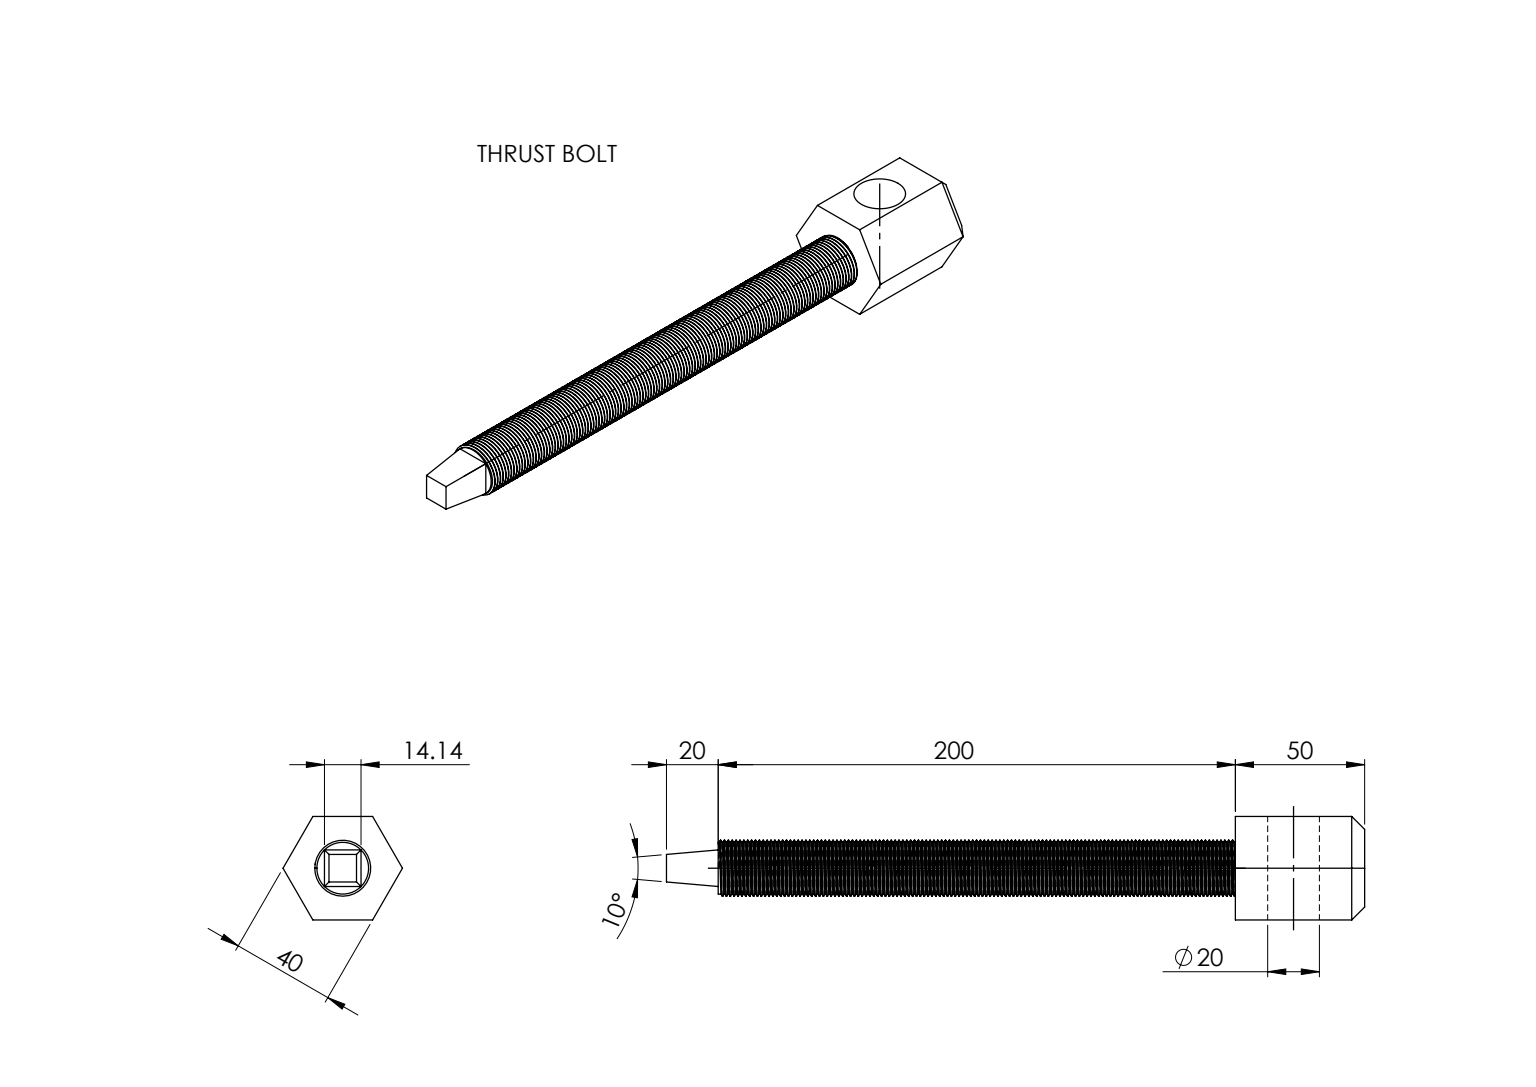
ISO-10303-21;
HEADER;
FILE_DESCRIPTION (('STEP AP203'),
    '1' );
FILE_NAME ('thrust bolt.step',
    '2026-09-28T05:57:06',
    ( '' ),
    ( '' ),
    'SwSTEP 2.0',
    'SolidWorks 2026',
    '' );
FILE_SCHEMA (( 'AUTOMOTIVE_DESIGN' ));
ENDSEC;

DATA;
#2=CARTESIAN_POINT ( 'NONE',  ( 10.81189881249999551, -6.242252689847874514, -42.15625000204836681 ) ) ;
#4=CARTESIAN_POINT ( 'NONE',  ( -10.81189881249999729, 1.324075727343319199E-15, -105.5937500020483810 ) ) ;
#5=CARTESIAN_POINT ( 'NONE',  ( 10.81189881249999729, 6.242252689847867408, -121.4062500020483810 ) ) ;
#6=VERTEX_POINT ( 'NONE', #18708 ) ;
#9=CARTESIAN_POINT ( 'NONE',  ( -5.000000000000003553, -8.660254037844383745, -26.49999999999996803 ) ) ;
#12=CARTESIAN_POINT ( 'NONE',  ( -2.293366432827344421E-15, -12.48450537969573659, -130.7187500020483810 ) ) ;
#14=CARTESIAN_POINT ( 'NONE',  ( -9.999999999999998224, 1.224646799147353059E-15, -200.0000000000000000 ) ) ;
#16=CARTESIAN_POINT ( 'NONE',  ( 5.000000000000000000, 8.660254037844385522, -194.1250000040967905 ) ) ;
#18=CARTESIAN_POINT ( 'NONE',  ( -2.293366432827344421E-15, -12.48450537969573659, -186.4062500020484094 ) ) ;
#19=CARTESIAN_POINT ( 'NONE',  ( 9.999999999999998224, 0.000000000000000000, -46.99999999999998579 ) ) ;
#20=CYLINDRICAL_SURFACE ( 'NONE', #32104, 9.999999999999998224 ) ;
#23=CARTESIAN_POINT ( 'NONE',  ( 5.405949406249999534, 9.363379034771803333, -58.09375000204835970 ) ) ;
#24=CARTESIAN_POINT ( 'NONE',  ( 7.644554776091147741E-16, 12.48450537969573659, -50.46875000204835970 ) ) ;
#26=CARTESIAN_POINT ( 'NONE',  ( 10.81189881249999551, -6.242252689847874514, -15.15625000204837036 ) ) ;
#30=CARTESIAN_POINT ( 'NONE',  ( 7.070501591499377789E-16, 11.54700538379251284, -105.1249999999999858 ) ) ;
#33=CARTESIAN_POINT ( 'NONE',  ( -5.000000000000003553, -8.660254037844383745, -27.99999999999996803 ) ) ;
#36=CARTESIAN_POINT ( 'NONE',  ( 10.81189881249999729, 6.242252689847867408, -113.9062500020483952 ) ) ;
#40=DIRECTION ( 'NONE',  ( -0.000000000000000000, -0.000000000000000000, 1.000000000000000000 ) ) ;
#42=ORIENTED_EDGE ( 'NONE', *, *, #41503, .T. ) ;
#43=CARTESIAN_POINT ( 'NONE',  ( 5.000000000000000000, 8.660254037844385522, -30.24999999999997158 ) ) ;
#44=CARTESIAN_POINT ( 'NONE',  ( 5.000000000000000000, 8.660254037844385522, -18.62500000409675494 ) ) ;
#45=CARTESIAN_POINT ( 'NONE',  ( -10.81189881249999729, 6.242252689847871849, -45.90625000204838102 ) ) ;
#46=CARTESIAN_POINT ( 'NONE',  ( 5.000000000000000000, 8.660254037844385522, -111.6250000040967763 ) ) ;
#48=CARTESIAN_POINT ( 'NONE',  ( 0.000000000000000000, 0.000000000000000000, -200.0000000000000000 ) ) ;
#49=CARTESIAN_POINT ( 'NONE',  ( -5.405949406250003975, -9.363379034771801557, -140.0312500020484094 ) ) ;
#50=CARTESIAN_POINT ( 'NONE',  ( -5.405949406250003975, -9.363379034771801557, -140.0312500020484094 ) ) ;
#51=CARTESIAN_POINT ( 'NONE',  ( -2.121150477449813534E-15, -11.54700538379251284, -123.8749999999999858 ) ) ;
#52=EDGE_LOOP ( 'NONE', ( #2862, #11579, #9941, #38309 ) ) ;
#53=ORIENTED_EDGE ( 'NONE', *, *, #4042, .F. ) ;
#54=ADVANCED_FACE ( 'NONE', ( #19135 ), #5555, .T. ) ;
#57=DIRECTION ( 'NONE',  ( -0.000000000000000000, -0.000000000000000000, 1.000000000000000000 ) ) ;
#58=CARTESIAN_POINT ( 'NONE',  ( -2.293366432827344421E-15, -12.48450537969573659, -177.2187500020484094 ) ) ;
#59=CARTESIAN_POINT ( 'NONE',  ( -10.81189881249999729, 1.324075727343319199E-15, -23.09375000204835615 ) ) ;
#60=CARTESIAN_POINT ( 'NONE',  ( -5.000000000000003553, -8.660254037844383745, -128.8750000040967905 ) ) ;
#61=CARTESIAN_POINT ( 'NONE',  ( 5.405949406249992428, -9.363379034771808662, -157.5937500020483810 ) ) ;
#62=CARTESIAN_POINT ( 'NONE',  ( 5.405949406249999534, 9.363379034771803333, -146.5937500020483810 ) ) ;
#63=CARTESIAN_POINT ( 'NONE',  ( 9.999999999999998224, 0.000000000000000000, -173.3750000040968189 ) ) ;
#66=CARTESIAN_POINT ( 'NONE',  ( 5.405949406249999534, 9.363379034771803333, -16.09375000204835260 ) ) ;
#72=CARTESIAN_POINT ( 'NONE',  ( -2.121150477449813534E-15, -11.54700538379251284, -17.37499999999997158 ) ) ;
#73=CARTESIAN_POINT ( 'NONE',  ( -5.405949406249996869, 9.363379034771805109, -72.84375000204838102 ) ) ;
#74=CARTESIAN_POINT ( 'NONE',  ( -5.405949406250003975, -9.363379034771801557, -39.53125000204838102 ) ) ;
#76=CARTESIAN_POINT ( 'NONE',  ( -2.121150477449813534E-15, -11.54700538379251284, -16.25000000409675849 ) ) ;
#78=VECTOR ( 'NONE', #7244, 1000.000000000000000 ) ;
#79=CARTESIAN_POINT ( 'NONE',  ( -5.000000000000003553, -8.660254037844383745, -130.0000000000000000 ) ) ;
#80=CARTESIAN_POINT ( 'NONE',  ( 7.644554776091147741E-16, 12.48450537969573659, -137.6562500020484094 ) ) ;
#82=CARTESIAN_POINT ( 'NONE',  ( -4.999999999999996447, 8.660254037844387298, -112.8750000040967763 ) ) ;
#85=( BOUNDED_CURVE ( )  B_SPLINE_CURVE ( 2, ( #33505, #9757, #39954, #703, #26171, #36305, #278 ),
 .UNSPECIFIED., .F., .F. ) 
 B_SPLINE_CURVE_WITH_KNOTS ( ( 3, 2, 2, 3 ),
 ( 0.9440298507462689948, 0.9452736318407963800, 0.9465174129353237653, 0.9477611940298510396 ),
 .UNSPECIFIED. ) 
 CURVE ( )  GEOMETRIC_REPRESENTATION_ITEM ( )  RATIONAL_B_SPLINE_CURVE ( ( 0.9999999999999641398, 0.8660254037844745678, 1.000000000000000000, 0.8660254037844387076, 1.000000000000000000, 0.8660254037844028474, 1.000000000000035971 ) ) 
 REPRESENTATION_ITEM ( '' )  );
#89=CARTESIAN_POINT ( 'NONE',  ( -10.81189881249999729, 1.324075727343319199E-15, -171.7812500020484094 ) ) ;
#90=CARTESIAN_POINT ( 'NONE',  ( 5.000000000000000000, 8.660254037844385522, -42.62500000409677625 ) ) ;
#93=CARTESIAN_POINT ( 'NONE',  ( 7.070501591499376803E-16, 11.54700538379251284, -101.0000000040967905 ) ) ;
#94=CARTESIAN_POINT ( 'NONE',  ( -10.81189881249999729, 1.324075727343319199E-15, -164.2812500020484094 ) ) ;
#95=CARTESIAN_POINT ( 'NONE',  ( 5.405949406249999534, 9.363379034771803333, -134.5937500020483810 ) ) ;
#96=DIRECTION ( 'NONE',  ( -0.000000000000000000, -0.000000000000000000, 1.000000000000000000 ) ) ;
#97=CARTESIAN_POINT ( 'NONE',  ( -9.999999999999998224, 1.224646799147353059E-15, -196.2500000000000000 ) ) ;
#98=ORIENTED_EDGE ( 'NONE', *, *, #19816, .T. ) ;
#100=VECTOR ( 'NONE', #1628, 1000.000000000000000 ) ;
#102=CARTESIAN_POINT ( 'NONE',  ( 5.405949406249999534, 9.363379034771803333, -70.28125000204838102 ) ) ;
#103=ORIENTED_EDGE ( 'NONE', *, *, #9830, .F. ) ;
#105=EDGE_CURVE ( 'NONE', #39394, #30784, #41849, .T. ) ;
#106=CARTESIAN_POINT ( 'NONE',  ( -2.293366432827344421E-15, -12.48450537969573659, -121.7187500020483952 ) ) ;
#107=VERTEX_POINT ( 'NONE', #25626 ) ;
#109=EDGE_CURVE ( 'NONE', #35866, #23028, #3547, .T. ) ;
#110=CARTESIAN_POINT ( 'NONE',  ( 10.81189881249999551, -6.242252689847874514, -23.96875000204836681 ) ) ;
#111=CARTESIAN_POINT ( 'NONE',  ( 10.81189881249999551, -6.242252689847874514, -197.9687500020484094 ) ) ;
#112=AXIS2_PLACEMENT_3D ( 'NONE', #13766, #17434, #17222 ) ;
#113=CARTESIAN_POINT ( 'NONE',  ( 10.81189881249999907, 6.242252689847868297, -50.71875000204835970 ) ) ;
#114=ADVANCED_FACE ( 'NONE', ( #26883 ), #29920, .T. ) ;
#117=CARTESIAN_POINT ( 'NONE',  ( -5.405949406249996869, 9.363379034771805109, -182.3437500020483810 ) ) ;
#118=CARTESIAN_POINT ( 'NONE',  ( 10.81189881249999729, 0.000000000000000000, -166.3437500020484094 ) ) ;
#123=FACE_OUTER_BOUND ( 'NONE', #11010, .T. ) ;
#125=CARTESIAN_POINT ( 'NONE',  ( 5.405949406249992428, -9.363379034771808662, -99.09375000204838102 ) ) ;
#127=CARTESIAN_POINT ( 'NONE',  ( -5.405949406250003975, -9.363379034771801557, -63.53125000204837391 ) ) ;
#129=CARTESIAN_POINT ( 'NONE',  ( 7.644554776091147741E-16, 12.48450537969573659, -164.6562500020484094 ) ) ;
#131=CARTESIAN_POINT ( 'NONE',  ( -9.999999999999998224, 1.224646799147353059E-15, -136.6250000040967620 ) ) ;
#137=ADVANCED_FACE ( 'NONE', ( #29707 ), #23658, .T. ) ;
#139=CARTESIAN_POINT ( 'NONE',  ( -10.81189881249999729, 1.324075727343319199E-15, -195.7812500020484094 ) ) ;
#140=LINE ( 'NONE', #33368, #22679 ) ;
#143=CARTESIAN_POINT ( 'NONE',  ( -4.999999999999996447, 8.660254037844387298, -58.49999999999997158 ) ) ;
#145=CARTESIAN_POINT ( 'NONE',  ( -5.000000000000003553, -8.660254037844383745, -62.87500000409676204 ) ) ;
#146=CARTESIAN_POINT ( 'NONE',  ( 7.070501591499376803E-16, 11.54700538379251284, -102.1250000000000000 ) ) ;
#147=CARTESIAN_POINT ( 'NONE',  ( 9.999999999999998224, 0.000000000000000000, -144.5000000000000000 ) ) ;
#149=CARTESIAN_POINT ( 'NONE',  ( -10.81189881249999729, -6.242252689847864744, -62.15625000204838813 ) ) ;
#152=CARTESIAN_POINT ( 'NONE',  ( 9.999999999999998224, 0.000000000000000000, -200.0000000000000000 ) ) ;
#153=CARTESIAN_POINT ( 'NONE',  ( -10.81189881249999907, -6.242252689847864744, -188.1562500020484094 ) ) ;
#155=CARTESIAN_POINT ( 'NONE',  ( 7.644554776091147741E-16, 12.48450537969573659, -0.9687500020483524876 ) ) ;
#157=( BOUNDED_CURVE ( )  B_SPLINE_CURVE ( 2, ( #19226, #13579, #9933, #13155, #20069, #32416, #9303 ),
 .UNSPECIFIED., .F., .F. ) 
 B_SPLINE_CURVE_WITH_KNOTS ( ( 3, 2, 2, 3 ),
 ( 0.3955223880597015795, 0.3967661691542289648, 0.3980099502487563501, 0.3992537313432836799 ),
 .UNSPECIFIED. ) 
 CURVE ( )  GEOMETRIC_REPRESENTATION_ITEM ( )  RATIONAL_B_SPLINE_CURVE ( ( 0.9999999999999880096, 0.8660254037844506980, 1.000000000000000000, 0.8660254037844387076, 1.000000000000000000, 0.8660254037844267172, 1.000000000000011990 ) ) 
 REPRESENTATION_ITEM ( '' )  );
#160=CARTESIAN_POINT ( 'NONE',  ( -10.00000000000000000, -5.773502691896251982, -167.6249999999999716 ) ) ;
#162=CARTESIAN_POINT ( 'NONE',  ( -2.293366432827344421E-15, -12.48450537969573659, -94.90625000204838102 ) ) ;
#163=ORIENTED_EDGE ( 'NONE', *, *, #36914, .F. ) ;
#164=CYLINDRICAL_SURFACE ( 'NONE', #41388, 9.999999999999998224 ) ;
#166=ORIENTED_EDGE ( 'NONE', *, *, #11173, .F. ) ;
#167=ORIENTED_EDGE ( 'NONE', *, *, #19593, .F. ) ;
#169=CARTESIAN_POINT ( 'NONE',  ( 10.81189881249999729, 0.000000000000000000, -31.34375000204836681 ) ) ;
#170=CARTESIAN_POINT ( 'NONE',  ( 10.81189881249999551, -6.242252689847874514, -22.65625000204837391 ) ) ;
#172=CARTESIAN_POINT ( 'NONE',  ( 5.405949406249999534, 9.363379034771803333, -71.59375000204836681 ) ) ;
#173=CARTESIAN_POINT ( 'NONE',  ( 0.000000000000000000, 0.000000000000000000, -200.0000000000000000 ) ) ;
#174=CARTESIAN_POINT ( 'NONE',  ( 5.405949406249992428, -9.363379034771808662, -192.0937500020484094 ) ) ;
#175=CARTESIAN_POINT ( 'NONE',  ( -2.293366432827344421E-15, -12.48450537969573659, -150.2187500020483810 ) ) ;
#176=CARTESIAN_POINT ( 'NONE',  ( 5.000000000000000000, 8.660254037844385522, -99.24999999999998579 ) ) ;
#179=CARTESIAN_POINT ( 'NONE',  ( -10.00000000000000000, -5.773502691896251982, -4.096743805827756695E-09 ) ) ;
#180=VECTOR ( 'NONE', #38036, 1000.000000000000000 ) ;
#181=CARTESIAN_POINT ( 'NONE',  ( -10.00000000000154188, 5.773502691895366468, -49.75000000409671230 ) ) ;
#182=ADVANCED_FACE ( 'NONE', ( #33380 ), #3374, .T. ) ;
#183=CARTESIAN_POINT ( 'NONE',  ( -10.81189881249999907, -6.242252689847864744, -123.4687500020483810 ) ) ;
#184=DIRECTION ( 'NONE',  ( -0.000000000000000000, -0.000000000000000000, 1.000000000000000000 ) ) ;
#185=CARTESIAN_POINT ( 'NONE',  ( 5.405949406249999534, 9.363379034771803333, -91.28125000204838102 ) ) ;
#186=CARTESIAN_POINT ( 'NONE',  ( 5.405949406249999534, 9.363379034771803333, -106.0937500020483810 ) ) ;
#189=CARTESIAN_POINT ( 'NONE',  ( 10.00000000000000000, 5.773502691896255534, -161.2500000040967905 ) ) ;
#195=FACE_OUTER_BOUND ( 'NONE', #14094, .T. ) ;
#197=CARTESIAN_POINT ( 'NONE',  ( 10.00000000000000000, 5.773502691896255534, -81.37499999999998579 ) ) ;
#199=CARTESIAN_POINT ( 'NONE',  ( -9.999999999999998224, 5.773502691896259087, -91.75000000409677625 ) ) ;
#202=CARTESIAN_POINT ( 'NONE',  ( -2.293366432827344421E-15, -12.48450537969573659, -84.40625000204838102 ) ) ;
#203=ORIENTED_EDGE ( 'NONE', *, *, #41316, .F. ) ;
#204=( BOUNDED_CURVE ( )  B_SPLINE_CURVE ( 2, ( #13200, #12782, #19064, #9770, #9143, #32665, #29001 ),
 .UNSPECIFIED., .F., .F. ) 
 B_SPLINE_CURVE_WITH_KNOTS ( ( 3, 2, 2, 3 ),
 ( 0.5373134328358210032, 0.5385572139303483885, 0.5398009950248757738, 0.5410447761194030480 ),
 .UNSPECIFIED. ) 
 CURVE ( )  GEOMETRIC_REPRESENTATION_ITEM ( )  RATIONAL_B_SPLINE_CURVE ( ( 0.9999999999999880096, 0.8660254037844506980, 1.000000000000000000, 0.8660254037844387076, 1.000000000000000000, 0.8660254037844267172, 1.000000000000011990 ) ) 
 REPRESENTATION_ITEM ( '' )  );
#209=CARTESIAN_POINT ( 'NONE',  ( 5.000000000000000000, 8.660254037844385522, -7.749999999999978684 ) ) ;
#210=CARTESIAN_POINT ( 'NONE',  ( -5.000000000000003553, -8.660254037844383745, -142.0000000000000000 ) ) ;
#211=CARTESIAN_POINT ( 'NONE',  ( -9.999999999999998224, 1.224646799147353059E-15, -200.0000000000000000 ) ) ;
#213=VECTOR ( 'NONE', #33847, 1000.000000000000000 ) ;
#214=CARTESIAN_POINT ( 'NONE',  ( 10.00000000000000000, 5.773502691896255534, -189.3750000000000000 ) ) ;
#216=CARTESIAN_POINT ( 'NONE',  ( 5.405949406249992428, -9.363379034771808662, -115.7812500020483952 ) ) ;
#217=ORIENTED_EDGE ( 'NONE', *, *, #1701, .T. ) ;
#219=CARTESIAN_POINT ( 'NONE',  ( -5.405949406249996869, 9.363379034771805109, -47.53125000204838813 ) ) ;
#221=CARTESIAN_POINT ( 'NONE',  ( -10.81189881249999907, -6.242252689847864744, -91.96875000204838102 ) ) ;
#222=CARTESIAN_POINT ( 'NONE',  ( -10.81189881249999729, -6.242252689847864744, -120.6562500020483810 ) ) ;
#224=CARTESIAN_POINT ( 'NONE',  ( -9.999999999999998224, 1.224646799147353059E-15, -112.2499999999999858 ) ) ;
#225=CARTESIAN_POINT ( 'NONE',  ( 4.999999999999992006, -8.660254037844389075, -116.2499999999999858 ) ) ;
#228=CARTESIAN_POINT ( 'NONE',  ( -10.81189881249999729, 6.242252689847871849, -129.7187500020483810 ) ) ;
#230=CYLINDRICAL_SURFACE ( 'NONE', #27006, 9.999999999999998224 ) ;
#232=CARTESIAN_POINT ( 'NONE',  ( 5.000000000000000000, 8.660254037844385522, -189.6250000040967905 ) ) ;
#234=CARTESIAN_POINT ( 'NONE',  ( -2.293366432827344421E-15, -12.48450537969573659, -189.4062500020484094 ) ) ;
#239=CARTESIAN_POINT ( 'NONE',  ( 5.405949406249999534, 9.363379034771803333, -64.09375000204836681 ) ) ;
#240=CARTESIAN_POINT ( 'NONE',  ( 5.405949406249992428, -9.363379034771808662, -51.09375000204835260 ) ) ;
#242=CARTESIAN_POINT ( 'NONE',  ( 10.81189881249999729, 0.000000000000000000, -18.03125000204835970 ) ) ;
#244=CARTESIAN_POINT ( 'NONE',  ( -5.000000000000003553, -8.660254037844383745, -124.3750000040967763 ) ) ;
#246=CARTESIAN_POINT ( 'NONE',  ( 9.999999999999998224, 0.000000000000000000, -108.4999999999999858 ) ) ;
#248=FACE_OUTER_BOUND ( 'NONE', #19771, .T. ) ;
#251=CARTESIAN_POINT ( 'NONE',  ( 5.405949406249999534, 9.363379034771803333, -112.2812500020483952 ) ) ;
#252=EDGE_CURVE ( 'NONE', #311, #38192, #33161, .T. ) ;
#258=VERTEX_POINT ( 'NONE', #36387 ) ;
#259=CARTESIAN_POINT ( 'NONE',  ( -4.999999999999996447, 8.660254037844387298, -35.99999999999997868 ) ) ;
#260=CARTESIAN_POINT ( 'NONE',  ( -5.000000000000003553, -8.660254037844383745, -20.87500000409675494 ) ) ;
#261=CARTESIAN_POINT ( 'NONE',  ( -10.81189881249999729, 6.242252689847871849, -39.90625000204835970 ) ) ;
#262=CARTESIAN_POINT ( 'NONE',  ( 9.999999999999998224, 0.000000000000000000, -35.37500000409676915 ) ) ;
#264=LINE ( 'NONE', #16194, #5231 ) ;
#265=CARTESIAN_POINT ( 'NONE',  ( 5.405949406249992428, -9.363379034771808662, -145.7812500020483810 ) ) ;
#266=CARTESIAN_POINT ( 'NONE',  ( -2.121150477449813534E-15, -11.54700538379251284, -110.3749999999999858 ) ) ;
#267=EDGE_LOOP ( 'NONE', ( #11226, #4653, #4074, #29262 ) ) ;
#271=DIRECTION ( 'NONE',  ( -0.000000000000000000, -0.000000000000000000, 1.000000000000000000 ) ) ;
#272=CARTESIAN_POINT ( 'NONE',  ( 7.644554776091147741E-16, 12.48450537969573659, -170.4687500020483810 ) ) ;
#273=CARTESIAN_POINT ( 'NONE',  ( -10.81189881249999907, -6.242252689847864744, -21.46875000204836681 ) ) ;
#275=CARTESIAN_POINT ( 'NONE',  ( -10.81189881249999729, 1.324075727343319199E-15, -153.5937500020483810 ) ) ;
#276=CARTESIAN_POINT ( 'NONE',  ( 10.81189881249999907, 6.242252689847868297, -143.7187500020483810 ) ) ;
#277=( BOUNDED_CURVE ( )  B_SPLINE_CURVE ( 2, ( #35244, #34601, #35030, #41688, #5459, #14928, #5032 ),
 .UNSPECIFIED., .F., .F. ) 
 B_SPLINE_CURVE_WITH_KNOTS ( ( 3, 2, 2, 3 ),
 ( 0.4962686567164180107, 0.4975124378109453960, 0.4987562189054727257, 0.5000000000000001110 ),
 .UNSPECIFIED. ) 
 CURVE ( )  GEOMETRIC_REPRESENTATION_ITEM ( )  RATIONAL_B_SPLINE_CURVE ( ( 0.9999999999999880096, 0.8660254037844506980, 1.000000000000000000, 0.8660254037844387076, 1.000000000000000000, 0.8660254037844267172, 1.000000000000011990 ) ) 
 REPRESENTATION_ITEM ( '' )  );
#278=CARTESIAN_POINT ( 'NONE',  ( 9.999999999999998224, 0.000000000000000000, -8.375000004096744277 ) ) ;
#281=CARTESIAN_POINT ( 'NONE',  ( -10.81189881249999729, 6.242252689847871849, -6.718750002048347270 ) ) ;
#284=CARTESIAN_POINT ( 'NONE',  ( 7.070501591499376803E-16, 11.54700538379251284, -120.1249999999999858 ) ) ;
#287=CARTESIAN_POINT ( 'NONE',  ( -5.405949406250003975, -9.363379034771801557, -70.84375000204836681 ) ) ;
#288=CARTESIAN_POINT ( 'NONE',  ( -10.81189881249999907, -6.242252689847864744, -44.15625000204838102 ) ) ;
#290=CARTESIAN_POINT ( 'NONE',  ( -1.040834085586084257E-14, -20.00000000000000355, 32.49999999999999289 ) ) ;
#292=CARTESIAN_POINT ( 'NONE',  ( 7.070501591499377789E-16, 11.54700538379251284, -127.6249999999999858 ) ) ;
#293=CARTESIAN_POINT ( 'NONE',  ( -5.405949406250003975, -9.363379034771801557, -138.5312500020484094 ) ) ;
#294=CARTESIAN_POINT ( 'NONE',  ( 9.999999999999998224, 0.000000000000000000, -150.5000000000000000 ) ) ;
#295=CARTESIAN_POINT ( 'NONE',  ( 9.999999999999996447, -5.773502691896262640, -118.0000000040967905 ) ) ;
#300=LINE ( 'NONE', #39765, #14626 ) ;
#301=CARTESIAN_POINT ( 'NONE',  ( -10.81189881249999729, 6.242252689847871849, -162.9062500020484094 ) ) ;
#302=CARTESIAN_POINT ( 'NONE',  ( -10.00000000000000000, -5.773502691896251982, -45.00000000409676204 ) ) ;
#304=CARTESIAN_POINT ( 'NONE',  ( 9.999999999999998224, 0.000000000000000000, -155.3750000040967905 ) ) ;
#306=CARTESIAN_POINT ( 'NONE',  ( 9.999999999999479527, 5.773502691896553074, -73.87499999999994316 ) ) ;
#307=CARTESIAN_POINT ( 'NONE',  ( -5.405949406249996869, 9.363379034771805109, -161.5312500020484094 ) ) ;
#308=CARTESIAN_POINT ( 'NONE',  ( 5.405949406249992428, -9.363379034771808662, -136.5937500020483810 ) ) ;
#309=CARTESIAN_POINT ( 'NONE',  ( -9.999999999999998224, 1.224646799147353059E-15, -100.2499999999999858 ) ) ;
#310=CARTESIAN_POINT ( 'NONE',  ( -5.000000000000003553, -8.660254037844383745, -196.0000000000000000 ) ) ;
#311=VERTEX_POINT ( 'NONE', #39824 ) ;
#313=CARTESIAN_POINT ( 'NONE',  ( 5.405949406249992428, -9.363379034771808662, -70.78125000204838102 ) ) ;
#314=ORIENTED_EDGE ( 'NONE', *, *, #31517, .F. ) ;
#316=CARTESIAN_POINT ( 'NONE',  ( -5.405949406249996869, 9.363379034771805109, -117.8437500020483810 ) ) ;
#317=VERTEX_POINT ( 'NONE', #16084 ) ;
#318=VERTEX_POINT ( 'NONE', #29279 ) ;
#319=CARTESIAN_POINT ( 'NONE',  ( 10.81189881249999551, -6.242252689847874514, -17.96875000204837036 ) ) ;
#321=CARTESIAN_POINT ( 'NONE',  ( 5.405949406249999534, 9.363379034771803333, -196.0937500020484094 ) ) ;
#322=CARTESIAN_POINT ( 'NONE',  ( -10.81189881249999907, -6.242252689847864744, -45.46875000204837391 ) ) ;
#323=CARTESIAN_POINT ( 'NONE',  ( 0.000000000000000000, 0.000000000000000000, -200.0000000000000000 ) ) ;
#324=DIRECTION ( 'NONE',  ( 1.000000000000000000, 0.000000000000000000, 0.000000000000000000 ) ) ;
#325=CARTESIAN_POINT ( 'NONE',  ( -10.81189881249999729, -6.242252689847864744, -183.4687500020484094 ) ) ;
#326=CARTESIAN_POINT ( 'NONE',  ( 10.81189881249999907, 6.242252689847868297, -170.7187500020483810 ) ) ;
#329=CARTESIAN_POINT ( 'NONE',  ( -9.999999999999998224, 1.224646799147353059E-15, -105.1250000040967763 ) ) ;
#333=CARTESIAN_POINT ( 'NONE',  ( -10.81189881249999729, 6.242252689847871849, -96.71875000204838102 ) ) ;
#334=CARTESIAN_POINT ( 'NONE',  ( -5.405949406250003975, -9.363379034771801557, -68.03125000204838102 ) ) ;
#337=CARTESIAN_POINT ( 'NONE',  ( -10.81189881249999907, -6.242252689847864744, -119.1562500020484237 ) ) ;
#338=CARTESIAN_POINT ( 'NONE',  ( 7.644554776091147741E-16, 12.48450537969573659, -163.1562500020483810 ) ) ;
#340=CARTESIAN_POINT ( 'NONE',  ( 5.000000000000000000, 8.660254037844385522, -137.1250000040967620 ) ) ;
#343=AXIS2_PLACEMENT_3D ( 'NONE', #16719, #354, #20184 ) ;
#346=CARTESIAN_POINT ( 'NONE',  ( -10.81189881249999729, 6.242252689847871849, -189.9062500020484379 ) ) ;
#350=CARTESIAN_POINT ( 'NONE',  ( 9.999999999999998224, 0.000000000000000000, -57.49999999999996447 ) ) ;
#352=CARTESIAN_POINT ( 'NONE',  ( -5.000000000000003553, -8.660254037844383745, -67.37500000409676204 ) ) ;
#353=EDGE_CURVE ( 'NONE', #4966, #40396, #23982, .T. ) ;
#354=DIRECTION ( 'NONE',  ( -0.000000000000000000, -0.000000000000000000, 1.000000000000000000 ) ) ;
#355=CARTESIAN_POINT ( 'NONE',  ( 9.999999999999998224, 0.000000000000000000, -71.37500000409677625 ) ) ;
#356=EDGE_CURVE ( 'NONE', #32390, #11765, #10047, .T. ) ;
#358=CARTESIAN_POINT ( 'NONE',  ( -5.405949406249996869, 9.363379034771805109, -61.03125000204837391 ) ) ;
#359=ADVANCED_FACE ( 'NONE', ( #16509 ), #6406, .T. ) ;
#362=DIRECTION ( 'NONE',  ( -0.000000000000000000, -0.000000000000000000, 1.000000000000000000 ) ) ;
#363=CARTESIAN_POINT ( 'NONE',  ( 10.81189881249999729, 0.000000000000000000, -184.5312500020484094 ) ) ;
#365=CARTESIAN_POINT ( 'NONE',  ( 5.405949406249999534, 9.363379034771803333, -1.093750002048365921 ) ) ;
#367=CARTESIAN_POINT ( 'NONE',  ( 4.999999999999992006, -8.660254037844389075, -45.74999999999998579 ) ) ;
#370=CARTESIAN_POINT ( 'NONE',  ( 7.070501591499377789E-16, 11.54700538379251284, -168.1250000000000000 ) ) ;
#371=CARTESIAN_POINT ( 'NONE',  ( -9.999999999999742428, -5.773502691896402084, -122.6249999999999858 ) ) ;
#372=CARTESIAN_POINT ( 'NONE',  ( 7.644554776091147741E-16, 12.48450537969573659, -92.65625000204839523 ) ) ;
#373=ORIENTED_EDGE ( 'NONE', *, *, #16628, .T. ) ;
#375=EDGE_CURVE ( 'NONE', #30674, #33916, #10463, .T. ) ;
#377=ORIENTED_EDGE ( 'NONE', *, *, #20105, .T. ) ;
#379=CARTESIAN_POINT ( 'NONE',  ( -5.405949406250003975, -9.363379034771801557, -36.34375000204836681 ) ) ;
#381=CARTESIAN_POINT ( 'NONE',  ( 10.81189881249999729, 0.000000000000000000, -24.03125000204836681 ) ) ;
#382=EDGE_CURVE ( 'NONE', #28565, #29057, #16244, .T. ) ;
#383=CARTESIAN_POINT ( 'NONE',  ( 10.81189881249999551, -6.242252689847874514, -70.46875000204840944 ) ) ;
#384=LINE ( 'NONE', #32964, #19456 ) ;
#386=CARTESIAN_POINT ( 'NONE',  ( 10.81189881249999907, 6.242252689847868297, -193.2187500020484094 ) ) ;
#387=CARTESIAN_POINT ( 'NONE',  ( 10.81189881249999729, 0.000000000000000000, -149.8437500020483810 ) ) ;
#388=CARTESIAN_POINT ( 'NONE',  ( 5.000000000000000000, 8.660254037844385522, -132.6250000040967620 ) ) ;
#389=DIRECTION ( 'NONE',  ( -0.000000000000000000, -0.000000000000000000, 1.000000000000000000 ) ) ;
#391=CARTESIAN_POINT ( 'NONE',  ( 7.070501591499377789E-16, 11.54700538379251284, -2.000000004096753159 ) ) ;
#392=CARTESIAN_POINT ( 'NONE',  ( 5.405949406249992428, -9.363379034771808662, -124.5937500020483952 ) ) ;
#394=CARTESIAN_POINT ( 'NONE',  ( 10.81189881249999551, -6.242252689847874514, -93.15625000204838102 ) ) ;
#395=CARTESIAN_POINT ( 'NONE',  ( 10.81189881249999729, 6.242252689847867408, -109.2187500020483810 ) ) ;
#398=CARTESIAN_POINT ( 'NONE',  ( 9.999999999999998224, 0.000000000000000000, -165.8750000040967905 ) ) ;
#404=CARTESIAN_POINT ( 'NONE',  ( -5.000000000000003553, -8.660254037844383745, -108.9999999999999858 ) ) ;
#406=CARTESIAN_POINT ( 'NONE',  ( -5.000000000000003553, -8.660254037844383745, -84.99999999999997158 ) ) ;
#408=CARTESIAN_POINT ( 'NONE',  ( -4.999999999999996447, 8.660254037844387298, -90.37500000409677625 ) ) ;
#409=VECTOR ( 'NONE', #32686, 1000.000000000000000 ) ;
#411=CARTESIAN_POINT ( 'NONE',  ( -4.999999999999996447, 8.660254037844387298, -115.4999999999999858 ) ) ;
#413=CARTESIAN_POINT ( 'NONE',  ( -10.81189881249999729, 6.242252689847871849, -84.90625000204838102 ) ) ;
#414=VERTEX_POINT ( 'NONE', #34229 ) ;
#417=CARTESIAN_POINT ( 'NONE',  ( 9.999999999999998224, 0.000000000000000000, -48.49999999999998579 ) ) ;
#420=CARTESIAN_POINT ( 'NONE',  ( 4.999999999999992006, -8.660254037844389075, -6.749999999999978684 ) ) ;
#421=CARTESIAN_POINT ( 'NONE',  ( -2.121150477449813534E-15, -11.54700538379251284, -141.8750000000000000 ) ) ;
#424=CARTESIAN_POINT ( 'NONE',  ( 4.999999999999992006, -8.660254037844389075, -194.2500000000000000 ) ) ;
#425=CARTESIAN_POINT ( 'NONE',  ( 7.070501591499376803E-16, 11.54700538379251284, -96.12500000000000000 ) ) ;
#426=CARTESIAN_POINT ( 'NONE',  ( -5.405949406250003975, -9.363379034771801557, -117.5312500020483952 ) ) ;
#427=ORIENTED_EDGE ( 'NONE', *, *, #34188, .T. ) ;
#428=CARTESIAN_POINT ( 'NONE',  ( 9.999999999999998224, 0.000000000000000000, -13.99999999999995737 ) ) ;
#429=AXIS2_PLACEMENT_3D ( 'NONE', #40358, #23353, #23565 ) ;
#431=EDGE_CURVE ( 'NONE', #17742, #13704, #21254, .T. ) ;
#432=AXIS2_PLACEMENT_3D ( 'NONE', #22811, #9638, #19552 ) ;
#433=CARTESIAN_POINT ( 'NONE',  ( 7.644554776091147741E-16, 12.48450537969573659, -49.15625000204837391 ) ) ;
#435=CARTESIAN_POINT ( 'NONE',  ( -10.81189881249999729, 6.242252689847871849, -96.71875000204838102 ) ) ;
#436=CARTESIAN_POINT ( 'NONE',  ( 5.405949406249992428, -9.363379034771808662, -121.7812500020483952 ) ) ;
#437=VERTEX_POINT ( 'NONE', #1633 ) ;
#439=CARTESIAN_POINT ( 'NONE',  ( -10.00000000000154188, 5.773502691895366468, -51.25000000409671941 ) ) ;
#440=CARTESIAN_POINT ( 'NONE',  ( 4.999999999999992006, -8.660254037844389075, -125.6250000040967620 ) ) ;
#443=CARTESIAN_POINT ( 'NONE',  ( -10.81189881249999729, 6.242252689847871849, -135.7187500020483810 ) ) ;
#445=CARTESIAN_POINT ( 'NONE',  ( -5.000000000000003553, -8.660254037844383745, -44.49999999999998579 ) ) ;
#447=CARTESIAN_POINT ( 'NONE',  ( -5.000000000000003553, -8.660254037844383745, -184.3750000040967905 ) ) ;
#449=CARTESIAN_POINT ( 'NONE',  ( -10.81189881249999729, -6.242252689847864744, -174.6562500020484094 ) ) ;
#451=CARTESIAN_POINT ( 'NONE',  ( 5.000000000000000000, 8.660254037844385522, -3.249999999999975131 ) ) ;
#452=CARTESIAN_POINT ( 'NONE',  ( 9.999999999999676703, 5.773502691896441164, -185.2500000040967620 ) ) ;
#454=CARTESIAN_POINT ( 'NONE',  ( 7.644554776091147741E-16, 12.48450537969573659, -59.46875000204837391 ) ) ;
#455=CARTESIAN_POINT ( 'NONE',  ( 10.81189881249999729, 0.000000000000000000, -40.34375000204837391 ) ) ;
#457=CARTESIAN_POINT ( 'NONE',  ( 10.81189881249999729, 0.000000000000000000, -19.53125000204835970 ) ) ;
#461=CARTESIAN_POINT ( 'NONE',  ( 4.999999999999992006, -8.660254037844389075, -105.7499999999999858 ) ) ;
#464=AXIS2_PLACEMENT_3D ( 'NONE', #4502, #8399, #24809 ) ;
#467=CARTESIAN_POINT ( 'NONE',  ( 7.644554776091147741E-16, 12.48450537969573659, -110.6562500020483810 ) ) ;
#468=VERTEX_POINT ( 'NONE', #30351 ) ;
#469=FACE_OUTER_BOUND ( 'NONE', #25673, .T. ) ;
#474=CARTESIAN_POINT ( 'NONE',  ( -9.999999999999998224, 1.224646799147353059E-15, -32.74999999999997158 ) ) ;
#475=CARTESIAN_POINT ( 'NONE',  ( 7.070501591499377789E-16, 11.54700538379251284, -21.50000000409676559 ) ) ;
#476=CARTESIAN_POINT ( 'NONE',  ( -2.293366432827344421E-15, -12.48450537969573659, -42.40625000204837391 ) ) ;
#477=DIRECTION ( 'NONE',  ( -0.000000000000000000, -0.000000000000000000, 1.000000000000000000 ) ) ;
#479=CARTESIAN_POINT ( 'NONE',  ( 7.070501591499376803E-16, 11.54700538379251284, -57.50000000409677625 ) ) ;
#480=EDGE_CURVE ( 'NONE', #37390, #31108, #781, .T. ) ;
#481=CARTESIAN_POINT ( 'NONE',  ( -5.405949406249996869, 9.363379034771805109, -145.0312500020483810 ) ) ;
#482=CARTESIAN_POINT ( 'NONE',  ( -2.121150477449813534E-15, -11.54700538379251284, -15.87499999999997868 ) ) ;
#485=CARTESIAN_POINT ( 'NONE',  ( 9.999999999999998224, 0.000000000000000000, -114.4999999999999858 ) ) ;
#486=EDGE_CURVE ( 'NONE', #18454, #8390, #35575, .T. ) ;
#487=CYLINDRICAL_SURFACE ( 'NONE', #21478, 9.999999999999998224 ) ;
#488=CARTESIAN_POINT ( 'NONE',  ( 10.81189881249999551, -6.242252689847874514, -176.9687500020483810 ) ) ;
#491=CARTESIAN_POINT ( 'NONE',  ( -5.405949406249996869, 9.363379034771805109, -26.34375000204835970 ) ) ;
#492=CARTESIAN_POINT ( 'NONE',  ( 10.00000000000000000, 5.773502691896255534, -170.2500000040967905 ) ) ;
#494=CARTESIAN_POINT ( 'NONE',  ( -5.405949406249996869, 9.363379034771805109, -158.3437500020483810 ) ) ;
#495=CARTESIAN_POINT ( 'NONE',  ( 10.81189881249999907, 6.242252689847868297, -133.2187500020483810 ) ) ;
#496=CARTESIAN_POINT ( 'NONE',  ( -2.121150477449813534E-15, -11.54700538379251284, -88.25000000409677625 ) ) ;
#500=CARTESIAN_POINT ( 'NONE',  ( 5.405949406249999534, 9.363379034771803333, -10.09375000204834549 ) ) ;
#503=CARTESIAN_POINT ( 'NONE',  ( 10.00000000000051159, -5.773502691895965988, -178.0000000040967336 ) ) ;
#505=CARTESIAN_POINT ( 'NONE',  ( -10.81189881249999729, 1.324075727343319199E-15, -86.09375000204836681 ) ) ;
#506=CARTESIAN_POINT ( 'NONE',  ( -5.405949406249996869, 9.363379034771805109, -74.34375000204838102 ) ) ;
#507=CARTESIAN_POINT ( 'NONE',  ( -5.405949406250003975, -9.363379034771801557, -41.03125000204838102 ) ) ;
#511=CARTESIAN_POINT ( 'NONE',  ( -10.00000000000000000, -5.773502691896251982, -130.1250000000000000 ) ) ;
#512=CARTESIAN_POINT ( 'NONE',  ( 7.644554776091147741E-16, 12.48450537969573659, -140.6562500020484094 ) ) ;
#513=CARTESIAN_POINT ( 'NONE',  ( 0.000000000000000000, 0.000000000000000000, -200.0000000000000000 ) ) ;
#515=CARTESIAN_POINT ( 'NONE',  ( 5.405949406249992428, -9.363379034771808662, -18.28125000204835970 ) ) ;
#520=CARTESIAN_POINT ( 'NONE',  ( -10.81189881249999907, -6.242252689847864744, -167.1562500020483810 ) ) ;
#521=CARTESIAN_POINT ( 'NONE',  ( 7.070501591499377789E-16, 11.54700538379251284, -44.00000000409676204 ) ) ;
#523=EDGE_CURVE ( 'NONE', #21106, #26311, #40206, .T. ) ;
#524=CARTESIAN_POINT ( 'NONE',  ( 5.405949406249999534, 9.363379034771803333, -164.7812500020484094 ) ) ;
#525=CARTESIAN_POINT ( 'NONE',  ( -2.293366432827344421E-15, -12.48450537969573659, -135.2187500020483810 ) ) ;
#527=EDGE_LOOP ( 'NONE', ( #24852, #22930, #27645, #38076 ) ) ;
#529=CARTESIAN_POINT ( 'NONE',  ( -10.81189881249999907, -6.242252689847864744, -62.15625000204838102 ) ) ;
#531=CARTESIAN_POINT ( 'NONE',  ( 5.405949406249992428, -9.363379034771808662, -115.5937500020483810 ) ) ;
#532=ORIENTED_EDGE ( 'NONE', *, *, #29928, .F. ) ;
#533=( BOUNDED_CURVE ( )  B_SPLINE_CURVE ( 2, ( #18878, #5294, #15199, #35083, #38941, #2694, #21690 ),
 .UNSPECIFIED., .F., .F. ) 
 B_SPLINE_CURVE_WITH_KNOTS ( ( 3, 2, 2, 3 ),
 ( 0.02611940298507465369, 0.02736318407960201815, 0.02860696517412938261, 0.02985074626865674360 ),
 .UNSPECIFIED. ) 
 CURVE ( )  GEOMETRIC_REPRESENTATION_ITEM ( )  RATIONAL_B_SPLINE_CURVE ( ( 0.9999999999999970024, 0.8660254037844417052, 1.000000000000000000, 0.8660254037844387076, 1.000000000000000000, 0.8660254037844357100, 1.000000000000003109 ) ) 
 REPRESENTATION_ITEM ( '' )  );
#534=CARTESIAN_POINT ( 'NONE',  ( 5.405949406249999534, 9.363379034771803333, -25.09375000204835970 ) ) ;
#535=CARTESIAN_POINT ( 'NONE',  ( -5.405949406250003975, -9.363379034771801557, -195.3437500020484094 ) ) ;
#536=CARTESIAN_POINT ( 'NONE',  ( 10.81189881249999729, 0.000000000000000000, -49.34375000204838102 ) ) ;
#537=DIRECTION ( 'NONE',  ( -0.000000000000000000, -0.000000000000000000, 1.000000000000000000 ) ) ;
#538=EDGE_CURVE ( 'NONE', #35065, #39621, #32792, .T. ) ;
#540=CARTESIAN_POINT ( 'NONE',  ( 7.644554776091147741E-16, 12.48450537969573659, -176.4687500020484094 ) ) ;
#541=CARTESIAN_POINT ( 'NONE',  ( -2.293366432827344421E-15, -12.48450537969573659, -169.7187500020483810 ) ) ;
#544=CARTESIAN_POINT ( 'NONE',  ( -5.000000000000003553, -8.660254037844383745, -104.8750000040967763 ) ) ;
#545=CARTESIAN_POINT ( 'NONE',  ( 9.999999999999998224, 0.000000000000000000, -188.3750000040967905 ) ) ;
#547=CARTESIAN_POINT ( 'NONE',  ( 5.405949406249992428, -9.363379034771808662, -97.59375000204838102 ) ) ;
#548=CARTESIAN_POINT ( 'NONE',  ( 5.405949406249999534, 9.363379034771803333, -65.78125000204838102 ) ) ;
#551=CARTESIAN_POINT ( 'NONE',  ( -5.405949406250003975, -9.363379034771801557, -125.0312500020483952 ) ) ;
#552=CARTESIAN_POINT ( 'NONE',  ( -2.293366432827344421E-15, -12.48450537969573659, -159.4062500020483810 ) ) ;
#554=CARTESIAN_POINT ( 'NONE',  ( 9.999999999999998224, 0.000000000000000000, -138.8750000040968189 ) ) ;
#559=CARTESIAN_POINT ( 'NONE',  ( -10.81189881249999729, 1.324075727343319199E-15, -188.2812500020484094 ) ) ;
#561=AXIS2_PLACEMENT_3D ( 'NONE', #36619, #6430, #2984 ) ;
#562=ORIENTED_EDGE ( 'NONE', *, *, #35604, .T. ) ;
#563=CARTESIAN_POINT ( 'NONE',  ( -9.999999999999998224, 5.773502691896259087, -53.87499999999996447 ) ) ;
#565=CARTESIAN_POINT ( 'NONE',  ( 7.070501591499377789E-16, 11.54700538379251284, -68.00000000409679046 ) ) ;
#567=CARTESIAN_POINT ( 'NONE',  ( 7.070501591499376803E-16, 11.54700538379251284, -179.0000000040967905 ) ) ;
#569=CARTESIAN_POINT ( 'NONE',  ( 5.405949406249992428, -9.363379034771808662, -58.78125000204836681 ) ) ;
#570=( BOUNDED_CURVE ( )  B_SPLINE_CURVE ( 2, ( #24153, #28024, #1483, #40729, #41154, #21541, #1270 ),
 .UNSPECIFIED., .F., .F. ) 
 B_SPLINE_CURVE_WITH_KNOTS ( ( 3, 2, 2, 3 ),
 ( 0.2201492537313433639, 0.2213930348258707215, 0.2226368159203980790, 0.2238805970149254365 ),
 .UNSPECIFIED. ) 
 CURVE ( )  GEOMETRIC_REPRESENTATION_ITEM ( )  RATIONAL_B_SPLINE_CURVE ( ( 0.9999999999999910072, 0.8660254037844477004, 1.000000000000000000, 0.8660254037844387076, 1.000000000000000000, 0.8660254037844327124, 1.000000000000005995 ) ) 
 REPRESENTATION_ITEM ( '' )  );
#573=DIRECTION ( 'NONE',  ( 1.000000000000000000, 0.000000000000000000, 0.000000000000000000 ) ) ;
#574=CARTESIAN_POINT ( 'NONE',  ( -5.405949406250003975, -9.363379034771801557, -182.0312500020483810 ) ) ;
#576=CARTESIAN_POINT ( 'NONE',  ( 5.000000000000000000, 8.660254037844385522, -85.74999999999998579 ) ) ;
#579=DIRECTION ( 'NONE',  ( -0.000000000000000000, -0.000000000000000000, 1.000000000000000000 ) ) ;
#582=CARTESIAN_POINT ( 'NONE',  ( -10.81189881249999729, 6.242252689847871849, -92.40625000204838102 ) ) ;
#584=CARTESIAN_POINT ( 'NONE',  ( -4.999999999999996447, 8.660254037844387298, -24.37500000409675849 ) ) ;
#586=ORIENTED_EDGE ( 'NONE', *, *, #41768, .F. ) ;
#588=CARTESIAN_POINT ( 'NONE',  ( -10.81189881249999729, 6.242252689847871849, -23.21875000204836326 ) ) ;
#589=CARTESIAN_POINT ( 'NONE',  ( -10.81189881249999729, 6.242252689847871849, -21.90625000204837036 ) ) ;
#590=( BOUNDED_CURVE ( )  B_SPLINE_CURVE ( 2, ( #31404, #18430, #8519, #21672, #31619, #26918, #41073 ),
 .UNSPECIFIED., .F., .F. ) 
 B_SPLINE_CURVE_WITH_KNOTS ( ( 3, 2, 2, 3 ),
 ( 0.02985074626865674360, 0.03109452736318411153, 0.03233830845771147600, 0.03358208955223884046 ),
 .UNSPECIFIED. ) 
 CURVE ( )  GEOMETRIC_REPRESENTATION_ITEM ( )  RATIONAL_B_SPLINE_CURVE ( ( 0.9999999999999970024, 0.8660254037844417052, 1.000000000000000000, 0.8660254037844387076, 1.000000000000000000, 0.8660254037844349329, 1.000000000000003775 ) ) 
 REPRESENTATION_ITEM ( '' )  );
#592=CARTESIAN_POINT ( 'NONE',  ( -10.81189881249999907, -6.242252689847864744, -70.96875000204840944 ) ) ;
#593=CARTESIAN_POINT ( 'NONE',  ( -10.00000000000012790, -5.773502691896178263, -174.0000000040968473 ) ) ;
#594=ADVANCED_FACE ( 'NONE', ( #20609 ), #33795, .T. ) ;
#596=CARTESIAN_POINT ( 'NONE',  ( 5.405949406249999534, 9.363379034771803333, -196.0937500020484094 ) ) ;
#597=CARTESIAN_POINT ( 'NONE',  ( 5.405949406249999534, 9.363379034771803333, -148.0937500020483810 ) ) ;
#598=EDGE_CURVE ( 'NONE', #33430, #41855, #8103, .T. ) ;
#599=CARTESIAN_POINT ( 'NONE',  ( -10.00000000000076916, 5.773502691895813221, -132.2500000040967620 ) ) ;
#600=FACE_OUTER_BOUND ( 'NONE', #38499, .T. ) ;
#602=CARTESIAN_POINT ( 'NONE',  ( -2.121150477449813534E-15, -11.54700538379251284, -2.750000004096756712 ) ) ;
#604=CARTESIAN_POINT ( 'NONE',  ( 5.405949406249999534, 9.363379034771803333, -124.0937500020483952 ) ) ;
#605=DIRECTION ( 'NONE',  ( -0.000000000000000000, -0.000000000000000000, 1.000000000000000000 ) ) ;
#606=CARTESIAN_POINT ( 'NONE',  ( 5.405949406249999534, 9.363379034771803333, -94.28125000204838102 ) ) ;
#607=CARTESIAN_POINT ( 'NONE',  ( 10.81189881249999729, 6.242252689847867408, -100.2187500020483810 ) ) ;
#610=CARTESIAN_POINT ( 'NONE',  ( 10.00000000000000000, 5.773502691896255534, -165.7500000040967905 ) ) ;
#613=DIRECTION ( 'NONE',  ( -0.000000000000000000, -0.000000000000000000, 1.000000000000000000 ) ) ;
#615=CARTESIAN_POINT ( 'NONE',  ( -2.121150477449813534E-15, -11.54700538379251284, -149.3750000000000000 ) ) ;
#617=CARTESIAN_POINT ( 'NONE',  ( -4.999999999999996447, 8.660254037844387298, -79.49999999999998579 ) ) ;
#619=CARTESIAN_POINT ( 'NONE',  ( 9.999999999999998224, 0.000000000000000000, -93.87500000409677625 ) ) ;
#622=CARTESIAN_POINT ( 'NONE',  ( 7.644554776091147741E-16, 12.48450537969573659, -83.65625000204838102 ) ) ;
#626=EDGE_LOOP ( 'NONE', ( #27970, #9734, #5629, #32320 ) ) ;
#627=CARTESIAN_POINT ( 'NONE',  ( -9.999999999999998224, 5.773502691896259087, -10.37499999999995381 ) ) ;
#629=CARTESIAN_POINT ( 'NONE',  ( -4.999999999999996447, 8.660254037844387298, -147.0000000000000000 ) ) ;
#631=EDGE_CURVE ( 'NONE', #26632, #15830, #7962, .T. ) ;
#632=VECTOR ( 'NONE', #19479, 1000.000000000000000 ) ;
#634=CARTESIAN_POINT ( 'NONE',  ( -9.999999999999998224, 5.773502691896259087, -188.8750000000000568 ) ) ;
#636=CARTESIAN_POINT ( 'NONE',  ( -5.405949406249996869, 9.363379034771805109, -118.0312500020483952 ) ) ;
#638=CARTESIAN_POINT ( 'NONE',  ( 4.999999999999992006, -8.660254037844389075, -74.62500000409677625 ) ) ;
#639=ORIENTED_EDGE ( 'NONE', *, *, #8724, .T. ) ;
#640=ORIENTED_EDGE ( 'NONE', *, *, #901, .F. ) ;
#641=CARTESIAN_POINT ( 'NONE',  ( 7.644554776091147741E-16, 12.48450537969573659, -43.15625000204838102 ) ) ;
#643=CARTESIAN_POINT ( 'NONE',  ( -10.81189881249999907, -6.242252689847864744, -94.96875000204838102 ) ) ;
#644=CARTESIAN_POINT ( 'NONE',  ( 10.81189881249999729, 0.000000000000000000, -120.0312500020483952 ) ) ;
#646=ORIENTED_EDGE ( 'NONE', *, *, #5501, .F. ) ;
#647=CARTESIAN_POINT ( 'NONE',  ( -9.999999999999998224, 1.224646799147353059E-15, -133.2499999999999716 ) ) ;
#648=CARTESIAN_POINT ( 'NONE',  ( 10.81189881249999729, 0.000000000000000000, -193.3437500020484094 ) ) ;
#649=ADVANCED_FACE ( 'NONE', ( #25782 ), #8323, .T. ) ;
#652=CARTESIAN_POINT ( 'NONE',  ( -5.405949406249996869, 9.363379034771805109, -129.8437500020484094 ) ) ;
#653=( BOUNDED_CURVE ( )  B_SPLINE_CURVE ( 2, ( #37800, #31773, #34793, #28743, #41870, #5213, #18149 ),
 .UNSPECIFIED., .F., .F. ) 
 B_SPLINE_CURVE_WITH_KNOTS ( ( 3, 2, 2, 3 ),
 ( 0.9328358208955226383, 0.9340796019900500236, 0.9353233830845774088, 0.9365671641791047941 ),
 .UNSPECIFIED. ) 
 CURVE ( )  GEOMETRIC_REPRESENTATION_ITEM ( )  RATIONAL_B_SPLINE_CURVE ( ( 0.9999999999999761302, 0.8660254037844625774, 1.000000000000000000, 0.8660254037844387076, 1.000000000000000000, 0.8660254037844028474, 1.000000000000035971 ) ) 
 REPRESENTATION_ITEM ( '' )  );
#658=CARTESIAN_POINT ( 'NONE',  ( 4.999999999999992006, -8.660254037844389075, -187.1250000040967905 ) ) ;
#660=CARTESIAN_POINT ( 'NONE',  ( -2.293366432827344421E-15, -12.48450537969573659, -178.9062500020484379 ) ) ;
#661=CARTESIAN_POINT ( 'NONE',  ( 9.999999999999998224, 0.000000000000000000, -200.0000000000000000 ) ) ;
#664=CARTESIAN_POINT ( 'NONE',  ( -5.405949406249996869, 9.363379034771805109, -63.84375000204836681 ) ) ;
#666=CARTESIAN_POINT ( 'NONE',  ( 10.81189881249999551, -6.242252689847874514, -44.96875000204836681 ) ) ;
#668=CARTESIAN_POINT ( 'NONE',  ( 5.405949406249999534, 9.363379034771803333, -19.28125000204835970 ) ) ;
#670=DIRECTION ( 'NONE',  ( 1.000000000000000000, 0.000000000000000000, 0.000000000000000000 ) ) ;
#672=CARTESIAN_POINT ( 'NONE',  ( 4.999999999999992006, -8.660254037844389075, -107.2499999999999858 ) ) ;
#677=CARTESIAN_POINT ( 'NONE',  ( -5.405949406249996869, 9.363379034771805109, -109.0312500020483810 ) ) ;
#678=ADVANCED_FACE ( 'NONE', ( #5078 ), #28601, .T. ) ;
#679=ORIENTED_EDGE ( 'NONE', *, *, #9216, .T. ) ;
#680=CARTESIAN_POINT ( 'NONE',  ( -4.999999999999996447, 8.660254037844387298, -160.5000000000000000 ) ) ;
#684=VERTEX_POINT ( 'NONE', #25360 ) ;
#685=CARTESIAN_POINT ( 'NONE',  ( -5.000000000000003553, -8.660254037844383745, -32.49999999999997158 ) ) ;
#686=CARTESIAN_POINT ( 'NONE',  ( 5.405949406249992428, -9.363379034771808662, -36.28125000204837391 ) ) ;
#688=CARTESIAN_POINT ( 'NONE',  ( -10.00000000000102496, 5.773502691895664007, -57.25000000409674072 ) ) ;
#689=CARTESIAN_POINT ( 'NONE',  ( -10.81189881249999729, 6.242252689847871849, -144.9062500020484094 ) ) ;
#690=CARTESIAN_POINT ( 'NONE',  ( -4.999999999999996447, 8.660254037844387298, -166.8750000040967905 ) ) ;
#692=VECTOR ( 'NONE', #41320, 1000.000000000000227 ) ;
#693=ORIENTED_EDGE ( 'NONE', *, *, #35509, .F. ) ;
#695=CYLINDRICAL_SURFACE ( 'NONE', #38038, 9.999999999999998224 ) ;
#696=( BOUNDED_CURVE ( )  B_SPLINE_CURVE ( 2, ( #32919, #42190, #13037, #42399, #26231, #3352, #25810 ),
 .UNSPECIFIED., .F., .F. ) 
 B_SPLINE_CURVE_WITH_KNOTS ( ( 3, 2, 2, 3 ),
 ( 0.3320895522388061516, 0.3333333333333334259, 0.3345771144278607556, 0.3358208955223880854 ),
 .UNSPECIFIED. ) 
 CURVE ( )  GEOMETRIC_REPRESENTATION_ITEM ( )  RATIONAL_B_SPLINE_CURVE ( ( 0.9999999999999820144, 0.8660254037844566932, 1.000000000000000000, 0.8660254037844387076, 1.000000000000000000, 0.8660254037844387076, 1.000000000000000000 ) ) 
 REPRESENTATION_ITEM ( '' )  );
#697=CARTESIAN_POINT ( 'NONE',  ( -10.81189881249999729, 6.242252689847871849, -164.2187500020483810 ) ) ;
#699=CARTESIAN_POINT ( 'NONE',  ( 5.405949406249999534, 9.363379034771803333, -16.09375000204835260 ) ) ;
#700=CARTESIAN_POINT ( 'NONE',  ( -12.99038105676667598, 7.500000000000051514, 49.99999999999998579 ) ) ;
#701=CARTESIAN_POINT ( 'NONE',  ( -10.81189881249999729, 6.242252689847871849, -158.2187500020483810 ) ) ;
#702=CARTESIAN_POINT ( 'NONE',  ( -5.405949406249996869, 9.363379034771805109, -138.8437500020484094 ) ) ;
#703=CARTESIAN_POINT ( 'NONE',  ( -2.121150477449813534E-15, -11.54700538379251284, -8.750000004096753159 ) ) ;
#707=CARTESIAN_POINT ( 'NONE',  ( -5.405949406250003975, -9.363379034771801557, -12.34375000204834905 ) ) ;
#710=CARTESIAN_POINT ( 'NONE',  ( -9.999999999999998224, 1.224646799147353059E-15, -178.6250000040968189 ) ) ;
#713=EDGE_CURVE ( 'NONE', #35715, #25539, #16503, .T. ) ;
#714=CARTESIAN_POINT ( 'NONE',  ( 10.81189881249999729, 0.000000000000000000, -82.34375000204836681 ) ) ;
#715=CARTESIAN_POINT ( 'NONE',  ( -5.405949406250003975, -9.363379034771801557, -63.34375000204836681 ) ) ;
#716=CARTESIAN_POINT ( 'NONE',  ( -9.999999999999998224, 1.224646799147353059E-15, -35.74999999999997868 ) ) ;
#717=CARTESIAN_POINT ( 'NONE',  ( -5.405949406249996869, 9.363379034771805109, -44.53125000204838102 ) ) ;
#719=CYLINDRICAL_SURFACE ( 'NONE', #31650, 9.999999999999998224 ) ;
#721=CARTESIAN_POINT ( 'NONE',  ( -10.00000000000000000, -5.773502691896251982, -131.6250000000000000 ) ) ;
#722=CARTESIAN_POINT ( 'NONE',  ( 10.81189881249999729, 0.000000000000000000, -138.0312500020484094 ) ) ;
#723=FACE_OUTER_BOUND ( 'NONE', #41523, .T. ) ;
#725=CARTESIAN_POINT ( 'NONE',  ( 5.405949406249999534, 9.363379034771803333, -17.78125000204835970 ) ) ;
#726=ORIENTED_EDGE ( 'NONE', *, *, #22094, .T. ) ;
#730=AXIS2_PLACEMENT_3D ( 'NONE', #35139, #34718, #14823 ) ;
#731=CARTESIAN_POINT ( 'NONE',  ( 9.999999999999996447, -5.773502691896262640, -44.50000000409676915 ) ) ;
#734=CARTESIAN_POINT ( 'NONE',  ( -10.81189881249999907, -6.242252689847864744, -152.1562500020484094 ) ) ;
#735=CARTESIAN_POINT ( 'NONE',  ( -5.405949406250003975, -9.363379034771801557, -133.8437500020484094 ) ) ;
#736=CARTESIAN_POINT ( 'NONE',  ( 9.999999999999479527, 5.773502691896553074, -150.3750000000000000 ) ) ;
#737=ORIENTED_EDGE ( 'NONE', *, *, #16143, .T. ) ;
#738=LINE ( 'NONE', #34393, #39657 ) ;
#739=CARTESIAN_POINT ( 'NONE',  ( -2.293366432827344421E-15, -12.48450537969573659, -63.40625000204838102 ) ) ;
#742=CARTESIAN_POINT ( 'NONE',  ( 7.644554776091147741E-16, 12.48450537969573659, -114.9687500020483668 ) ) ;
#743=ORIENTED_EDGE ( 'NONE', *, *, #17051, .T. ) ;
#744=CARTESIAN_POINT ( 'NONE',  ( 7.644554776091147741E-16, 12.48450537969573659, -18.96875000204837391 ) ) ;
#745=CARTESIAN_POINT ( 'NONE',  ( 5.405949406249999534, 9.363379034771803333, -188.5937500020483810 ) ) ;
#746=CARTESIAN_POINT ( 'NONE',  ( 5.405949406249999534, 9.363379034771803333, -46.09375000204838102 ) ) ;
#747=CARTESIAN_POINT ( 'NONE',  ( 9.999999999998456346, 5.773502691897149042, -62.25000000409676204 ) ) ;
#749=AXIS2_PLACEMENT_3D ( 'NONE', #21637, #18173, #15569 ) ;
#750=CARTESIAN_POINT ( 'NONE',  ( -10.81189881249999729, -6.242252689847864744, -180.4687500020484094 ) ) ;
#751=CARTESIAN_POINT ( 'NONE',  ( -5.405949406250003975, -9.363379034771801557, -163.8437500020484094 ) ) ;
#754=CYLINDRICAL_SURFACE ( 'NONE', #21930, 9.999999999999998224 ) ;
#757=CARTESIAN_POINT ( 'NONE',  ( -10.81189881249999729, 1.324075727343319199E-15, -92.09375000204838102 ) ) ;
#758=CARTESIAN_POINT ( 'NONE',  ( -2.293366432827344421E-15, -12.48450537969573659, -69.40625000204838102 ) ) ;
#760=CARTESIAN_POINT ( 'NONE',  ( -5.405949406250003975, -9.363379034771801557, -122.0312500020483952 ) ) ;
#761=CARTESIAN_POINT ( 'NONE',  ( 10.81189881249999551, -6.242252689847874514, -162.1562500020484094 ) ) ;
#763=CARTESIAN_POINT ( 'NONE',  ( -9.999999999999998224, 5.773502691896259087, -136.7500000040967905 ) ) ;
#768=CARTESIAN_POINT ( 'NONE',  ( -5.405949406250003975, -9.363379034771801557, -188.0312500020484094 ) ) ;
#770=ORIENTED_EDGE ( 'NONE', *, *, #21485, .F. ) ;
#771=CARTESIAN_POINT ( 'NONE',  ( -9.999999999999998224, 1.224646799147353059E-15, -52.24999999999996447 ) ) ;
#773=CARTESIAN_POINT ( 'NONE',  ( 9.999999999999996447, -5.773502691896262640, -62.50000000409677625 ) ) ;
#774=DIRECTION ( 'NONE',  ( 1.000000000000000000, 0.000000000000000000, 0.000000000000000000 ) ) ;
#775=CARTESIAN_POINT ( 'NONE',  ( 5.000000000000000000, 8.660254037844385522, -179.1250000040968189 ) ) ;
#777=CARTESIAN_POINT ( 'NONE',  ( 7.644554776091147741E-16, 12.48450537969573659, -56.65625000204837391 ) ) ;
#778=ADVANCED_FACE ( 'NONE', ( #8529 ), #41731, .T. ) ;
#781=LINE ( 'NONE', #14330, #22809 ) ;
#782=CARTESIAN_POINT ( 'NONE',  ( -2.293366432827344421E-15, -12.48450537969573659, -174.4062500020483810 ) ) ;
#786=DIRECTION ( 'NONE',  ( 1.000000000000000000, 4.506943796211477094E-16, 0.000000000000000000 ) ) ;
#789=LINE ( 'NONE', #29930, #38601 ) ;
#790=CARTESIAN_POINT ( 'NONE',  ( 5.405949406249992428, -9.363379034771808662, -85.78125000204838102 ) ) ;
#792=CYLINDRICAL_SURFACE ( 'NONE', #42070, 9.999999999999998224 ) ;
#793=DIRECTION ( 'NONE',  ( 0.000000000000000000, 0.000000000000000000, -1.000000000000000000 ) ) ;
#794=ORIENTED_EDGE ( 'NONE', *, *, #33571, .F. ) ;
#795=VERTEX_POINT ( 'NONE', #5721 ) ;
#796=CARTESIAN_POINT ( 'NONE',  ( 10.81189881249999551, -6.242252689847874514, -26.96875000204837747 ) ) ;
#797=CARTESIAN_POINT ( 'NONE',  ( 5.405949406249999534, 9.363379034771803333, -20.78125000204836326 ) ) ;
#799=CARTESIAN_POINT ( 'NONE',  ( -10.81189881249999729, 6.242252689847871849, -69.71875000204838102 ) ) ;
#802=CARTESIAN_POINT ( 'NONE',  ( -10.81189881249999729, 1.324075727343319199E-15, -183.5937500020483810 ) ) ;
#803=AXIS2_PLACEMENT_3D ( 'NONE', #35661, #19239, #32428 ) ;
#804=CARTESIAN_POINT ( 'NONE',  ( -9.999999999999998224, 1.224646799147353059E-15, -178.6250000040968189 ) ) ;
#805=CARTESIAN_POINT ( 'NONE',  ( -10.00000000000051337, 5.773502691895962435, -98.87499999999997158 ) ) ;
#806=CARTESIAN_POINT ( 'NONE',  ( -9.999999999999998224, 1.224646799147353059E-15, -95.74999999999998579 ) ) ;
#807=CARTESIAN_POINT ( 'NONE',  ( 9.999999999999996447, -5.773502691896262640, -1.000000004096748496 ) ) ;
#810=CARTESIAN_POINT ( 'NONE',  ( 5.405949406249999534, 9.363379034771803333, -118.0937500020483810 ) ) ;
#811=CARTESIAN_POINT ( 'NONE',  ( -9.999999999999998224, 1.224646799147353059E-15, -109.2499999999999858 ) ) ;
#812=CARTESIAN_POINT ( 'NONE',  ( 5.405949406249999534, 9.363379034771803333, -89.78125000204838102 ) ) ;
#813=CARTESIAN_POINT ( 'NONE',  ( 5.405949406249992428, -9.363379034771808662, -97.59375000204838102 ) ) ;
#816=CARTESIAN_POINT ( 'NONE',  ( 9.999999999999998224, 0.000000000000000000, -159.8750000040967905 ) ) ;
#817=( BOUNDED_CURVE ( )  B_SPLINE_CURVE ( 2, ( #10105, #39880, #23929, #23502, #17205, #20245, #37073 ),
 .UNSPECIFIED., .F., .F. ) 
 B_SPLINE_CURVE_WITH_KNOTS ( ( 3, 2, 2, 3 ),
 ( 0.9141791044776121922, 0.9154228855721395774, 0.9166666666666669627, 0.9179104477611943480 ),
 .UNSPECIFIED. ) 
 CURVE ( )  GEOMETRIC_REPRESENTATION_ITEM ( )  RATIONAL_B_SPLINE_CURVE ( ( 0.9999999999999761302, 0.8660254037844625774, 1.000000000000000000, 0.8660254037844387076, 1.000000000000000000, 0.8660254037844028474, 1.000000000000035971 ) ) 
 REPRESENTATION_ITEM ( '' )  );
#820=VECTOR ( 'NONE', #41436, 1000.000000000000000 ) ;
#822=CARTESIAN_POINT ( 'NONE',  ( -9.999999999999998224, 1.224646799147353059E-15, -149.7500000000000000 ) ) ;
#825=CARTESIAN_POINT ( 'NONE',  ( -5.000000000000003553, -8.660254037844383745, -77.49999999999998579 ) ) ;
#827=CARTESIAN_POINT ( 'NONE',  ( -9.999999999999998224, 1.224646799147353059E-15, -93.12500000409677625 ) ) ;
#829=CARTESIAN_POINT ( 'NONE',  ( 5.405949406249999534, 9.363379034771803333, -86.78125000204838102 ) ) ;
#833=ORIENTED_EDGE ( 'NONE', *, *, #26459, .F. ) ;
#834=CARTESIAN_POINT ( 'NONE',  ( 9.999999999999996447, -5.773502691896262640, -11.12499999999995737 ) ) ;
#836=EDGE_CURVE ( 'NONE', #16464, #23854, #11860, .T. ) ;
#837=CARTESIAN_POINT ( 'NONE',  ( 9.999999999999996447, -5.773502691896262640, -147.6250000000000000 ) ) ;
#838=CARTESIAN_POINT ( 'NONE',  ( 9.999999999999998224, 0.000000000000000000, -200.0000000000000000 ) ) ;
#840=CARTESIAN_POINT ( 'NONE',  ( 7.644554776091147741E-16, 12.48450537969573659, -134.6562500020483810 ) ) ;
#842=CARTESIAN_POINT ( 'NONE',  ( -2.121150477449813534E-15, -11.54700538379251284, -188.3750000000000284 ) ) ;
#843=DIRECTION ( 'NONE',  ( -1.000000000000000000, -4.506943796211477094E-16, 0.000000000000000000 ) ) ;
#844=APPLICATION_CONTEXT ( 'configuration controlled 3d designs of mechanical parts and assemblies' ) ;
#845=CARTESIAN_POINT ( 'NONE',  ( 10.81189881249999907, 6.242252689847868297, -113.9062500020483952 ) ) ;
#846=EDGE_LOOP ( 'NONE', ( #39244, #16924, #7522, #35832 ) ) ;
#847=CARTESIAN_POINT ( 'NONE',  ( -4.999999999999996447, 8.660254037844387298, -36.37500000409676915 ) ) ;
#848=VERTEX_POINT ( 'NONE', #12170 ) ;
#850=CARTESIAN_POINT ( 'NONE',  ( 5.405949406249999534, 9.363379034771803333, -49.28125000204838813 ) ) ;
#852=VECTOR ( 'NONE', #22630, 1000.000000000000000 ) ;
#853=CARTESIAN_POINT ( 'NONE',  ( -5.405949406250003975, -9.363379034771801557, -93.34375000204838102 ) ) ;
#854=CARTESIAN_POINT ( 'NONE',  ( 10.81189881249999729, 6.242252689847867408, -122.9062500020483810 ) ) ;
#857=CARTESIAN_POINT ( 'NONE',  ( 5.405949406249999534, 9.363379034771803333, -194.5937500020484094 ) ) ;
#859=CARTESIAN_POINT ( 'NONE',  ( -2.121150477449813534E-15, -11.54700538379251284, -68.37499999999998579 ) ) ;
#860=CARTESIAN_POINT ( 'NONE',  ( -10.81189881249999729, 1.324075727343319199E-15, -128.0937500020483810 ) ) ;
#862=CYLINDRICAL_SURFACE ( 'NONE', #31845, 9.999999999999998224 ) ;
#864=CARTESIAN_POINT ( 'NONE',  ( 7.070501591499377789E-16, 11.54700538379251284, -188.0000000040967905 ) ) ;
#866=CARTESIAN_POINT ( 'NONE',  ( 5.405949406249992428, -9.363379034771808662, -180.2812500020484094 ) ) ;
#870=CARTESIAN_POINT ( 'NONE',  ( -10.81189881249999729, 1.324075727343319199E-15, -50.09375000204835260 ) ) ;
#871=CARTESIAN_POINT ( 'NONE',  ( 10.81189881249999551, -6.242252689847874514, -41.96875000204835970 ) ) ;
#873=CARTESIAN_POINT ( 'NONE',  ( 10.81189881249999729, 0.000000000000000000, -12.03125000204835438 ) ) ;
#877=CARTESIAN_POINT ( 'NONE',  ( 4.999999999999992006, -8.660254037844389075, -102.7500000000000000 ) ) ;
#881=CARTESIAN_POINT ( 'NONE',  ( -5.405949406249996869, 9.363379034771805109, -106.0312500020483810 ) ) ;
#883=CARTESIAN_POINT ( 'NONE',  ( 4.999999999999992006, -8.660254037844389075, -6.749999999999978684 ) ) ;
#885=CARTESIAN_POINT ( 'NONE',  ( 10.00000000000011013, -5.773502691896197803, -194.5000000040968189 ) ) ;
#888=CARTESIAN_POINT ( 'NONE',  ( -9.999999999999998224, 5.773502691896259087, -29.87499999999994671 ) ) ;
#889=EDGE_CURVE ( 'NONE', #21756, #21702, #32549, .T. ) ;
#890=CARTESIAN_POINT ( 'NONE',  ( 7.644554776091147741E-16, 12.48450537969573659, -35.65625000204835260 ) ) ;
#891=CARTESIAN_POINT ( 'NONE',  ( -2.121150477449813534E-15, -11.54700538379251284, -90.87500000000000000 ) ) ;
#894=ADVANCED_FACE ( 'NONE', ( #15403, #36540 ), #12798, .F. ) ;
#896=CARTESIAN_POINT ( 'NONE',  ( -5.405949406250003975, -9.363379034771801557, -138.5312500020484094 ) ) ;
#898=CARTESIAN_POINT ( 'NONE',  ( -4.999999999999996447, 8.660254037844387298, -174.3750000040968189 ) ) ;
#899=ORIENTED_EDGE ( 'NONE', *, *, #28328, .T. ) ;
#900=VERTEX_POINT ( 'NONE', #13639 ) ;
#901=EDGE_CURVE ( 'NONE', #35538, #22217, #21188, .T. ) ;
#903=CARTESIAN_POINT ( 'NONE',  ( 9.999999999999998224, 0.000000000000000000, -105.8750000040967763 ) ) ;
#904=CARTESIAN_POINT ( 'NONE',  ( -10.81189881249999907, -6.242252689847864744, -163.9687500020484094 ) ) ;
#905=ADVANCED_FACE ( 'NONE', ( #38935 ), #13216, .T. ) ;
#907=CARTESIAN_POINT ( 'NONE',  ( -2.293366432827344421E-15, -12.48450537969573659, -16.71875000204836326 ) ) ;
#908=DIRECTION ( 'NONE',  ( 1.000000000000000000, 0.000000000000000000, 0.000000000000000000 ) ) ;
#909=CARTESIAN_POINT ( 'NONE',  ( -5.405949406250003975, -9.363379034771801557, -144.3437500020483810 ) ) ;
#910=CARTESIAN_POINT ( 'NONE',  ( 5.405949406249992428, -9.363379034771808662, -141.0937500020483810 ) ) ;
#911=CARTESIAN_POINT ( 'NONE',  ( 10.81189881249999729, 0.000000000000000000, -109.5312500020483810 ) ) ;
#915=CARTESIAN_POINT ( 'NONE',  ( -10.81189881249999907, -6.242252689847864744, -13.96875000204836681 ) ) ;
#918=CARTESIAN_POINT ( 'NONE',  ( 10.00000000000051159, -5.773502691895965988, -96.62499999999998579 ) ) ;
#921=CARTESIAN_POINT ( 'NONE',  ( -10.81189881249999729, -6.242252689847864744, -84.46875000204836681 ) ) ;
#922=CARTESIAN_POINT ( 'NONE',  ( 10.81189881249999551, -6.242252689847874514, -64.46875000204838102 ) ) ;
#923=CARTESIAN_POINT ( 'NONE',  ( 10.81189881249999907, 6.242252689847868297, -37.40625000204836681 ) ) ;
#925=DIRECTION ( 'NONE',  ( 1.000000000000000000, 0.000000000000000000, 0.000000000000000000 ) ) ;
#927=CARTESIAN_POINT ( 'NONE',  ( -2.121150477449813534E-15, -11.54700538379251284, -128.3750000000000000 ) ) ;
#928=CARTESIAN_POINT ( 'NONE',  ( 5.405949406249992428, -9.363379034771808662, -127.7812500020483810 ) ) ;
#929=EDGE_CURVE ( 'NONE', #29237, #40403, #1924, .T. ) ;
#932=CARTESIAN_POINT ( 'NONE',  ( -5.405949406249996869, 9.363379034771805109, -22.03125000204836326 ) ) ;
#933=VERTEX_POINT ( 'NONE', #36122 ) ;
#936=CARTESIAN_POINT ( 'NONE',  ( -4.999999999999996447, 8.660254037844387298, -38.99999999999997868 ) ) ;
#937=CARTESIAN_POINT ( 'NONE',  ( -10.00000000000000000, -5.773502691896251982, -33.00000000409676204 ) ) ;
#940=CARTESIAN_POINT ( 'NONE',  ( 9.999999999999998224, 0.000000000000000000, -146.0000000000000000 ) ) ;
#941=CARTESIAN_POINT ( 'NONE',  ( -2.293366432827344421E-15, -12.48450537969573659, -151.9062500020483810 ) ) ;
#942=CARTESIAN_POINT ( 'NONE',  ( -5.405949406250003975, -9.363379034771801557, -136.8437500020484094 ) ) ;
#943=CARTESIAN_POINT ( 'NONE',  ( -9.999999999999998224, 1.224646799147353059E-15, -199.2500000000000000 ) ) ;
#945=CYLINDRICAL_SURFACE ( 'NONE', #32114, 9.999999999999998224 ) ;
#947=( BOUNDED_CURVE ( )  B_SPLINE_CURVE ( 2, ( #24537, #27764, #27336, #11550, #27982, #24759, #4887 ),
 .UNSPECIFIED., .F., .F. ) 
 B_SPLINE_CURVE_WITH_KNOTS ( ( 3, 2, 2, 3 ),
 ( 0.07835820895522395413, 0.07960199004975131165, 0.08084577114427868305, 0.08208955223880604057 ),
 .UNSPECIFIED. ) 
 CURVE ( )  GEOMETRIC_REPRESENTATION_ITEM ( )  RATIONAL_B_SPLINE_CURVE ( ( 0.9999999999999924505, 0.8660254037844461461, 1.000000000000000000, 0.8660254037844387076, 1.000000000000000000, 0.8660254037844312691, 1.000000000000007550 ) ) 
 REPRESENTATION_ITEM ( '' )  );
#948=EDGE_CURVE ( 'NONE', #41544, #2239, #13723, .T. ) ;
#949=ORIENTED_EDGE ( 'NONE', *, *, #14043, .F. ) ;
#951=CARTESIAN_POINT ( 'NONE',  ( -2.293366432827344421E-15, -12.48450537969573659, -109.7187500020483668 ) ) ;
#952=ORIENTED_EDGE ( 'NONE', *, *, #12475, .F. ) ;
#954=CARTESIAN_POINT ( 'NONE',  ( 10.81189881249999729, 0.000000000000000000, -193.3437500020484094 ) ) ;
#955=CARTESIAN_POINT ( 'NONE',  ( 10.81189881249999907, 6.242252689847868297, -35.71875000204835970 ) ) ;
#957=CARTESIAN_POINT ( 'NONE',  ( -9.999999999998456346, -5.773502691897145489, -10.50000000409672296 ) ) ;
#958=CARTESIAN_POINT ( 'NONE',  ( -5.405949406249996869, 9.363379034771805109, -183.8437500020483810 ) ) ;
#959=CARTESIAN_POINT ( 'NONE',  ( 10.81189881249999551, -6.242252689847874514, -158.9687500020484094 ) ) ;
#963=CARTESIAN_POINT ( 'NONE',  ( -4.999999999999996447, 8.660254037844387298, -86.99999999999998579 ) ) ;
#964=DIRECTION ( 'NONE',  ( -0.000000000000000000, -0.000000000000000000, 1.000000000000000000 ) ) ;
#966=CARTESIAN_POINT ( 'NONE',  ( 7.644554776091147741E-16, 12.48450537969573659, -87.96875000204838102 ) ) ;
#968=CARTESIAN_POINT ( 'NONE',  ( -2.293366432827344421E-15, -12.48450537969573659, -66.40625000204838102 ) ) ;
#971=CARTESIAN_POINT ( 'NONE',  ( 7.644554776091147741E-16, 12.48450537969573659, -121.1562500020483952 ) ) ;
#972=CARTESIAN_POINT ( 'NONE',  ( -10.81189881249999729, 6.242252689847871849, -158.4062500020483810 ) ) ;
#974=CARTESIAN_POINT ( 'NONE',  ( -9.999999999999998224, 5.773502691896259087, -132.2500000040967905 ) ) ;
#976=ORIENTED_EDGE ( 'NONE', *, *, #7502, .F. ) ;
#980=CARTESIAN_POINT ( 'NONE',  ( -2.293366432827344421E-15, -12.48450537969573659, -184.9062500020484094 ) ) ;
#982=VERTEX_POINT ( 'NONE', #26410 ) ;
#983=CARTESIAN_POINT ( 'NONE',  ( 5.000000000000000000, 8.660254037844385522, -48.24999999999998579 ) ) ;
#985=CARTESIAN_POINT ( 'NONE',  ( 9.999999999999998224, 0.000000000000000000, -56.37500000409676204 ) ) ;
#986=CARTESIAN_POINT ( 'NONE',  ( -5.000000000000003553, -8.660254037844383745, -179.5000000000000000 ) ) ;
#989=CARTESIAN_POINT ( 'NONE',  ( 7.644554776091147741E-16, 12.48450537969573659, -62.65625000204838813 ) ) ;
#993=CARTESIAN_POINT ( 'NONE',  ( 10.81189881249999551, -6.242252689847874514, -177.1562500020484094 ) ) ;
#995=LINE ( 'NONE', #11531, #18049 ) ;
#996=DIRECTION ( 'NONE',  ( 0.000000000000000000, -0.08715574274765837404, -0.9961946980917455452 ) ) ;
#997=CARTESIAN_POINT ( 'NONE',  ( 5.000000000000000000, 8.660254037844385522, -154.7500000000000000 ) ) ;
#999=CARTESIAN_POINT ( 'NONE',  ( -5.000000000000003553, -8.660254037844383745, -122.5000000000000000 ) ) ;
#1000=EDGE_CURVE ( 'NONE', #28982, #14499, #28136, .T. ) ;
#1001=CARTESIAN_POINT ( 'NONE',  ( 5.405949406249992428, -9.363379034771808662, -84.28125000204838102 ) ) ;
#1004=CARTESIAN_POINT ( 'NONE',  ( -4.999999999999996447, 8.660254037844387298, -80.99999999999998579 ) ) ;
#1005=EDGE_LOOP ( 'NONE', ( #25428, #30555, #16181, #13108 ) ) ;
#1006=ORIENTED_EDGE ( 'NONE', *, *, #30835, .F. ) ;
#1007=CARTESIAN_POINT ( 'NONE',  ( 5.405949406249992428, -9.363379034771808662, -34.59375000204836681 ) ) ;
#1008=CARTESIAN_POINT ( 'NONE',  ( -10.81189881249999729, 1.324075727343319199E-15, -27.59375000204836326 ) ) ;
#1009=CARTESIAN_POINT ( 'NONE',  ( -5.405949406249996869, 9.363379034771805109, -13.03125000204835615 ) ) ;
#1010=CARTESIAN_POINT ( 'NONE',  ( -2.293366432827344421E-15, -12.48450537969573659, -63.21875000204839523 ) ) ;
#1012=CARTESIAN_POINT ( 'NONE',  ( -5.405949406249996869, 9.363379034771805109, -183.8437500020483810 ) ) ;
#1014=EDGE_CURVE ( 'NONE', #18719, #21484, #32476, .T. ) ;
#1015=CARTESIAN_POINT ( 'NONE',  ( 7.070501591499376803E-16, 11.54700538379251284, -175.6250000000000000 ) ) ;
#1016=CARTESIAN_POINT ( 'NONE',  ( 9.999999999999998224, 0.000000000000000000, -200.0000000000000000 ) ) ;
#1017=CARTESIAN_POINT ( 'NONE',  ( 4.999999999999992006, -8.660254037844389075, -20.62500000409675494 ) ) ;
#1019=CARTESIAN_POINT ( 'NONE',  ( 10.81189881249999729, 0.000000000000000000, -116.8437500020483810 ) ) ;
#1020=CARTESIAN_POINT ( 'NONE',  ( 0.000000000000000000, 0.000000000000000000, -200.0000000000000000 ) ) ;
#1021=CARTESIAN_POINT ( 'NONE',  ( 10.81189881249999551, -6.242252689847874514, -88.65625000204838102 ) ) ;
#1022=CARTESIAN_POINT ( 'NONE',  ( -5.405949406249996869, 9.363379034771805109, -99.84375000204838102 ) ) ;
#1025=CARTESIAN_POINT ( 'NONE',  ( -9.999999999999998224, 1.224646799147353059E-15, -156.1250000040967905 ) ) ;
#1029=CYLINDRICAL_SURFACE ( 'NONE', #35783, 9.999999999999998224 ) ;
#1032=CARTESIAN_POINT ( 'NONE',  ( 9.999999999999996447, -5.773502691896262640, -75.62499999999998579 ) ) ;
#1034=CARTESIAN_POINT ( 'NONE',  ( 5.000000000000000000, 8.660254037844385522, -87.62500000409677625 ) ) ;
#1036=CARTESIAN_POINT ( 'NONE',  ( -2.293366432827344421E-15, -12.48450537969573659, -79.90625000204838102 ) ) ;
#1038=CARTESIAN_POINT ( 'NONE',  ( -9.999999999999998224, 1.224646799147353059E-15, -200.0000000000000000 ) ) ;
#1041=CARTESIAN_POINT ( 'NONE',  ( -2.121150477449813534E-15, -11.54700538379251284, -3.874999999999953815 ) ) ;
#1043=CARTESIAN_POINT ( 'NONE',  ( -10.81189881249999729, 6.242252689847871849, -12.71875000204837569 ) ) ;
#1044=CYLINDRICAL_SURFACE ( 'NONE', #33100, 9.999999999999998224 ) ;
#1046=CARTESIAN_POINT ( 'NONE',  ( -5.405949406250003975, -9.363379034771801557, -128.0312500020484094 ) ) ;
#1048=CARTESIAN_POINT ( 'NONE',  ( 10.00000000000000000, 5.773502691896255534, -183.3750000000000000 ) ) ;
#1050=CARTESIAN_POINT ( 'NONE',  ( 7.644554776091147741E-16, 12.48450537969573659, -113.6562500020483952 ) ) ;
#1053=VERTEX_POINT ( 'NONE', #42366 ) ;
#1055=CARTESIAN_POINT ( 'NONE',  ( -10.81189881249999729, 6.242252689847871849, -39.90625000204835970 ) ) ;
#1057=CARTESIAN_POINT ( 'NONE',  ( -2.293366432827344421E-15, -12.48450537969573659, -91.71875000204838102 ) ) ;
#1058=CARTESIAN_POINT ( 'NONE',  ( 0.000000000000000000, 0.000000000000000000, -200.0000000000000000 ) ) ;
#1059=CARTESIAN_POINT ( 'NONE',  ( -9.999999999999998224, 1.224646799147353059E-15, -200.0000000000000000 ) ) ;
#1060=VECTOR ( 'NONE', #37117, 1000.000000000000000 ) ;
#1061=FACE_OUTER_BOUND ( 'NONE', #23770, .T. ) ;
#1062=( BOUNDED_SURFACE ( )  B_SPLINE_SURFACE ( 1, 2, ( 
 ( #28852, #5971, #23214, #2527, #42619, #26242, #6592, #13048, #16280, #39391, #22790, #19749, #42199, #35952, #29477, #23005, #15652, #16072, #32515, #9618, #12840, #18911, #3151, #2729, #16495, #26446, #41988, #32929, #3362, #29693, #139, #13260, #19534, #39598, #29061, #12417, #6393, #25611, #32094, #32718, #9195, #38974, #22365, #12625, #19122, #9410, #22574, #25819, #35753, #10032, #6181, #32307, #15861, #19320, #2944, #1193, #7660, #39810, #37213, #40026, #10665, #19962, #27300, #20177, #10242, #3787, #20381, #20596, #4206, #33572, #16712, #16921, #3994, #7442, #33999, #24072, #20813, #346, #17138, #30122, #30339, #27516, #4420, #36793, #36578, #17560, #30760, #26660, #24293, #13468, #559, #26871, #768, #14316, #23430, #11090, #10456, #13680, #33367, #23647, #17349, #40436, #7231, #40648, #13894, #27087, #40230, #6807, #33148, #7025, #3578, #23859, #37007, #29907, #10879, #33783, #30553, #980, #14098, #8520, #34856, #21457, #4634, #4850, #8312, #38079, #21890, #11952, #8736, #30977, #34641, #34430, #5067, #15398, #35069, #24721, #24500, #5496, #18646, #14536, #12164, #1406, #17993, #14752, #18215, #31840, #40866, #41726, #27947, #31193, #21244, #41074, #5278, #27730, #28595, #31405, #11737, #15184, #17780, #1623, #2054, #2277, #21028, #11519, #37437, #21673, #37867, #1840, #28381, #7880, #41522, #34218, #11307, #25143, #14966, #37653, #8093, #28164, #41299, #24936, #18431, #31620, #38290, #8947, #6347, #32677, #12997, #19491, #22744, #3106, #29222, #26194, #5924, #42361, #35910, #16234, #22110, #22531, #38930, #32472, #19276, #25356, #9570, #9155, #22961, #32886, #35284, #29434, #42576, #39342, #9781, #36116, #25987, #6549, #35498, #5717, #12794, #18869, #29646, #16026, #32049, #2683, #89, #19075, #28809, #15818, #29014, #32256, #42153, #2896, #38504, #19703, #22323, #3316, #16448, #2478, #15607, #41941, #12374, #25570, #38722, #39138, #12584, #25777, #9362, #35704, #6133, #18116, #4535, #19913, #33319, #31311, #36536, #16662, #3744, #16874, #23386, #30079, #34330, #520, #37767, #37341, #14219, #10200, #8212, #14659, #3526, #1526, #27419, #17677, #26405, #4748, #26617, #29863, #6977, #40555, #27632, #11212, #10999, #23165, #20131, #24193, #14440, #40981, #31093, #27848, #6759, #7787, #20931, #34113, #34544, #11424, #30872, #301, #24619, #21361, #33102, #13211, #13421, #1307, #40771, #24412, #4970, #39766, #39555, #37553, #7991, #21144, #17894, #9986, #36328, #18975, #2169, #25261, #15507, #41192, #1954, #2380, #38617, #14869, #15080, #35396, #8848, #28280, #41417, #28712, #25472, #41838, #9054, #22221, #12276, #5398, #24838, #37985, #8429, #18336, #38195, #11633, #34760, #2590, #28066, #18762, #5820, #32160, #31951, #35181, #15719, #12067, #1743, #18550, #21582, #5182, #31525, #8639, #11853, #25052, #21794, #34974, #31740, #15304, #28501, #41631, #38406, #22006, #5607, #12960, #19453, #25741, #35246, #42536, #22924, #19244, #5461, #18611, #9322, #32221, #2647, #9116, #15360, #35666, #31804, #2235, #12549, #38894, #25320, #28558, #35875, #32011, #26156, #19037, #22287, #22491, #22072, #12334, #6307, #38682, #12129, #41901, #15571, #35458, #5883, #15779, #32643, #9535, #6097, #5678, #15990, #42115, #28977, #2859, #3070, #25533, #41690, #32434, #39306, #2436, #29187, #22706, #16196, #18827, #38466, #29396, #42326, #28772, #8908, #9743, #12752, #25948, #39097, #36498, #265, #23765, #16623, #33060, #3487, #23560, #481, #689, #10578, #10795, #26788, #6723, #29826, #32852, #36079, #26999, #26578, #39728, #6934, #13808, #20089, #10163, #29606, #33697, #36294, #7146, #7362, #13386, #39937, #16835, #16407, #23346, #36920, #10369, #36707, #30036, #33281, #14013, #17052, #20299, #19664, #26368, #13175, #3706, #40150, #3916, #50, #17264, #3280, #4123, #23129, #13596, #33490, #30251, #20511, #39521, #27207, #30468, #896, #40352, #9950, #6515, #19876, #37994, #7572, #34126, #5191, #24632, #4546, #20941, #31321, #8440, #1753, #21591, #34770, #14881, #37562, #17477, #30672, #1102, #24202, #27641, #33915, #40563, #28288, #20726, #4981, #28076, #11645, #18125, #21370, #41205, #27858, #24847, #17687, #40991, #34554, #18347, #4334, #21153, #8004, #31103, #17906, #23984, #8221, #7797, #31534, #1963, #14227, #15092, #41427, #37126, #27429, #11008, #37777, #37351, #30882, #1317, #11434, #14449, #40782, #14670, #11223, #24422, #34340, #4757, #1535, #31959, #2388, #22018, #15516, #32381, #28721, #35823, #35404, #41846, #8859, #6254, #12286, #25481, #28509, #25891, #15727, #25061, #2806, #25270, #15313, #35189, #38627, #25686, #9267, #9063, #21804, #5620, #22232, #12494, #39045, #29135, #9482, #5410, #5829, #18771, #18983, #32591, #22651, #32170, #41640, #19401, #3016, #31750, #29339, #18560, #2599, #28927, #42064, #16139, #12075, #11863, #38839, #22435, #38416, #35614, #2179, #38203, #6042, #19192, #15937, #42270, #12696, #8648, #34983, #39467, #9901, #29984, #6882, #7098, #17001, #17210, #33228, #13118, #23077, #39257, #42481, #33439, #33006, #3435, #36235, #16783, #10320, #3866, #26103, #39674, #13335, #20034, #36448, #12907, #26732, #26317, #40099, #7308, #9690, #30200, #636, #20250, #13752, #23506, #426, #36656, #6667, #22866, #3657, #36029, #4071, #13548, #6466, #19818, #19608, #16571, #3227, #29773, #216, #26525, #10110, #26942, #23286, #23714, #39886, #10531, #36867, #20459, #33647, #32788, #16350, #29550, #31849, #845, #8169, #1050, #33858, #27375, #1268, #1481, #27806, #14393, #40300, #40510, #27589, #31050, #14824, #4926, #1698, #23934, #40727, #10955, #11170, #8388, #28022, #17636, #17424, #41152, #11590, #7521, #5143, #37077, #24151, #7738, #24367, #24798, #4283, #34719, #20885, #37292, #14174, #34071, #40937, #20672, #21539, #37509, #4703, #21317, #10743, #4493, #37726, #37943, #13964, #30830, #30412, #14617, #7952, #21102, #30621, #27159, #34289, #11380, #17854, #24578, #34506, #18076, #31270, #21960, #28238, #5781, #18291, #35775, #25427, #38571, #38154, #41373, #5994, #2128, #38997, #31912, #35140, #9013, #34930, #25220, #19143, #8803, #25012, #12026, #28460, #5565, #18718, #15468, #32331, #22388, #22181, #5351, #28878, #12234, #2339, #15677, #2757, #38365, #31478, #28669, #9433, #15260, #42011, #35566, #15882, #18506, #11809, #29084, #41798, #31696, #8597, #25841, #35352, #12440, #41593, #18935, #32119, #42221, #2550, #25634, #38793, #9219, #12650, #22598, #1911, #15041, #21751, #19555, #3178, #2966, #6207, #6617, #19983, #16093, #22816, #13494, #19770, #39417, #42432, #3811, #6415, #33172, #20199, #16304, #39620, #29718, #29287, #29500, #23453, #23236, #10058, #162, #9850, #26891, #29932, #36396, #32538, #39206, #26055, #32953, #26682, #16733, #12861, #30143, #9643, #16945, #35977, #16520, #3604, #372, #23027, #582, #32740, #42642, #13070, #36179, #26265, #13285, #26471, #13699, #33388, #6827, #39834, #3383, #10267, #36601, #7048, #40045, #10476, #23667, #19351, #41094, #20406, #17800, #1426, #24521, #30997, #17158, #4015, #11326, #10687, #17370, #11110, #4652, #27749, #33594, #34018, #7681, #1214, #30780, #36815, #21046, #20616, #34450, #1641, #30359, #40884, #37672, #14559, #8112, #21264, #37456, #4869, #4229, #790, #40670, #13913, #11535, #27537, #27108, #14119, #7255, #30571, #40251, #27321, #40456, #1001, #10903, #18017, #24092, #31215, #17581, #37233, #33805, #14769, #20833, #4440, #23880, #27965, #24313, #37030, #7467, #14339, #7899, #34238, #38308, #38516, #22124, #8750, #34662, #34873, #21905, #25370, #9165, #41953, #38735, #18232, #35085, #21692, #5510, #2696, #22335, #11967, #11754, #35511, #5938, #1859, #42166, #31422, #5296, #2072, #18660, #19086, #28183, #29027, #15203, #18451, #8540, #28402, #35299, #14985, #15829, #31858, #41743, #2492, #5086, #31638, #32061, #32272, #8332, #41540, #24741, #8960, #25163, #2290, #15620, #37887, #28823, #21479, #41317, #15413, #28609, #12178, #5729, #18881, #12386, #25582, #24955, #38097, #23179, #6561, #3118, #9998, #13432, #6359, #30092, #19503, #3756, #39152, #36339, #29874, #16676, #42373, #22543, #23397, #32688, #26000, #6149, #20146, #39356, #6771, #9582, #13015, #16247, #313, #35921, #22758, #29447, #102, #19717, #19928, #26628, #12595, #3330, #42589, #26205, #9376, #25787, #9795, #26415, #35716, #29233, #33116, #22973, #36129, #19290, #10212, #12807, #39566, #39778, #32897, #16463, #29660, #32483, #13227, #36547, #3541, #6992, #33330, #16888, #38943, #2909, #16040, #26839, #33540, #20351, #27862, #8444, #11650, #36761, #25065, #39990, #11867, #30304, #11439, #41210, #37999, #17910, #38208, #23616, #17104, #3964, #31107, #739, #8225, #24636, #8654, #15096, #21373, #13861, #21807, #18566, #14886, #529, #13648, #4986, #40995, #37781, #4761, #10423, #31325, #7195, #27057, #34557, #18129, #40201, #10632, #31539, #23817, #34988, #14675, #1540, #1757, #36974, #8010, #1970, #34344, #21157, #28082, #5416, #24850, #21595, #34774, #5195, #18351, #28292, #41431, #15317, #41851, #12912, #32385, #12289, #28725, #39049, #3020, #9488, #29344, #16146, #22655, #2603, #25275, #38421, #8863, #31965, #35408, #41645, #5625, #36033, #28513, #12700, #35828, #19405, #25896, #12081, #22025, #6258, #18776, #25485, #6046, #42277, #32596, #35196, #28932, #15731, #38844, #25693, #31754, #15941, #15521, #42485, #39261, #2392, #26108, #9694, #22871, #6470, #2183, #2810, #38633, #9069, #22236, #35618, #5833, #18988, #22440, #32174, #42068, #12498, #9271, #19196, #29138, #10114, #29778, #23294, #40104, #39680, #850, #433, #36452, #16576, #13969, #6886, #20038, #36241, #33654, #23511, #32797, #10535, #33010, #23081, #219, #33233, #33444, #17008, #3660, #29555, #13339, #16788, #20256, #4077, #36872, #17215, #13122, #29987, #26531, #13552, #40306, #30420, #26739, #6674, #27164, #10748, #39471, #37083, #26321, #39893, #10324, #36660, #23939, #19825, #19612, #7102, #3871, #3439, #30205, #641, #13760, #26947, #23721, #7314, #3231, #20465, #16356, #2, #9905, #7527, #34511, #34076, #5148, #15047, #4290, #11597, #24804, #28030, #37949, #31276, #8175, #18081, #17642, #33863, #11388, #1055, #11815, #40942, #14181, #27594, #25017, #30836, #10959, #40734, #11176, #1273, #24372, #41157, #37516, #31484, #31055, #7957, #4498, #1918, #21107, #34294, #24157, #21544, #24584, #20678, #8394, #20892, #37299, #14400, #4710, #21323, #4931, #17860, #17430, #1486, #14624, #1705, #34724, #18297, #28244, #27380, #27812, #37731, #14829, #41378, #30626, #40516, #7743, #6213, #9440, #15266, #12867, #2133, #18725, #15473, #35358, #19358, #41598, #42440, #28674, #31916, #21965, #41803, #35572, #28466, #16100, #18941, #12445, #15888, #5357, #35147, #2762, #22605, #21757, #5571, #32544, #38798, #2346, #12239, #29090, #35781, #42230, #2972, #29293, #12656, #9020, #31702, #12031, #25224, #38370, #25434, #18514, #8809, #38159, #34936, #19148, #25850, #39004, #32337, #38577, #22185, #8603, #5786, #32124, #2556, #15682, #28884, #42018, #25642, #9225, #22394, #5999, #32749, #6625, #3390, #23243, #36821, #29507, #30367, #16527, #19777, #9858, #29725, #23461, #3185, #4021, #6835, #381, #3819, #35986, #23034, #33395, #40053, #9650, #36188, #7262, #26689, #32962, #170, #16953, #10484, #30151, #23674, #20414, #589, #39626, #19562, #16312, #42650, #26272, #13292, #6422, #13077, #797, #22823, #7056, #13707, #26898, #20206, #39425, #26479, #33602, #10065, #36402, #13501, #36608, #17165, #19989, #33180, #3611, #16740, #29940, #26062, #10274, #39842, #39213, #21489, #10694, #18026, #31221, #34457, #1648, #37679, #14567, #24529, #24102, #40257, #17809, #7473, #18240, #4659, #20622, #34026, #31430, #37241, #17378, #4448, #17589, #7688, #30788, #4878, #1222, #37895, #37464, #14347, #10911, #8339, #27545, #40679, #30578, #27974, #31005, #27115, #14778, #27329, #1009, #20843, #11118, #27756, #11335, #24320, #23889, #7907, #21055, #40892, #41101, #11543, #24749, #33812, #34245, #1434, #8119, #34671, #21271, #5094, #13921, #37037, #4236, #14128, #40463, #15835, #22343, #15422, #38105, #8549, #21700, #2079, #5517, #11763, #18458, #6156, #28191, #25588, #9172, #32279, #38743, #24964, #34882, #19096, #31646, #25172, #18889, #12394, #35519, #41325, #41751, #28619, #8966, #38524, #1867, #28830, #28409, #42174, #9386, #5305, #5948, #2704, #29035, #12601, #25795, #2503, #38951, #11977, #15210, #5736, #41547, #19297, #35306, #38316, #21912, #14993, #8757, #35092, #18668, #31865, #2297, #12186, #22551, #25377, #35726, #22131, #32069, #15627, #41961, #6568, #32904, #6367, #3762, #36347, #2918, #10218, #3126, #35927, #29454, #3338, #3550, #29881, #16470, #42383, #42597, #29668, #33123, #16895, #6999 ),
 ( #7204, #13022, #19510, #9801, #22980, #26214, #36136, #23404, #19724, #13654, #13234, #111, #39364, #26845, #26422, #39573, #32695, #30097, #6778, #16048, #36553, #16254, #10006, #23186, #19935, #16685, #321, #13440, #12815, #26635, #39785, #20151, #535, #33341, #39997, #26008, #10430, #23622, #36767, #32491, #29240, #39159, #9590, #22765, #34398, #40208, #37839, #27063, #954, #40407, #17532, #31164, #23828, #24693, #10852, #14072, #4179, #24043, #17748, #10638, #41046, #1163, #37410, #40839, #30311, #17323, #27700, #4818, #3971, #30526, #1595, #21000, #27267, #37184, #11278, #17964, #24473, #14723, #27915, #37622, #33973, #13867, #36981, #7417, #20567, #7631, #745, #33758, #20357, #17111, #1377, #8065, #21214, #14506, #20784, #4392, #11489, #30733, #14287, #7852, #30944, #33546, #27487, #40622, #11062, #24263, #34190, #4608, #35253, #34827, #5890, #15788, #5040, #12342, #25541, #28780, #38690, #32018, #8917, #18185, #5251, #15579, #22295, #34614, #18403, #32229, #22080, #31592, #2024, #41911, #35467, #9123, #19047, #2655, #28985, #21862, #1811, #14938, #28138, #8493, #11924, #31377, #24904, #12555, #41270, #2446, #42123, #25749, #8280, #11708, #38053, #21428, #21646, #15154, #25329, #18838, #28352, #41488, #5468, #35042, #15367, #2247, #25117, #5688, #38261, #8708, #18617, #31814, #28568, #41698, #12136, #38474, #19884, #39527, #6730, #6315, #22500, #58, #32441, #488, #29613, #2867, #16202, #13602, #19462, #42332, #29403, #42545, #32648, #12968, #16632, #26165, #20096, #19671, #39313, #35881, #33290, #9751, #22932, #12763, #10170, #13182, #9332, #29834, #9542, #25957, #3076, #36086, #9958, #36300, #6521, #6105, #32858, #3287, #23136, #23355, #13393, #36506, #15998, #16417, #26375, #33068, #16843, #6944, #3493, #39103, #3715, #30042, #29193, #38903, #22715, #272, #26585, #39735, #35675, #19250, #31112, #17271, #20517, #10585, #4130, #24211, #3923, #4767, #7582, #1110, #4556, #30679, #39946, #17696, #40156, #30258, #23773, #40360, #40573, #37361, #10801, #36713, #36927, #23991, #27437, #11231, #1327, #40790, #20306, #37134, #7370, #20735, #17916, #24430, #14020, #13816, #37573, #8016, #17060, #1546, #33498, #33705, #30476, #33922, #21162, #697, #26796, #904, #27212, #4346, #17486, #7804, #27008, #10377, #14236, #11016, #30890, #7154, #20952, #34135, #34349, #23567, #14458, #27649, #15324, #24855, #11656, #22032, #28732, #35204, #12296, #41859, #5634, #28300, #8231, #21381, #34564, #14892, #18357, #24643, #31332, #18997, #41000, #38428, #18783, #2399, #8870, #37787, #4993, #31971, #1762, #38006, #31762, #25283, #15529, #11444, #11875, #41437, #21814, #8661, #14679, #41652, #41217, #25493, #22244, #18136, #38641, #9077, #35415, #5840, #32181, #28522, #27866, #8451, #28090, #18575, #21601, #34781, #5423, #5201, #31546, #1978, #15103, #25071, #38215, #34995, #2191, #12089, #3825, #26485, #23679, #33185, #39631, #3395, #36826, #10071, #23248, #35626, #26903, #7268, #4027, #10279, #2609, #15739, #39846, #3617, #16744, #36408, #25701, #23466, #28939, #42076, #26694, #36613, #6053, #22449, #10490, #175, #12506, #29944, #387, #7061, #29729, #6841, #20421, #19994, #32968, #13505, #20211, #33400, #16961, #30157, #33609, #38851, #597, #13296, #13714, #40059, #9278, #19204, #16532, #34925, #16456, #5346, #32892, #25007, #9577, #16240, #3113, #28233, #8382, #9789, #18501, #11805, #34713, #6555, #25216, #39146, #38149, #41588, #31690, #29441, #21745, #8592, #2123, #29229, #6141, #6353, #42582, #41146, #32478, #15253, #28454, #37937, #11584, #12020, #12800, #21532, #15035, #19498, #38937, #9368, #5136, #39348, #41368, #25995, #13007, #22538, #2904, #35710, #18283, #19284, #26200, #16033, #42368, #22751, #35917, #19711, #32683, #22968, #24791, #31472, #1905, #36124, #3322, #40196, #23171, #10839, #26412, #40394, #16670, #39985, #27052, #23813, #3749, #24034, #9992, #3534, #33110, #16883, #29867, #36755, #10416, #37173, #942, #7190, #308, #20139, #39772, #33325, #7409, #6983, #7621, #23609, #30086, #26624, #20774, #525, #13641, #13427, #14061, #33537, #95, #20556, #10206, #23392, #36542, #26833, #735, #10626, #20345, #39561, #3959, #17098, #30298, #27254, #4167, #33963, #36334, #13855, #36966, #33746, #4384, #29654, #17312, #30516, #13218, #6765, #19921, #35032, #24250, #40827, #37612, #14715, #28342, #20991, #21853, #8056, #11269, #1366, #21203, #14930, #37400, #38254, #41038, #34603, #38044, #27475, #14497, #24895, #31583, #1151, #27690, #41480, #18176, #24465, #34389, #8486, #2015, #21639, #15146, #11913, #34819, #31154, #11054, #7843, #34178, #17736, #4807, #40611, #4597, #17523, #14274, #41259, #5242, #18395, #11699, #30930, #17955, #25107, #1587, #27904, #5034, #28128, #8700, #11481, #24683, #37829, #8272, #21418, #30724, #1802, #31368, #26003, #19931, #36764, #39359, #39569, #19720, #7200, #39780, #3544, #42376, #6362, #35923, #106, #23400, #26631, #9585, #39993, #12810, #26842, #3121, #26418, #13435, #13017, #16680, #23182, #36550, #33334, #33543, #6774, #29450, #26209, #39154, #16043, #16466, #29877, #22761, #32691, #6995, #29662, #6563, #19506, #13651, #16250, #316, #30094, #9797, #33119, #10001, #42592, #22976, #10215, #20354, #36132, #36342, #32900, #29236, #20148, #3759, #3333, #13230, #16891, #531, #10426, #23619, #40204, #28515, #742, #15319, #33754, #14282, #1374, #40835, #20781, #41647, #27060, #20564, #7414, #33969, #4176, #11059, #27484, #12083, #18569, #24258, #17320, #25278, #22027, #17744, #3968, #17107, #7849, #30731, #1160, #7627, #13864, #34184, #30307, #10635, #37407, #20997, #23821, #36977, #34990, #30523, #38423, #17529, #4389, #4605, #951, #10849, #5418, #37180, #14069, #40402, #27262, #40619, #30938, #14503, #31756, #8657, #27697, #24041, #11869, #25067, #38210, #21809, #2186, #8865, #9907, #42071, #26323, #18990, #3022, #9696, #39263, #22238, #2394, #3233, #28934, #5835, #28727, #4, #19198, #32598, #32176, #35620, #12501, #22875, #15734, #2605, #38636, #9273, #9071, #42279, #2812, #13125, #6472, #12702, #35410, #29557, #35198, #6262, #5628, #18778, #39051, #32388, #15944, #38846, #15523, #22657, #31967, #41854, #25898, #9490, #12291, #25487, #36035, #25695, #39474, #6048, #22442, #35830, #29140, #19408, #19614, #16148, #29346, #42487, #12914, #26110, #32799, #16358, #10750, #27166, #30207, #39682, #33656, #17010, #13554, #20468, #23941, #16790, #40518, #29990, #14183, #6888, #4079, #40308, #37086, #10116, #33012, #33866, #435, #36454, #16578, #30628, #7104, #17217, #20041, #23514, #26741, #7529, #3662, #33236, #39895, #10537, #643, #30422, #20680, #23083, #13762, #10326, #36663, #19827, #36243, #20259, #36874, #3441, #23296, #853, #33446, #3874, #29781, #4292, #26950, #7316, #17432, #40106, #23723, #13971, #221, #13342, #1057, #27382, #6676, #26533, #14627, #31704, #34727, #41159, #37302, #1275, #30838, #37733, #18299, #21547, #4500, #34938, #7746, #21760, #40737, #21325, #8397, #5150, #27814, #5359, #34078, #27597, #34513, #18516, #25019, #31278, #11179, #2135, #28469, #24806, #10962, #24159, #14831, #8177, #4934, #40944, #20894, #11599, #17644, #14402, #18084, #1707, #24374, #37518, #41380, #7959, #15269, #24586, #11390, #28032, #21109, #17862, #11818, #1491, #34296, #4712, #31057, #37951, #31486, #1920, #38161, #15049, #28246, #8606, #9443, #35573, #32126, #39006, #42442, #35361, #16313, #5788, #32750, #25436, #22607, #16102, #2975, #28676, #8811, #9652, #18942, #12242, #35149, #6424, #25643, #35784, #38578, #42020, #2559, #29295, #22188, #9022, #15684, #29093, #6002, #6215, #12869, #41599, #32339, #28887, #12447, #38373, #12033, #38800, #12658, #21967, #15475, #19361, #9227, #22396, #5573, #39215, #41806, #25852, #26064, #19150, #2765, #15890, #18727, #31919, #42232, #19565, #32546, #22825, #35989, #3186, #25226, #2348, #13078, #19779, #6628, #13502, #36822, #40055, #23035, #10696, #26274, #40259, #16529, #39843, #26899, #23675, #3614, #23890, #9861, #3392, #32963, #16742, #29726, #36609, #26482, #16956, #7057, #7264, #4023, #4237, #20207, #172, #39628, #39427, #29509, #29941, #592, #36190, #13293, #20416, #383, #19991, #10067, #27117, #23245, #13710, #799, #36404, #33396, #10276, #6838, #33182, #3820, #7474, #26690, #23462, #30153, #20625, #10486, #33604, #17167, #30369, #13923, #37038, #33813, #42653, #10912, #41326, #14129, #28193, #4449, #27757, #14779, #11544, #34247, #11764, #40464, #34027, #20844, #4660, #17590, #24530, #40893, #24965, #31431, #37680, #30789, #38106, #34883, #31223, #17379, #30579, #21272, #1435, #14568, #21056, #27330, #4879, #1010, #24104, #8120, #34459, #37243, #7689, #5095, #1223, #8550, #31006, #17810, #18027, #14348, #24321, #18241, #7908, #27547, #11119, #40680, #11336, #1649, #27975, #1868, #21490, #41102, #37465, #24750, #37897, #8340, #34672, #14994, #21701, #22766, #12187, #39160, #31866, #15837, #22552, #9387, #35093, #15211, #16050, #41752, #18669, #41548, #12817, #32070, #2705, #2298, #5737, #25378, #35727, #28620, #15423, #25589, #5519, #42384, #5306, #19098, #18459, #31647, #9173, #2504, #15628, #8967, #28410, #35520, #2081, #11978, #12395, #38744, #25174, #38317, #6157, #38525, #26009, #18890, #22133, #22344, #21913, #35307, #19298, #28831, #8758, #41962, #5949, #32280, #29036, #42175, #32492, #2919, #12602, #25796, #38952, #29241, #9591, #33342, #36768, #29670, #10639, #113, #27064, #19725, #3763, #10432, #39999, #22981, #3127, #3972, #13235, #39786, #536, #7205, #13655, #33547, #20358, #26846, #6780, #29455, #42598, #13024, #36137, #39574, #16255, #9802, #40209, #19511, #16896, #23623, #17112, #30098, #26216, #39365, #30312, #6569, #16471, #10219, #746, #13868, #32696, #33125, #19936, #322, #29882, #35928, #20152, #32905, #3339, #6368, #13441, #26423, #10008, #23187, #36348, #3552, #36554, #16686, #26636, #23405, #7001, #17325, #28139, #14508, #30527, #1164, #41272, #4393, #27269, #14288, #27488, #33974, #40623, #1596, #11064, #5041, #4609, #24265, #20786, #18186, #37411, #7853, #21001, #21215, #24694, #17533, #23830, #30734, #14939, #7633, #34399, #41047, #27916, #10853, #33759, #34191, #37185, #1812, #17749, #31378, #30945, #4819, #1378, #27702, #40840, #11490, #11279, #24474, #37624, #8066, #17966, #31166, #37840, #36982, #14724, #8281, #21430, #20568, #7418, #34615, #4180, #955, #40408, #14073, #24044, #2249, #5252, #9333, #11925, #25542, #25750, #21863, #2447, #35255, #34828, #21647, #15580, #32442, #35043, #5690, #15368, #2869, #35468, #41912, #38054, #2025, #31593, #38475, #19048, #22296, #18404, #35676, #8494, #22501, #41490, #22081, #9125, #5891, #28569, #6106, #15155, #28353, #25118, #41699, #38262, #18839, #32019, #19252, #38904, #28781, #8709, #15999, #29194, #38692, #11709, #24906, #12343, #8919, #32230, #12137, #5470, #2656, #18618, #31816, #15790, #28986, #25330, #42125, #12557, #26167, #20308, #13184, #16418, #33069, #16203, #6522, #491, #32859, #6317, #36087, #9753, #29615, #3289, #39528, #30044, #3717, #6731, #29406, #10171, #36301, #39314, #22934, #29836, #19886, #6945, #16846, #17062, #3494, #12969, #19672, #39104, #42333, #59, #13394, #9543, #42546, #20098, #26377, #9959, #35882, #39948, #23137, #26586, #13604, #16634, #273, #39737, #22717, #19464, #23356, #33501, #36508, #33291, #26798, #3925, #10380, #23569, #25958, #32649, #3077, #36716, #7156, #12764, #23776, #11446, #27011, #41002, #17273, #40576, #27651, #24432, #4348, #24646, #10588, #4132, #33707, #17489, #30478, #37363, #11019, #37789, #1548, #7806, #907, #8233, #4997, #1329, #30260, #699, #34139, #14238, #27439, #33924, #40158, #17698, #13818, #36929, #20954, #4558, #7373, #20519, #17918, #14022, #21383, #1112, #30682, #30892, #27216, #37136, #31115, #20737, #40362, #23994, #10803, #24212, #14461, #40792, #14681, #34351, #11233, #7584, #37575, #8020, #21164, #4769, #27868, #34566, #35629, #25073, #9280, #1981, #28734, #35417, #22246, #5204, #28092, #21816, #31548, #38853, #5425, #25703, #2193, #15531, #15105, #18577, #38218, #5842, #41439, #12509, #18138, #31973, #31334, #1765, #22034, #15326, #28524, #34997, #41219, #5636, #14894, #11658, #25285, #38430, #38008, #24857, #18999, #28302, #22451, #31764, #41655, #8872, #34783, #8663, #32183, #12092, #8453, #11877, #35206, #18785, #2401, #41861, #2611, #15741, #12298, #18359, #25495, #38645, #9079, #28941, #42078, #21604, #24110, #12919, #40469, #32605, #17174, #23896, #10701, #35835, #15950, #9703, #19415, #27335, #36041, #14135, #32807, #4028, #3029, #6477, #26114, #37043, #29353, #16156, #42492, #36827, #13133, #13927, #7481, #6055, #39480, #39268, #22882, #2818 ) ),
 .UNSPECIFIED., .F., .F., .F. ) 
 B_SPLINE_SURFACE_WITH_KNOTS ( ( 2, 2 ),
 ( 3, 2, 2, 2, 2, 2, 2, 2, 2, 2, 2, 2, 2, 2, 2, 2, 2, 2, 2, 2, 2, 2, 2, 2, 2, 2, 2, 2, 2, 2, 2, 2, 2, 2, 2, 2, 2, 2, 2, 2, 2, 2, 2, 2, 2, 2, 2, 2, 2, 2, 2, 2, 2, 2, 2, 2, 2, 2, 2, 2, 2, 2, 2, 2, 2, 2, 2, 2, 2, 2, 2, 2, 2, 2, 2, 2, 2, 2, 2, 2, 2, 2, 2, 2, 2, 2, 2, 2, 2, 2, 2, 2, 2, 2, 2, 2, 2, 2, 2, 2, 2, 2, 2, 2, 2, 2, 2, 2, 2, 2, 2, 2, 2, 2, 2, 2, 2, 2, 2, 2, 2, 2, 2, 2, 2, 2, 2, 2, 2, 2, 2, 2, 2, 2, 2, 2, 2, 2, 2, 2, 2, 2, 2, 2, 2, 2, 2, 2, 2, 2, 2, 2, 2, 2, 2, 2, 2, 2, 2, 2, 2, 2, 2, 2, 2, 2, 2, 2, 2, 2, 2, 2, 2, 2, 2, 2, 2, 2, 2, 2, 2, 2, 2, 2, 2, 2, 2, 2, 2, 2, 2, 2, 2, 2, 2, 2, 2, 2, 2, 2, 2, 2, 2, 2, 2, 2, 2, 2, 2, 2, 2, 2, 2, 2, 2, 2, 2, 2, 2, 2, 2, 2, 2, 2, 2, 2, 2, 2, 2, 2, 2, 2, 2, 2, 2, 2, 2, 2, 2, 2, 2, 2, 2, 2, 2, 2, 2, 2, 2, 2, 2, 2, 2, 2, 2, 2, 2, 2, 2, 2, 2, 2, 2, 2, 2, 2, 2, 2, 2, 2, 2, 2, 2, 2, 2, 2, 2, 2, 2, 2, 2, 2, 2, 2, 2, 2, 2, 2, 2, 2, 2, 2, 2, 2, 2, 2, 2, 2, 2, 2, 2, 2, 2, 2, 2, 2, 2, 2, 2, 2, 2, 2, 2, 2, 2, 2, 2, 2, 2, 2, 2, 2, 2, 2, 2, 2, 2, 2, 2, 2, 2, 2, 2, 2, 2, 2, 2, 2, 2, 2, 2, 2, 2, 2, 2, 2, 2, 2, 2, 2, 2, 2, 2, 2, 2, 2, 2, 2, 2, 2, 2, 2, 2, 2, 2, 2, 2, 2, 2, 2, 2, 2, 2, 2, 2, 2, 2, 2, 2, 2, 2, 2, 2, 2, 2, 2, 2, 2, 2, 2, 2, 2, 2, 2, 2, 2, 2, 2, 2, 2, 2, 2, 2, 2, 2, 2, 2, 2, 2, 2, 2, 2, 2, 2, 2, 2, 2, 2, 2, 2, 2, 2, 2, 2, 2, 2, 2, 2, 2, 2, 2, 2, 2, 2, 2, 2, 2, 2, 2, 2, 2, 2, 2, 2, 2, 2, 2, 2, 2, 2, 2, 2, 2, 2, 2, 2, 2, 2, 2, 2, 2, 2, 2, 2, 2, 2, 2, 2, 2, 2, 2, 2, 2, 2, 2, 2, 2, 2, 2, 2, 2, 2, 2, 2, 2, 2, 2, 2, 2, 2, 2, 2, 2, 2, 2, 2, 2, 2, 2, 2, 2, 2, 2, 2, 2, 2, 2, 2, 2, 2, 2, 2, 2, 2, 2, 2, 2, 2, 2, 2, 2, 2, 2, 2, 2, 2, 2, 2, 2, 2, 2, 2, 2, 2, 2, 2, 2, 2, 2, 2, 2, 2, 2, 2, 2, 2, 2, 2, 2, 2, 2, 2, 2, 2, 2, 2, 2, 2, 2, 2, 2, 2, 2, 2, 2, 2, 2, 2, 2, 2, 2, 2, 2, 2, 2, 2, 2, 2, 2, 2, 2, 2, 2, 2, 2, 2, 2, 2, 2, 2, 2, 2, 2, 2, 2, 2, 2, 2, 2, 2, 2, 2, 2, 2, 2, 2, 2, 2, 2, 2, 2, 2, 2, 2, 2, 2, 2, 2, 2, 2, 2, 2, 2, 2, 2, 2, 2, 2, 2, 2, 2, 2, 2, 2, 2, 2, 2, 2, 2, 2, 2, 2, 2, 2, 2, 2, 2, 2, 2, 2, 2, 2, 2, 2, 2, 2, 2, 2, 2, 2, 2, 2, 2, 2, 2, 2, 2, 2, 2, 2, 2, 2, 2, 2, 2, 2, 2, 2, 2, 2, 2, 2, 2, 2, 2, 2, 2, 2, 2, 2, 2, 2, 2, 2, 2, 2, 2, 2, 2, 2, 2, 2, 2, 2, 2, 2, 2, 2, 2, 2, 2, 2, 2, 2, 2, 2, 2, 2, 2, 2, 2, 2, 2, 2, 2, 2, 2, 2, 2, 2, 2, 2, 2, 2, 2, 2, 2, 2, 2, 2, 2, 2, 2, 2, 2, 2, 2, 2, 2, 2, 2, 2, 2, 2, 2, 2, 2, 2, 2, 2, 2, 2, 2, 2, 2, 2, 2, 2, 2, 2, 2, 2, 2, 2, 2, 2, 2, 2, 2, 2, 2, 2, 2, 2, 2, 2, 2, 2, 2, 2, 2, 2, 2, 2, 2, 2, 2, 2, 2, 2, 3 ),
 ( 0.000000000000000000, 1.000000000000000000 ),
 ( 0.000000000000000000, 0.001243781094527363160, 0.002487562189054726321, 0.003731343283582089481, 0.004975124378109452641, 0.006218905472636816235, 0.007462686567164178962, 0.008706467661691542556, 0.009950248756218905283, 0.01119402985074626801, 0.01243781094527363247, 0.01368159203980099520, 0.01492537313432835792, 0.01616915422885572065, 0.01741293532338308511, 0.01865671641791044610, 0.01990049751243781057, 0.02114427860696517503, 0.02238805970149253602, 0.02363184079601990048, 0.02487562189054726494, 0.02611940298507462593, 0.02736318407960199039, 0.02860696517412935486, 0.02985074626865671585, 0.03109452736318408031, 0.03233830845771144130, 0.03358208955223880576, 0.03482587064676617022, 0.03606965174129353469, 0.03731343283582089221, 0.03855721393034825667, 0.03980099502487562113, 0.04104477611940298559, 0.04228855721393035005, 0.04353233830845771452, 0.04477611940298507204, 0.04601990049751243650, 0.04726368159203980096, 0.04850746268656716542, 0.04975124378109452988, 0.05099502487562188741, 0.05223880597014925187, 0.05348258706467661633, 0.05472636815920398079, 0.05597014925373134525, 0.05721393034825870971, 0.05845771144278606724, 0.05970149253731343170, 0.06094527363184079616, 0.06218905472636816062, 0.06343283582089552508, 0.06467661691542288260, 0.06592039800995025400, 0.06716417910447761153, 0.06840796019900496905, 0.06965174129353234045, 0.07089552238805969797, 0.07213930348258706937, 0.07338308457711442689, 0.07462686567164178442, 0.07587064676616915582, 0.07711442786069651334, 0.07835820895522388474, 0.07960199004975124226, 0.08084577114427861366, 0.08208955223880597118, 0.08333333333333332871, 0.08457711442786070011, 0.08582089552238805763, 0.08706467661691542903, 0.08830845771144278655, 0.08955223880597014408, 0.09079601990049751548, 0.09203980099502487300, 0.09328358208955224440, 0.09452736318407960192, 0.09577114427860695944, 0.09701492537313433084, 0.09825870646766168837, 0.09950248756218905977, 0.1007462686567164173, 0.1019900497512437748, 0.1032338308457711462, 0.1044776119402985037, 0.1057213930348258751, 0.1069651741293532327, 0.1082089552238805902, 0.1094527363184079616, 0.1106965174129353191, 0.1119402985074626905, 0.1131840796019900480, 0.1144278606965174194, 0.1156716417910447769, 0.1169154228855721345, 0.1181592039800995059, 0.1194029850746268634, 0.1206467661691542348, 0.1218905472636815923, 0.1231343283582089498, 0.1243781094527363212, 0.1256218905472636926, 0.1268656716417910502, 0.1281094527363184077, 0.1293532338308457652, 0.1305970149253731227, 0.1318407960199005080, 0.1330845771144278655, 0.1343283582089552231, 0.1355721393034825806, 0.1368159203980099381, 0.1380597014925373234, 0.1393034825870646809, 0.1405472636815920384, 0.1417910447761193959, 0.1430348258706467535, 0.1442786069651741387, 0.1455223880597014963, 0.1467661691542288538, 0.1480099502487562113, 0.1492537313432835688, 0.1504975124378109541, 0.1517412935323383116, 0.1529850746268656692, 0.1542288557213930267, 0.1554726368159203842, 0.1567164179104477695, 0.1579601990049751270, 0.1592039800995024845, 0.1604477611940298420, 0.1616915422885572273, 0.1629353233830845848, 0.1641791044776119424, 0.1654228855721392999, 0.1666666666666666574, 0.1679104477611940427, 0.1691542288557214002, 0.1703980099502487577, 0.1716417910447761153, 0.1728855721393034728, 0.1741293532338308581, 0.1753731343283582156, 0.1766169154228855731, 0.1778606965174129306, 0.1791044776119402882, 0.1803482587064676734, 0.1815920398009950310, 0.1828358208955223885, 0.1840796019900497460, 0.1853233830845771035, 0.1865671641791044888, 0.1878109452736318463, 0.1890547263681592038, 0.1902985074626865614, 0.1915422885572139189, 0.1927860696517413042, 0.1940298507462686617, 0.1952736318407960192, 0.1965174129353233767, 0.1977611940298507343, 0.1990049751243781195, 0.2002487562189054771, 0.2014925373134328346, 0.2027363184079601921, 0.2039800995024875496, 0.2052238805970149349, 0.2064676616915422924, 0.2077114427860696499, 0.2089552238805970075, 0.2101990049751243650, 0.2114427860696517503, 0.2126865671641791078, 0.2139303482587064653, 0.2151741293532338228, 0.2164179104477611804, 0.2176616915422885656, 0.2189054726368159232, 0.2201492537313432807, 0.2213930348258706382, 0.2226368159203980235, 0.2238805970149253810, 0.2251243781094527385, 0.2263681592039800961, 0.2276119402985074536, 0.2288557213930348389, 0.2300995024875621964, 0.2313432835820895539, 0.2325870646766169114, 0.2338308457711442689, 0.2350746268656716542, 0.2363184079601990117, 0.2375621890547263693, 0.2388059701492537268, 0.2400497512437810843, 0.2412935323383084696, 0.2425373134328358271, 0.2437810945273631846, 0.2450248756218905422, 0.2462686567164178997, 0.2475124378109452850, 0.2487562189054726425, 0.2500000000000000000, 0.2512437810945273853, 0.2524875621890547150, 0.2537313432835821003, 0.2549751243781094301, 0.2562189054726368154, 0.2574626865671642006, 0.2587064676616915304, 0.2599502487562189157, 0.2611940298507462455, 0.2624378109452736307, 0.2636815920398010160, 0.2649253731343283458, 0.2661691542288557311, 0.2674129353233830608, 0.2686567164179104461, 0.2699004975124378314, 0.2711442786069651611, 0.2723880597014925464, 0.2736318407960198762, 0.2748756218905472615, 0.2761194029850746468, 0.2773631840796019765, 0.2786069651741293618, 0.2798507462686566916, 0.2810945273631840768, 0.2823383084577114621, 0.2835820895522387919, 0.2848258706467661772, 0.2860696517412935069, 0.2873134328358208922, 0.2885572139303482775, 0.2898009950248756073, 0.2910447761194029925, 0.2922885572139303223, 0.2935323383084577076, 0.2947761194029850929, 0.2960199004975124226, 0.2972636815920398079, 0.2985074626865671377, 0.2997512437810945229, 0.3009950248756219082, 0.3022388059701492380, 0.3034825870646766233, 0.3047263681592039530, 0.3059701492537313383, 0.3072139303482587236, 0.3084577114427860534, 0.3097014925373134386, 0.3109452736318407684, 0.3121890547263681537, 0.3134328358208955390, 0.3146766169154228687, 0.3159203980099502540, 0.3171641791044776393, 0.3184079601990049690, 0.3196517412935323543, 0.3208955223880596841, 0.3221393034825870694, 0.3233830845771144546, 0.3246268656716417844, 0.3258706467661691697, 0.3271144278606964995, 0.3283582089552238847, 0.3296019900497512700, 0.3308457711442785998, 0.3320895522388059851, 0.3333333333333333148, 0.3345771144278607001, 0.3358208955223880854, 0.3370646766169154152, 0.3383084577114428004, 0.3395522388059701302, 0.3407960199004975155, 0.3420398009950249008, 0.3432835820895522305, 0.3445273631840796158, 0.3457711442786069456, 0.3470149253731343308, 0.3482587064676617161, 0.3495024875621890459, 0.3507462686567164312, 0.3519900497512437609, 0.3532338308457711462, 0.3544776119402985315, 0.3557213930348258613, 0.3569651741293532465, 0.3582089552238805763, 0.3594527363184079616, 0.3606965174129353469, 0.3619402985074626766, 0.3631840796019900619, 0.3644278606965173917, 0.3656716417910447769, 0.3669154228855721622, 0.3681592039800994920, 0.3694029850746268773, 0.3706467661691542070, 0.3718905472636815923, 0.3731343283582089776, 0.3743781094527363074, 0.3756218905472636926, 0.3768656716417910224, 0.3781094527363184077, 0.3793532338308457930, 0.3805970149253731227, 0.3818407960199005080, 0.3830845771144278378, 0.3843283582089552231, 0.3855721393034826083, 0.3868159203980099381, 0.3880597014925373234, 0.3893034825870646531, 0.3905472636815920384, 0.3917910447761194237, 0.3930348258706467535, 0.3942786069651741387, 0.3955223880597014685, 0.3967661691542288538, 0.3980099502487562391, 0.3992537313432835688, 0.4004975124378109541, 0.4017412935323382839, 0.4029850746268656692, 0.4042288557213930544, 0.4054726368159203842, 0.4067164179104477695, 0.4079601990049750992, 0.4092039800995024845, 0.4104477611940298698, 0.4116915422885571996, 0.4129353233830845848, 0.4141791044776119146, 0.4154228855721392999, 0.4166666666666666852, 0.4179104477611940149, 0.4191542288557214002, 0.4203980099502487300, 0.4216417910447761153, 0.4228855721393035005, 0.4241293532338308303, 0.4253731343283582156, 0.4266169154228855454, 0.4278606965174129306, 0.4291044776119403159, 0.4303482587064676457, 0.4315920398009950310, 0.4328358208955223607, 0.4340796019900497460, 0.4353233830845771313, 0.4365671641791044610, 0.4378109452736318463, 0.4390547263681592316, 0.4402985074626865614, 0.4415422885572139466, 0.4427860696517412764, 0.4440298507462686617, 0.4452736318407960470, 0.4465174129353233767, 0.4477611940298507620, 0.4490049751243780918, 0.4502487562189054771, 0.4514925373134328623, 0.4527363184079601921, 0.4539800995024875774, 0.4552238805970149071, 0.4564676616915422924, 0.4577114427860696777, 0.4589552238805970075, 0.4601990049751243927, 0.4614427860696517225, 0.4626865671641791078, 0.4639303482587064931, 0.4651741293532338228, 0.4664179104477612081, 0.4676616915422885379, 0.4689054726368159232, 0.4701492537313433084, 0.4713930348258706382, 0.4726368159203980235, 0.4738805970149253532, 0.4751243781094527385, 0.4763681592039801238, 0.4776119402985074536, 0.4788557213930348389, 0.4800995024875621686, 0.4813432835820895539, 0.4825870646766169392, 0.4838308457711442689, 0.4850746268656716542, 0.4863184079601989840, 0.4875621890547263693, 0.4888059701492537545, 0.4900497512437810843, 0.4912935323383084696, 0.4925373134328357994, 0.4937810945273631846, 0.4950248756218905699, 0.4962686567164178997, 0.4975124378109452850, 0.4987562189054726147, 0.5000000000000000000, 0.5012437810945273853, 0.5024875621890547706, 0.5037313432835820448, 0.5049751243781094301, 0.5062189054726368154, 0.5074626865671642006, 0.5087064676616915859, 0.5099502487562188602, 0.5111940298507462455, 0.5124378109452736307, 0.5136815920398010160, 0.5149253731343284013, 0.5161691542288556755, 0.5174129353233830608, 0.5186567164179104461, 0.5199004975124378314, 0.5211442786069652167, 0.5223880597014924909, 0.5236318407960198762, 0.5248756218905472615, 0.5261194029850746468, 0.5273631840796020320, 0.5286069651741293063, 0.5298507462686566916, 0.5310945273631840768, 0.5323383084577114621, 0.5335820895522388474, 0.5348258706467661217, 0.5360696517412935069, 0.5373134328358208922, 0.5385572139303482775, 0.5398009950248756628, 0.5410447761194029370, 0.5422885572139303223, 0.5435323383084577076, 0.5447761194029850929, 0.5460199004975124781, 0.5472636815920397524, 0.5485074626865671377, 0.5497512437810945229, 0.5509950248756219082, 0.5522388059701492935, 0.5534825870646765678, 0.5547263681592039530, 0.5559701492537313383, 0.5572139303482587236, 0.5584577114427861089, 0.5597014925373133831, 0.5609452736318407684, 0.5621890547263681537, 0.5634328358208955390, 0.5646766169154229242, 0.5659203980099501985, 0.5671641791044775838, 0.5684079601990049690, 0.5696517412935323543, 0.5708955223880597396, 0.5721393034825870139, 0.5733830845771143991, 0.5746268656716417844, 0.5758706467661691697, 0.5771144278606965550, 0.5783582089552238292, 0.5796019900497512145, 0.5808457711442785998, 0.5820895522388059851, 0.5833333333333333703, 0.5845771144278606446, 0.5858208955223880299, 0.5870646766169154152, 0.5883084577114428004, 0.5895522388059701857, 0.5907960199004974600, 0.5920398009950248452, 0.5932835820895522305, 0.5945273631840796158, 0.5957711442786070011, 0.5970149253731342753, 0.5982587064676616606, 0.5995024875621890459, 0.6007462686567164312, 0.6019900497512438164, 0.6032338308457710907, 0.6044776119402984760, 0.6057213930348258613, 0.6069651741293532465, 0.6082089552238806318, 0.6094527363184079061, 0.6106965174129352913, 0.6119402985074626766, 0.6131840796019900619, 0.6144278606965174472, 0.6156716417910447214, 0.6169154228855721067, 0.6181592039800994920, 0.6194029850746268773, 0.6206467661691542625, 0.6218905472636815368, 0.6231343283582089221, 0.6243781094527363074, 0.6256218905472636926, 0.6268656716417910779, 0.6281094527363184632, 0.6293532338308457375, 0.6305970149253731227, 0.6318407960199005080, 0.6330845771144278933, 0.6343283582089552786, 0.6355721393034825528, 0.6368159203980099381, 0.6380597014925373234, 0.6393034825870647087, 0.6405472636815920939, 0.6417910447761193682, 0.6430348258706467535, 0.6442786069651741387, 0.6455223880597015240, 0.6467661691542289093, 0.6480099502487561836, 0.6492537313432835688, 0.6504975124378109541, 0.6517412935323383394, 0.6529850746268657247, 0.6542288557213929989, 0.6554726368159203842, 0.6567164179104477695, 0.6579601990049751548, 0.6592039800995025400, 0.6604477611940298143, 0.6616915422885571996, 0.6629353233830845848, 0.6641791044776119701, 0.6654228855721393554, 0.6666666666666666297, 0.6679104477611940149, 0.6691542288557214002, 0.6703980099502487855, 0.6716417910447761708, 0.6728855721393034450, 0.6741293532338308303, 0.6753731343283582156, 0.6766169154228856009, 0.6778606965174129861, 0.6791044776119402604, 0.6803482587064676457, 0.6815920398009950310, 0.6828358208955224162, 0.6840796019900498015, 0.6853233830845770758, 0.6865671641791044610, 0.6878109452736318463, 0.6890547263681592316, 0.6902985074626866169, 0.6915422885572138911, 0.6927860696517412764, 0.6940298507462686617, 0.6952736318407960470, 0.6965174129353234322, 0.6977611940298507065, 0.6990049751243780918, 0.7002487562189054771, 0.7014925373134328623, 0.7027363184079602476, 0.7039800995024875219, 0.7052238805970149071, 0.7064676616915422924, 0.7077114427860696777, 0.7089552238805970630, 0.7101990049751243372, 0.7114427860696517225, 0.7126865671641791078, 0.7139303482587064931, 0.7151741293532338783, 0.7164179104477611526, 0.7176616915422885379, 0.7189054726368159232, 0.7201492537313433084, 0.7213930348258706937, 0.7226368159203979680, 0.7238805970149253532, 0.7251243781094527385, 0.7263681592039801238, 0.7276119402985075091, 0.7288557213930347833, 0.7300995024875621686, 0.7313432835820895539, 0.7325870646766169392, 0.7338308457711443245, 0.7350746268656715987, 0.7363184079601989840, 0.7375621890547263693, 0.7388059701492537545, 0.7400497512437811398, 0.7412935323383084141, 0.7425373134328357994, 0.7437810945273631846, 0.7450248756218905699, 0.7462686567164179552, 0.7475124378109452294, 0.7487562189054726147, 0.7500000000000000000, 0.7512437810945273853, 0.7524875621890547706, 0.7537313432835820448, 0.7549751243781094301, 0.7562189054726368154, 0.7574626865671642006, 0.7587064676616915859, 0.7599502487562188602, 0.7611940298507462455, 0.7624378109452736307, 0.7636815920398010160, 0.7649253731343284013, 0.7661691542288556755, 0.7674129353233830608, 0.7686567164179104461, 0.7699004975124378314, 0.7711442786069652167, 0.7723880597014924909, 0.7736318407960198762, 0.7748756218905472615, 0.7761194029850746468, 0.7773631840796020320, 0.7786069651741293063, 0.7798507462686566916, 0.7810945273631840768, 0.7823383084577114621, 0.7835820895522388474, 0.7848258706467661217, 0.7860696517412935069, 0.7873134328358208922, 0.7885572139303482775, 0.7898009950248756628, 0.7910447761194029370, 0.7922885572139303223, 0.7935323383084577076, 0.7947761194029850929, 0.7960199004975124781, 0.7972636815920397524, 0.7985074626865671377, 0.7997512437810945229, 0.8009950248756219082, 0.8022388059701492935, 0.8034825870646765678, 0.8047263681592039530, 0.8059701492537313383, 0.8072139303482587236, 0.8084577114427861089, 0.8097014925373133831, 0.8109452736318407684, 0.8121890547263681537, 0.8134328358208955390, 0.8146766169154229242, 0.8159203980099501985, 0.8171641791044775838, 0.8184079601990049690, 0.8196517412935323543, 0.8208955223880597396, 0.8221393034825870139, 0.8233830845771143991, 0.8246268656716417844, 0.8258706467661691697, 0.8271144278606965550, 0.8283582089552238292, 0.8296019900497512145, 0.8308457711442785998, 0.8320895522388059851, 0.8333333333333333703, 0.8345771144278606446, 0.8358208955223880299, 0.8370646766169154152, 0.8383084577114428004, 0.8395522388059701857, 0.8407960199004974600, 0.8420398009950248452, 0.8432835820895522305, 0.8445273631840796158, 0.8457711442786070011, 0.8470149253731342753, 0.8482587064676616606, 0.8495024875621890459, 0.8507462686567164312, 0.8519900497512438164, 0.8532338308457710907, 0.8544776119402984760, 0.8557213930348258613, 0.8569651741293532465, 0.8582089552238806318, 0.8594527363184079061, 0.8606965174129352913, 0.8619402985074626766, 0.8631840796019900619, 0.8644278606965174472, 0.8656716417910447214, 0.8669154228855721067, 0.8681592039800994920, 0.8694029850746268773, 0.8706467661691542625, 0.8718905472636815368, 0.8731343283582089221, 0.8743781094527363074, 0.8756218905472636926, 0.8768656716417910779, 0.8781094527363184632, 0.8793532338308457375, 0.8805970149253731227, 0.8818407960199005080, 0.8830845771144278933, 0.8843283582089552786, 0.8855721393034825528, 0.8868159203980099381, 0.8880597014925373234, 0.8893034825870647087, 0.8905472636815920939, 0.8917910447761193682, 0.8930348258706467535, 0.8942786069651741387, 0.8955223880597015240, 0.8967661691542289093, 0.8980099502487561836, 0.8992537313432835688, 0.9004975124378109541, 0.9017412935323383394, 0.9029850746268657247, 0.9042288557213929989, 0.9054726368159203842, 0.9067164179104477695, 0.9079601990049751548, 0.9092039800995025400, 0.9104477611940298143, 0.9116915422885571996, 0.9129353233830845848, 0.9141791044776119701, 0.9154228855721393554, 0.9166666666666666297, 0.9179104477611940149, 0.9191542288557214002, 0.9203980099502487855, 0.9216417910447761708, 0.9228855721393034450, 0.9241293532338308303, 0.9253731343283582156, 0.9266169154228856009, 0.9278606965174129861, 0.9291044776119402604, 0.9303482587064676457, 0.9315920398009950310, 0.9328358208955224162, 0.9340796019900498015, 0.9353233830845770758, 0.9365671641791044610, 0.9378109452736318463, 0.9390547263681592316, 0.9402985074626866169, 0.9415422885572138911, 0.9427860696517412764, 0.9440298507462686617, 0.9452736318407960470, 0.9465174129353234322, 0.9477611940298507065, 0.9490049751243780918, 0.9502487562189054771, 0.9514925373134328623, 0.9527363184079602476, 0.9539800995024875219, 0.9552238805970149071, 0.9564676616915422924, 0.9577114427860696777, 0.9589552238805970630, 0.9601990049751243372, 0.9614427860696517225, 0.9626865671641791078, 0.9639303482587064931, 0.9651741293532338783, 0.9664179104477611526, 0.9676616915422885379, 0.9689054726368159232, 0.9701492537313433084, 0.9713930348258706937, 0.9726368159203979680, 0.9738805970149253532, 0.9751243781094527385, 0.9763681592039801238, 0.9776119402985075091, 0.9788557213930347833, 0.9800995024875621686, 0.9813432835820895539, 0.9825870646766169392, 0.9838308457711443245, 0.9850746268656715987, 0.9863184079601989840, 0.9875621890547263693, 0.9888059701492537545, 0.9900497512437811398, 0.9912935323383084141, 0.9925373134328357994, 0.9937810945273631846, 0.9950248756218905699 ),
 .UNSPECIFIED. ) 
 GEOMETRIC_REPRESENTATION_ITEM ( )  RATIONAL_B_SPLINE_SURFACE ( (
 ( 1.000000000000000000, 0.8660254037844387076, 1.000000000000000000, 0.8660254037844387076, 1.000000000000000000, 0.8660254037844387076, 1.000000000000000000, 0.8660254037844387076, 1.000000000000000000, 0.8660254037844387076, 1.000000000000000000, 0.8660254037844387076, 1.000000000000000000, 0.8660254037844387076, 1.000000000000000000, 0.8660254037844387076, 1.000000000000000000, 0.8660254037844387076, 1.000000000000000000, 0.8660254037844387076, 1.000000000000000000, 0.8660254037844387076, 1.000000000000000000, 0.8660254037844387076, 1.000000000000000000, 0.8660254037844387076, 1.000000000000000000, 0.8660254037844387076, 1.000000000000000000, 0.8660254037844387076, 1.000000000000000000, 0.8660254037844387076, 1.000000000000000000, 0.8660254037844387076, 1.000000000000000000, 0.8660254037844387076, 1.000000000000000000, 0.8660254037844387076, 1.000000000000000000, 0.8660254037844387076, 1.000000000000000000, 0.8660254037844387076, 1.000000000000000000, 0.8660254037844387076, 1.000000000000000000, 0.8660254037844387076, 1.000000000000000000, 0.8660254037844387076, 1.000000000000000000, 0.8660254037844387076, 1.000000000000000000, 0.8660254037844387076, 1.000000000000000000, 0.8660254037844387076, 1.000000000000000000, 0.8660254037844387076, 1.000000000000000000, 0.8660254037844387076, 1.000000000000000000, 0.8660254037844387076, 1.000000000000000000, 0.8660254037844387076, 1.000000000000000000, 0.8660254037844387076, 1.000000000000000000, 0.8660254037844387076, 1.000000000000000000, 0.8660254037844387076, 1.000000000000000000, 0.8660254037844387076, 1.000000000000000000, 0.8660254037844387076, 1.000000000000000000, 0.8660254037844387076, 1.000000000000000000, 0.8660254037844387076, 1.000000000000000000, 0.8660254037844387076, 1.000000000000000000, 0.8660254037844387076, 1.000000000000000000, 0.8660254037844387076, 1.000000000000000000, 0.8660254037844387076, 1.000000000000000000, 0.8660254037844387076, 1.000000000000000000, 0.8660254037844387076, 1.000000000000000000, 0.8660254037844387076, 1.000000000000000000, 0.8660254037844387076, 1.000000000000000000, 0.8660254037844387076, 1.000000000000000000, 0.8660254037844387076, 1.000000000000000000, 0.8660254037844387076, 1.000000000000000000, 0.8660254037844387076, 1.000000000000000000, 0.8660254037844387076, 1.000000000000000000, 0.8660254037844387076, 1.000000000000000000, 0.8660254037844387076, 1.000000000000000000, 0.8660254037844387076, 1.000000000000000000, 0.8660254037844387076, 1.000000000000000000, 0.8660254037844387076, 1.000000000000000000, 0.8660254037844387076, 1.000000000000000000, 0.8660254037844387076, 1.000000000000000000, 0.8660254037844387076, 1.000000000000000000, 0.8660254037844387076, 1.000000000000000000, 0.8660254037844387076, 1.000000000000000000, 0.8660254037844387076, 1.000000000000000000, 0.8660254037844387076, 1.000000000000000000, 0.8660254037844387076, 1.000000000000000000, 0.8660254037844387076, 1.000000000000000000, 0.8660254037844387076, 1.000000000000000000, 0.8660254037844387076, 1.000000000000000000, 0.8660254037844387076, 1.000000000000000000, 0.8660254037844387076, 1.000000000000000000, 0.8660254037844387076, 1.000000000000000000, 0.8660254037844387076, 1.000000000000000000, 0.8660254037844387076, 1.000000000000000000, 0.8660254037844387076, 1.000000000000000000, 0.8660254037844387076, 1.000000000000000000, 0.8660254037844387076, 1.000000000000000000, 0.8660254037844387076, 1.000000000000000000, 0.8660254037844387076, 1.000000000000000000, 0.8660254037844387076, 1.000000000000000000, 0.8660254037844387076, 1.000000000000000000, 0.8660254037844387076, 1.000000000000000000, 0.8660254037844387076, 1.000000000000000000, 0.8660254037844387076, 1.000000000000000000, 0.8660254037844387076, 1.000000000000000000, 0.8660254037844387076, 1.000000000000000000, 0.8660254037844387076, 1.000000000000000000, 0.8660254037844387076, 1.000000000000000000, 0.8660254037844387076, 1.000000000000000000, 0.8660254037844387076, 1.000000000000000000, 0.8660254037844387076, 1.000000000000000000, 0.8660254037844387076, 1.000000000000000000, 0.8660254037844387076, 1.000000000000000000, 0.8660254037844387076, 1.000000000000000000, 0.8660254037844387076, 1.000000000000000000, 0.8660254037844387076, 1.000000000000000000, 0.8660254037844387076, 1.000000000000000000, 0.8660254037844387076, 1.000000000000000000, 0.8660254037844387076, 1.000000000000000000, 0.8660254037844387076, 1.000000000000000000, 0.8660254037844387076, 1.000000000000000000, 0.8660254037844387076, 1.000000000000000000, 0.8660254037844387076, 1.000000000000000000, 0.8660254037844387076, 1.000000000000000000, 0.8660254037844387076, 1.000000000000000000, 0.8660254037844387076, 1.000000000000000000, 0.8660254037844387076, 1.000000000000000000, 0.8660254037844387076, 1.000000000000000000, 0.8660254037844387076, 1.000000000000000000, 0.8660254037844387076, 1.000000000000000000, 0.8660254037844387076, 1.000000000000000000, 0.8660254037844387076, 1.000000000000000000, 0.8660254037844387076, 1.000000000000000000, 0.8660254037844387076, 1.000000000000000000, 0.8660254037844387076, 1.000000000000000000, 0.8660254037844387076, 1.000000000000000000, 0.8660254037844387076, 1.000000000000000000, 0.8660254037844387076, 1.000000000000000000, 0.8660254037844387076, 1.000000000000000000, 0.8660254037844387076, 1.000000000000000000, 0.8660254037844387076, 1.000000000000000000, 0.8660254037844387076, 1.000000000000000000, 0.8660254037844387076, 1.000000000000000000, 0.8660254037844387076, 1.000000000000000000, 0.8660254037844387076, 1.000000000000000000, 0.8660254037844387076, 1.000000000000000000, 0.8660254037844387076, 1.000000000000000000, 0.8660254037844387076, 1.000000000000000000, 0.8660254037844387076, 1.000000000000000000, 0.8660254037844387076, 1.000000000000000000, 0.8660254037844387076, 1.000000000000000000, 0.8660254037844387076, 1.000000000000000000, 0.8660254037844387076, 1.000000000000000000, 0.8660254037844387076, 1.000000000000000000, 0.8660254037844387076, 1.000000000000000000, 0.8660254037844387076, 1.000000000000000000, 0.8660254037844387076, 1.000000000000000000, 0.8660254037844387076, 1.000000000000000000, 0.8660254037844387076, 1.000000000000000000, 0.8660254037844387076, 1.000000000000000000, 0.8660254037844387076, 1.000000000000000000, 0.8660254037844387076, 1.000000000000000000, 0.8660254037844387076, 1.000000000000000000, 0.8660254037844387076, 1.000000000000000000, 0.8660254037844387076, 1.000000000000000000, 0.8660254037844387076, 1.000000000000000000, 0.8660254037844387076, 1.000000000000000000, 0.8660254037844387076, 1.000000000000000000, 0.8660254037844387076, 1.000000000000000000, 0.8660254037844387076, 1.000000000000000000, 0.8660254037844387076, 1.000000000000000000, 0.8660254037844387076, 1.000000000000000000, 0.8660254037844387076, 1.000000000000000000, 0.8660254037844387076, 1.000000000000000000, 0.8660254037844387076, 1.000000000000000000, 0.8660254037844387076, 1.000000000000000000, 0.8660254037844387076, 1.000000000000000000, 0.8660254037844387076, 1.000000000000000000, 0.8660254037844387076, 1.000000000000000000, 0.8660254037844387076, 1.000000000000000000, 0.8660254037844387076, 1.000000000000000000, 0.8660254037844387076, 1.000000000000000000, 0.8660254037844387076, 1.000000000000000000, 0.8660254037844387076, 1.000000000000000000, 0.8660254037844387076, 1.000000000000000000, 0.8660254037844387076, 1.000000000000000000, 0.8660254037844387076, 1.000000000000000000, 0.8660254037844387076, 1.000000000000000000, 0.8660254037844387076, 1.000000000000000000, 0.8660254037844387076, 1.000000000000000000, 0.8660254037844387076, 1.000000000000000000, 0.8660254037844387076, 1.000000000000000000, 0.8660254037844387076, 1.000000000000000000, 0.8660254037844387076, 1.000000000000000000, 0.8660254037844387076, 1.000000000000000000, 0.8660254037844387076, 1.000000000000000000, 0.8660254037844387076, 1.000000000000000000, 0.8660254037844387076, 1.000000000000000000, 0.8660254037844387076, 1.000000000000000000, 0.8660254037844387076, 1.000000000000000000, 0.8660254037844387076, 1.000000000000000000, 0.8660254037844387076, 1.000000000000000000, 0.8660254037844387076, 1.000000000000000000, 0.8660254037844387076, 1.000000000000000000, 0.8660254037844387076, 1.000000000000000000, 0.8660254037844387076, 1.000000000000000000, 0.8660254037844387076, 1.000000000000000000, 0.8660254037844387076, 1.000000000000000000, 0.8660254037844387076, 1.000000000000000000, 0.8660254037844387076, 1.000000000000000000, 0.8660254037844387076, 1.000000000000000000, 0.8660254037844387076, 1.000000000000000000, 0.8660254037844387076, 1.000000000000000000, 0.8660254037844387076, 1.000000000000000000, 0.8660254037844387076, 1.000000000000000000, 0.8660254037844387076, 1.000000000000000000, 0.8660254037844387076, 1.000000000000000000, 0.8660254037844387076, 1.000000000000000000, 0.8660254037844387076, 1.000000000000000000, 0.8660254037844387076, 1.000000000000000000, 0.8660254037844387076, 1.000000000000000000, 0.8660254037844387076, 1.000000000000000000, 0.8660254037844387076, 1.000000000000000000, 0.8660254037844387076, 1.000000000000000000, 0.8660254037844387076, 1.000000000000000000, 0.8660254037844387076, 1.000000000000000000, 0.8660254037844387076, 1.000000000000000000, 0.8660254037844387076, 1.000000000000000000, 0.8660254037844387076, 1.000000000000000000, 0.8660254037844387076, 1.000000000000000000, 0.8660254037844387076, 1.000000000000000000, 0.8660254037844387076, 1.000000000000000000, 0.8660254037844387076, 1.000000000000000000, 0.8660254037844387076, 1.000000000000000000, 0.8660254037844387076, 1.000000000000000000, 0.8660254037844387076, 1.000000000000000000, 0.8660254037844387076, 1.000000000000000000, 0.8660254037844387076, 1.000000000000000000, 0.8660254037844387076, 1.000000000000000000, 0.8660254037844387076, 1.000000000000000000, 0.8660254037844387076, 1.000000000000000000, 0.8660254037844387076, 1.000000000000000000, 0.8660254037844387076, 1.000000000000000000, 0.8660254037844387076, 1.000000000000000000, 0.8660254037844387076, 1.000000000000000000, 0.8660254037844387076, 1.000000000000000000, 0.8660254037844387076, 1.000000000000000000, 0.8660254037844387076, 1.000000000000000000, 0.8660254037844387076, 1.000000000000000000, 0.8660254037844387076, 1.000000000000000000, 0.8660254037844387076, 1.000000000000000000, 0.8660254037844387076, 1.000000000000000000, 0.8660254037844387076, 1.000000000000000000, 0.8660254037844387076, 1.000000000000000000, 0.8660254037844387076, 1.000000000000000000, 0.8660254037844387076, 1.000000000000000000, 0.8660254037844387076, 1.000000000000000000, 0.8660254037844387076, 1.000000000000000000, 0.8660254037844387076, 1.000000000000000000, 0.8660254037844387076, 1.000000000000000000, 0.8660254037844387076, 1.000000000000000000, 0.8660254037844387076, 1.000000000000000000, 0.8660254037844387076, 1.000000000000000000, 0.8660254037844387076, 1.000000000000000000, 0.8660254037844387076, 1.000000000000000000, 0.8660254037844387076, 1.000000000000000000, 0.8660254037844387076, 1.000000000000000000, 0.8660254037844387076, 1.000000000000000000, 0.8660254037844387076, 1.000000000000000000, 0.8660254037844387076, 1.000000000000000000, 0.8660254037844387076, 1.000000000000000000, 0.8660254037844387076, 1.000000000000000000, 0.8660254037844387076, 1.000000000000000000, 0.8660254037844387076, 1.000000000000000000, 0.8660254037844387076, 1.000000000000000000, 0.8660254037844387076, 1.000000000000000000, 0.8660254037844387076, 1.000000000000000000, 0.8660254037844387076, 1.000000000000000000, 0.8660254037844387076, 1.000000000000000000, 0.8660254037844387076, 1.000000000000000000, 0.8660254037844387076, 1.000000000000000000, 0.8660254037844387076, 1.000000000000000000, 0.8660254037844387076, 1.000000000000000000, 0.8660254037844387076, 1.000000000000000000, 0.8660254037844387076, 1.000000000000000000, 0.8660254037844387076, 1.000000000000000000, 0.8660254037844387076, 1.000000000000000000, 0.8660254037844387076, 1.000000000000000000, 0.8660254037844387076, 1.000000000000000000, 0.8660254037844387076, 1.000000000000000000, 0.8660254037844387076, 1.000000000000000000, 0.8660254037844387076, 1.000000000000000000, 0.8660254037844387076, 1.000000000000000000, 0.8660254037844387076, 1.000000000000000000, 0.8660254037844387076, 1.000000000000000000, 0.8660254037844387076, 1.000000000000000000, 0.8660254037844387076, 1.000000000000000000, 0.8660254037844387076, 1.000000000000000000, 0.8660254037844387076, 1.000000000000000000, 0.8660254037844387076, 1.000000000000000000, 0.8660254037844387076, 1.000000000000000000, 0.8660254037844387076, 1.000000000000000000, 0.8660254037844387076, 1.000000000000000000, 0.8660254037844387076, 1.000000000000000000, 0.8660254037844387076, 1.000000000000000000, 0.8660254037844387076, 1.000000000000000000, 0.8660254037844387076, 1.000000000000000000, 0.8660254037844387076, 1.000000000000000000, 0.8660254037844387076, 1.000000000000000000, 0.8660254037844387076, 1.000000000000000000, 0.8660254037844387076, 1.000000000000000000, 0.8660254037844387076, 1.000000000000000000, 0.8660254037844387076, 1.000000000000000000, 0.8660254037844387076, 1.000000000000000000, 0.8660254037844387076, 1.000000000000000000, 0.8660254037844387076, 1.000000000000000000, 0.8660254037844387076, 1.000000000000000000, 0.8660254037844387076, 1.000000000000000000, 0.8660254037844387076, 1.000000000000000000, 0.8660254037844387076, 1.000000000000000000, 0.8660254037844387076, 1.000000000000000000, 0.8660254037844387076, 1.000000000000000000, 0.8660254037844387076, 1.000000000000000000, 0.8660254037844387076, 1.000000000000000000, 0.8660254037844387076, 1.000000000000000000, 0.8660254037844387076, 1.000000000000000000, 0.8660254037844387076, 1.000000000000000000, 0.8660254037844387076, 1.000000000000000000, 0.8660254037844387076, 1.000000000000000000, 0.8660254037844387076, 1.000000000000000000, 0.8660254037844387076, 1.000000000000000000, 0.8660254037844387076, 1.000000000000000000, 0.8660254037844387076, 1.000000000000000000, 0.8660254037844387076, 1.000000000000000000, 0.8660254037844387076, 1.000000000000000000, 0.8660254037844387076, 1.000000000000000000, 0.8660254037844387076, 1.000000000000000000, 0.8660254037844387076, 1.000000000000000000, 0.8660254037844387076, 1.000000000000000000, 0.8660254037844387076, 1.000000000000000000, 0.8660254037844387076, 1.000000000000000000, 0.8660254037844387076, 1.000000000000000000, 0.8660254037844387076, 1.000000000000000000, 0.8660254037844387076, 1.000000000000000000, 0.8660254037844387076, 1.000000000000000000, 0.8660254037844387076, 1.000000000000000000, 0.8660254037844387076, 1.000000000000000000, 0.8660254037844387076, 1.000000000000000000, 0.8660254037844387076, 1.000000000000000000, 0.8660254037844387076, 1.000000000000000000, 0.8660254037844387076, 1.000000000000000000, 0.8660254037844387076, 1.000000000000000000, 0.8660254037844387076, 1.000000000000000000, 0.8660254037844387076, 1.000000000000000000, 0.8660254037844387076, 1.000000000000000000, 0.8660254037844387076, 1.000000000000000000, 0.8660254037844387076, 1.000000000000000000, 0.8660254037844387076, 1.000000000000000000, 0.8660254037844387076, 1.000000000000000000, 0.8660254037844387076, 1.000000000000000000, 0.8660254037844387076, 1.000000000000000000, 0.8660254037844387076, 1.000000000000000000, 0.8660254037844387076, 1.000000000000000000, 0.8660254037844387076, 1.000000000000000000, 0.8660254037844387076, 1.000000000000000000, 0.8660254037844387076, 1.000000000000000000, 0.8660254037844387076, 1.000000000000000000, 0.8660254037844387076, 1.000000000000000000, 0.8660254037844387076, 1.000000000000000000, 0.8660254037844387076, 1.000000000000000000, 0.8660254037844387076, 1.000000000000000000, 0.8660254037844387076, 1.000000000000000000, 0.8660254037844387076, 1.000000000000000000, 0.8660254037844387076, 1.000000000000000000, 0.8660254037844387076, 1.000000000000000000, 0.8660254037844387076, 1.000000000000000000, 0.8660254037844387076, 1.000000000000000000, 0.8660254037844387076, 1.000000000000000000, 0.8660254037844387076, 1.000000000000000000, 0.8660254037844387076, 1.000000000000000000, 0.8660254037844387076, 1.000000000000000000, 0.8660254037844387076, 1.000000000000000000, 0.8660254037844387076, 1.000000000000000000, 0.8660254037844387076, 1.000000000000000000, 0.8660254037844387076, 1.000000000000000000, 0.8660254037844387076, 1.000000000000000000, 0.8660254037844387076, 1.000000000000000000, 0.8660254037844387076, 1.000000000000000000, 0.8660254037844387076, 1.000000000000000000, 0.8660254037844387076, 1.000000000000000000, 0.8660254037844387076, 1.000000000000000000, 0.8660254037844387076, 1.000000000000000000, 0.8660254037844387076, 1.000000000000000000, 0.8660254037844387076, 1.000000000000000000, 0.8660254037844387076, 1.000000000000000000, 0.8660254037844387076, 1.000000000000000000, 0.8660254037844387076, 1.000000000000000000, 0.8660254037844387076, 1.000000000000000000, 0.8660254037844387076, 1.000000000000000000, 0.8660254037844387076, 1.000000000000000000, 0.8660254037844387076, 1.000000000000000000, 0.8660254037844387076, 1.000000000000000000, 0.8660254037844387076, 1.000000000000000000, 0.8660254037844387076, 1.000000000000000000, 0.8660254037844387076, 1.000000000000000000, 0.8660254037844387076, 1.000000000000000000, 0.8660254037844387076, 1.000000000000000000, 0.8660254037844387076, 1.000000000000000000, 0.8660254037844387076, 1.000000000000000000, 0.8660254037844387076, 1.000000000000000000, 0.8660254037844387076, 1.000000000000000000, 0.8660254037844387076, 1.000000000000000000, 0.8660254037844387076, 1.000000000000000000, 0.8660254037844387076, 1.000000000000000000, 0.8660254037844387076, 1.000000000000000000, 0.8660254037844387076, 1.000000000000000000, 0.8660254037844387076, 1.000000000000000000, 0.8660254037844387076, 1.000000000000000000, 0.8660254037844387076, 1.000000000000000000, 0.8660254037844387076, 1.000000000000000000, 0.8660254037844387076, 1.000000000000000000, 0.8660254037844387076, 1.000000000000000000, 0.8660254037844387076, 1.000000000000000000, 0.8660254037844387076, 1.000000000000000000, 0.8660254037844387076, 1.000000000000000000, 0.8660254037844387076, 1.000000000000000000, 0.8660254037844387076, 1.000000000000000000, 0.8660254037844387076, 1.000000000000000000, 0.8660254037844387076, 1.000000000000000000, 0.8660254037844387076, 1.000000000000000000, 0.8660254037844387076, 1.000000000000000000, 0.8660254037844387076, 1.000000000000000000, 0.8660254037844387076, 1.000000000000000000, 0.8660254037844387076, 1.000000000000000000, 0.8660254037844387076, 1.000000000000000000, 0.8660254037844387076, 1.000000000000000000, 0.8660254037844387076, 1.000000000000000000, 0.8660254037844387076, 1.000000000000000000, 0.8660254037844387076, 1.000000000000000000, 0.8660254037844387076, 1.000000000000000000, 0.8660254037844387076, 1.000000000000000000, 0.8660254037844387076, 1.000000000000000000, 0.8660254037844387076, 1.000000000000000000, 0.8660254037844387076, 1.000000000000000000, 0.8660254037844387076, 1.000000000000000000, 0.8660254037844387076, 1.000000000000000000, 0.8660254037844387076, 1.000000000000000000, 0.8660254037844387076, 1.000000000000000000, 0.8660254037844387076, 1.000000000000000000, 0.8660254037844387076, 1.000000000000000000, 0.8660254037844387076, 1.000000000000000000, 0.8660254037844387076, 1.000000000000000000, 0.8660254037844387076, 1.000000000000000000, 0.8660254037844387076, 1.000000000000000000, 0.8660254037844387076, 1.000000000000000000, 0.8660254037844387076, 1.000000000000000000, 0.8660254037844387076, 1.000000000000000000, 0.8660254037844387076, 1.000000000000000000, 0.8660254037844387076, 1.000000000000000000, 0.8660254037844387076, 1.000000000000000000, 0.8660254037844387076, 1.000000000000000000, 0.8660254037844387076, 1.000000000000000000, 0.8660254037844387076, 1.000000000000000000, 0.8660254037844387076, 1.000000000000000000, 0.8660254037844387076, 1.000000000000000000, 0.8660254037844387076, 1.000000000000000000, 0.8660254037844387076, 1.000000000000000000, 0.8660254037844387076, 1.000000000000000000, 0.8660254037844387076, 1.000000000000000000, 0.8660254037844387076, 1.000000000000000000, 0.8660254037844387076, 1.000000000000000000, 0.8660254037844387076, 1.000000000000000000, 0.8660254037844387076, 1.000000000000000000, 0.8660254037844387076, 1.000000000000000000, 0.8660254037844387076, 1.000000000000000000, 0.8660254037844387076, 1.000000000000000000, 0.8660254037844387076, 1.000000000000000000, 0.8660254037844387076, 1.000000000000000000, 0.8660254037844387076, 1.000000000000000000, 0.8660254037844387076, 1.000000000000000000, 0.8660254037844387076, 1.000000000000000000, 0.8660254037844387076, 1.000000000000000000, 0.8660254037844387076, 1.000000000000000000, 0.8660254037844387076, 1.000000000000000000, 0.8660254037844387076, 1.000000000000000000, 0.8660254037844387076, 1.000000000000000000, 0.8660254037844387076, 1.000000000000000000, 0.8660254037844387076, 1.000000000000000000, 0.8660254037844387076, 1.000000000000000000, 0.8660254037844387076, 1.000000000000000000, 0.8660254037844387076, 1.000000000000000000, 0.8660254037844387076, 1.000000000000000000, 0.8660254037844387076, 1.000000000000000000, 0.8660254037844387076, 1.000000000000000000, 0.8660254037844387076, 1.000000000000000000, 0.8660254037844387076, 1.000000000000000000, 0.8660254037844387076, 1.000000000000000000, 0.8660254037844387076, 1.000000000000000000, 0.8660254037844387076, 1.000000000000000000, 0.8660254037844387076, 1.000000000000000000, 0.8660254037844387076, 1.000000000000000000, 0.8660254037844387076, 1.000000000000000000, 0.8660254037844387076, 1.000000000000000000, 0.8660254037844387076, 1.000000000000000000, 0.8660254037844387076, 1.000000000000000000, 0.8660254037844387076, 1.000000000000000000, 0.8660254037844387076, 1.000000000000000000, 0.8660254037844387076, 1.000000000000000000, 0.8660254037844387076, 1.000000000000000000, 0.8660254037844387076, 1.000000000000000000, 0.8660254037844387076, 1.000000000000000000, 0.8660254037844387076, 1.000000000000000000, 0.8660254037844387076, 1.000000000000000000, 0.8660254037844387076, 1.000000000000000000, 0.8660254037844387076, 1.000000000000000000, 0.8660254037844387076, 1.000000000000000000, 0.8660254037844387076, 1.000000000000000000, 0.8660254037844387076, 1.000000000000000000, 0.8660254037844387076, 1.000000000000000000, 0.8660254037844387076, 1.000000000000000000, 0.8660254037844387076, 1.000000000000000000, 0.8660254037844387076, 1.000000000000000000, 0.8660254037844387076, 1.000000000000000000, 0.8660254037844387076, 1.000000000000000000, 0.8660254037844387076, 1.000000000000000000, 0.8660254037844387076, 1.000000000000000000, 0.8660254037844387076, 1.000000000000000000, 0.8660254037844387076, 1.000000000000000000, 0.8660254037844387076, 1.000000000000000000, 0.8660254037844387076, 1.000000000000000000, 0.8660254037844387076, 1.000000000000000000, 0.8660254037844387076, 1.000000000000000000, 0.8660254037844387076, 1.000000000000000000, 0.8660254037844387076, 1.000000000000000000, 0.8660254037844387076, 1.000000000000000000, 0.8660254037844387076, 1.000000000000000000, 0.8660254037844387076, 1.000000000000000000, 0.8660254037844387076, 1.000000000000000000, 0.8660254037844387076, 1.000000000000000000, 0.8660254037844387076, 1.000000000000000000, 0.8660254037844387076, 1.000000000000000000, 0.8660254037844387076, 1.000000000000000000, 0.8660254037844387076, 1.000000000000000000, 0.8660254037844387076, 1.000000000000000000, 0.8660254037844387076, 1.000000000000000000, 0.8660254037844387076, 1.000000000000000000, 0.8660254037844387076, 1.000000000000000000, 0.8660254037844387076, 1.000000000000000000, 0.8660254037844387076, 1.000000000000000000, 0.8660254037844387076, 1.000000000000000000, 0.8660254037844387076, 1.000000000000000000, 0.8660254037844387076, 1.000000000000000000, 0.8660254037844387076, 1.000000000000000000, 0.8660254037844387076, 1.000000000000000000, 0.8660254037844387076, 1.000000000000000000, 0.8660254037844387076, 1.000000000000000000, 0.8660254037844387076, 1.000000000000000000, 0.8660254037844387076, 1.000000000000000000, 0.8660254037844387076, 1.000000000000000000, 0.8660254037844387076, 1.000000000000000000, 0.8660254037844387076, 1.000000000000000000, 0.8660254037844387076, 1.000000000000000000, 0.8660254037844387076, 1.000000000000000000, 0.8660254037844387076, 1.000000000000000000, 0.8660254037844387076, 1.000000000000000000, 0.8660254037844387076, 1.000000000000000000, 0.8660254037844387076, 1.000000000000000000, 0.8660254037844387076, 1.000000000000000000, 0.8660254037844387076, 1.000000000000000000, 0.8660254037844387076, 1.000000000000000000, 0.8660254037844387076, 1.000000000000000000, 0.8660254037844387076, 1.000000000000000000, 0.8660254037844387076, 1.000000000000000000, 0.8660254037844387076, 1.000000000000000000, 0.8660254037844387076, 1.000000000000000000, 0.8660254037844387076, 1.000000000000000000, 0.8660254037844387076, 1.000000000000000000, 0.8660254037844387076, 1.000000000000000000, 0.8660254037844387076, 1.000000000000000000, 0.8660254037844387076, 1.000000000000000000, 0.8660254037844387076, 1.000000000000000000, 0.8660254037844387076, 1.000000000000000000, 0.8660254037844387076, 1.000000000000000000, 0.8660254037844387076, 1.000000000000000000, 0.8660254037844387076, 1.000000000000000000, 0.8660254037844387076, 1.000000000000000000, 0.8660254037844387076, 1.000000000000000000, 0.8660254037844387076, 1.000000000000000000, 0.8660254037844387076, 1.000000000000000000, 0.8660254037844387076, 1.000000000000000000, 0.8660254037844387076, 1.000000000000000000, 0.8660254037844387076, 1.000000000000000000, 0.8660254037844387076, 1.000000000000000000, 0.8660254037844387076, 1.000000000000000000, 0.8660254037844387076, 1.000000000000000000, 0.8660254037844387076, 1.000000000000000000, 0.8660254037844387076, 1.000000000000000000, 0.8660254037844387076, 1.000000000000000000, 0.8660254037844387076, 1.000000000000000000, 0.8660254037844387076, 1.000000000000000000, 0.8660254037844387076, 1.000000000000000000, 0.8660254037844387076, 1.000000000000000000, 0.8660254037844387076, 1.000000000000000000, 0.8660254037844387076, 1.000000000000000000, 0.8660254037844387076, 1.000000000000000000, 0.8660254037844387076, 1.000000000000000000, 0.8660254037844387076, 1.000000000000000000, 0.8660254037844387076, 1.000000000000000000, 0.8660254037844387076, 1.000000000000000000, 0.8660254037844387076, 1.000000000000000000, 0.8660254037844387076, 1.000000000000000000, 0.8660254037844387076, 1.000000000000000000, 0.8660254037844387076, 1.000000000000000000, 0.8660254037844387076, 1.000000000000000000, 0.8660254037844387076, 1.000000000000000000, 0.8660254037844387076, 1.000000000000000000, 0.8660254037844387076, 1.000000000000000000, 0.8660254037844387076, 1.000000000000000000, 0.8660254037844387076, 1.000000000000000000, 0.8660254037844387076, 1.000000000000000000, 0.8660254037844387076, 1.000000000000000000, 0.8660254037844387076, 1.000000000000000000, 0.8660254037844387076, 1.000000000000000000, 0.8660254037844387076, 1.000000000000000000, 0.8660254037844387076, 1.000000000000000000, 0.8660254037844387076, 1.000000000000000000, 0.8660254037844387076, 1.000000000000000000, 0.8660254037844387076, 1.000000000000000000, 0.8660254037844387076, 1.000000000000000000, 0.8660254037844387076, 1.000000000000000000, 0.8660254037844387076, 1.000000000000000000, 0.8660254037844387076, 1.000000000000000000, 0.8660254037844387076, 1.000000000000000000, 0.8660254037844387076, 1.000000000000000000, 0.8660254037844387076, 1.000000000000000000, 0.8660254037844387076, 1.000000000000000000, 0.8660254037844387076, 1.000000000000000000, 0.8660254037844387076, 1.000000000000000000, 0.8660254037844387076, 1.000000000000000000, 0.8660254037844387076, 1.000000000000000000, 0.8660254037844387076, 1.000000000000000000, 0.8660254037844387076, 1.000000000000000000, 0.8660254037844387076, 1.000000000000000000, 0.8660254037844387076, 1.000000000000000000, 0.8660254037844387076, 1.000000000000000000, 0.8660254037844387076, 1.000000000000000000, 0.8660254037844387076, 1.000000000000000000, 0.8660254037844387076, 1.000000000000000000, 0.8660254037844387076, 1.000000000000000000, 0.8660254037844387076, 1.000000000000000000, 0.8660254037844387076, 1.000000000000000000, 0.8660254037844387076, 1.000000000000000000, 0.8660254037844387076, 1.000000000000000000, 0.8660254037844387076, 1.000000000000000000, 0.8660254037844387076, 1.000000000000000000, 0.8660254037844387076, 1.000000000000000000, 0.8660254037844387076, 1.000000000000000000, 0.8660254037844387076, 1.000000000000000000, 0.8660254037844387076, 1.000000000000000000, 0.8660254037844387076, 1.000000000000000000, 0.8660254037844387076, 1.000000000000000000, 0.8660254037844387076, 1.000000000000000000, 0.8660254037844387076, 1.000000000000000000, 0.8660254037844387076, 1.000000000000000000, 0.8660254037844387076, 1.000000000000000000, 0.8660254037844387076, 1.000000000000000000, 0.8660254037844387076, 1.000000000000000000, 0.8660254037844387076, 1.000000000000000000, 0.8660254037844387076, 1.000000000000000000, 0.8660254037844387076, 1.000000000000000000, 0.8660254037844387076, 1.000000000000000000, 0.8660254037844387076, 1.000000000000000000, 0.8660254037844387076, 1.000000000000000000, 0.8660254037844387076, 1.000000000000000000, 0.8660254037844387076, 1.000000000000000000, 0.8660254037844387076, 1.000000000000000000, 0.8660254037844387076, 1.000000000000000000, 0.8660254037844387076, 1.000000000000000000, 0.8660254037844387076, 1.000000000000000000, 0.8660254037844387076, 1.000000000000000000, 0.8660254037844387076, 1.000000000000000000, 0.8660254037844387076, 1.000000000000000000, 0.8660254037844387076, 1.000000000000000000, 0.8660254037844387076, 1.000000000000000000, 0.8660254037844387076, 1.000000000000000000, 0.8660254037844387076, 1.000000000000000000, 0.8660254037844387076, 1.000000000000000000, 0.8660254037844387076, 1.000000000000000000, 0.8660254037844387076, 1.000000000000000000, 0.8660254037844387076, 1.000000000000000000, 0.8660254037844387076, 1.000000000000000000, 0.8660254037844387076, 1.000000000000000000, 0.8660254037844387076, 1.000000000000000000, 0.8660254037844387076, 1.000000000000000000, 0.8660254037844387076, 1.000000000000000000, 0.8660254037844387076, 1.000000000000000000, 0.8660254037844387076, 1.000000000000000000, 0.8660254037844387076, 1.000000000000000000, 0.8660254037844387076, 1.000000000000000000, 0.8660254037844387076, 1.000000000000000000, 0.8660254037844387076, 1.000000000000000000, 0.8660254037844387076, 1.000000000000000000, 0.8660254037844387076, 1.000000000000000000, 0.8660254037844387076, 1.000000000000000000, 0.8660254037844387076, 1.000000000000000000, 0.8660254037844387076, 1.000000000000000000, 0.8660254037844387076, 1.000000000000000000, 0.8660254037844387076, 1.000000000000000000, 0.8660254037844387076, 1.000000000000000000, 0.8660254037844387076, 1.000000000000000000, 0.8660254037844387076, 1.000000000000000000, 0.8660254037844387076, 1.000000000000000000, 0.8660254037844387076, 1.000000000000000000, 0.8660254037844387076, 1.000000000000000000, 0.8660254037844387076, 1.000000000000000000, 0.8660254037844387076, 1.000000000000000000, 0.8660254037844387076, 1.000000000000000000, 0.8660254037844387076, 1.000000000000000000, 0.8660254037844387076, 1.000000000000000000, 0.8660254037844387076, 1.000000000000000000, 0.8660254037844387076, 1.000000000000000000, 0.8660254037844387076, 1.000000000000000000, 0.8660254037844387076, 1.000000000000000000, 0.8660254037844387076, 1.000000000000000000, 0.8660254037844387076, 1.000000000000000000, 0.8660254037844387076, 1.000000000000000000, 0.8660254037844387076, 1.000000000000000000, 0.8660254037844387076, 1.000000000000000000, 0.8660254037844387076, 1.000000000000000000, 0.8660254037844387076, 1.000000000000000000, 0.8660254037844387076, 1.000000000000000000, 0.8660254037844387076, 1.000000000000000000, 0.8660254037844387076, 1.000000000000000000, 0.8660254037844387076, 1.000000000000000000, 0.8660254037844387076, 1.000000000000000000, 0.8660254037844387076, 1.000000000000000000, 0.8660254037844387076, 1.000000000000000000, 0.8660254037844387076, 1.000000000000000000, 0.8660254037844387076, 1.000000000000000000, 0.8660254037844387076, 1.000000000000000000, 0.8660254037844387076, 1.000000000000000000, 0.8660254037844387076, 1.000000000000000000, 0.8660254037844387076, 1.000000000000000000, 0.8660254037844387076, 1.000000000000000000, 0.8660254037844387076, 1.000000000000000000, 0.8660254037844387076, 1.000000000000000000, 0.8660254037844387076, 1.000000000000000000, 0.8660254037844387076, 1.000000000000000000, 0.8660254037844387076, 1.000000000000000000, 0.8660254037844387076, 1.000000000000000000, 0.8660254037844387076, 1.000000000000000000, 0.8660254037844387076, 1.000000000000000000, 0.8660254037844387076, 1.000000000000000000, 0.8660254037844387076, 1.000000000000000000, 0.8660254037844387076, 1.000000000000000000, 0.8660254037844387076, 1.000000000000000000, 0.8660254037844387076, 1.000000000000000000, 0.8660254037844387076, 1.000000000000000000, 0.8660254037844387076, 1.000000000000000000, 0.8660254037844387076, 1.000000000000000000, 0.8660254037844387076, 1.000000000000000000, 0.8660254037844387076, 1.000000000000000000, 0.8660254037844387076, 1.000000000000000000, 0.8660254037844387076, 1.000000000000000000, 0.8660254037844387076, 1.000000000000000000, 0.8660254037844387076, 1.000000000000000000, 0.8660254037844387076, 1.000000000000000000, 0.8660254037844387076, 1.000000000000000000, 0.8660254037844387076, 1.000000000000000000, 0.8660254037844387076, 1.000000000000000000, 0.8660254037844387076, 1.000000000000000000, 0.8660254037844387076, 1.000000000000000000, 0.8660254037844387076, 1.000000000000000000, 0.8660254037844387076, 1.000000000000000000, 0.8660254037844387076, 1.000000000000000000, 0.8660254037844387076, 1.000000000000000000, 0.8660254037844387076, 1.000000000000000000, 0.8660254037844387076, 1.000000000000000000, 0.8660254037844387076, 1.000000000000000000, 0.8660254037844387076, 1.000000000000000000, 0.8660254037844387076, 1.000000000000000000, 0.8660254037844387076, 1.000000000000000000, 0.8660254037844387076, 1.000000000000000000, 0.8660254037844387076, 1.000000000000000000, 0.8660254037844387076, 1.000000000000000000, 0.8660254037844387076, 1.000000000000000000, 0.8660254037844387076, 1.000000000000000000, 0.8660254037844387076, 1.000000000000000000, 0.8660254037844387076, 1.000000000000000000, 0.8660254037844387076, 1.000000000000000000, 0.8660254037844387076, 1.000000000000000000, 0.8660254037844387076, 1.000000000000000000, 0.8660254037844387076, 1.000000000000000000, 0.8660254037844387076, 1.000000000000000000, 0.8660254037844387076, 1.000000000000000000, 0.8660254037844387076, 1.000000000000000000, 0.8660254037844387076, 1.000000000000000000, 0.8660254037844387076, 1.000000000000000000, 0.8660254037844387076, 1.000000000000000000, 0.8660254037844387076, 1.000000000000000000, 0.8660254037844387076, 1.000000000000000000, 0.8660254037844387076, 1.000000000000000000, 0.8660254037844387076, 1.000000000000000000, 0.8660254037844387076, 1.000000000000000000, 0.8660254037844387076, 1.000000000000000000, 0.8660254037844387076, 1.000000000000000000, 0.8660254037844387076, 1.000000000000000000, 0.8660254037844387076, 1.000000000000000000, 0.8660254037844387076, 1.000000000000000000, 0.8660254037844387076, 1.000000000000000000, 0.8660254037844387076, 1.000000000000000000, 0.8660254037844387076, 1.000000000000000000, 0.8660254037844387076, 1.000000000000000000, 0.8660254037844387076, 1.000000000000000000, 0.8660254037844387076, 1.000000000000000000, 0.8660254037844387076, 1.000000000000000000, 0.8660254037844387076, 1.000000000000000000, 0.8660254037844387076, 1.000000000000000000, 0.8660254037844387076, 1.000000000000000000, 0.8660254037844387076, 1.000000000000000000, 0.8660254037844387076, 1.000000000000000000, 0.8660254037844387076, 1.000000000000000000),
 ( 1.000000000000000000, 0.8660254037844387076, 1.000000000000000000, 0.8660254037844387076, 1.000000000000000000, 0.8660254037844387076, 1.000000000000000000, 0.8660254037844387076, 1.000000000000000000, 0.8660254037844387076, 1.000000000000000000, 0.8660254037844387076, 1.000000000000000000, 0.8660254037844387076, 1.000000000000000000, 0.8660254037844387076, 1.000000000000000000, 0.8660254037844387076, 1.000000000000000000, 0.8660254037844387076, 1.000000000000000000, 0.8660254037844387076, 1.000000000000000000, 0.8660254037844387076, 1.000000000000000000, 0.8660254037844387076, 1.000000000000000000, 0.8660254037844387076, 1.000000000000000000, 0.8660254037844387076, 1.000000000000000000, 0.8660254037844387076, 1.000000000000000000, 0.8660254037844387076, 1.000000000000000000, 0.8660254037844387076, 1.000000000000000000, 0.8660254037844387076, 1.000000000000000000, 0.8660254037844387076, 1.000000000000000000, 0.8660254037844387076, 1.000000000000000000, 0.8660254037844387076, 1.000000000000000000, 0.8660254037844387076, 1.000000000000000000, 0.8660254037844387076, 1.000000000000000000, 0.8660254037844387076, 1.000000000000000000, 0.8660254037844387076, 1.000000000000000000, 0.8660254037844387076, 1.000000000000000000, 0.8660254037844387076, 1.000000000000000000, 0.8660254037844387076, 1.000000000000000000, 0.8660254037844387076, 1.000000000000000000, 0.8660254037844387076, 1.000000000000000000, 0.8660254037844387076, 1.000000000000000000, 0.8660254037844387076, 1.000000000000000000, 0.8660254037844387076, 1.000000000000000000, 0.8660254037844387076, 1.000000000000000000, 0.8660254037844387076, 1.000000000000000000, 0.8660254037844387076, 1.000000000000000000, 0.8660254037844387076, 1.000000000000000000, 0.8660254037844387076, 1.000000000000000000, 0.8660254037844387076, 1.000000000000000000, 0.8660254037844387076, 1.000000000000000000, 0.8660254037844387076, 1.000000000000000000, 0.8660254037844387076, 1.000000000000000000, 0.8660254037844387076, 1.000000000000000000, 0.8660254037844387076, 1.000000000000000000, 0.8660254037844387076, 1.000000000000000000, 0.8660254037844387076, 1.000000000000000000, 0.8660254037844387076, 1.000000000000000000, 0.8660254037844387076, 1.000000000000000000, 0.8660254037844387076, 1.000000000000000000, 0.8660254037844387076, 1.000000000000000000, 0.8660254037844387076, 1.000000000000000000, 0.8660254037844387076, 1.000000000000000000, 0.8660254037844387076, 1.000000000000000000, 0.8660254037844387076, 1.000000000000000000, 0.8660254037844387076, 1.000000000000000000, 0.8660254037844387076, 1.000000000000000000, 0.8660254037844387076, 1.000000000000000000, 0.8660254037844387076, 1.000000000000000000, 0.8660254037844387076, 1.000000000000000000, 0.8660254037844387076, 1.000000000000000000, 0.8660254037844387076, 1.000000000000000000, 0.8660254037844387076, 1.000000000000000000, 0.8660254037844387076, 1.000000000000000000, 0.8660254037844387076, 1.000000000000000000, 0.8660254037844387076, 1.000000000000000000, 0.8660254037844387076, 1.000000000000000000, 0.8660254037844387076, 1.000000000000000000, 0.8660254037844387076, 1.000000000000000000, 0.8660254037844387076, 1.000000000000000000, 0.8660254037844387076, 1.000000000000000000, 0.8660254037844387076, 1.000000000000000000, 0.8660254037844387076, 1.000000000000000000, 0.8660254037844387076, 1.000000000000000000, 0.8660254037844387076, 1.000000000000000000, 0.8660254037844387076, 1.000000000000000000, 0.8660254037844387076, 1.000000000000000000, 0.8660254037844387076, 1.000000000000000000, 0.8660254037844387076, 1.000000000000000000, 0.8660254037844387076, 1.000000000000000000, 0.8660254037844387076, 1.000000000000000000, 0.8660254037844387076, 1.000000000000000000, 0.8660254037844387076, 1.000000000000000000, 0.8660254037844387076, 1.000000000000000000, 0.8660254037844387076, 1.000000000000000000, 0.8660254037844387076, 1.000000000000000000, 0.8660254037844387076, 1.000000000000000000, 0.8660254037844387076, 1.000000000000000000, 0.8660254037844387076, 1.000000000000000000, 0.8660254037844387076, 1.000000000000000000, 0.8660254037844387076, 1.000000000000000000, 0.8660254037844387076, 1.000000000000000000, 0.8660254037844387076, 1.000000000000000000, 0.8660254037844387076, 1.000000000000000000, 0.8660254037844387076, 1.000000000000000000, 0.8660254037844387076, 1.000000000000000000, 0.8660254037844387076, 1.000000000000000000, 0.8660254037844387076, 1.000000000000000000, 0.8660254037844387076, 1.000000000000000000, 0.8660254037844387076, 1.000000000000000000, 0.8660254037844387076, 1.000000000000000000, 0.8660254037844387076, 1.000000000000000000, 0.8660254037844387076, 1.000000000000000000, 0.8660254037844387076, 1.000000000000000000, 0.8660254037844387076, 1.000000000000000000, 0.8660254037844387076, 1.000000000000000000, 0.8660254037844387076, 1.000000000000000000, 0.8660254037844387076, 1.000000000000000000, 0.8660254037844387076, 1.000000000000000000, 0.8660254037844387076, 1.000000000000000000, 0.8660254037844387076, 1.000000000000000000, 0.8660254037844387076, 1.000000000000000000, 0.8660254037844387076, 1.000000000000000000, 0.8660254037844387076, 1.000000000000000000, 0.8660254037844387076, 1.000000000000000000, 0.8660254037844387076, 1.000000000000000000, 0.8660254037844387076, 1.000000000000000000, 0.8660254037844387076, 1.000000000000000000, 0.8660254037844387076, 1.000000000000000000, 0.8660254037844387076, 1.000000000000000000, 0.8660254037844387076, 1.000000000000000000, 0.8660254037844387076, 1.000000000000000000, 0.8660254037844387076, 1.000000000000000000, 0.8660254037844387076, 1.000000000000000000, 0.8660254037844387076, 1.000000000000000000, 0.8660254037844387076, 1.000000000000000000, 0.8660254037844387076, 1.000000000000000000, 0.8660254037844387076, 1.000000000000000000, 0.8660254037844387076, 1.000000000000000000, 0.8660254037844387076, 1.000000000000000000, 0.8660254037844387076, 1.000000000000000000, 0.8660254037844387076, 1.000000000000000000, 0.8660254037844387076, 1.000000000000000000, 0.8660254037844387076, 1.000000000000000000, 0.8660254037844387076, 1.000000000000000000, 0.8660254037844387076, 1.000000000000000000, 0.8660254037844387076, 1.000000000000000000, 0.8660254037844387076, 1.000000000000000000, 0.8660254037844387076, 1.000000000000000000, 0.8660254037844387076, 1.000000000000000000, 0.8660254037844387076, 1.000000000000000000, 0.8660254037844387076, 1.000000000000000000, 0.8660254037844387076, 1.000000000000000000, 0.8660254037844387076, 1.000000000000000000, 0.8660254037844387076, 1.000000000000000000, 0.8660254037844387076, 1.000000000000000000, 0.8660254037844387076, 1.000000000000000000, 0.8660254037844387076, 1.000000000000000000, 0.8660254037844387076, 1.000000000000000000, 0.8660254037844387076, 1.000000000000000000, 0.8660254037844387076, 1.000000000000000000, 0.8660254037844387076, 1.000000000000000000, 0.8660254037844387076, 1.000000000000000000, 0.8660254037844387076, 1.000000000000000000, 0.8660254037844387076, 1.000000000000000000, 0.8660254037844387076, 1.000000000000000000, 0.8660254037844387076, 1.000000000000000000, 0.8660254037844387076, 1.000000000000000000, 0.8660254037844387076, 1.000000000000000000, 0.8660254037844387076, 1.000000000000000000, 0.8660254037844387076, 1.000000000000000000, 0.8660254037844387076, 1.000000000000000000, 0.8660254037844387076, 1.000000000000000000, 0.8660254037844387076, 1.000000000000000000, 0.8660254037844387076, 1.000000000000000000, 0.8660254037844387076, 1.000000000000000000, 0.8660254037844387076, 1.000000000000000000, 0.8660254037844387076, 1.000000000000000000, 0.8660254037844387076, 1.000000000000000000, 0.8660254037844387076, 1.000000000000000000, 0.8660254037844387076, 1.000000000000000000, 0.8660254037844387076, 1.000000000000000000, 0.8660254037844387076, 1.000000000000000000, 0.8660254037844387076, 1.000000000000000000, 0.8660254037844387076, 1.000000000000000000, 0.8660254037844387076, 1.000000000000000000, 0.8660254037844387076, 1.000000000000000000, 0.8660254037844387076, 1.000000000000000000, 0.8660254037844387076, 1.000000000000000000, 0.8660254037844387076, 1.000000000000000000, 0.8660254037844387076, 1.000000000000000000, 0.8660254037844387076, 1.000000000000000000, 0.8660254037844387076, 1.000000000000000000, 0.8660254037844387076, 1.000000000000000000, 0.8660254037844387076, 1.000000000000000000, 0.8660254037844387076, 1.000000000000000000, 0.8660254037844387076, 1.000000000000000000, 0.8660254037844387076, 1.000000000000000000, 0.8660254037844387076, 1.000000000000000000, 0.8660254037844387076, 1.000000000000000000, 0.8660254037844387076, 1.000000000000000000, 0.8660254037844387076, 1.000000000000000000, 0.8660254037844387076, 1.000000000000000000, 0.8660254037844387076, 1.000000000000000000, 0.8660254037844387076, 1.000000000000000000, 0.8660254037844387076, 1.000000000000000000, 0.8660254037844387076, 1.000000000000000000, 0.8660254037844387076, 1.000000000000000000, 0.8660254037844387076, 1.000000000000000000, 0.8660254037844387076, 1.000000000000000000, 0.8660254037844387076, 1.000000000000000000, 0.8660254037844387076, 1.000000000000000000, 0.8660254037844387076, 1.000000000000000000, 0.8660254037844387076, 1.000000000000000000, 0.8660254037844387076, 1.000000000000000000, 0.8660254037844387076, 1.000000000000000000, 0.8660254037844387076, 1.000000000000000000, 0.8660254037844387076, 1.000000000000000000, 0.8660254037844387076, 1.000000000000000000, 0.8660254037844387076, 1.000000000000000000, 0.8660254037844387076, 1.000000000000000000, 0.8660254037844387076, 1.000000000000000000, 0.8660254037844387076, 1.000000000000000000, 0.8660254037844387076, 1.000000000000000000, 0.8660254037844387076, 1.000000000000000000, 0.8660254037844387076, 1.000000000000000000, 0.8660254037844387076, 1.000000000000000000, 0.8660254037844387076, 1.000000000000000000, 0.8660254037844387076, 1.000000000000000000, 0.8660254037844387076, 1.000000000000000000, 0.8660254037844387076, 1.000000000000000000, 0.8660254037844387076, 1.000000000000000000, 0.8660254037844387076, 1.000000000000000000, 0.8660254037844387076, 1.000000000000000000, 0.8660254037844387076, 1.000000000000000000, 0.8660254037844387076, 1.000000000000000000, 0.8660254037844387076, 1.000000000000000000, 0.8660254037844387076, 1.000000000000000000, 0.8660254037844387076, 1.000000000000000000, 0.8660254037844387076, 1.000000000000000000, 0.8660254037844387076, 1.000000000000000000, 0.8660254037844387076, 1.000000000000000000, 0.8660254037844387076, 1.000000000000000000, 0.8660254037844387076, 1.000000000000000000, 0.8660254037844387076, 1.000000000000000000, 0.8660254037844387076, 1.000000000000000000, 0.8660254037844387076, 1.000000000000000000, 0.8660254037844387076, 1.000000000000000000, 0.8660254037844387076, 1.000000000000000000, 0.8660254037844387076, 1.000000000000000000, 0.8660254037844387076, 1.000000000000000000, 0.8660254037844387076, 1.000000000000000000, 0.8660254037844387076, 1.000000000000000000, 0.8660254037844387076, 1.000000000000000000, 0.8660254037844387076, 1.000000000000000000, 0.8660254037844387076, 1.000000000000000000, 0.8660254037844387076, 1.000000000000000000, 0.8660254037844387076, 1.000000000000000000, 0.8660254037844387076, 1.000000000000000000, 0.8660254037844387076, 1.000000000000000000, 0.8660254037844387076, 1.000000000000000000, 0.8660254037844387076, 1.000000000000000000, 0.8660254037844387076, 1.000000000000000000, 0.8660254037844387076, 1.000000000000000000, 0.8660254037844387076, 1.000000000000000000, 0.8660254037844387076, 1.000000000000000000, 0.8660254037844387076, 1.000000000000000000, 0.8660254037844387076, 1.000000000000000000, 0.8660254037844387076, 1.000000000000000000, 0.8660254037844387076, 1.000000000000000000, 0.8660254037844387076, 1.000000000000000000, 0.8660254037844387076, 1.000000000000000000, 0.8660254037844387076, 1.000000000000000000, 0.8660254037844387076, 1.000000000000000000, 0.8660254037844387076, 1.000000000000000000, 0.8660254037844387076, 1.000000000000000000, 0.8660254037844387076, 1.000000000000000000, 0.8660254037844387076, 1.000000000000000000, 0.8660254037844387076, 1.000000000000000000, 0.8660254037844387076, 1.000000000000000000, 0.8660254037844387076, 1.000000000000000000, 0.8660254037844387076, 1.000000000000000000, 0.8660254037844387076, 1.000000000000000000, 0.8660254037844387076, 1.000000000000000000, 0.8660254037844387076, 1.000000000000000000, 0.8660254037844387076, 1.000000000000000000, 0.8660254037844387076, 1.000000000000000000, 0.8660254037844387076, 1.000000000000000000, 0.8660254037844387076, 1.000000000000000000, 0.8660254037844387076, 1.000000000000000000, 0.8660254037844387076, 1.000000000000000000, 0.8660254037844387076, 1.000000000000000000, 0.8660254037844387076, 1.000000000000000000, 0.8660254037844387076, 1.000000000000000000, 0.8660254037844387076, 1.000000000000000000, 0.8660254037844387076, 1.000000000000000000, 0.8660254037844387076, 1.000000000000000000, 0.8660254037844387076, 1.000000000000000000, 0.8660254037844387076, 1.000000000000000000, 0.8660254037844387076, 1.000000000000000000, 0.8660254037844387076, 1.000000000000000000, 0.8660254037844387076, 1.000000000000000000, 0.8660254037844387076, 1.000000000000000000, 0.8660254037844387076, 1.000000000000000000, 0.8660254037844387076, 1.000000000000000000, 0.8660254037844387076, 1.000000000000000000, 0.8660254037844387076, 1.000000000000000000, 0.8660254037844387076, 1.000000000000000000, 0.8660254037844387076, 1.000000000000000000, 0.8660254037844387076, 1.000000000000000000, 0.8660254037844387076, 1.000000000000000000, 0.8660254037844387076, 1.000000000000000000, 0.8660254037844387076, 1.000000000000000000, 0.8660254037844387076, 1.000000000000000000, 0.8660254037844387076, 1.000000000000000000, 0.8660254037844387076, 1.000000000000000000, 0.8660254037844387076, 1.000000000000000000, 0.8660254037844387076, 1.000000000000000000, 0.8660254037844387076, 1.000000000000000000, 0.8660254037844387076, 1.000000000000000000, 0.8660254037844387076, 1.000000000000000000, 0.8660254037844387076, 1.000000000000000000, 0.8660254037844387076, 1.000000000000000000, 0.8660254037844387076, 1.000000000000000000, 0.8660254037844387076, 1.000000000000000000, 0.8660254037844387076, 1.000000000000000000, 0.8660254037844387076, 1.000000000000000000, 0.8660254037844387076, 1.000000000000000000, 0.8660254037844387076, 1.000000000000000000, 0.8660254037844387076, 1.000000000000000000, 0.8660254037844387076, 1.000000000000000000, 0.8660254037844387076, 1.000000000000000000, 0.8660254037844387076, 1.000000000000000000, 0.8660254037844387076, 1.000000000000000000, 0.8660254037844387076, 1.000000000000000000, 0.8660254037844387076, 1.000000000000000000, 0.8660254037844387076, 1.000000000000000000, 0.8660254037844387076, 1.000000000000000000, 0.8660254037844387076, 1.000000000000000000, 0.8660254037844387076, 1.000000000000000000, 0.8660254037844387076, 1.000000000000000000, 0.8660254037844387076, 1.000000000000000000, 0.8660254037844387076, 1.000000000000000000, 0.8660254037844387076, 1.000000000000000000, 0.8660254037844387076, 1.000000000000000000, 0.8660254037844387076, 1.000000000000000000, 0.8660254037844387076, 1.000000000000000000, 0.8660254037844387076, 1.000000000000000000, 0.8660254037844387076, 1.000000000000000000, 0.8660254037844387076, 1.000000000000000000, 0.8660254037844387076, 1.000000000000000000, 0.8660254037844387076, 1.000000000000000000, 0.8660254037844387076, 1.000000000000000000, 0.8660254037844387076, 1.000000000000000000, 0.8660254037844387076, 1.000000000000000000, 0.8660254037844387076, 1.000000000000000000, 0.8660254037844387076, 1.000000000000000000, 0.8660254037844387076, 1.000000000000000000, 0.8660254037844387076, 1.000000000000000000, 0.8660254037844387076, 1.000000000000000000, 0.8660254037844387076, 1.000000000000000000, 0.8660254037844387076, 1.000000000000000000, 0.8660254037844387076, 1.000000000000000000, 0.8660254037844387076, 1.000000000000000000, 0.8660254037844387076, 1.000000000000000000, 0.8660254037844387076, 1.000000000000000000, 0.8660254037844387076, 1.000000000000000000, 0.8660254037844387076, 1.000000000000000000, 0.8660254037844387076, 1.000000000000000000, 0.8660254037844387076, 1.000000000000000000, 0.8660254037844387076, 1.000000000000000000, 0.8660254037844387076, 1.000000000000000000, 0.8660254037844387076, 1.000000000000000000, 0.8660254037844387076, 1.000000000000000000, 0.8660254037844387076, 1.000000000000000000, 0.8660254037844387076, 1.000000000000000000, 0.8660254037844387076, 1.000000000000000000, 0.8660254037844387076, 1.000000000000000000, 0.8660254037844387076, 1.000000000000000000, 0.8660254037844387076, 1.000000000000000000, 0.8660254037844387076, 1.000000000000000000, 0.8660254037844387076, 1.000000000000000000, 0.8660254037844387076, 1.000000000000000000, 0.8660254037844387076, 1.000000000000000000, 0.8660254037844387076, 1.000000000000000000, 0.8660254037844387076, 1.000000000000000000, 0.8660254037844387076, 1.000000000000000000, 0.8660254037844387076, 1.000000000000000000, 0.8660254037844387076, 1.000000000000000000, 0.8660254037844387076, 1.000000000000000000, 0.8660254037844387076, 1.000000000000000000, 0.8660254037844387076, 1.000000000000000000, 0.8660254037844387076, 1.000000000000000000, 0.8660254037844387076, 1.000000000000000000, 0.8660254037844387076, 1.000000000000000000, 0.8660254037844387076, 1.000000000000000000, 0.8660254037844387076, 1.000000000000000000, 0.8660254037844387076, 1.000000000000000000, 0.8660254037844387076, 1.000000000000000000, 0.8660254037844387076, 1.000000000000000000, 0.8660254037844387076, 1.000000000000000000, 0.8660254037844387076, 1.000000000000000000, 0.8660254037844387076, 1.000000000000000000, 0.8660254037844387076, 1.000000000000000000, 0.8660254037844387076, 1.000000000000000000, 0.8660254037844387076, 1.000000000000000000, 0.8660254037844387076, 1.000000000000000000, 0.8660254037844387076, 1.000000000000000000, 0.8660254037844387076, 1.000000000000000000, 0.8660254037844387076, 1.000000000000000000, 0.8660254037844387076, 1.000000000000000000, 0.8660254037844387076, 1.000000000000000000, 0.8660254037844387076, 1.000000000000000000, 0.8660254037844387076, 1.000000000000000000, 0.8660254037844387076, 1.000000000000000000, 0.8660254037844387076, 1.000000000000000000, 0.8660254037844387076, 1.000000000000000000, 0.8660254037844387076, 1.000000000000000000, 0.8660254037844387076, 1.000000000000000000, 0.8660254037844387076, 1.000000000000000000, 0.8660254037844387076, 1.000000000000000000, 0.8660254037844387076, 1.000000000000000000, 0.8660254037844387076, 1.000000000000000000, 0.8660254037844387076, 1.000000000000000000, 0.8660254037844387076, 1.000000000000000000, 0.8660254037844387076, 1.000000000000000000, 0.8660254037844387076, 1.000000000000000000, 0.8660254037844387076, 1.000000000000000000, 0.8660254037844387076, 1.000000000000000000, 0.8660254037844387076, 1.000000000000000000, 0.8660254037844387076, 1.000000000000000000, 0.8660254037844387076, 1.000000000000000000, 0.8660254037844387076, 1.000000000000000000, 0.8660254037844387076, 1.000000000000000000, 0.8660254037844387076, 1.000000000000000000, 0.8660254037844387076, 1.000000000000000000, 0.8660254037844387076, 1.000000000000000000, 0.8660254037844387076, 1.000000000000000000, 0.8660254037844387076, 1.000000000000000000, 0.8660254037844387076, 1.000000000000000000, 0.8660254037844387076, 1.000000000000000000, 0.8660254037844387076, 1.000000000000000000, 0.8660254037844387076, 1.000000000000000000, 0.8660254037844387076, 1.000000000000000000, 0.8660254037844387076, 1.000000000000000000, 0.8660254037844387076, 1.000000000000000000, 0.8660254037844387076, 1.000000000000000000, 0.8660254037844387076, 1.000000000000000000, 0.8660254037844387076, 1.000000000000000000, 0.8660254037844387076, 1.000000000000000000, 0.8660254037844387076, 1.000000000000000000, 0.8660254037844387076, 1.000000000000000000, 0.8660254037844387076, 1.000000000000000000, 0.8660254037844387076, 1.000000000000000000, 0.8660254037844387076, 1.000000000000000000, 0.8660254037844387076, 1.000000000000000000, 0.8660254037844387076, 1.000000000000000000, 0.8660254037844387076, 1.000000000000000000, 0.8660254037844387076, 1.000000000000000000, 0.8660254037844387076, 1.000000000000000000, 0.8660254037844387076, 1.000000000000000000, 0.8660254037844387076, 1.000000000000000000, 0.8660254037844387076, 1.000000000000000000, 0.8660254037844387076, 1.000000000000000000, 0.8660254037844387076, 1.000000000000000000, 0.8660254037844387076, 1.000000000000000000, 0.8660254037844387076, 1.000000000000000000, 0.8660254037844387076, 1.000000000000000000, 0.8660254037844387076, 1.000000000000000000, 0.8660254037844387076, 1.000000000000000000, 0.8660254037844387076, 1.000000000000000000, 0.8660254037844387076, 1.000000000000000000, 0.8660254037844387076, 1.000000000000000000, 0.8660254037844387076, 1.000000000000000000, 0.8660254037844387076, 1.000000000000000000, 0.8660254037844387076, 1.000000000000000000, 0.8660254037844387076, 1.000000000000000000, 0.8660254037844387076, 1.000000000000000000, 0.8660254037844387076, 1.000000000000000000, 0.8660254037844387076, 1.000000000000000000, 0.8660254037844387076, 1.000000000000000000, 0.8660254037844387076, 1.000000000000000000, 0.8660254037844387076, 1.000000000000000000, 0.8660254037844387076, 1.000000000000000000, 0.8660254037844387076, 1.000000000000000000, 0.8660254037844387076, 1.000000000000000000, 0.8660254037844387076, 1.000000000000000000, 0.8660254037844387076, 1.000000000000000000, 0.8660254037844387076, 1.000000000000000000, 0.8660254037844387076, 1.000000000000000000, 0.8660254037844387076, 1.000000000000000000, 0.8660254037844387076, 1.000000000000000000, 0.8660254037844387076, 1.000000000000000000, 0.8660254037844387076, 1.000000000000000000, 0.8660254037844387076, 1.000000000000000000, 0.8660254037844387076, 1.000000000000000000, 0.8660254037844387076, 1.000000000000000000, 0.8660254037844387076, 1.000000000000000000, 0.8660254037844387076, 1.000000000000000000, 0.8660254037844387076, 1.000000000000000000, 0.8660254037844387076, 1.000000000000000000, 0.8660254037844387076, 1.000000000000000000, 0.8660254037844387076, 1.000000000000000000, 0.8660254037844387076, 1.000000000000000000, 0.8660254037844387076, 1.000000000000000000, 0.8660254037844387076, 1.000000000000000000, 0.8660254037844387076, 1.000000000000000000, 0.8660254037844387076, 1.000000000000000000, 0.8660254037844387076, 1.000000000000000000, 0.8660254037844387076, 1.000000000000000000, 0.8660254037844387076, 1.000000000000000000, 0.8660254037844387076, 1.000000000000000000, 0.8660254037844387076, 1.000000000000000000, 0.8660254037844387076, 1.000000000000000000, 0.8660254037844387076, 1.000000000000000000, 0.8660254037844387076, 1.000000000000000000, 0.8660254037844387076, 1.000000000000000000, 0.8660254037844387076, 1.000000000000000000, 0.8660254037844387076, 1.000000000000000000, 0.8660254037844387076, 1.000000000000000000, 0.8660254037844387076, 1.000000000000000000, 0.8660254037844387076, 1.000000000000000000, 0.8660254037844387076, 1.000000000000000000, 0.8660254037844387076, 1.000000000000000000, 0.8660254037844387076, 1.000000000000000000, 0.8660254037844387076, 1.000000000000000000, 0.8660254037844387076, 1.000000000000000000, 0.8660254037844387076, 1.000000000000000000, 0.8660254037844387076, 1.000000000000000000, 0.8660254037844387076, 1.000000000000000000, 0.8660254037844387076, 1.000000000000000000, 0.8660254037844387076, 1.000000000000000000, 0.8660254037844387076, 1.000000000000000000, 0.8660254037844387076, 1.000000000000000000, 0.8660254037844387076, 1.000000000000000000, 0.8660254037844387076, 1.000000000000000000, 0.8660254037844387076, 1.000000000000000000, 0.8660254037844387076, 1.000000000000000000, 0.8660254037844387076, 1.000000000000000000, 0.8660254037844387076, 1.000000000000000000, 0.8660254037844387076, 1.000000000000000000, 0.8660254037844387076, 1.000000000000000000, 0.8660254037844387076, 1.000000000000000000, 0.8660254037844387076, 1.000000000000000000, 0.8660254037844387076, 1.000000000000000000, 0.8660254037844387076, 1.000000000000000000, 0.8660254037844387076, 1.000000000000000000, 0.8660254037844387076, 1.000000000000000000, 0.8660254037844387076, 1.000000000000000000, 0.8660254037844387076, 1.000000000000000000, 0.8660254037844387076, 1.000000000000000000, 0.8660254037844387076, 1.000000000000000000, 0.8660254037844387076, 1.000000000000000000, 0.8660254037844387076, 1.000000000000000000, 0.8660254037844387076, 1.000000000000000000, 0.8660254037844387076, 1.000000000000000000, 0.8660254037844387076, 1.000000000000000000, 0.8660254037844387076, 1.000000000000000000, 0.8660254037844387076, 1.000000000000000000, 0.8660254037844387076, 1.000000000000000000, 0.8660254037844387076, 1.000000000000000000, 0.8660254037844387076, 1.000000000000000000, 0.8660254037844387076, 1.000000000000000000, 0.8660254037844387076, 1.000000000000000000, 0.8660254037844387076, 1.000000000000000000, 0.8660254037844387076, 1.000000000000000000, 0.8660254037844387076, 1.000000000000000000, 0.8660254037844387076, 1.000000000000000000, 0.8660254037844387076, 1.000000000000000000, 0.8660254037844387076, 1.000000000000000000, 0.8660254037844387076, 1.000000000000000000, 0.8660254037844387076, 1.000000000000000000, 0.8660254037844387076, 1.000000000000000000, 0.8660254037844387076, 1.000000000000000000, 0.8660254037844387076, 1.000000000000000000, 0.8660254037844387076, 1.000000000000000000, 0.8660254037844387076, 1.000000000000000000, 0.8660254037844387076, 1.000000000000000000, 0.8660254037844387076, 1.000000000000000000, 0.8660254037844387076, 1.000000000000000000, 0.8660254037844387076, 1.000000000000000000, 0.8660254037844387076, 1.000000000000000000, 0.8660254037844387076, 1.000000000000000000, 0.8660254037844387076, 1.000000000000000000, 0.8660254037844387076, 1.000000000000000000, 0.8660254037844387076, 1.000000000000000000, 0.8660254037844387076, 1.000000000000000000, 0.8660254037844387076, 1.000000000000000000, 0.8660254037844387076, 1.000000000000000000, 0.8660254037844387076, 1.000000000000000000, 0.8660254037844387076, 1.000000000000000000, 0.8660254037844387076, 1.000000000000000000, 0.8660254037844387076, 1.000000000000000000, 0.8660254037844387076, 1.000000000000000000, 0.8660254037844387076, 1.000000000000000000, 0.8660254037844387076, 1.000000000000000000, 0.8660254037844387076, 1.000000000000000000, 0.8660254037844387076, 1.000000000000000000, 0.8660254037844387076, 1.000000000000000000, 0.8660254037844387076, 1.000000000000000000, 0.8660254037844387076, 1.000000000000000000, 0.8660254037844387076, 1.000000000000000000, 0.8660254037844387076, 1.000000000000000000, 0.8660254037844387076, 1.000000000000000000, 0.8660254037844387076, 1.000000000000000000, 0.8660254037844387076, 1.000000000000000000, 0.8660254037844387076, 1.000000000000000000, 0.8660254037844387076, 1.000000000000000000, 0.8660254037844387076, 1.000000000000000000, 0.8660254037844387076, 1.000000000000000000, 0.8660254037844387076, 1.000000000000000000, 0.8660254037844387076, 1.000000000000000000, 0.8660254037844387076, 1.000000000000000000, 0.8660254037844387076, 1.000000000000000000, 0.8660254037844387076, 1.000000000000000000, 0.8660254037844387076, 1.000000000000000000, 0.8660254037844387076, 1.000000000000000000, 0.8660254037844387076, 1.000000000000000000, 0.8660254037844387076, 1.000000000000000000, 0.8660254037844387076, 1.000000000000000000, 0.8660254037844387076, 1.000000000000000000, 0.8660254037844387076, 1.000000000000000000, 0.8660254037844387076, 1.000000000000000000, 0.8660254037844387076, 1.000000000000000000, 0.8660254037844387076, 1.000000000000000000, 0.8660254037844387076, 1.000000000000000000, 0.8660254037844387076, 1.000000000000000000, 0.8660254037844387076, 1.000000000000000000, 0.8660254037844387076, 1.000000000000000000, 0.8660254037844387076, 1.000000000000000000, 0.8660254037844387076, 1.000000000000000000, 0.8660254037844387076, 1.000000000000000000, 0.8660254037844387076, 1.000000000000000000, 0.8660254037844387076, 1.000000000000000000, 0.8660254037844387076, 1.000000000000000000, 0.8660254037844387076, 1.000000000000000000, 0.8660254037844387076, 1.000000000000000000, 0.8660254037844387076, 1.000000000000000000, 0.8660254037844387076, 1.000000000000000000, 0.8660254037844387076, 1.000000000000000000, 0.8660254037844387076, 1.000000000000000000, 0.8660254037844387076, 1.000000000000000000, 0.8660254037844387076, 1.000000000000000000, 0.8660254037844387076, 1.000000000000000000, 0.8660254037844387076, 1.000000000000000000, 0.8660254037844387076, 1.000000000000000000, 0.8660254037844387076, 1.000000000000000000, 0.8660254037844387076, 1.000000000000000000, 0.8660254037844387076, 1.000000000000000000, 0.8660254037844387076, 1.000000000000000000, 0.8660254037844387076, 1.000000000000000000, 0.8660254037844387076, 1.000000000000000000, 0.8660254037844387076, 1.000000000000000000, 0.8660254037844387076, 1.000000000000000000, 0.8660254037844387076, 1.000000000000000000, 0.8660254037844387076, 1.000000000000000000, 0.8660254037844387076, 1.000000000000000000, 0.8660254037844387076, 1.000000000000000000, 0.8660254037844387076, 1.000000000000000000, 0.8660254037844387076, 1.000000000000000000, 0.8660254037844387076, 1.000000000000000000, 0.8660254037844387076, 1.000000000000000000, 0.8660254037844387076, 1.000000000000000000, 0.8660254037844387076, 1.000000000000000000, 0.8660254037844387076, 1.000000000000000000, 0.8660254037844387076, 1.000000000000000000, 0.8660254037844387076, 1.000000000000000000, 0.8660254037844387076, 1.000000000000000000, 0.8660254037844387076, 1.000000000000000000, 0.8660254037844387076, 1.000000000000000000, 0.8660254037844387076, 1.000000000000000000, 0.8660254037844387076, 1.000000000000000000, 0.8660254037844387076, 1.000000000000000000, 0.8660254037844387076, 1.000000000000000000, 0.8660254037844387076, 1.000000000000000000, 0.8660254037844387076, 1.000000000000000000, 0.8660254037844387076, 1.000000000000000000, 0.8660254037844387076, 1.000000000000000000, 0.8660254037844387076, 1.000000000000000000, 0.8660254037844387076, 1.000000000000000000, 0.8660254037844387076, 1.000000000000000000, 0.8660254037844387076, 1.000000000000000000, 0.8660254037844387076, 1.000000000000000000, 0.8660254037844387076, 1.000000000000000000, 0.8660254037844387076, 1.000000000000000000, 0.8660254037844387076, 1.000000000000000000, 0.8660254037844387076, 1.000000000000000000, 0.8660254037844387076, 1.000000000000000000, 0.8660254037844387076, 1.000000000000000000, 0.8660254037844387076, 1.000000000000000000, 0.8660254037844387076, 1.000000000000000000, 0.8660254037844387076, 1.000000000000000000, 0.8660254037844387076, 1.000000000000000000, 0.8660254037844387076, 1.000000000000000000, 0.8660254037844387076, 1.000000000000000000, 0.8660254037844387076, 1.000000000000000000, 0.8660254037844387076, 1.000000000000000000, 0.8660254037844387076, 1.000000000000000000, 0.8660254037844387076, 1.000000000000000000, 0.8660254037844387076, 1.000000000000000000, 0.8660254037844387076, 1.000000000000000000, 0.8660254037844387076, 1.000000000000000000, 0.8660254037844387076, 1.000000000000000000, 0.8660254037844387076, 1.000000000000000000, 0.8660254037844387076, 1.000000000000000000, 0.8660254037844387076, 1.000000000000000000, 0.8660254037844387076, 1.000000000000000000, 0.8660254037844387076, 1.000000000000000000, 0.8660254037844387076, 1.000000000000000000, 0.8660254037844387076, 1.000000000000000000, 0.8660254037844387076, 1.000000000000000000, 0.8660254037844387076, 1.000000000000000000, 0.8660254037844387076, 1.000000000000000000, 0.8660254037844387076, 1.000000000000000000, 0.8660254037844387076, 1.000000000000000000, 0.8660254037844387076, 1.000000000000000000, 0.8660254037844387076, 1.000000000000000000, 0.8660254037844387076, 1.000000000000000000, 0.8660254037844387076, 1.000000000000000000, 0.8660254037844387076, 1.000000000000000000, 0.8660254037844387076, 1.000000000000000000, 0.8660254037844387076, 1.000000000000000000, 0.8660254037844387076, 1.000000000000000000, 0.8660254037844387076, 1.000000000000000000, 0.8660254037844387076, 1.000000000000000000, 0.8660254037844387076, 1.000000000000000000, 0.8660254037844387076, 1.000000000000000000, 0.8660254037844387076, 1.000000000000000000, 0.8660254037844387076, 1.000000000000000000, 0.8660254037844387076, 1.000000000000000000, 0.8660254037844387076, 1.000000000000000000, 0.8660254037844387076, 1.000000000000000000, 0.8660254037844387076, 1.000000000000000000, 0.8660254037844387076, 1.000000000000000000, 0.8660254037844387076, 1.000000000000000000, 0.8660254037844387076, 1.000000000000000000, 0.8660254037844387076, 1.000000000000000000, 0.8660254037844387076, 1.000000000000000000, 0.8660254037844387076, 1.000000000000000000, 0.8660254037844387076, 1.000000000000000000, 0.8660254037844387076, 1.000000000000000000, 0.8660254037844387076, 1.000000000000000000, 0.8660254037844387076, 1.000000000000000000, 0.8660254037844387076, 1.000000000000000000, 0.8660254037844387076, 1.000000000000000000, 0.8660254037844387076, 1.000000000000000000, 0.8660254037844387076, 1.000000000000000000, 0.8660254037844387076, 1.000000000000000000, 0.8660254037844387076, 1.000000000000000000, 0.8660254037844387076, 1.000000000000000000, 0.8660254037844387076, 1.000000000000000000, 0.8660254037844387076, 1.000000000000000000, 0.8660254037844387076, 1.000000000000000000, 0.8660254037844387076, 1.000000000000000000, 0.8660254037844387076, 1.000000000000000000, 0.8660254037844387076, 1.000000000000000000, 0.8660254037844387076, 1.000000000000000000, 0.8660254037844387076, 1.000000000000000000, 0.8660254037844387076, 1.000000000000000000, 0.8660254037844387076, 1.000000000000000000, 0.8660254037844387076, 1.000000000000000000, 0.8660254037844387076, 1.000000000000000000, 0.8660254037844387076, 1.000000000000000000, 0.8660254037844387076, 1.000000000000000000, 0.8660254037844387076, 1.000000000000000000, 0.8660254037844387076, 1.000000000000000000, 0.8660254037844387076, 1.000000000000000000, 0.8660254037844387076, 1.000000000000000000, 0.8660254037844387076, 1.000000000000000000, 0.8660254037844387076, 1.000000000000000000, 0.8660254037844387076, 1.000000000000000000, 0.8660254037844387076, 1.000000000000000000, 0.8660254037844387076, 1.000000000000000000, 0.8660254037844387076, 1.000000000000000000, 0.8660254037844387076, 1.000000000000000000, 0.8660254037844387076, 1.000000000000000000, 0.8660254037844387076, 1.000000000000000000, 0.8660254037844387076, 1.000000000000000000, 0.8660254037844387076, 1.000000000000000000, 0.8660254037844387076, 1.000000000000000000, 0.8660254037844387076, 1.000000000000000000, 0.8660254037844387076, 1.000000000000000000, 0.8660254037844387076, 1.000000000000000000, 0.8660254037844387076, 1.000000000000000000, 0.8660254037844387076, 1.000000000000000000, 0.8660254037844387076, 1.000000000000000000, 0.8660254037844387076, 1.000000000000000000, 0.8660254037844387076, 1.000000000000000000, 0.8660254037844387076, 1.000000000000000000, 0.8660254037844387076, 1.000000000000000000, 0.8660254037844387076, 1.000000000000000000, 0.8660254037844387076, 1.000000000000000000, 0.8660254037844387076, 1.000000000000000000, 0.8660254037844387076, 1.000000000000000000, 0.8660254037844387076, 1.000000000000000000, 0.8660254037844387076, 1.000000000000000000, 0.8660254037844387076, 1.000000000000000000, 0.8660254037844387076, 1.000000000000000000, 0.8660254037844387076, 1.000000000000000000, 0.8660254037844387076, 1.000000000000000000, 0.8660254037844387076, 1.000000000000000000, 0.8660254037844387076, 1.000000000000000000, 0.8660254037844387076, 1.000000000000000000, 0.8660254037844387076, 1.000000000000000000, 0.8660254037844387076, 1.000000000000000000, 0.8660254037844387076, 1.000000000000000000, 0.8660254037844387076, 1.000000000000000000, 0.8660254037844387076, 1.000000000000000000, 0.8660254037844387076, 1.000000000000000000, 0.8660254037844387076, 1.000000000000000000) ) ) 
 REPRESENTATION_ITEM ( '' )  SURFACE ( )  );
#1064=CARTESIAN_POINT ( 'NONE',  ( 7.216878364870408014, 17.50000000000005684, 49.99999999999998579 ) ) ;
#1065=EDGE_CURVE ( 'NONE', #26359, #40867, #25993, .T. ) ;
#1066=CARTESIAN_POINT ( 'NONE',  ( -10.81189881249999729, -6.242252689847864744, -124.9687500020483810 ) ) ;
#1070=CARTESIAN_POINT ( 'NONE',  ( 7.070501591499377789E-16, 11.54700538379251284, -183.5000000040968189 ) ) ;
#1072=CARTESIAN_POINT ( 'NONE',  ( -5.405949406249996869, 9.363379034771805109, -179.5312500020483810 ) ) ;
#1073=DIRECTION ( 'NONE',  ( -0.000000000000000000, -0.000000000000000000, 1.000000000000000000 ) ) ;
#1075=CARTESIAN_POINT ( 'NONE',  ( 10.81189881249999551, -6.242252689847874514, -55.46875000204837391 ) ) ;
#1076=CARTESIAN_POINT ( 'NONE',  ( 5.405949406249992428, -9.363379034771808662, -43.59375000204837391 ) ) ;
#1078=CARTESIAN_POINT ( 'NONE',  ( 7.644554776091147741E-16, 12.48450537969573659, -11.65625000204835438 ) ) ;
#1082=CARTESIAN_POINT ( 'NONE',  ( -4.999999999999996447, 8.660254037844387298, -97.49999999999998579 ) ) ;
#1084=CARTESIAN_POINT ( 'NONE',  ( 9.999999999999998224, 0.000000000000000000, -111.8750000040967763 ) ) ;
#1085=CARTESIAN_POINT ( 'NONE',  ( 10.00000000000102318, -5.773502691895667560, -26.50000000409674783 ) ) ;
#1088=CARTESIAN_POINT ( 'NONE',  ( -10.81189881249999729, 6.242252689847871849, -104.4062500020483810 ) ) ;
#1089=ORIENTED_EDGE ( 'NONE', *, *, #19593, .T. ) ;
#1094=VERTEX_POINT ( 'NONE', #3320 ) ;
#1095=CARTESIAN_POINT ( 'NONE',  ( 9.999999999999996447, -5.773502691896262640, -23.12499999999998224 ) ) ;
#1096=CARTESIAN_POINT ( 'NONE',  ( -10.81189881249999729, -6.242252689847864744, -38.15625000204835260 ) ) ;
#1097=CARTESIAN_POINT ( 'NONE',  ( -2.121150477449813534E-15, -11.54700538379251284, -159.8750000000000000 ) ) ;
#1098=CARTESIAN_POINT ( 'NONE',  ( -9.999999999999998224, 1.224646799147353059E-15, -200.0000000000000000 ) ) ;
#1102=CARTESIAN_POINT ( 'NONE',  ( -10.81189881249999729, 6.242252689847871849, -135.9062500020484094 ) ) ;
#1103=CARTESIAN_POINT ( 'NONE',  ( -9.999999999999998224, 1.224646799147353059E-15, -110.7499999999999858 ) ) ;
#1105=ORIENTED_EDGE ( 'NONE', *, *, #20888, .F. ) ;
#1106=ORIENTED_EDGE ( 'NONE', *, *, #39009, .F. ) ;
#1107=EDGE_LOOP ( 'NONE', ( #37460, #22915, #24371, #22762 ) ) ;
#1109=CARTESIAN_POINT ( 'NONE',  ( 10.00000000000051159, -5.773502691895965988, -146.5000000040967620 ) ) ;
#1110=CARTESIAN_POINT ( 'NONE',  ( -10.81189881249999729, 6.242252689847871849, -168.7187500020483810 ) ) ;
#1112=CARTESIAN_POINT ( 'NONE',  ( -10.81189881249999729, 1.324075727343319199E-15, -14.09375000204834905 ) ) ;
#1113=CARTESIAN_POINT ( 'NONE',  ( -9.999999999999872102, -5.773502691896326589, -157.5000000040968189 ) ) ;
#1114=EDGE_CURVE ( 'NONE', #36127, #7309, #20938, .T. ) ;
#1115=CARTESIAN_POINT ( 'NONE',  ( 10.81189881249999729, 6.242252689847867408, -148.2187500020484094 ) ) ;
#1116=CARTESIAN_POINT ( 'NONE',  ( -5.405949406250003975, -9.363379034771801557, -133.8437500020484094 ) ) ;
#1118=CARTESIAN_POINT ( 'NONE',  ( -10.81189881249999729, 6.242252689847871849, -108.9062500020483810 ) ) ;
#1123=CARTESIAN_POINT ( 'NONE',  ( 5.405949406249999534, 9.363379034771803333, -8.593750002048345493 ) ) ;
#1125=CARTESIAN_POINT ( 'NONE',  ( -10.81189881249999729, 6.242252689847871849, -198.9062500020484094 ) ) ;
#1126=CARTESIAN_POINT ( 'NONE',  ( -9.999999999999941380, -5.773502691896284844, -196.5000000040967905 ) ) ;
#1129=CARTESIAN_POINT ( 'NONE',  ( -2.293366432827344421E-15, -12.48450537969573659, -75.21875000204839523 ) ) ;
#1130=CARTESIAN_POINT ( 'NONE',  ( -2.293366432827344421E-15, -12.48450537969573659, -61.71875000204838102 ) ) ;
#1132=CARTESIAN_POINT ( 'NONE',  ( -5.405949406250003975, -9.363379034771801557, -38.03125000204838102 ) ) ;
#1134=CARTESIAN_POINT ( 'NONE',  ( 9.999999999999676703, 5.773502691896441164, -186.3749999999999716 ) ) ;
#1136=CARTESIAN_POINT ( 'NONE',  ( -10.00000000000000000, -5.773502691896251982, -121.1250000000000000 ) ) ;
#1137=CARTESIAN_POINT ( 'NONE',  ( 10.81189881249999551, -6.242252689847874514, -129.1562500020483810 ) ) ;
#1140=CARTESIAN_POINT ( 'NONE',  ( 5.405949406249992428, -9.363379034771808662, -15.28125000204835793 ) ) ;
#1145=CARTESIAN_POINT ( 'NONE',  ( 7.070501591499377789E-16, 11.54700538379251284, -30.50000000409674428 ) ) ;
#1146=EDGE_CURVE ( 'NONE', #1053, #28503, #9337, .T. ) ;
#1147=DIRECTION ( 'NONE',  ( -0.000000000000000000, -0.000000000000000000, 1.000000000000000000 ) ) ;
#1150=CARTESIAN_POINT ( 'NONE',  ( -10.81189881249999729, 1.324075727343319199E-15, -152.2812500020484094 ) ) ;
#1151=CARTESIAN_POINT ( 'NONE',  ( 7.644554776091147741E-16, 12.48450537969573659, -128.4687500020483810 ) ) ;
#1153=EDGE_CURVE ( 'NONE', #2376, #36659, #12347, .T. ) ;
#1155=ORIENTED_EDGE ( 'NONE', *, *, #36440, .T. ) ;
#1156=( BOUNDED_CURVE ( )  B_SPLINE_CURVE ( 2, ( #33824, #34256, #7918, #20635, #8132, #1445, #30162 ),
 .UNSPECIFIED., .F., .F. ) 
 B_SPLINE_CURVE_WITH_KNOTS ( ( 3, 2, 2, 3 ),
 ( 0.5410447761194030480, 0.5422885572139304333, 0.5435323383084578186, 0.5447761194029852039 ),
 .UNSPECIFIED. ) 
 CURVE ( )  GEOMETRIC_REPRESENTATION_ITEM ( )  RATIONAL_B_SPLINE_CURVE ( ( 0.9999999999999880096, 0.8660254037844506980, 1.000000000000000000, 0.8660254037844387076, 1.000000000000000000, 0.8660254037844267172, 1.000000000000011990 ) ) 
 REPRESENTATION_ITEM ( '' )  );
#1158=ORIENTED_EDGE ( 'NONE', *, *, #32558, .F. ) ;
#1159=ORIENTED_EDGE ( 'NONE', *, *, #42513, .F. ) ;
#1160=CARTESIAN_POINT ( 'NONE',  ( -10.81189881249999729, 6.242252689847871849, -111.7187500020483810 ) ) ;
#1163=CARTESIAN_POINT ( 'NONE',  ( 10.81189881249999907, 6.242252689847868297, -191.7187500020484094 ) ) ;
#1164=CARTESIAN_POINT ( 'NONE',  ( -10.81189881249999729, 6.242252689847871849, -42.71875000204835970 ) ) ;
#1165=CARTESIAN_POINT ( 'NONE',  ( 8.614196012143711556, -6.533971456633876684, 2.775557561562891351E-14 ) ) ;
#1166=CARTESIAN_POINT ( 'NONE',  ( -9.999999999999998224, 1.224646799147353059E-15, -186.1250000040967905 ) ) ;
#1167=EDGE_CURVE ( 'NONE', #36659, #35302, #38582, .T. ) ;
#1168=CARTESIAN_POINT ( 'NONE',  ( 10.81189881249999729, 0.000000000000000000, -169.3437500020484094 ) ) ;
#1169=CARTESIAN_POINT ( 'NONE',  ( 10.81189881249999551, -6.242252689847874514, -157.4687500020484094 ) ) ;
#1173=ADVANCED_FACE ( 'NONE', ( #14059 ), #17521, .T. ) ;
#1174=CARTESIAN_POINT ( 'NONE',  ( -9.999999999999998224, 1.224646799147353059E-15, -133.6250000040967620 ) ) ;
#1177=EDGE_CURVE ( 'NONE', #32541, #42118, #16755, .T. ) ;
#1178=CARTESIAN_POINT ( 'NONE',  ( -5.405949406250003975, -9.363379034771801557, -90.34375000204838102 ) ) ;
#1179=CARTESIAN_POINT ( 'NONE',  ( 5.000000000000000000, 8.660254037844385522, -180.6250000040967905 ) ) ;
#1180=CARTESIAN_POINT ( 'NONE',  ( -2.293366432827344421E-15, -12.48450537969573659, -61.90625000204838813 ) ) ;
#1181=CARTESIAN_POINT ( 'NONE',  ( -4.999999999999996447, 8.660254037844387298, -145.8750000040967905 ) ) ;
#1183=CARTESIAN_POINT ( 'NONE',  ( 10.81189881249999907, 6.242252689847868297, -121.4062500020483810 ) ) ;
#1184=CARTESIAN_POINT ( 'NONE',  ( -5.405949406250003975, -9.363379034771801557, -155.0312500020484094 ) ) ;
#1185=LINE ( 'NONE', #16759, #26838 ) ;
#1187=CARTESIAN_POINT ( 'NONE',  ( 9.999999999999998224, 0.000000000000000000, -131.3750000040967905 ) ) ;
#1193=CARTESIAN_POINT ( 'NONE',  ( -10.81189881249999907, -6.242252689847864744, -192.6562500020484094 ) ) ;
#1195=CARTESIAN_POINT ( 'NONE',  ( -10.00000000000000000, -5.773502691896251982, -46.12499999999996447 ) ) ;
#1197=CARTESIAN_POINT ( 'NONE',  ( -10.00000000000000000, -5.773502691896251982, -61.50000000409677625 ) ) ;
#1198=PLANE ( 'NONE',  #2272 ) ;
#1200=CARTESIAN_POINT ( 'NONE',  ( -2.293366432827344421E-15, -12.48450537969573659, -48.40625000204836681 ) ) ;
#1206=CARTESIAN_POINT ( 'NONE',  ( 7.644554776091147741E-16, 12.48450537969573659, -173.6562500020483810 ) ) ;
#1210=CARTESIAN_POINT ( 'NONE',  ( 9.999999999999742428, 5.773502691896404748, -154.8749999999999716 ) ) ;
#1211=CYLINDRICAL_SURFACE ( 'NONE', #38312, 9.999999999999998224 ) ;
#1212=( BOUNDED_CURVE ( )  B_SPLINE_CURVE ( 2, ( #485, #9385, #10375, #13814, #17269, #27005, #40154 ),
 .UNSPECIFIED., .F., .F. ) 
 B_SPLINE_CURVE_WITH_KNOTS ( ( 3, 2, 2, 3 ),
 ( 0.4253731343283583266, 0.4266169154228856564, 0.4278606965174130417, 0.4291044776119404269 ),
 .UNSPECIFIED. ) 
 CURVE ( )  GEOMETRIC_REPRESENTATION_ITEM ( )  RATIONAL_B_SPLINE_CURVE ( ( 0.9999999999999880096, 0.8660254037844506980, 1.000000000000000000, 0.8660254037844387076, 1.000000000000000000, 0.8660254037844267172, 1.000000000000011990 ) ) 
 REPRESENTATION_ITEM ( '' )  );
#1213=CARTESIAN_POINT ( 'NONE',  ( 4.999999999999992006, -8.660254037844389075, -20.24999999999996092 ) ) ;
#1214=CARTESIAN_POINT ( 'NONE',  ( -10.81189881249999729, 1.324075727343319199E-15, -87.78125000204838102 ) ) ;
#1215=EDGE_LOOP ( 'NONE', ( #11227, #37033, #21372, #11979 ) ) ;
#1217=CARTESIAN_POINT ( 'NONE',  ( 9.999999999999998224, 0.000000000000000000, -128.3750000040967905 ) ) ;
#1218=ORIENTED_EDGE ( 'NONE', *, *, #3677, .T. ) ;
#1219=ORIENTED_EDGE ( 'NONE', *, *, #1586, .T. ) ;
#1220=CARTESIAN_POINT ( 'NONE',  ( -10.81189881249999729, 1.324075727343319199E-15, -35.09375000204836681 ) ) ;
#1221=CARTESIAN_POINT ( 'NONE',  ( 10.81189881249999907, 6.242252689847868297, -29.71875000204834194 ) ) ;
#1222=CARTESIAN_POINT ( 'NONE',  ( 5.405949406249999534, 9.363379034771803333, -14.78125000204835793 ) ) ;
#1223=CARTESIAN_POINT ( 'NONE',  ( -5.405949406249996869, 9.363379034771805109, -62.34375000204836681 ) ) ;
#1224=CARTESIAN_POINT ( 'NONE',  ( 9.999999999999998224, 0.000000000000000000, -17.37500000409675138 ) ) ;
#1226=CARTESIAN_POINT ( 'NONE',  ( -5.405949406250003975, -9.363379034771801557, -187.8437500020483810 ) ) ;
#1228=CARTESIAN_POINT ( 'NONE',  ( -9.999999999999998224, 1.224646799147353059E-15, -43.24999999999998579 ) ) ;
#1230=CARTESIAN_POINT ( 'NONE',  ( -10.00000000000051337, 5.773502691895962435, -140.8750000000000000 ) ) ;
#1233=CARTESIAN_POINT ( 'NONE',  ( 10.81189881249999729, 0.000000000000000000, -115.3437500020483810 ) ) ;
#1236=CARTESIAN_POINT ( 'NONE',  ( -5.405949406250003975, -9.363379034771801557, -81.53125000204839523 ) ) ;
#1237=CARTESIAN_POINT ( 'NONE',  ( 10.81189881249999551, -6.242252689847874514, -103.4687500020483668 ) ) ;
#1241=CARTESIAN_POINT ( 'NONE',  ( 9.999999999999996447, -5.773502691896262640, -157.0000000040968189 ) ) ;
#1245=EDGE_CURVE ( 'NONE', #22331, #11539, #29776, .T. ) ;
#1247=DIRECTION ( 'NONE',  ( 1.000000000000000000, 0.000000000000000000, 0.000000000000000000 ) ) ;
#1249=CARTESIAN_POINT ( 'NONE',  ( 5.000000000000000000, 8.660254037844385522, -120.6250000040967905 ) ) ;
#1250=CARTESIAN_POINT ( 'NONE',  ( 9.999999999999996447, -5.773502691896262640, -72.62499999999995737 ) ) ;
#1252=CARTESIAN_POINT ( 'NONE',  ( 9.999999999999996447, -5.773502691896262640, -82.00000000409676204 ) ) ;
#1253=DIRECTION ( 'NONE',  ( -0.000000000000000000, -0.000000000000000000, 1.000000000000000000 ) ) ;
#1255=CARTESIAN_POINT ( 'NONE',  ( 7.644554776091147741E-16, 12.48450537969573659, -73.15625000204836681 ) ) ;
#1259=EDGE_LOOP ( 'NONE', ( #38574, #7850, #2382, #2551 ) ) ;
#1260=CARTESIAN_POINT ( 'NONE',  ( -4.999999999999996447, 8.660254037844387298, 2.775557561562891351E-14 ) ) ;
#1262=CARTESIAN_POINT ( 'NONE',  ( -5.405949406250003975, -9.363379034771801557, -15.34375000204835082 ) ) ;
#1263=CARTESIAN_POINT ( 'NONE',  ( 10.00000000000044764, -5.773502691896004180, -176.5000000040967905 ) ) ;
#1265=CARTESIAN_POINT ( 'NONE',  ( 10.81189881249999551, -6.242252689847874514, -130.6562500020484094 ) ) ;
#1266=CARTESIAN_POINT ( 'NONE',  ( 9.999999999999996447, -5.773502691896262640, -180.6250000000000284 ) ) ;
#1267=DIRECTION ( 'NONE',  ( -0.000000000000000000, -0.000000000000000000, 1.000000000000000000 ) ) ;
#1268=CARTESIAN_POINT ( 'NONE',  ( -10.81189881249999729, 1.324075727343319199E-15, -113.2812500020483952 ) ) ;
#1269=VERTEX_POINT ( 'NONE', #17953 ) ;
#1270=CARTESIAN_POINT ( 'NONE',  ( 9.999999999999998224, 0.000000000000000000, -153.8750000040967905 ) ) ;
#1271=EDGE_LOOP ( 'NONE', ( #25258, #42176, #4809, #27326 ) ) ;
#1272=ORIENTED_EDGE ( 'NONE', *, *, #2506, .F. ) ;
#1273=CARTESIAN_POINT ( 'NONE',  ( 7.644554776091147741E-16, 12.48450537969573659, -38.65625000204835260 ) ) ;
#1275=CARTESIAN_POINT ( 'NONE',  ( -10.81189881249999729, 1.324075727343319199E-15, -90.59375000204838102 ) ) ;
#1278=LINE ( 'NONE', #14406, #27426 ) ;
#1280=CARTESIAN_POINT ( 'NONE',  ( -4.999999999999996447, 8.660254037844387298, -58.49999999999997158 ) ) ;
#1281=CARTESIAN_POINT ( 'NONE',  ( -5.405949406250003975, -9.363379034771801557, -121.8437500020483952 ) ) ;
#1283=CARTESIAN_POINT ( 'NONE',  ( -10.81189881249999729, 1.324075727343319199E-15, -2.281250002048373915 ) ) ;
#1284=CARTESIAN_POINT ( 'NONE',  ( 0.000000000000000000, 0.000000000000000000, -200.0000000000000000 ) ) ;
#1286=CARTESIAN_POINT ( 'NONE',  ( -2.121150477449813534E-15, -11.54700538379251284, -179.7500000040967905 ) ) ;
#1288=CARTESIAN_POINT ( 'NONE',  ( -5.405949406249996869, 9.363379034771805109, -176.5312500020483810 ) ) ;
#1289=CARTESIAN_POINT ( 'NONE',  ( -7.423074889580966840, 12.85714285714296246, 52.14285714285716011 ) ) ;
#1292=CARTESIAN_POINT ( 'NONE',  ( 5.405949406249999534, 9.363379034771803333, -55.09375000204835970 ) ) ;
#1294=CARTESIAN_POINT ( 'NONE',  ( -10.81189881249999729, 6.242252689847871849, -11.40625000204835438 ) ) ;
#1297=CARTESIAN_POINT ( 'NONE',  ( -10.00000000000000000, -5.773502691896251982, -95.62499999999998579 ) ) ;
#1299=CARTESIAN_POINT ( 'NONE',  ( 7.070501591499377789E-16, 11.54700538379251284, -102.5000000040967763 ) ) ;
#1300=CARTESIAN_POINT ( 'NONE',  ( 0.000000000000000000, 0.000000000000000000, -200.0000000000000000 ) ) ;
#1303=CARTESIAN_POINT ( 'NONE',  ( -10.81189881249999729, 1.324075727343319199E-15, -107.2812500020483810 ) ) ;
#1305=LINE ( 'NONE', #40341, #10004 ) ;
#1307=CARTESIAN_POINT ( 'NONE',  ( 10.81189881249999551, -6.242252689847874514, -162.1562500020484379 ) ) ;
#1310=CARTESIAN_POINT ( 'NONE',  ( 5.000000000000000000, 8.660254037844385522, -28.74999999999997158 ) ) ;
#1311=CARTESIAN_POINT ( 'NONE',  ( -5.405949406250003975, -9.363379034771801557, -36.53125000204837391 ) ) ;
#1312=CARTESIAN_POINT ( 'NONE',  ( -9.999999999999998224, 5.773502691896259087, -163.3750000000000000 ) ) ;
#1313=EDGE_CURVE ( 'NONE', #37408, #38561, #36933, .T. ) ;
#1314=CARTESIAN_POINT ( 'NONE',  ( -9.999999999999998224, 1.224646799147353059E-15, -135.1250000040967620 ) ) ;
#1317=CARTESIAN_POINT ( 'NONE',  ( -10.81189881249999907, -6.242252689847864744, -131.1562500020483810 ) ) ;
#1318=CARTESIAN_POINT ( 'NONE',  ( 9.999999999998969713, 5.773502691896851502, -46.87499999999994316 ) ) ;
#1319=CARTESIAN_POINT ( 'NONE',  ( 0.000000000000000000, 0.000000000000000000, -200.0000000000000000 ) ) ;
#1320=ORIENTED_EDGE ( 'NONE', *, *, #37835, .T. ) ;
#1321=( BOUNDED_CURVE ( )  B_SPLINE_CURVE ( 2, ( #28186, #41956, #11757, #24958, #2496, #12181, #25372 ),
 .UNSPECIFIED., .F., .F. ) 
 B_SPLINE_CURVE_WITH_KNOTS ( ( 3, 2, 2, 3 ),
 ( 0.2947761194029852039, 0.2960199004975125336, 0.2972636815920398634, 0.2985074626865671932 ),
 .UNSPECIFIED. ) 
 CURVE ( )  GEOMETRIC_REPRESENTATION_ITEM ( )  RATIONAL_B_SPLINE_CURVE ( ( 0.9999999999999880096, 0.8660254037844506980, 1.000000000000000000, 0.8660254037844387076, 1.000000000000000000, 0.8660254037844327124, 1.000000000000005995 ) ) 
 REPRESENTATION_ITEM ( '' )  );
#1323=ORIENTED_EDGE ( 'NONE', *, *, #1691, .F. ) ;
#1326=DIRECTION ( 'NONE',  ( 1.000000000000000000, 0.000000000000000000, 0.000000000000000000 ) ) ;
#1327=CARTESIAN_POINT ( 'NONE',  ( 5.405949406249992428, -9.363379034771808662, -166.5937500020484094 ) ) ;
#1329=CARTESIAN_POINT ( 'NONE',  ( 10.81189881249999729, 0.000000000000000000, -16.34375000204835260 ) ) ;
#1330=VECTOR ( 'NONE', #32095, 1000.000000000000000 ) ;
#1332=CARTESIAN_POINT ( 'NONE',  ( 5.405949406249999534, 9.363379034771803333, -151.0937500020483810 ) ) ;
#1333=CARTESIAN_POINT ( 'NONE',  ( 5.405949406249999534, 9.363379034771803333, -134.5937500020483810 ) ) ;
#1334=CARTESIAN_POINT ( 'NONE',  ( 10.81189881249999551, -6.242252689847874514, -109.6562500020483810 ) ) ;
#1338=CARTESIAN_POINT ( 'NONE',  ( -9.999999999999998224, 1.224646799147353059E-15, -198.1250000040967905 ) ) ;
#1341=AXIS2_PLACEMENT_3D ( 'NONE', #35377, #16116, #22841 ) ;
#1342=CARTESIAN_POINT ( 'NONE',  ( -2.121150477449813534E-15, -11.54700538379251284, -178.2500000040968189 ) ) ;
#1345=CARTESIAN_POINT ( 'NONE',  ( -5.405949406249996869, 9.363379034771805109, -78.84375000204838102 ) ) ;
#1346=CARTESIAN_POINT ( 'NONE',  ( -10.81189881249999729, 6.242252689847871849, -68.21875000204838102 ) ) ;
#1348=CARTESIAN_POINT ( 'NONE',  ( 10.81189881249999729, 0.000000000000000000, -31.53125000204837391 ) ) ;
#1351=CARTESIAN_POINT ( 'NONE',  ( -10.00000000000000000, -5.773502691896251982, -122.6250000000000000 ) ) ;
#1352=CARTESIAN_POINT ( 'NONE',  ( 10.81189881249999729, 6.242252689847867408, -128.9062500020483810 ) ) ;
#1355=CARTESIAN_POINT ( 'NONE',  ( -10.81189881249999729, 6.242252689847871849, -21.90625000204837036 ) ) ;
#1356=ORIENTED_EDGE ( 'NONE', *, *, #105, .T. ) ;
#1360=CARTESIAN_POINT ( 'NONE',  ( 9.999999999999998224, 0.000000000000000000, -35.37500000409676915 ) ) ;
#1361=CARTESIAN_POINT ( 'NONE',  ( 9.999999999999998224, 0.000000000000000000, -61.99999999999997158 ) ) ;
#1363=CARTESIAN_POINT ( 'NONE',  ( 5.000000000000000000, 8.660254037844385522, -147.2500000000000000 ) ) ;
#1364=CARTESIAN_POINT ( 'NONE',  ( -5.405949406249996869, 9.363379034771805109, -157.0312500020484094 ) ) ;
#1365=AXIS2_PLACEMENT_3D ( 'NONE', #20346, #13856, #29869 ) ;
#1366=CARTESIAN_POINT ( 'NONE',  ( 7.644554776091147741E-16, 12.48450537969573659, -129.9687500020483810 ) ) ;
#1367=DIRECTION ( 'NONE',  ( -0.000000000000000000, -0.000000000000000000, 1.000000000000000000 ) ) ;
#1368=ADVANCED_FACE ( 'NONE', ( #12127 ), #31366, .T. ) ;
#1371=VERTEX_POINT ( 'NONE', #25318 ) ;
#1374=CARTESIAN_POINT ( 'NONE',  ( -10.81189881249999907, -6.242252689847864744, -114.4687500020483810 ) ) ;
#1376=CARTESIAN_POINT ( 'NONE',  ( 9.999999999999998224, 0.000000000000000000, -200.0000000000000000 ) ) ;
#1377=CARTESIAN_POINT ( 'NONE',  ( -10.81189881249999729, 1.324075727343319199E-15, -188.0937500020483810 ) ) ;
#1378=CARTESIAN_POINT ( 'NONE',  ( -10.81189881249999729, 1.324075727343319199E-15, -38.09375000204837391 ) ) ;
#1379=CARTESIAN_POINT ( 'NONE',  ( -1.290480703760489067, -10.30757810694964327, 1.243155832063081332E-14 ) ) ;
#1381=CARTESIAN_POINT ( 'NONE',  ( -10.81189881249999729, -6.242252689847864744, -168.4687500020483526 ) ) ;
#1382=CARTESIAN_POINT ( 'NONE',  ( -10.81189881249999729, 1.324075727343319199E-15, -164.0937500020484094 ) ) ;
#1387=CARTESIAN_POINT ( 'NONE',  ( 9.999999999999998224, 0.000000000000000000, -52.99999999999996447 ) ) ;
#1390=VECTOR ( 'NONE', #16568, 1000.000000000000000 ) ;
#1391=CARTESIAN_POINT ( 'NONE',  ( 10.81189881249999729, 0.000000000000000000, -89.84375000204838102 ) ) ;
#1392=CARTESIAN_POINT ( 'NONE',  ( -2.121150477449813534E-15, -11.54700538379251284, -113.3749999999999858 ) ) ;
#1393=CARTESIAN_POINT ( 'NONE',  ( -10.81189881249999729, 1.324075727343319199E-15, -57.78125000204836681 ) ) ;
#1396=CARTESIAN_POINT ( 'NONE',  ( 10.81189881249999729, 0.000000000000000000, -115.5312500020483952 ) ) ;
#1397=CARTESIAN_POINT ( 'NONE',  ( 10.81189881249999729, 0.000000000000000000, -151.5312500020484094 ) ) ;
#1400=CARTESIAN_POINT ( 'NONE',  ( -9.999999999999998224, 5.773502691896259087, -126.2500000040967763 ) ) ;
#1402=VERTEX_POINT ( 'NONE', #9114 ) ;
#1406=CARTESIAN_POINT ( 'NONE',  ( -2.293366432827344421E-15, -12.48450537969573659, -181.9062500020483810 ) ) ;
#1407=ORIENTED_EDGE ( 'NONE', *, *, #13176, .T. ) ;
#1408=CARTESIAN_POINT ( 'NONE',  ( 5.000000000000000000, 8.660254037844385522, -51.24999999999996447 ) ) ;
#1410=CARTESIAN_POINT ( 'NONE',  ( 7.070501591499377789E-16, 11.54700538379251284, -57.50000000409677625 ) ) ;
#1411=CYLINDRICAL_SURFACE ( 'NONE', #40297, 9.999999999999998224 ) ;
#1413=DIRECTION ( 'NONE',  ( -0.000000000000000000, -0.000000000000000000, 1.000000000000000000 ) ) ;
#1415=CARTESIAN_POINT ( 'NONE',  ( -10.81189881249999729, 6.242252689847871849, -51.90625000204837391 ) ) ;
#1418=DIRECTION ( 'NONE',  ( 1.000000000000000000, 0.000000000000000000, 0.000000000000000000 ) ) ;
#1419=CARTESIAN_POINT ( 'NONE',  ( -5.405949406249996869, 9.363379034771805109, -178.0312500020483810 ) ) ;
#1421=EDGE_CURVE ( 'NONE', #4387, #32685, #21851, .T. ) ;
#1424=ADVANCED_FACE ( 'NONE', ( #11911 ), #22284, .T. ) ;
#1426=CARTESIAN_POINT ( 'NONE',  ( -5.405949406249996869, 9.363379034771805109, -89.53125000204838102 ) ) ;
#1428=SHAPE_REPRESENTATION_RELATIONSHIP ( 'NONE' , 'NONE' ,  #31964, #34104 ) ;
#1429=ORIENTED_EDGE ( 'NONE', *, *, #13096, .F. ) ;
#1431=ORIENTED_EDGE ( 'NONE', *, *, #16931, .T. ) ;
#1432=CARTESIAN_POINT ( 'NONE',  ( 10.81189881249999729, 0.000000000000000000, -37.34375000204836681 ) ) ;
#1433=CARTESIAN_POINT ( 'NONE',  ( -2.293366432827344421E-15, -12.48450537969573659, -25.71875000204837391 ) ) ;
#1434=CARTESIAN_POINT ( 'NONE',  ( -10.81189881249999907, -6.242252689847864744, -11.15625000204838457 ) ) ;
#1435=CARTESIAN_POINT ( 'NONE',  ( -5.405949406249996869, 9.363379034771805109, -63.84375000204836681 ) ) ;
#1436=CARTESIAN_POINT ( 'NONE',  ( 9.999999999999998224, 0.000000000000000000, -28.99999999999997158 ) ) ;
#1438=CARTESIAN_POINT ( 'NONE',  ( 5.405949406249992428, -9.363379034771808662, -183.0937500020483810 ) ) ;
#1441=FACE_OUTER_BOUND ( 'NONE', #10733, .T. ) ;
#1443=CARTESIAN_POINT ( 'NONE',  ( -2.121150477449813534E-15, -11.54700538379251284, -20.75000000409677980 ) ) ;
#1444=EDGE_CURVE ( 'NONE', #25484, #3061, #25619, .T. ) ;
#1445=CARTESIAN_POINT ( 'NONE',  ( 10.00000000000051159, -5.773502691895965988, -89.50000000409677625 ) ) ;
#1446=CARTESIAN_POINT ( 'NONE',  ( 7.644554776091147741E-16, 12.48450537969573659, -110.4687500020483668 ) ) ;
#1448=CARTESIAN_POINT ( 'NONE',  ( 10.81189881249999729, 0.000000000000000000, -84.03125000204838102 ) ) ;
#1449=CARTESIAN_POINT ( 'NONE',  ( -5.405949406250003975, -9.363379034771801557, -102.3437500020483810 ) ) ;
#1452=CARTESIAN_POINT ( 'NONE',  ( 9.999999999999996447, -5.773502691896262640, -154.0000000040968189 ) ) ;
#1454=( BOUNDED_CURVE ( )  B_SPLINE_CURVE ( 2, ( #8593, #18502, #15255, #21956, #5562, #18714, #31907 ),
 .UNSPECIFIED., .F., .F. ) 
 B_SPLINE_CURVE_WITH_KNOTS ( ( 3, 2, 2, 3 ),
 ( 0.03731343283582092690, 0.03855721393034829136, 0.03980099502487565583, 0.04104477611940302029 ),
 .UNSPECIFIED. ) 
 CURVE ( )  GEOMETRIC_REPRESENTATION_ITEM ( )  RATIONAL_B_SPLINE_CURVE ( ( 0.9999999999999963363, 0.8660254037844424824, 1.000000000000000000, 0.8660254037844387076, 1.000000000000000000, 0.8660254037844349329, 1.000000000000003775 ) ) 
 REPRESENTATION_ITEM ( '' )  );
#1458=CARTESIAN_POINT ( 'NONE',  ( -2.121150477449813534E-15, -11.54700538379251284, -174.8750000000000000 ) ) ;
#1459=DIRECTION ( 'NONE',  ( 1.000000000000000000, 0.000000000000000000, 0.000000000000000000 ) ) ;
#1462=CARTESIAN_POINT ( 'NONE',  ( -9.999999999999998224, 1.224646799147353059E-15, -73.24999999999998579 ) ) ;
#1464=CARTESIAN_POINT ( 'NONE',  ( 4.999999999999992006, -8.660254037844389075, -80.62500000409677625 ) ) ;
#1467=CARTESIAN_POINT ( 'NONE',  ( -2.293366432827344421E-15, -12.48450537969573659, -72.40625000204836681 ) ) ;
#1468=( BOUNDED_CURVE ( )  B_SPLINE_CURVE ( 2, ( #18781, #9276, #28730, #2815, #31970, #15947, #19412 ),
 .UNSPECIFIED., .F., .F. ) 
 B_SPLINE_CURVE_WITH_KNOTS ( ( 3, 2, 2, 3 ),
 ( 0.1156716417910447492, 0.1169154228855721483, 0.1181592039800995753, 0.1194029850746269744 ),
 .UNSPECIFIED. ) 
 CURVE ( )  GEOMETRIC_REPRESENTATION_ITEM ( )  RATIONAL_B_SPLINE_CURVE ( ( 1.000000000000003109, 0.8660254037844358210, 1.000000000000000000, 0.8660254037844387076, 1.000000000000000000, 0.8660254037844267172, 1.000000000000011990 ) ) 
 REPRESENTATION_ITEM ( '' )  );
#1470=CARTESIAN_POINT ( 'NONE',  ( 5.000000000000000000, 8.660254037844385522, -21.24999999999996447 ) ) ;
#1472=ORIENTED_EDGE ( 'NONE', *, *, #16310, .F. ) ;
#1473=CARTESIAN_POINT ( 'NONE',  ( -10.81189881249999729, 6.242252689847871849, -198.9062500020484094 ) ) ;
#1475=CARTESIAN_POINT ( 'NONE',  ( 5.405949406249999534, 9.363379034771803333, -10.09375000204834549 ) ) ;
#1476=CARTESIAN_POINT ( 'NONE',  ( -10.00000000000051337, 5.773502691895962435, -142.3750000000000000 ) ) ;
#1478=CARTESIAN_POINT ( 'NONE',  ( 7.644554776091147741E-16, 12.48450537969573659, -133.1562500020483810 ) ) ;
#1479=CARTESIAN_POINT ( 'NONE',  ( -4.999999999999996447, 8.660254037844387298, -180.0000000000000000 ) ) ;
#1480=FACE_OUTER_BOUND ( 'NONE', #34425, .T. ) ;
#1481=CARTESIAN_POINT ( 'NONE',  ( -10.81189881249999907, -6.242252689847864744, -113.1562500020483952 ) ) ;
#1483=CARTESIAN_POINT ( 'NONE',  ( -5.000000000000003553, -8.660254037844383745, -154.3750000040967905 ) ) ;
#1485=ORIENTED_EDGE ( 'NONE', *, *, #41503, .F. ) ;
#1486=CARTESIAN_POINT ( 'NONE',  ( 7.644554776091147741E-16, 12.48450537969573659, -35.65625000204835260 ) ) ;
#1490=ADVANCED_FACE ( 'NONE', ( #8269 ), #15358, .T. ) ;
#1491=CARTESIAN_POINT ( 'NONE',  ( -10.81189881249999729, 1.324075727343319199E-15, -84.59375000204836681 ) ) ;
#1492=CYLINDRICAL_SURFACE ( 'NONE', #13918, 9.999999999999998224 ) ;
#1493=DIRECTION ( 'NONE',  ( 1.000000000000000000, 0.000000000000000000, 0.000000000000000000 ) ) ;
#1494=CARTESIAN_POINT ( 'NONE',  ( 7.070501591499376803E-16, 11.54700538379251284, -170.0000000040967905 ) ) ;
#1496=CARTESIAN_POINT ( 'NONE',  ( -4.999999999999996447, 8.660254037844387298, -54.37500000409675494 ) ) ;
#1497=CARTESIAN_POINT ( 'NONE',  ( -10.81189881249999729, 6.242252689847871849, -123.7187500020483952 ) ) ;
#1500=CARTESIAN_POINT ( 'NONE',  ( -10.81189881249999729, -6.242252689847864744, -3.656250002048349046 ) ) ;
#1503=CARTESIAN_POINT ( 'NONE',  ( 4.999999999999992006, -8.660254037844389075, -181.1250000040967905 ) ) ;
#1505=CARTESIAN_POINT ( 'NONE',  ( -10.81189881249999729, 6.242252689847871849, -167.4062500020484094 ) ) ;
#1509=CARTESIAN_POINT ( 'NONE',  ( 10.81189881249999729, 6.242252689847867408, -53.71875000204838102 ) ) ;
#1511=CARTESIAN_POINT ( 'NONE',  ( -10.81189881249999729, 1.324075727343319199E-15, -12.78125000204835615 ) ) ;
#1513=CARTESIAN_POINT ( 'NONE',  ( 4.999999999999992006, -8.660254037844389075, -152.6250000040967905 ) ) ;
#1515=CARTESIAN_POINT ( 'NONE',  ( 4.999999999999992006, -8.660254037844389075, -93.74999999999998579 ) ) ;
#1517=CARTESIAN_POINT ( 'NONE',  ( 7.070501591499377789E-16, 11.54700538379251284, -110.0000000040968047 ) ) ;
#1518=CARTESIAN_POINT ( 'NONE',  ( -2.121150477449813534E-15, -11.54700538379251284, -49.25000000409676915 ) ) ;
#1521=CARTESIAN_POINT ( 'NONE',  ( 7.644554776091147741E-16, 12.48450537969573659, -100.1562500020483952 ) ) ;
#1525=CARTESIAN_POINT ( 'NONE',  ( 8.614196012143711556, -6.533971456633876684, 2.775557561562891351E-14 ) ) ;
#1526=CARTESIAN_POINT ( 'NONE',  ( 7.644554776091147741E-16, 12.48450537969573659, -166.1562500020483810 ) ) ;
#1529=CARTESIAN_POINT ( 'NONE',  ( 9.999999999999996447, -5.773502691896262640, -27.62499999999998579 ) ) ;
#1530=CARTESIAN_POINT ( 'NONE',  ( -5.405949406250003975, -9.363379034771801557, -24.53125000204836681 ) ) ;
#1531=CARTESIAN_POINT ( 'NONE',  ( 9.999999999999996447, -5.773502691896262640, -162.6250000000000284 ) ) ;
#1532=CARTESIAN_POINT ( 'NONE',  ( 10.00000000000051159, -5.773502691895965988, -102.6249999999999858 ) ) ;
#1534=CARTESIAN_POINT ( 'NONE',  ( 4.999999999999992006, -8.660254037844389075, -33.74999999999997158 ) ) ;
#1535=CARTESIAN_POINT ( 'NONE',  ( -5.405949406249996869, 9.363379034771805109, -130.0312500020484094 ) ) ;
#1536=CARTESIAN_POINT ( 'NONE',  ( 0.6477615133710965534, 10.23212146006973278, 1.249419088690773332E-14 ) ) ;
#1538=LINE ( 'NONE', #14672, #12785 ) ;
#1539=VERTEX_POINT ( 'NONE', #38464 ) ;
#1540=CARTESIAN_POINT ( 'NONE',  ( 10.81189881249999907, 6.242252689847868297, -59.90625000204838813 ) ) ;
#1542=VERTEX_POINT ( 'NONE', #8906 ) ;
#1546=CARTESIAN_POINT ( 'NONE',  ( 10.81189881249999551, -6.242252689847874514, -164.9687500020484094 ) ) ;
#1548=CARTESIAN_POINT ( 'NONE',  ( -10.81189881249999907, -6.242252689847864744, -16.96875000204836681 ) ) ;
#1549=DIRECTION ( 'NONE',  ( -0.000000000000000000, -0.000000000000000000, 1.000000000000000000 ) ) ;
#1550=CARTESIAN_POINT ( 'NONE',  ( -5.405949406249996869, 9.363379034771805109, -150.8437500020483810 ) ) ;
#1551=CARTESIAN_POINT ( 'NONE',  ( 7.644554776091147741E-16, 12.48450537969573659, -125.4687500020483952 ) ) ;
#1552=CARTESIAN_POINT ( 'NONE',  ( 7.644554776091147741E-16, 12.48450537969573659, -104.6562500020483810 ) ) ;
#1554=CARTESIAN_POINT ( 'NONE',  ( 7.070501591499376803E-16, 11.54700538379251284, -55.62499999999997158 ) ) ;
#1556=CARTESIAN_POINT ( 'NONE',  ( -5.405949406250003975, -9.363379034771801557, -4.843750002048369474 ) ) ;
#1559=CARTESIAN_POINT ( 'NONE',  ( -9.999999999998969713, -5.773502691896847949, -55.12499999999995737 ) ) ;
#1564=CARTESIAN_POINT ( 'NONE',  ( -10.81189881249999729, 6.242252689847871849, -74.21875000204836681 ) ) ;
#1565=CARTESIAN_POINT ( 'NONE',  ( -5.405949406250003975, -9.363379034771801557, -64.84375000204836681 ) ) ;
#1567=CARTESIAN_POINT ( 'NONE',  ( 10.81189881249999907, 6.242252689847868297, -32.90625000204835970 ) ) ;
#1571=CARTESIAN_POINT ( 'NONE',  ( -2.121150477449813534E-15, -11.54700538379251284, -123.8749999999999858 ) ) ;
#1572=CARTESIAN_POINT ( 'NONE',  ( -10.81189881249999729, 6.242252689847871849, -134.4062500020483810 ) ) ;
#1573=PLANE ( 'NONE',  #12756 ) ;
#1575=CARTESIAN_POINT ( 'NONE',  ( -5.405949406249996869, 9.363379034771805109, -11.53125000204835438 ) ) ;
#1579=CARTESIAN_POINT ( 'NONE',  ( 9.999999999999998224, 0.000000000000000000, -200.0000000000000000 ) ) ;
#1580=CARTESIAN_POINT ( 'NONE',  ( -2.121150477449813534E-15, -11.54700538379251284, -31.25000000409675494 ) ) ;
#1581=LINE ( 'NONE', #26150, #8392 ) ;
#1583=( BOUNDED_CURVE ( )  B_SPLINE_CURVE ( 2, ( #40246, #7044, #7248, #26260, #19765, #39409, #20398 ),
 .UNSPECIFIED., .F., .F. ) 
 B_SPLINE_CURVE_WITH_KNOTS ( ( 3, 2, 2, 3 ),
 ( 0.1716417910447761430, 0.1728855721393035005, 0.1741293532338308858, 0.1753731343283582433 ),
 .UNSPECIFIED. ) 
 CURVE ( )  GEOMETRIC_REPRESENTATION_ITEM ( )  RATIONAL_B_SPLINE_CURVE ( ( 0.9999999999999970024, 0.8660254037844417052, 1.000000000000000000, 0.8660254037844387076, 1.000000000000000000, 0.8660254037844357100, 1.000000000000003109 ) ) 
 REPRESENTATION_ITEM ( '' )  );
#1584=CARTESIAN_POINT ( 'NONE',  ( -10.00000000000051337, 5.773502691895962435, -146.8749999999999716 ) ) ;
#1585=CARTESIAN_POINT ( 'NONE',  ( 7.644554776091147741E-16, 12.48450537969573659, -151.1562500020484094 ) ) ;
#1586=EDGE_CURVE ( 'NONE', #5725, #17896, #277, .T. ) ;
#1587=CARTESIAN_POINT ( 'NONE',  ( -5.405949406250003975, -9.363379034771801557, -124.8437500020483810 ) ) ;
#1588=LINE ( 'NONE', #17524, #37896 ) ;
#1589=ORIENTED_EDGE ( 'NONE', *, *, #31560, .F. ) ;
#1590=LINE ( 'NONE', #23815, #20361 ) ;
#1592=ORIENTED_EDGE ( 'NONE', *, *, #14066, .T. ) ;
#1594=CARTESIAN_POINT ( 'NONE',  ( 5.000000000000000000, 8.660254037844385522, -189.2500000000000000 ) ) ;
#1595=CARTESIAN_POINT ( 'NONE',  ( 5.405949406249992428, -9.363379034771808662, -190.5937500020484094 ) ) ;
#1596=CARTESIAN_POINT ( 'NONE',  ( 10.81189881249999907, 6.242252689847868297, -41.71875000204835260 ) ) ;
#1597=CARTESIAN_POINT ( 'NONE',  ( -3.354946414818984479, -9.739129128211180486, 6.879861566379088064E-16 ) ) ;
#1598=CARTESIAN_POINT ( 'NONE',  ( 10.81189881249999551, -6.242252689847874514, -170.9687500020483810 ) ) ;
#1599=CARTESIAN_POINT ( 'NONE',  ( 5.405949406249999534, 9.363379034771803333, -151.0937500020483810 ) ) ;
#1600=CARTESIAN_POINT ( 'NONE',  ( 4.999999999999992006, -8.660254037844389075, -65.62500000409676204 ) ) ;
#1604=CARTESIAN_POINT ( 'NONE',  ( 7.070501591499376803E-16, 11.54700538379251284, -126.5000000040967763 ) ) ;
#1607=CARTESIAN_POINT ( 'NONE',  ( -5.405949406249996869, 9.363379034771805109, -86.34375000204836681 ) ) ;
#1608=CYLINDRICAL_SURFACE ( 'NONE', #42379, 9.999999999999998224 ) ;
#1609=CARTESIAN_POINT ( 'NONE',  ( 7.644554776091147741E-16, 12.48450537969573659, -58.15625000204838102 ) ) ;
#1610=FACE_OUTER_BOUND ( 'NONE', #15524, .T. ) ;
#1611=EDGE_CURVE ( 'NONE', #20180, #24638, #19344, .T. ) ;
#1613=CARTESIAN_POINT ( 'NONE',  ( -5.405949406249996869, 9.363379034771805109, -118.0312500020483952 ) ) ;
#1614=CARTESIAN_POINT ( 'NONE',  ( 7.644554776091147741E-16, 12.48450537969573659, -152.6562500020484094 ) ) ;
#1615=CARTESIAN_POINT ( 'NONE',  ( -9.999999999999998224, 1.224646799147353059E-15, -11.74999999999995559 ) ) ;
#1617=CARTESIAN_POINT ( 'NONE',  ( -5.000000000000003553, -8.660254037844383745, -133.3750000040967905 ) ) ;
#1622=DIRECTION ( 'NONE',  ( -0.000000000000000000, 1.000000000000000000, -0.000000000000000000 ) ) ;
#1623=CARTESIAN_POINT ( 'NONE',  ( 7.644554776091147741E-16, 12.48450537969573659, -179.6562500020484094 ) ) ;
#1626=CARTESIAN_POINT ( 'NONE',  ( -4.999999999999996447, 8.660254037844387298, -54.37500000409675494 ) ) ;
#1627=DIRECTION ( 'NONE',  ( 1.000000000000000000, 0.000000000000000000, 0.000000000000000000 ) ) ;
#1628=DIRECTION ( 'NONE',  ( -0.000000000000000000, -0.000000000000000000, 1.000000000000000000 ) ) ;
#1630=CARTESIAN_POINT ( 'NONE',  ( -5.405949406250003975, -9.363379034771801557, -51.53125000204835970 ) ) ;
#1633=CARTESIAN_POINT ( 'NONE',  ( -9.999999999999998224, 1.224646799147353059E-15, -192.1250000040967905 ) ) ;
#1634=CARTESIAN_POINT ( 'NONE',  ( 7.644554776091147741E-16, 12.48450537969573659, -176.6562500020484094 ) ) ;
#1635=LINE ( 'NONE', #30992, #16622 ) ;
#1638=CARTESIAN_POINT ( 'NONE',  ( 9.999999999999998224, 0.000000000000000000, -77.37500000409677625 ) ) ;
#1640=CARTESIAN_POINT ( 'NONE',  ( -9.999999999999998224, 1.224646799147353059E-15, -73.24999999999998579 ) ) ;
#1641=CARTESIAN_POINT ( 'NONE',  ( 10.81189881249999729, 0.000000000000000000, -87.03125000204838102 ) ) ;
#1642=ORIENTED_EDGE ( 'NONE', *, *, #20048, .F. ) ;
#1645=ORIENTED_EDGE ( 'NONE', *, *, #37760, .T. ) ;
#1646=CARTESIAN_POINT ( 'NONE',  ( -10.81189881249999729, -6.242252689847864744, -33.46875000204834549 ) ) ;
#1648=CARTESIAN_POINT ( 'NONE',  ( -10.81189881249999729, 1.324075727343319199E-15, -17.28125000204835970 ) ) ;
#1649=CARTESIAN_POINT ( 'NONE',  ( -10.81189881249999729, 6.242252689847871849, -60.71875000204838102 ) ) ;
#1651=CARTESIAN_POINT ( 'NONE',  ( 10.00000000000025402, -5.773502691896113426, -131.1250000000000000 ) ) ;
#1653=CARTESIAN_POINT ( 'NONE',  ( 5.405949406249999534, 9.363379034771803333, -182.5937500020483810 ) ) ;
#1656=CARTESIAN_POINT ( 'NONE',  ( -4.999999999999996447, 8.660254037844387298, -199.5000000000000000 ) ) ;
#1659=CARTESIAN_POINT ( 'NONE',  ( -5.405949406249996869, 9.363379034771805109, -114.8437500020483810 ) ) ;
#1661=CARTESIAN_POINT ( 'NONE',  ( -2.293366432827344421E-15, -12.48450537969573659, -85.90625000204839523 ) ) ;
#1662=EDGE_CURVE ( 'NONE', #4880, #35877, #28340, .T. ) ;
#1663=CARTESIAN_POINT ( 'NONE',  ( 10.81189881249999729, 6.242252689847867408, -95.71875000204838102 ) ) ;
#1668=CARTESIAN_POINT ( 'NONE',  ( -9.999999999999998224, 1.224646799147353059E-15, -151.6250000040967905 ) ) ;
#1670=EDGE_CURVE ( 'NONE', #32685, #13020, #6513, .T. ) ;
#1673=CARTESIAN_POINT ( 'NONE',  ( 10.00000000000154010, -5.773502691895370020, -13.00000000409671941 ) ) ;
#1674=FACE_OUTER_BOUND ( 'NONE', #527, .T. ) ;
#1676=CARTESIAN_POINT ( 'NONE',  ( -4.999999999999996447, 8.660254037844387298, -42.37500000409677625 ) ) ;
#1677=CARTESIAN_POINT ( 'NONE',  ( -9.999999999999998224, 1.224646799147353059E-15, -71.74999999999998579 ) ) ;
#1679=CARTESIAN_POINT ( 'NONE',  ( 5.000000000000000000, 8.660254037844385522, -78.62500000409677625 ) ) ;
#1682=CARTESIAN_POINT ( 'NONE',  ( -5.405949406250003975, -9.363379034771801557, -78.53125000204838102 ) ) ;
#1684=CARTESIAN_POINT ( 'NONE',  ( -10.00000000000051337, 5.773502691895962435, -112.7500000040967620 ) ) ;
#1687=CARTESIAN_POINT ( 'NONE',  ( 9.999999999999998224, 0.000000000000000000, -1.999999999999974021 ) ) ;
#1689=CARTESIAN_POINT ( 'NONE',  ( -5.405949406250003975, -9.363379034771801557, -13.84375000204834905 ) ) ;
#1690=CARTESIAN_POINT ( 'NONE',  ( -9.999999999999998224, 1.224646799147353059E-15, -13.62500000409674961 ) ) ;
#1691=EDGE_CURVE ( 'NONE', #31210, #317, #22583, .T. ) ;
#1693=CARTESIAN_POINT ( 'NONE',  ( -9.999999999999998224, 1.224646799147353059E-15, -196.2500000000000000 ) ) ;
#1694=CARTESIAN_POINT ( 'NONE',  ( 5.405949406249992428, -9.363379034771808662, -130.7812500020483810 ) ) ;
#1696=CARTESIAN_POINT ( 'NONE',  ( 10.00000000000000000, 5.773502691896255534, -184.8750000000000000 ) ) ;
#1697=CARTESIAN_POINT ( 'NONE',  ( -5.000000000000003553, -8.660254037844383745, -35.87500000409676915 ) ) ;
#1698=CARTESIAN_POINT ( 'NONE',  ( -5.405949406249996869, 9.363379034771805109, -112.0312500020483810 ) ) ;
#1700=DIRECTION ( 'NONE',  ( 1.000000000000000000, 0.000000000000000000, 0.000000000000000000 ) ) ;
#1701=EDGE_CURVE ( 'NONE', #8431, #29237, #19242, .T. ) ;
#1702=ORIENTED_EDGE ( 'NONE', *, *, #36445, .T. ) ;
#1705=CARTESIAN_POINT ( 'NONE',  ( -10.81189881249999729, 6.242252689847871849, -35.40625000204836681 ) ) ;
#1706=MECHANICAL_CONTEXT ( 'NONE', #34764, 'mechanical' ) ;
#1707=CARTESIAN_POINT ( 'NONE',  ( -10.81189881249999729, 1.324075727343319199E-15, -86.09375000204836681 ) ) ;
#1710=( BOUNDED_CURVE ( )  B_SPLINE_CURVE ( 2, ( #32609, #42082, #25707, #9284, #6060, #9500, #15955 ),
 .UNSPECIFIED., .F., .F. ) 
 B_SPLINE_CURVE_WITH_KNOTS ( ( 3, 2, 2, 3 ),
 ( 0.2574626865671643117, 0.2587064676616916414, 0.2599502487562190267, 0.2611940298507463565 ),
 .UNSPECIFIED. ) 
 CURVE ( )  GEOMETRIC_REPRESENTATION_ITEM ( )  RATIONAL_B_SPLINE_CURVE ( ( 0.9999999999999880096, 0.8660254037844506980, 1.000000000000000000, 0.8660254037844387076, 1.000000000000000000, 0.8660254037844267172, 1.000000000000011990 ) ) 
 REPRESENTATION_ITEM ( '' )  );
#1711=LINE ( 'NONE', #23570, #15010 ) ;
#1714=CARTESIAN_POINT ( 'NONE',  ( 7.644554776091147741E-16, 12.48450537969573659, -120.9687500020483952 ) ) ;
#1716=CARTESIAN_POINT ( 'NONE',  ( -9.999999999999998224, 1.224646799147353059E-15, -166.6250000040967905 ) ) ;
#1719=CARTESIAN_POINT ( 'NONE',  ( 9.999999999999996447, -5.773502691896262640, -181.0000000040968189 ) ) ;
#1720=CARTESIAN_POINT ( 'NONE',  ( 10.81189881249999551, -6.242252689847874514, -168.1562500020484094 ) ) ;
#1723=LINE ( 'NONE', #15488, #13715 ) ;
#1726=CARTESIAN_POINT ( 'NONE',  ( -2.293366432827344421E-15, -12.48450537969573659, -51.21875000204836681 ) ) ;
#1729=CARTESIAN_POINT ( 'NONE',  ( 5.405949406249999534, 9.363379034771803333, -8.781250002048352599 ) ) ;
#1731=CARTESIAN_POINT ( 'NONE',  ( -9.999999999999998224, 1.224646799147353059E-15, -91.24999999999998579 ) ) ;
#1733=CARTESIAN_POINT ( 'NONE',  ( 9.999999999999996447, -5.773502691896262640, -101.1250000000000000 ) ) ;
#1735=CARTESIAN_POINT ( 'NONE',  ( 4.999999999999992006, -8.660254037844389075, -107.6250000040967763 ) ) ;
#1736=FACE_OUTER_BOUND ( 'NONE', #34180, .T. ) ;
#1739=CARTESIAN_POINT ( 'NONE',  ( -2.293366432827344421E-15, -12.48450537969573659, -100.9062500020483952 ) ) ;
#1740=ORIENTED_EDGE ( 'NONE', *, *, #6099, .T. ) ;
#1742=CARTESIAN_POINT ( 'NONE',  ( 9.999999999999998224, 0.000000000000000000, -165.8750000040967905 ) ) ;
#1743=CARTESIAN_POINT ( 'NONE',  ( 10.81189881249999729, 0.000000000000000000, -156.0312500020484094 ) ) ;
#1746=CARTESIAN_POINT ( 'NONE',  ( -4.999999999999996447, 8.660254037844387298, -28.49999999999997158 ) ) ;
#1747=CARTESIAN_POINT ( 'NONE',  ( 10.81189881249999729, 6.242252689847867408, -31.40625000204834905 ) ) ;
#1748=CARTESIAN_POINT ( 'NONE',  ( 4.999999999999992006, -8.660254037844389075, -164.2500000000000000 ) ) ;
#1749=CYLINDRICAL_SURFACE ( 'NONE', #11124, 9.999999999999998224 ) ;
#1752=CARTESIAN_POINT ( 'NONE',  ( 9.999999999999998224, 0.000000000000000000, -33.49999999999997158 ) ) ;
#1753=CARTESIAN_POINT ( 'NONE',  ( 5.405949406249992428, -9.363379034771808662, -136.7812500020483810 ) ) ;
#1754=CARTESIAN_POINT ( 'NONE',  ( 8.934005281565452705, 5.771751285519217234, -7.741086494507744060E-15 ) ) ;
#1755=CARTESIAN_POINT ( 'NONE',  ( -9.999999999999479527, -5.773502691896549521, -69.00000000409677625 ) ) ;
#1757=CARTESIAN_POINT ( 'NONE',  ( 5.405949406249999534, 9.363379034771803333, -59.78125000204836681 ) ) ;
#1759=ORIENTED_EDGE ( 'NONE', *, *, #41440, .T. ) ;
#1760=VERTEX_POINT ( 'NONE', #10162 ) ;
#1761=DIRECTION ( 'NONE',  ( -0.000000000000000000, -0.000000000000000000, 1.000000000000000000 ) ) ;
#1762=CARTESIAN_POINT ( 'NONE',  ( 5.405949406249999534, 9.363379034771803333, -158.5937500020483810 ) ) ;
#1765=CARTESIAN_POINT ( 'NONE',  ( -10.81189881249999729, 1.324075727343319199E-15, -8.093750002048343717 ) ) ;
#1766=DIRECTION ( 'NONE',  ( -0.000000000000000000, -0.000000000000000000, 1.000000000000000000 ) ) ;
#1767=CARTESIAN_POINT ( 'NONE',  ( -2.293366432827344421E-15, -12.48450537969573659, -147.2187500020484094 ) ) ;
#1768=CARTESIAN_POINT ( 'NONE',  ( -10.81189881249999907, -6.242252689847864744, -104.1562500020483668 ) ) ;
#1771=CARTESIAN_POINT ( 'NONE',  ( 5.405949406249999534, 9.363379034771803333, -2.593750002048367254 ) ) ;
#1773=CARTESIAN_POINT ( 'NONE',  ( 5.405949406249999534, 9.363379034771803333, -194.7812500020484094 ) ) ;
#1774=CARTESIAN_POINT ( 'NONE',  ( 9.999999999999998224, 0.000000000000000000, -200.0000000000000000 ) ) ;
#1777=CARTESIAN_POINT ( 'NONE',  ( -10.81189881249999729, 1.324075727343319199E-15, -75.59375000204838102 ) ) ;
#1778=CARTESIAN_POINT ( 'NONE',  ( -10.81189881249999907, -6.242252689847864744, -60.46875000204838102 ) ) ;
#1780=CARTESIAN_POINT ( 'NONE',  ( -5.405949406250003975, -9.363379034771801557, -33.53125000204837391 ) ) ;
#1784=CARTESIAN_POINT ( 'NONE',  ( 9.999999999999998224, 0.000000000000000000, -125.0000000000000000 ) ) ;
#1788=CARTESIAN_POINT ( 'NONE',  ( 10.81189881249999551, -6.242252689847874514, -10.65625000204838280 ) ) ;
#1792=DIRECTION ( 'NONE',  ( 1.000000000000000000, 0.000000000000000000, 0.000000000000000000 ) ) ;
#1794=ADVANCED_FACE ( 'NONE', ( #19875 ), #16405, .T. ) ;
#1795=CARTESIAN_POINT ( 'NONE',  ( -9.999999999999998224, 5.773502691896259087, -37.75000000409676204 ) ) ;
#1796=VECTOR ( 'NONE', #15573, 1000.000000000000000 ) ;
#1798=CYLINDRICAL_SURFACE ( 'NONE', #42121, 9.999999999999998224 ) ;
#1801=CARTESIAN_POINT ( 'NONE',  ( 5.405949406249992428, -9.363379034771808662, -147.2812500020483810 ) ) ;
#1802=CARTESIAN_POINT ( 'NONE',  ( -10.81189881249999907, -6.242252689847864744, -123.4687500020483810 ) ) ;
#1805=ORIENTED_EDGE ( 'NONE', *, *, #14608, .F. ) ;
#1806=EDGE_CURVE ( 'NONE', #22821, #35538, #264, .T. ) ;
#1808=ORIENTED_EDGE ( 'NONE', *, *, #29272, .F. ) ;
#1811=CARTESIAN_POINT ( 'NONE',  ( -5.405949406249996869, 9.363379034771805109, -182.3437500020483810 ) ) ;
#1812=CARTESIAN_POINT ( 'NONE',  ( 10.81189881249999907, 6.242252689847868297, -38.71875000204835260 ) ) ;
#1813=CARTESIAN_POINT ( 'NONE',  ( 7.070501591499376803E-16, 11.54700538379251284, -118.6250000000000142 ) ) ;
#1814=CARTESIAN_POINT ( 'NONE',  ( -10.81189881249999729, 1.324075727343319199E-15, -173.0937500020484094 ) ) ;
#1816=CARTESIAN_POINT ( 'NONE',  ( -5.405949406249996869, 9.363379034771805109, -156.8437500020483810 ) ) ;
#1817=CARTESIAN_POINT ( 'NONE',  ( -9.999999999999998224, 1.224646799147353059E-15, -123.1250000040967905 ) ) ;
#1821=CARTESIAN_POINT ( 'NONE',  ( -9.999999999999998224, 1.224646799147353059E-15, -134.7499999999999716 ) ) ;
#1822=CARTESIAN_POINT ( 'NONE',  ( 9.999999999999998224, 0.000000000000000000, -177.8750000040967905 ) ) ;
#1824=CARTESIAN_POINT ( 'NONE',  ( -5.405949406249996869, 9.363379034771805109, -81.84375000204838102 ) ) ;
#1825=CARTESIAN_POINT ( 'NONE',  ( 10.81189881249999907, 6.242252689847868297, -56.90625000204837391 ) ) ;
#1828=CARTESIAN_POINT ( 'NONE',  ( 7.644554776091147741E-16, 12.48450537969573659, -110.6562500020483952 ) ) ;
#1829=CARTESIAN_POINT ( 'NONE',  ( 5.405949406249992428, -9.363379034771808662, -156.2812500020484094 ) ) ;
#1830=CARTESIAN_POINT ( 'NONE',  ( 5.000000000000000000, 8.660254037844385522, -15.62500000409675138 ) ) ;
#1832=CARTESIAN_POINT ( 'NONE',  ( -4.999999999999996447, 8.660254037844387298, -132.3750000040967905 ) ) ;
#1834=( BOUNDED_CURVE ( )  B_SPLINE_CURVE ( 2, ( #17768, #11077, #4194, #40015, #10445, #23637, #33560 ),
 .UNSPECIFIED., .F., .F. ) 
 B_SPLINE_CURVE_WITH_KNOTS ( ( 3, 2, 2, 3 ),
 ( 0.5037313432835821558, 0.5049751243781095411, 0.5062189054726369264, 0.5074626865671643117 ),
 .UNSPECIFIED. ) 
 CURVE ( )  GEOMETRIC_REPRESENTATION_ITEM ( )  RATIONAL_B_SPLINE_CURVE ( ( 0.9999999999999880096, 0.8660254037844506980, 1.000000000000000000, 0.8660254037844387076, 1.000000000000000000, 0.8660254037844267172, 1.000000000000011990 ) ) 
 REPRESENTATION_ITEM ( '' )  );
#1836=ORIENTED_EDGE ( 'NONE', *, *, #19334, .F. ) ;
#1840=CARTESIAN_POINT ( 'NONE',  ( 10.81189881249999551, -6.242252689847874514, -178.6562500020484094 ) ) ;
#1841=VERTEX_POINT ( 'NONE', #25739 ) ;
#1843=CARTESIAN_POINT ( 'NONE',  ( -2.121150477449813534E-15, -11.54700538379251284, -61.25000000409677625 ) ) ;
#1845=CARTESIAN_POINT ( 'NONE',  ( 9.999999999999742428, 5.773502691896404748, -130.8749999999999716 ) ) ;
#1851=CARTESIAN_POINT ( 'NONE',  ( -5.405949406250003975, -9.363379034771801557, -165.5312500020484094 ) ) ;
#1852=CARTESIAN_POINT ( 'NONE',  ( 9.999999999997939426, 5.773502691897446581, -7.874999999999921840 ) ) ;
#1853=FACE_OUTER_BOUND ( 'NONE', #36551, .T. ) ;
#1854=EDGE_CURVE ( 'NONE', #24638, #18719, #14148, .T. ) ;
#1855=ORIENTED_EDGE ( 'NONE', *, *, #6433, .T. ) ;
#1856=CARTESIAN_POINT ( 'NONE',  ( 7.070501591499376803E-16, 11.54700538379251284, -84.50000000409677625 ) ) ;
#1857=CARTESIAN_POINT ( 'NONE',  ( -2.121150477449813534E-15, -11.54700538379251284, -153.8749999999999716 ) ) ;
#1858=CARTESIAN_POINT ( 'NONE',  ( -9.999999999999998224, 1.224646799147353059E-15, -163.6250000040967905 ) ) ;
#1859=CARTESIAN_POINT ( 'NONE',  ( 5.405949406249999534, 9.363379034771803333, -79.28125000204838102 ) ) ;
#1863=ORIENTED_EDGE ( 'NONE', *, *, #34252, .F. ) ;
#1865=CARTESIAN_POINT ( 'NONE',  ( -10.81189881249999729, 1.324075727343319199E-15, -38.09375000204837391 ) ) ;
#1867=CARTESIAN_POINT ( 'NONE',  ( 5.405949406249992428, -9.363379034771808662, -6.281250002048377468 ) ) ;
#1868=CARTESIAN_POINT ( 'NONE',  ( -10.81189881249999907, -6.242252689847864744, -60.46875000204838102 ) ) ;
#1869=ORIENTED_EDGE ( 'NONE', *, *, #25929, .F. ) ;
#1872=CARTESIAN_POINT ( 'NONE',  ( 5.405949406249999534, 9.363379034771803333, -197.5937500020484094 ) ) ;
#1873=CARTESIAN_POINT ( 'NONE',  ( 7.644554776091147741E-16, 12.48450537969573659, -180.9687500020484094 ) ) ;
#1876=CARTESIAN_POINT ( 'NONE',  ( 10.00000000000000000, 5.773502691896255534, -199.8750000000000284 ) ) ;
#1878=CARTESIAN_POINT ( 'NONE',  ( 10.81189881249999729, 0.000000000000000000, -113.8437500020483810 ) ) ;
#1879=FACE_OUTER_BOUND ( 'NONE', #40938, .T. ) ;
#1880=CARTESIAN_POINT ( 'NONE',  ( -5.405949406250003975, -9.363379034771801557, -83.03125000204838102 ) ) ;
#1881=CARTESIAN_POINT ( 'NONE',  ( -2.293366432827344421E-15, -12.48450537969573659, -93.21875000204838102 ) ) ;
#1883=CARTESIAN_POINT ( 'NONE',  ( -9.999999999999998224, 1.224646799147353059E-15, -153.1250000040967905 ) ) ;
#1887=CARTESIAN_POINT ( 'NONE',  ( -9.999999999999479527, -5.773502691896549521, -40.12499999999995026 ) ) ;
#1891=CARTESIAN_POINT ( 'NONE',  ( 9.999999999999998224, 0.000000000000000000, -69.49999999999997158 ) ) ;
#1893=CARTESIAN_POINT ( 'NONE',  ( -5.000000000000003553, -8.660254037844383745, -85.37500000409677625 ) ) ;
#1896=CARTESIAN_POINT ( 'NONE',  ( 10.81189881249999729, 6.242252689847867408, -76.40625000204836681 ) ) ;
#1900=ORIENTED_EDGE ( 'NONE', *, *, #36380, .T. ) ;
#1901=CARTESIAN_POINT ( 'NONE',  ( -2.293366432827344421E-15, -12.48450537969573659, -198.4062500020484094 ) ) ;
#1903=CARTESIAN_POINT ( 'NONE',  ( -10.81189881249999729, 6.242252689847871849, -3.718750002048365477 ) ) ;
#1904=CARTESIAN_POINT ( 'NONE',  ( -5.000000000000003553, -8.660254037844383745, -64.37500000409676204 ) ) ;
#1905=CARTESIAN_POINT ( 'NONE',  ( 5.405949406249992428, -9.363379034771808662, -139.5937500020483810 ) ) ;
#1906=CARTESIAN_POINT ( 'NONE',  ( 10.00000000000076916, -5.773502691895816774, -107.5000000040967620 ) ) ;
#1907=CARTESIAN_POINT ( 'NONE',  ( 9.999999999999998224, 0.000000000000000000, -200.0000000000000000 ) ) ;
#1908=CARTESIAN_POINT ( 'NONE',  ( -5.405949406249996869, 9.363379034771805109, -128.5312500020484094 ) ) ;
#1909=CARTESIAN_POINT ( 'NONE',  ( 10.00000000000000000, 5.773502691896255534, -181.8750000000000000 ) ) ;
#1910=CARTESIAN_POINT ( 'NONE',  ( 5.000000000000000000, 8.660254037844385522, -176.1250000040968189 ) ) ;
#1911=CARTESIAN_POINT ( 'NONE',  ( -10.81189881249999729, 1.324075727343319199E-15, -98.28125000204839523 ) ) ;
#1912=ORIENTED_EDGE ( 'NONE', *, *, #2506, .T. ) ;
#1916=EDGE_CURVE ( 'NONE', #32801, #14436, #26787, .T. ) ;
#1918=CARTESIAN_POINT ( 'NONE',  ( 10.81189881249999551, -6.242252689847874514, -37.65625000204836681 ) ) ;
#1920=CARTESIAN_POINT ( 'NONE',  ( 10.81189881249999729, 0.000000000000000000, -83.84375000204836681 ) ) ;
#1921=CARTESIAN_POINT ( 'NONE',  ( 5.000000000000000000, 8.660254037844385522, -128.1250000040967620 ) ) ;
#1922=AXIS2_PLACEMENT_3D ( 'NONE', #7273, #40268, #30377 ) ;
#1923=DIRECTION ( 'NONE',  ( 1.000000000000000000, 0.000000000000000000, 0.000000000000000000 ) ) ;
#1924=( BOUNDED_CURVE ( )  B_SPLINE_CURVE ( 2, ( #23390, #306, #9366, #16881, #19709, #35915, #13425 ),
 .UNSPECIFIED., .F., .F. ) 
 B_SPLINE_CURVE_WITH_KNOTS ( ( 3, 2, 2, 3 ),
 ( 0.6268656716417911889, 0.6281094527363185742, 0.6293532338308458485, 0.6305970149253732338 ),
 .UNSPECIFIED. ) 
 CURVE ( )  GEOMETRIC_REPRESENTATION_ITEM ( )  RATIONAL_B_SPLINE_CURVE ( ( 0.9999999999999880096, 0.8660254037844506980, 1.000000000000000000, 0.8660254037844387076, 1.000000000000000000, 0.8660254037844267172, 1.000000000000011990 ) ) 
 REPRESENTATION_ITEM ( '' )  );
#1925=CARTESIAN_POINT ( 'NONE',  ( 4.999999999999992006, -8.660254037844389075, -32.62500000409676915 ) ) ;
#1928=CARTESIAN_POINT ( 'NONE',  ( -10.81189881249999729, -6.242252689847864744, -115.9687500020483810 ) ) ;
#1933=CARTESIAN_POINT ( 'NONE',  ( 4.999999999999992006, -8.660254037844389075, -175.1250000040968189 ) ) ;
#1934=CARTESIAN_POINT ( 'NONE',  ( -10.81189881249999729, 1.324075727343319199E-15, -167.2812500020484094 ) ) ;
#1935=CARTESIAN_POINT ( 'NONE',  ( 5.000000000000000000, 8.660254037844385522, -102.6250000040967905 ) ) ;
#1938=CARTESIAN_POINT ( 'NONE',  ( 10.81189881249999729, 0.000000000000000000, -43.34375000204837391 ) ) ;
#1940=CARTESIAN_POINT ( 'NONE',  ( 5.405949406249992428, -9.363379034771808662, -6.281250002048377468 ) ) ;
#1942=CARTESIAN_POINT ( 'NONE',  ( -9.999999999999998224, 1.224646799147353059E-15, -53.74999999999996447 ) ) ;
#1944=CARTESIAN_POINT ( 'NONE',  ( 7.070501591499377789E-16, 11.54700538379251284, -99.12500000000000000 ) ) ;
#1946=CARTESIAN_POINT ( 'NONE',  ( -9.999999999999998224, 5.773502691896259087, -102.2500000040967763 ) ) ;
#1947=CARTESIAN_POINT ( 'NONE',  ( -4.999999999999996447, 8.660254037844387298, -82.49999999999998579 ) ) ;
#1950=CARTESIAN_POINT ( 'NONE',  ( 5.405949406249992428, -9.363379034771808662, -99.28125000204839523 ) ) ;
#1951=ORIENTED_EDGE ( 'NONE', *, *, #16415, .F. ) ;
#1953=CARTESIAN_POINT ( 'NONE',  ( -9.999999999999998224, 1.224646799147353059E-15, -55.24999999999996447 ) ) ;
#1954=CARTESIAN_POINT ( 'NONE',  ( -5.405949406249996869, 9.363379034771805109, -160.0312500020484094 ) ) ;
#1956=ORIENTED_EDGE ( 'NONE', *, *, #19624, .F. ) ;
#1957=CARTESIAN_POINT ( 'NONE',  ( 5.000000000000000000, 8.660254037844385522, -24.24999999999996447 ) ) ;
#1958=CARTESIAN_POINT ( 'NONE',  ( -5.405949406250003975, -9.363379034771801557, -26.03125000204836681 ) ) ;
#1959=CARTESIAN_POINT ( 'NONE',  ( -2.121150477449813534E-15, -11.54700538379251284, -161.3750000000000000 ) ) ;
#1962=CARTESIAN_POINT ( 'NONE',  ( -9.999999999999479527, -5.773502691896549521, -81.00000000409674783 ) ) ;
#1963=CARTESIAN_POINT ( 'NONE',  ( -2.293366432827344421E-15, -12.48450537969573659, -132.4062500020483810 ) ) ;
#1964=FACE_OUTER_BOUND ( 'NONE', #28728, .T. ) ;
#1967=VERTEX_POINT ( 'NONE', #17262 ) ;
#1968=EDGE_CURVE ( 'NONE', #25274, #27810, #13476, .T. ) ;
#1969=( BOUNDED_CURVE ( )  B_SPLINE_CURVE ( 2, ( #14952, #28150, #24707, #41284, #11723, #4620, #30960 ),
 .UNSPECIFIED., .F., .F. ) 
 B_SPLINE_CURVE_WITH_KNOTS ( ( 3, 2, 2, 3 ),
 ( 0.3171641791044778058, 0.3184079601990050801, 0.3196517412935324653, 0.3208955223880597396 ),
 .UNSPECIFIED. ) 
 CURVE ( )  GEOMETRIC_REPRESENTATION_ITEM ( )  RATIONAL_B_SPLINE_CURVE ( ( 0.9999999999999820144, 0.8660254037844566932, 1.000000000000000000, 0.8660254037844387076, 1.000000000000000000, 0.8660254037844327124, 1.000000000000005995 ) ) 
 REPRESENTATION_ITEM ( '' )  );
#1970=CARTESIAN_POINT ( 'NONE',  ( -10.81189881249999729, 6.242252689847871849, -59.40625000204838813 ) ) ;
#1972=EDGE_CURVE ( 'NONE', #24961, #41628, #30250, .T. ) ;
#1974=ORIENTED_EDGE ( 'NONE', *, *, #5249, .F. ) ;
#1975=CARTESIAN_POINT ( 'NONE',  ( -2.121150477449813534E-15, -11.54700538379251284, -46.25000000409676915 ) ) ;
#1977=CARTESIAN_POINT ( 'NONE',  ( -9.999999999999998224, 1.224646799147353059E-15, -200.0000000000000000 ) ) ;
#1978=CARTESIAN_POINT ( 'NONE',  ( -2.293366432827344421E-15, -12.48450537969573659, -154.7187500020483810 ) ) ;
#1981=CARTESIAN_POINT ( 'NONE',  ( -5.405949406250003975, -9.363379034771801557, -10.84375000204834727 ) ) ;
#1982=CARTESIAN_POINT ( 'NONE',  ( -10.81189881249999729, -6.242252689847864744, -138.4687500020483810 ) ) ;
#1983=CARTESIAN_POINT ( 'NONE',  ( -5.405949406249996869, 9.363379034771805109, -97.03125000204839523 ) ) ;
#1985=CARTESIAN_POINT ( 'NONE',  ( 9.999999999999998224, 0.000000000000000000, -180.8750000040967905 ) ) ;
#1987=CARTESIAN_POINT ( 'NONE',  ( 5.405949406249999534, 9.363379034771803333, -1.093750002048365921 ) ) ;
#1989=CARTESIAN_POINT ( 'NONE',  ( -5.405949406250003975, -9.363379034771801557, -195.5312500020484094 ) ) ;
#1990=CARTESIAN_POINT ( 'NONE',  ( 0.000000000000000000, 0.000000000000000000, -200.0000000000000000 ) ) ;
#1993=EDGE_CURVE ( 'NONE', #5068, #24022, #30032, .T. ) ;
#1994=CARTESIAN_POINT ( 'NONE',  ( 10.81189881249999729, 6.242252689847867408, -73.21875000204836681 ) ) ;
#1995=CARTESIAN_POINT ( 'NONE',  ( -5.405949406249996869, 9.363379034771805109, -56.34375000204835970 ) ) ;
#1997=CARTESIAN_POINT ( 'NONE',  ( 5.405949406249992428, -9.363379034771808662, -22.78125000204836326 ) ) ;
#2000=CARTESIAN_POINT ( 'NONE',  ( -4.999999999999996447, 8.660254037844387298, -124.5000000000000000 ) ) ;
#2004=CARTESIAN_POINT ( 'NONE',  ( 10.81189881249999729, 0.000000000000000000, -9.031250002048352599 ) ) ;
#2005=ORIENTED_EDGE ( 'NONE', *, *, #26483, .T. ) ;
#2010=CARTESIAN_POINT ( 'NONE',  ( 5.000000000000000000, 8.660254037844385522, -29.12500000409676204 ) ) ;
#2011=LINE ( 'NONE', #18170, #26980 ) ;
#2014=CARTESIAN_POINT ( 'NONE',  ( -10.81189881249999729, 6.242252689847871849, -143.4062500020484094 ) ) ;
#2015=CARTESIAN_POINT ( 'NONE',  ( 5.405949406249992428, -9.363379034771808662, -127.5937500020483668 ) ) ;
#2016=CARTESIAN_POINT ( 'NONE',  ( -9.999999999999998224, 1.224646799147353059E-15, -14.74999999999995737 ) ) ;
#2018=DIRECTION ( 'NONE',  ( -0.000000000000000000, -0.000000000000000000, 1.000000000000000000 ) ) ;
#2019=VERTEX_POINT ( 'NONE', #31473 ) ;
#2020=AXIS2_PLACEMENT_3D ( 'NONE', #5758, #34905, #15016 ) ;
#2021=ORIENTED_EDGE ( 'NONE', *, *, #14598, .T. ) ;
#2022=EDGE_LOOP ( 'NONE', ( #31999, #38521, #40889, #7106 ) ) ;
#2024=CARTESIAN_POINT ( 'NONE',  ( -5.405949406250003975, -9.363379034771801557, -183.3437500020483810 ) ) ;
#2025=CARTESIAN_POINT ( 'NONE',  ( 10.81189881249999907, 6.242252689847868297, -32.71875000204834549 ) ) ;
#2027=CARTESIAN_POINT ( 'NONE',  ( 9.999999999999998224, 0.000000000000000000, -90.49999999999998579 ) ) ;
#2028=CARTESIAN_POINT ( 'NONE',  ( -5.405949406250003975, -9.363379034771801557, -172.8437500020484094 ) ) ;
#2029=CARTESIAN_POINT ( 'NONE',  ( 10.81189881249999729, 0.000000000000000000, -149.8437500020483810 ) ) ;
#2030=CARTESIAN_POINT ( 'NONE',  ( 0.000000000000000000, 0.000000000000000000, -200.0000000000000000 ) ) ;
#2034=CARTESIAN_POINT ( 'NONE',  ( 0.000000000000000000, 0.000000000000000000, -200.0000000000000000 ) ) ;
#2035=CARTESIAN_POINT ( 'NONE',  ( 5.000000000000000000, 8.660254037844385522, -70.74999999999998579 ) ) ;
#2037=CARTESIAN_POINT ( 'NONE',  ( -5.405949406249996869, 9.363379034771805109, -80.34375000204838102 ) ) ;
#2038=CARTESIAN_POINT ( 'NONE',  ( 9.999999999999998224, 0.000000000000000000, -112.9999999999999858 ) ) ;
#2039=CARTESIAN_POINT ( 'NONE',  ( 5.405949406249992428, -9.363379034771808662, -60.28125000204836681 ) ) ;
#2040=CYLINDRICAL_SURFACE ( 'NONE', #21999, 9.999999999999998224 ) ;
#2042=CARTESIAN_POINT ( 'NONE',  ( 5.405949406249992428, -9.363379034771808662, -115.7812500020483952 ) ) ;
#2043=CARTESIAN_POINT ( 'NONE',  ( -10.81189881249999729, -6.242252689847864744, -144.6562500020484094 ) ) ;
#2047=CARTESIAN_POINT ( 'NONE',  ( -5.000000000000003553, -8.660254037844383745, -119.8750000040967905 ) ) ;
#2049=EDGE_LOOP ( 'NONE', ( #3538, #34072, #39048, #41696 ) ) ;
#2052=CARTESIAN_POINT ( 'NONE',  ( 5.000000000000000000, 8.660254037844385522, -68.12500000409677625 ) ) ;
#2053=AXIS2_PLACEMENT_3D ( 'NONE', #3803, #16942, #30139 ) ;
#2054=CARTESIAN_POINT ( 'NONE',  ( -5.405949406249996869, 9.363379034771805109, -179.5312500020483810 ) ) ;
#2055=EDGE_LOOP ( 'NONE', ( #1805, #11917, #19083, #26416 ) ) ;
#2057=CARTESIAN_POINT ( 'NONE',  ( 9.999999999999996447, -5.773502691896262640, -47.50000000409677625 ) ) ;
#2058=CARTESIAN_POINT ( 'NONE',  ( 10.00000000000102318, -5.773502691895667560, -18.62499999999994671 ) ) ;
#2062=AXIS2_PLACEMENT_3D ( 'NONE', #513, #3519, #33313 ) ;
#2064=DIRECTION ( 'NONE',  ( -0.000000000000000000, -0.000000000000000000, 1.000000000000000000 ) ) ;
#2065=CARTESIAN_POINT ( 'NONE',  ( -2.293366432827344421E-15, -12.48450537969573659, -172.9062500020484379 ) ) ;
#2066=DIRECTION ( 'NONE',  ( 1.000000000000000000, 0.000000000000000000, 0.000000000000000000 ) ) ;
#2069=CARTESIAN_POINT ( 'NONE',  ( -9.999999999999998224, 1.224646799147353059E-15, -84.12500000409677625 ) ) ;
#2070=CARTESIAN_POINT ( 'NONE',  ( -4.999999999999996447, 8.660254037844387298, -123.3750000040967905 ) ) ;
#2071=CARTESIAN_POINT ( 'NONE',  ( 9.999999999998969713, 5.773502691896851502, -39.75000000409674072 ) ) ;
#2072=CARTESIAN_POINT ( 'NONE',  ( -10.81189881249999729, 1.324075727343319199E-15, -78.78125000204838102 ) ) ;
#2074=CARTESIAN_POINT ( 'NONE',  ( 9.999999999999998224, 0.000000000000000000, -119.0000000000000000 ) ) ;
#2075=EDGE_LOOP ( 'NONE', ( #25697, #38619, #32120, #34720 ) ) ;
#2076=ORIENTED_EDGE ( 'NONE', *, *, #15327, .F. ) ;
#2077=CARTESIAN_POINT ( 'NONE',  ( -2.293366432827344421E-15, -12.48450537969573659, -25.71875000204837391 ) ) ;
#2079=CARTESIAN_POINT ( 'NONE',  ( 10.81189881249999551, -6.242252689847874514, -9.156250002048375691 ) ) ;
#2081=CARTESIAN_POINT ( 'NONE',  ( -5.405949406249996869, 9.363379034771805109, -54.84375000204835970 ) ) ;
#2082=VERTEX_POINT ( 'NONE', #36919 ) ;
#2083=CARTESIAN_POINT ( 'NONE',  ( 18.76388374866293773, 2.499999999999956923, 49.99999999999998579 ) ) ;
#2085=CARTESIAN_POINT ( 'NONE',  ( -2.293366432827344421E-15, -12.48450537969573659, -195.2187500020484094 ) ) ;
#2086=CARTESIAN_POINT ( 'NONE',  ( -10.81189881249999907, -6.242252689847864744, -178.9687500020484094 ) ) ;
#2088=( BOUNDED_CURVE ( )  B_SPLINE_CURVE ( 2, ( #35542, #12841, #5972, #35118, #19123, #38548, #32308 ),
 .UNSPECIFIED., .F., .F. ) 
 B_SPLINE_CURVE_WITH_KNOTS ( ( 3, 2, 2, 3 ),
 ( 0.7350746268656719318, 0.7363184079601993171, 0.7375621890547265913, 0.7388059701492539766 ),
 .UNSPECIFIED. ) 
 CURVE ( )  GEOMETRIC_REPRESENTATION_ITEM ( )  RATIONAL_B_SPLINE_CURVE ( ( 0.9999999999999641398, 0.8660254037844745678, 1.000000000000000000, 0.8660254037844387076, 1.000000000000000000, 0.8660254037844148378, 1.000000000000023981 ) ) 
 REPRESENTATION_ITEM ( '' )  );
#2090=DIRECTION ( 'NONE',  ( -0.000000000000000000, -0.000000000000000000, 1.000000000000000000 ) ) ;
#2091=CARTESIAN_POINT ( 'NONE',  ( -9.999999999998456346, -5.773502691897145489, -25.12499999999994316 ) ) ;
#2093=CARTESIAN_POINT ( 'NONE',  ( 10.81189881249999551, -6.242252689847874514, -107.9687500020483810 ) ) ;
#2095=CARTESIAN_POINT ( 'NONE',  ( -10.81189881249999907, -6.242252689847864744, -80.15625000204839523 ) ) ;
#2096=CARTESIAN_POINT ( 'NONE',  ( 7.644554776091147741E-16, 12.48450537969573659, -89.46875000204838102 ) ) ;
#2098=CARTESIAN_POINT ( 'NONE',  ( -2.121150477449813534E-15, -11.54700538379251284, -142.2500000040967905 ) ) ;
#2101=ORIENTED_EDGE ( 'NONE', *, *, #35354, .T. ) ;
#2104=CARTESIAN_POINT ( 'NONE',  ( 10.00000000000102318, -5.773502691895667560, -39.62499999999992895 ) ) ;
#2105=CARTESIAN_POINT ( 'NONE',  ( 9.999999999999998224, 0.000000000000000000, -27.87500000409676204 ) ) ;
#2108=CARTESIAN_POINT ( 'NONE',  ( -9.999999999999998224, 1.224646799147353059E-15, -65.74999999999997158 ) ) ;
#2110=CARTESIAN_POINT ( 'NONE',  ( -5.000000000000003553, -8.660254037844383745, -79.37500000409677625 ) ) ;
#2112=LINE ( 'NONE', #2325, #18986 ) ;
#2114=CARTESIAN_POINT ( 'NONE',  ( 10.81189881249999551, -6.242252689847874514, -79.65625000204838102 ) ) ;
#2116=FACE_OUTER_BOUND ( 'NONE', #38256, .T. ) ;
#2119=CARTESIAN_POINT ( 'NONE',  ( 7.644554776091147741E-16, 12.48450537969573659, -196.1562500020484379 ) ) ;
#2121=CARTESIAN_POINT ( 'NONE',  ( 5.405949406249999534, 9.363379034771803333, -8.593750002048345493 ) ) ;
#2123=CARTESIAN_POINT ( 'NONE',  ( -5.405949406250003975, -9.363379034771801557, -144.3437500020483810 ) ) ;
#2124=CARTESIAN_POINT ( 'NONE',  ( -9.999999999999998224, 1.224646799147353059E-15, -63.12500000409676204 ) ) ;
#2125=DIRECTION ( 'NONE',  ( -0.8660254037844382635, -0.5000000000000008882, 0.000000000000000000 ) ) ;
#2126=CARTESIAN_POINT ( 'NONE',  ( 10.00000000000000000, 5.773502691896255534, -171.3750000000000000 ) ) ;
#2127=LINE ( 'NONE', #4925, #21375 ) ;
#2128=CARTESIAN_POINT ( 'NONE',  ( 7.644554776091147741E-16, 12.48450537969573659, -104.6562500020483810 ) ) ;
#2129=ORIENTED_EDGE ( 'NONE', *, *, #22815, .F. ) ;
#2132=VERTEX_POINT ( 'NONE', #18070 ) ;
#2133=CARTESIAN_POINT ( 'NONE',  ( -2.293366432827344421E-15, -12.48450537969573659, -33.40625000204835970 ) ) ;
#2135=CARTESIAN_POINT ( 'NONE',  ( -5.405949406249996869, 9.363379034771805109, -87.84375000204836681 ) ) ;
#2137=CARTESIAN_POINT ( 'NONE',  ( -9.999999999999998224, 1.224646799147353059E-15, -125.7499999999999716 ) ) ;
#2140=CARTESIAN_POINT ( 'NONE',  ( 9.999999999999998224, 0.000000000000000000, -11.37500000409674783 ) ) ;
#2141=CARTESIAN_POINT ( 'NONE',  ( -5.000000000000003553, -8.660254037844383745, -77.49999999999998579 ) ) ;
#2143=CARTESIAN_POINT ( 'NONE',  ( 5.405949406249992428, -9.363379034771808662, -120.0937500020483952 ) ) ;
#2147=CARTESIAN_POINT ( 'NONE',  ( 4.999999999999992006, -8.660254037844389075, -178.1250000040968189 ) ) ;
#2148=CARTESIAN_POINT ( 'NONE',  ( -10.81189881249999729, 6.242252689847871849, -173.4062500020483810 ) ) ;
#2149=CARTESIAN_POINT ( 'NONE',  ( -9.999999999998969713, -5.773502691896847949, -1.500000004096725403 ) ) ;
#2152=CARTESIAN_POINT ( 'NONE',  ( 5.405949406249992428, -9.363379034771808662, -42.09375000204837391 ) ) ;
#2154=CARTESIAN_POINT ( 'NONE',  ( -10.81189881249999729, 6.242252689847871849, -2.406250002048375247 ) ) ;
#2156=CARTESIAN_POINT ( 'NONE',  ( 4.999999999999992006, -8.660254037844389075, -193.1250000040967905 ) ) ;
#2158=EDGE_CURVE ( 'NONE', #8575, #38512, #33280, .T. ) ;
#2159=CARTESIAN_POINT ( 'NONE',  ( -9.999999999999998224, 1.224646799147353059E-15, -89.74999999999998579 ) ) ;
#2161=CARTESIAN_POINT ( 'NONE',  ( -4.999999999999996447, 8.660254037844387298, -109.8750000040967763 ) ) ;
#2165=CARTESIAN_POINT ( 'NONE',  ( -5.405949406249996869, 9.363379034771805109, -98.53125000204839523 ) ) ;
#2166=ORIENTED_EDGE ( 'NONE', *, *, #6386, .F. ) ;
#2168=CARTESIAN_POINT ( 'NONE',  ( 9.999999999999479527, 5.773502691896553074, -72.37499999999997158 ) ) ;
#2169=CARTESIAN_POINT ( 'NONE',  ( 10.81189881249999729, 0.000000000000000000, -160.5312500020484094 ) ) ;
#2171=EDGE_LOOP ( 'NONE', ( #33284, #15417, #26687, #53 ) ) ;
#2172=CARTESIAN_POINT ( 'NONE',  ( -9.999999999999998224, 5.773502691896259087, -17.87499999999997513 ) ) ;
#2173=CARTESIAN_POINT ( 'NONE',  ( -2.293366432827344421E-15, -12.48450537969573659, -25.90625000204839168 ) ) ;
#2174=CARTESIAN_POINT ( 'NONE',  ( 4.999999999999992006, -8.660254037844389075, -153.7500000000000000 ) ) ;
#2176=AXIS2_PLACEMENT_3D ( 'NONE', #10835, #17308, #13636 ) ;
#2178=CARTESIAN_POINT ( 'NONE',  ( -5.000000000000003553, -8.660254037844383745, -80.87500000409677625 ) ) ;
#2179=CARTESIAN_POINT ( 'NONE',  ( 10.81189881249999729, 0.000000000000000000, -123.0312500020483952 ) ) ;
#2182=ORIENTED_EDGE ( 'NONE', *, *, #9425, .F. ) ;
#2183=CARTESIAN_POINT ( 'NONE',  ( -10.81189881249999729, 1.324075727343319199E-15, -51.78125000204835970 ) ) ;
#2185=VECTOR ( 'NONE', #6823, 1000.000000000000000 ) ;
#2186=CARTESIAN_POINT ( 'NONE',  ( 7.644554776091147741E-16, 12.48450537969573659, -107.4687500020483668 ) ) ;
#2187=ORIENTED_EDGE ( 'NONE', *, *, #38630, .T. ) ;
#2188=VERTEX_POINT ( 'NONE', #1693 ) ;
#2189=DIRECTION ( 'NONE',  ( -0.000000000000000000, -0.000000000000000000, 1.000000000000000000 ) ) ;
#2190=FACE_OUTER_BOUND ( 'NONE', #25433, .T. ) ;
#2191=CARTESIAN_POINT ( 'NONE',  ( 5.405949406249999534, 9.363379034771803333, -154.0937500020483810 ) ) ;
#2193=CARTESIAN_POINT ( 'NONE',  ( -10.81189881249999907, -6.242252689847864744, -9.468750002048359704 ) ) ;
#2194=CARTESIAN_POINT ( 'NONE',  ( 5.405949406249999534, 9.363379034771803333, -143.5937500020483810 ) ) ;
#2196=CARTESIAN_POINT ( 'NONE',  ( -4.999999999999996447, 8.660254037844387298, -190.8750000040967905 ) ) ;
#2198=CARTESIAN_POINT ( 'NONE',  ( 10.81189881249999729, 0.000000000000000000, -4.343750002048368586 ) ) ;
#2201=CARTESIAN_POINT ( 'NONE',  ( -2.293366432827344421E-15, -12.48450537969573659, -192.4062500020484094 ) ) ;
#2206=CARTESIAN_POINT ( 'NONE',  ( 10.81189881249999551, -6.242252689847874514, -68.96875000204838102 ) ) ;
#2207=CARTESIAN_POINT ( 'NONE',  ( 10.81189881249999551, -6.242252689847874514, -58.46875000204836681 ) ) ;
#2209=CARTESIAN_POINT ( 'NONE',  ( 10.81189881249999907, 6.242252689847868297, -28.40625000204838813 ) ) ;
#2211=CARTESIAN_POINT ( 'NONE',  ( 9.999999999999998224, 0.000000000000000000, -37.99999999999997868 ) ) ;
#2214=CARTESIAN_POINT ( 'NONE',  ( -4.999999999999996447, 8.660254037844387298, -112.4999999999999858 ) ) ;
#2215=CARTESIAN_POINT ( 'NONE',  ( 10.00000000000012257, -5.773502691896187144, -170.1250000000000000 ) ) ;
#2216=EDGE_CURVE ( 'NONE', #17639, #19092, #3050, .T. ) ;
#2219=CARTESIAN_POINT ( 'NONE',  ( 5.405949406249992428, -9.363379034771808662, -10.78125000204835438 ) ) ;
#2221=EDGE_CURVE ( 'NONE', #5513, #38469, #34186, .T. ) ;
#2222=VERTEX_POINT ( 'NONE', #5563 ) ;
#2223=CARTESIAN_POINT ( 'NONE',  ( 9.999999999999998224, 0.000000000000000000, -176.0000000000000000 ) ) ;
#2227=CARTESIAN_POINT ( 'NONE',  ( 9.999999999999996447, -5.773502691896262640, -48.62499999999997868 ) ) ;
#2228=CARTESIAN_POINT ( 'NONE',  ( 9.999999999999996447, -5.773502691896262640, -23.50000000409677625 ) ) ;
#2232=( BOUNDED_CURVE ( )  B_SPLINE_CURVE ( 2, ( #8298, #14738, #1179, #24921, #17766, #11505, #27715 ),
 .UNSPECIFIED., .F., .F. ) 
 B_SPLINE_CURVE_WITH_KNOTS ( ( 3, 2, 2, 3 ),
 ( 0.08955223880597024122, 0.09079601990049755711, 0.09203980099502487300, 0.09328358208955218889 ),
 .UNSPECIFIED. ) 
 CURVE ( )  GEOMETRIC_REPRESENTATION_ITEM ( )  RATIONAL_B_SPLINE_CURVE ( ( 0.9999999999999895639, 0.8660254037844491437, 1.000000000000000000, 0.8660254037844387076, 1.000000000000000000, 0.8660254037844447028, 0.9999999999999940048 ) ) 
 REPRESENTATION_ITEM ( '' )  );
#2234=CARTESIAN_POINT ( 'NONE',  ( -5.405949406249996869, 9.363379034771805109, -142.0312500020483810 ) ) ;
#2235=CARTESIAN_POINT ( 'NONE',  ( -2.293366432827344421E-15, -12.48450537969573659, -151.9062500020483810 ) ) ;
#2237=EDGE_CURVE ( 'NONE', #31040, #30574, #2753, .T. ) ;
#2238=CARTESIAN_POINT ( 'NONE',  ( 4.999999999999992006, -8.660254037844389075, -127.1250000040967620 ) ) ;
#2239=VERTEX_POINT ( 'NONE', #35563 ) ;
#2240=VECTOR ( 'NONE', #34079, 1000.000000000000000 ) ;
#2242=EDGE_CURVE ( 'NONE', #7196, #19666, #21957, .T. ) ;
#2243=ORIENTED_EDGE ( 'NONE', *, *, #42575, .T. ) ;
#2245=EDGE_CURVE ( 'NONE', #3757, #15077, #8800, .T. ) ;
#2247=CARTESIAN_POINT ( 'NONE',  ( -10.81189881249999729, 6.242252689847871849, -179.2187500020483810 ) ) ;
#2249=CARTESIAN_POINT ( 'NONE',  ( -10.81189881249999729, 6.242252689847871849, -35.21875000204835260 ) ) ;
#2250=CARTESIAN_POINT ( 'NONE',  ( 9.999999999999998224, 0.000000000000000000, -119.0000000000000000 ) ) ;
#2251=CARTESIAN_POINT ( 'NONE',  ( -5.405949406250003975, -9.363379034771801557, -165.3437500020484094 ) ) ;
#2252=CARTESIAN_POINT ( 'NONE',  ( -5.405949406249996869, 9.363379034771805109, -149.3437500020483810 ) ) ;
#2253=EDGE_CURVE ( 'NONE', #14889, #10615, #26993, .T. ) ;
#2254=LINE ( 'NONE', #18408, #29341 ) ;
#2258=CARTESIAN_POINT ( 'NONE',  ( 5.000000000000000000, 8.660254037844385522, -129.2499999999999716 ) ) ;
#2259=CARTESIAN_POINT ( 'NONE',  ( -9.999999999999998224, 1.224646799147353059E-15, -200.0000000000000000 ) ) ;
#2261=CARTESIAN_POINT ( 'NONE',  ( 10.81189881249999729, 0.000000000000000000, -80.84375000204838102 ) ) ;
#2262=CARTESIAN_POINT ( 'NONE',  ( 0.000000000000000000, 0.000000000000000000, -200.0000000000000000 ) ) ;
#2263=CARTESIAN_POINT ( 'NONE',  ( 10.81189881249999551, -6.242252689847874514, -48.15625000204836681 ) ) ;
#2264=CARTESIAN_POINT ( 'NONE',  ( -9.999999999999998224, 1.224646799147353059E-15, -59.74999999999997158 ) ) ;
#2266=CARTESIAN_POINT ( 'NONE',  ( -9.999999999999998224, 1.224646799147353059E-15, -137.7499999999999716 ) ) ;
#2267=CARTESIAN_POINT ( 'NONE',  ( -5.405949406250003975, -9.363379034771801557, -147.5312500020483810 ) ) ;
#2268=CARTESIAN_POINT ( 'NONE',  ( -9.999999999999998224, 1.224646799147353059E-15, -142.6250000040967905 ) ) ;
#2270=CARTESIAN_POINT ( 'NONE',  ( -9.999999999999998224, 1.224646799147353059E-15, -123.1250000040967905 ) ) ;
#2272=AXIS2_PLACEMENT_3D ( 'NONE', #14325, #20388, #33375 ) ;
#2273=ORIENTED_EDGE ( 'NONE', *, *, #17957, .T. ) ;
#2276=CARTESIAN_POINT ( 'NONE',  ( -2.121150477449813534E-15, -11.54700538379251284, -48.87499999999997158 ) ) ;
#2277=CARTESIAN_POINT ( 'NONE',  ( -10.81189881249999729, 6.242252689847871849, -179.4062500020484094 ) ) ;
#2278=ORIENTED_EDGE ( 'NONE', *, *, #27004, .F. ) ;
#2279=CARTESIAN_POINT ( 'NONE',  ( 10.00000000000000000, 5.773502691896255534, -48.75000000409676204 ) ) ;
#2280=CARTESIAN_POINT ( 'NONE',  ( 5.000000000000000000, 8.660254037844385522, -130.7499999999999716 ) ) ;
#2282=CARTESIAN_POINT ( 'NONE',  ( 0.000000000000000000, 0.000000000000000000, -200.0000000000000000 ) ) ;
#2283=CARTESIAN_POINT ( 'NONE',  ( -5.405949406250003975, -9.363379034771801557, -173.0312500020484094 ) ) ;
#2284=CARTESIAN_POINT ( 'NONE',  ( 7.070501591499376803E-16, 11.54700538379251284, -7.624999999999972466 ) ) ;
#2285=CARTESIAN_POINT ( 'NONE',  ( 10.00000000000154010, -5.773502691895370020, -56.12499999999992895 ) ) ;
#2287=CARTESIAN_POINT ( 'NONE',  ( 0.000000000000000000, 0.000000000000000000, -200.0000000000000000 ) ) ;
#2289=CARTESIAN_POINT ( 'NONE',  ( 4.999999999999992006, -8.660254037844389075, -71.24999999999998579 ) ) ;
#2290=CARTESIAN_POINT ( 'NONE',  ( -10.81189881249999729, 1.324075727343319199E-15, -75.78125000204838102 ) ) ;
#2291=VERTEX_POINT ( 'NONE', #38994 ) ;
#2292=CARTESIAN_POINT ( 'NONE',  ( -9.999999999999998224, 1.224646799147353059E-15, -98.74999999999998579 ) ) ;
#2293=VERTEX_POINT ( 'NONE', #5990 ) ;
#2294=ORIENTED_EDGE ( 'NONE', *, *, #14066, .F. ) ;
#2295=CARTESIAN_POINT ( 'NONE',  ( -2.293366432827344421E-15, -12.48450537969573659, -30.21875000204834549 ) ) ;
#2297=CARTESIAN_POINT ( 'NONE',  ( 10.81189881249999729, 0.000000000000000000, -3.031250002048374803 ) ) ;
#2298=CARTESIAN_POINT ( 'NONE',  ( -2.293366432827344421E-15, -12.48450537969573659, -57.21875000204835970 ) ) ;
#2299=EDGE_LOOP ( 'NONE', ( #17913, #27942, #12689, #35616 ) ) ;
#2301=CARTESIAN_POINT ( 'NONE',  ( -2.293366432827344421E-15, -12.48450537969573659, -190.7187500020484094 ) ) ;
#2302=CARTESIAN_POINT ( 'NONE',  ( 10.81189881249999907, 6.242252689847868297, -179.7187500020484094 ) ) ;
#2303=( BOUNDED_CURVE ( )  B_SPLINE_CURVE ( 2, ( #1822, #2666, #28791, #19058, #41922, #35478, #28578 ),
 .UNSPECIFIED., .F., .F. ) 
 B_SPLINE_CURVE_WITH_KNOTS ( ( 3, 2, 2, 3 ),
 ( 0.1044776119402986148, 0.1057213930348259306, 0.1069651741293532465, 0.1082089552238805485 ),
 .UNSPECIFIED. ) 
 CURVE ( )  GEOMETRIC_REPRESENTATION_ITEM ( )  RATIONAL_B_SPLINE_CURVE ( ( 0.9999999999999880096, 0.8660254037844506980, 1.000000000000000000, 0.8660254037844387076, 1.000000000000000000, 0.8660254037844431485, 0.9999999999999955591 ) ) 
 REPRESENTATION_ITEM ( '' )  );
#2306=CARTESIAN_POINT ( 'NONE',  ( 4.999999999999992006, -8.660254037844389075, -75.74999999999998579 ) ) ;
#2307=LINE ( 'NONE', #42185, #12936 ) ;
#2309=CARTESIAN_POINT ( 'NONE',  ( -5.405949406250003975, -9.363379034771801557, -105.3437500020483810 ) ) ;
#2310=CARTESIAN_POINT ( 'NONE',  ( 5.405949406249992428, -9.363379034771808662, -70.78125000204838102 ) ) ;
#2311=CARTESIAN_POINT ( 'NONE',  ( 10.81189881249999729, 0.000000000000000000, -92.84375000204838102 ) ) ;
#2313=CARTESIAN_POINT ( 'NONE',  ( -9.999999999999998224, 1.224646799147353059E-15, -148.6250000040967905 ) ) ;
#2321=CARTESIAN_POINT ( 'NONE',  ( -10.00000000000000000, -5.773502691896251982, -62.62499999999996447 ) ) ;
#2323=CARTESIAN_POINT ( 'NONE',  ( -10.00000000000000000, -5.773502691896251982, -76.50000000409677625 ) ) ;
#2325=CARTESIAN_POINT ( 'NONE',  ( 9.999999999999998224, 0.000000000000000000, -200.0000000000000000 ) ) ;
#2327=CARTESIAN_POINT ( 'NONE',  ( 10.81189881249999551, -6.242252689847874514, -66.15625000204839523 ) ) ;
#2329=FACE_OUTER_BOUND ( 'NONE', #10062, .T. ) ;
#2332=CARTESIAN_POINT ( 'NONE',  ( 5.405949406249992428, -9.363379034771808662, -190.7812500020484094 ) ) ;
#2333=ADVANCED_FACE ( 'NONE', ( #6201 ), #9430, .T. ) ;
#2335=CARTESIAN_POINT ( 'NONE',  ( 10.81189881249999551, -6.242252689847874514, -8.968750002048359704 ) ) ;
#2337=CARTESIAN_POINT ( 'NONE',  ( 9.999999999999998224, 0.000000000000000000, -177.5000000000000000 ) ) ;
#2338=CARTESIAN_POINT ( 'NONE',  ( 5.000000000000000000, 8.660254037844385522, -1.749999999999973799 ) ) ;
#2339=CARTESIAN_POINT ( 'NONE',  ( 10.81189881249999729, 0.000000000000000000, -102.0312500020483952 ) ) ;
#2342=VERTEX_POINT ( 'NONE', #42008 ) ;
#2343=ORIENTED_EDGE ( 'NONE', *, *, #6261, .T. ) ;
#2344=EDGE_CURVE ( 'NONE', #5784, #15394, #41602, .T. ) ;
#2345=( BOUNDED_CURVE ( )  B_SPLINE_CURVE ( 2, ( #21279, #34465, #7482, #31231, #34681, #37044, #18249 ),
 .UNSPECIFIED., .F., .F. ) 
 B_SPLINE_CURVE_WITH_KNOTS ( ( 3, 2, 2, 3 ),
 ( 0.6940298507462688837, 0.6952736318407962690, 0.6965174129353237653, 0.6977611940298510396 ),
 .UNSPECIFIED. ) 
 CURVE ( )  GEOMETRIC_REPRESENTATION_ITEM ( )  RATIONAL_B_SPLINE_CURVE ( ( 0.9999999999999761302, 0.8660254037844625774, 1.000000000000000000, 0.8660254037844387076, 1.000000000000000000, 0.8660254037844028474, 1.000000000000035971 ) ) 
 REPRESENTATION_ITEM ( '' )  );
#2346=CARTESIAN_POINT ( 'NONE',  ( 5.405949406249992428, -9.363379034771808662, -30.28125000204837036 ) ) ;
#2348=CARTESIAN_POINT ( 'NONE',  ( -5.405949406250003975, -9.363379034771801557, -75.34375000204838102 ) ) ;
#2353=CARTESIAN_POINT ( 'NONE',  ( -9.999999999999998224, 1.224646799147353059E-15, -10.62500000409674605 ) ) ;
#2354=CARTESIAN_POINT ( 'NONE',  ( -9.999999999999998224, 1.224646799147353059E-15, -86.74999999999998579 ) ) ;
#2355=CARTESIAN_POINT ( 'NONE',  ( 7.644554776091147741E-16, 12.48450537969573659, -129.9687500020483810 ) ) ;
#2356=CARTESIAN_POINT ( 'NONE',  ( 10.81189881249999551, -6.242252689847874514, -113.9687500020483668 ) ) ;
#2359=CARTESIAN_POINT ( 'NONE',  ( 9.999999999999998224, 0.000000000000000000, -168.8750000040967905 ) ) ;
#2360=CARTESIAN_POINT ( 'NONE',  ( -10.81189881249999729, 1.324075727343319199E-15, -173.2812500020484094 ) ) ;
#2361=CARTESIAN_POINT ( 'NONE',  ( 9.999999999999998224, 0.000000000000000000, -27.87500000409676204 ) ) ;
#2364=CARTESIAN_POINT ( 'NONE',  ( 10.81189881249999729, 6.242252689847867408, -44.71875000204837391 ) ) ;
#2366=CARTESIAN_POINT ( 'NONE',  ( 9.999999999999998224, 0.000000000000000000, -86.37500000409677625 ) ) ;
#2368=DIRECTION ( 'NONE',  ( -0.000000000000000000, -0.000000000000000000, 1.000000000000000000 ) ) ;
#2370=CARTESIAN_POINT ( 'NONE',  ( 4.999999999999992006, -8.660254037844389075, -92.24999999999998579 ) ) ;
#2372=CARTESIAN_POINT ( 'NONE',  ( -4.999999999999996447, 8.660254037844387298, -96.37500000409677625 ) ) ;
#2373=CARTESIAN_POINT ( 'NONE',  ( -9.999999999999998224, 1.224646799147353059E-15, -150.1250000040967905 ) ) ;
#2375=CARTESIAN_POINT ( 'NONE',  ( 10.81189881249999551, -6.242252689847874514, -102.1562500020483952 ) ) ;
#2376=VERTEX_POINT ( 'NONE', #38567 ) ;
#2377=EDGE_CURVE ( 'NONE', #33916, #36657, #22178, .T. ) ;
#2380=CARTESIAN_POINT ( 'NONE',  ( -10.81189881249999729, 6.242252689847871849, -159.9062500020483810 ) ) ;
#2382=ORIENTED_EDGE ( 'NONE', *, *, #1313, .F. ) ;
#2383=CARTESIAN_POINT ( 'NONE',  ( 4.999999999999992006, -8.660254037844389075, -18.74999999999996092 ) ) ;
#2384=CARTESIAN_POINT ( 'NONE',  ( -10.81189881249999729, 6.242252689847871849, -26.40625000204837747 ) ) ;
#2385=CARTESIAN_POINT ( 'NONE',  ( 4.999999999999992006, -8.660254037844389075, -156.7500000000000000 ) ) ;
#2388=CARTESIAN_POINT ( 'NONE',  ( -10.81189881249999729, 1.324075727343319199E-15, -129.7812500020483810 ) ) ;
#2391=ORIENTED_EDGE ( 'NONE', *, *, #21343, .F. ) ;
#2392=CARTESIAN_POINT ( 'NONE',  ( 10.81189881249999907, 6.242252689847868297, -52.40625000204838813 ) ) ;
#2394=CARTESIAN_POINT ( 'NONE',  ( 10.81189881249999907, 6.242252689847868297, -106.2187500020483668 ) ) ;
#2395=EDGE_CURVE ( 'NONE', #15576, #38192, #6322, .T. ) ;
#2396=ORIENTED_EDGE ( 'NONE', *, *, #1177, .T. ) ;
#2397=ORIENTED_EDGE ( 'NONE', *, *, #41638, .T. ) ;
#2398=CYLINDRICAL_SURFACE ( 'NONE', #14178, 9.999999999999998224 ) ;
#2399=CARTESIAN_POINT ( 'NONE',  ( -2.293366432827344421E-15, -12.48450537969573659, -159.2187500020483810 ) ) ;
#2401=CARTESIAN_POINT ( 'NONE',  ( -2.293366432827344421E-15, -12.48450537969573659, -4.718750002048369474 ) ) ;
#2403=CARTESIAN_POINT ( 'NONE',  ( -5.405949406249996869, 9.363379034771805109, -141.8437500020483810 ) ) ;
#2405=CARTESIAN_POINT ( 'NONE',  ( 9.999999999998456346, 5.773502691897149042, -55.87499999999995026 ) ) ;
#2407=CARTESIAN_POINT ( 'NONE',  ( -9.999999999999998224, 5.773502691896259087, -193.7500000040967905 ) ) ;
#2409=CARTESIAN_POINT ( 'NONE',  ( -10.81189881249999729, 6.242252689847871849, -192.9062500020484094 ) ) ;
#2413=CARTESIAN_POINT ( 'NONE',  ( 10.81189881249999551, -6.242252689847874514, -70.46875000204839523 ) ) ;
#2414=CARTESIAN_POINT ( 'NONE',  ( -10.81189881249999729, 6.242252689847871849, -54.71875000204838102 ) ) ;
#2416=CARTESIAN_POINT ( 'NONE',  ( -5.405949406250003975, -9.363379034771801557, -29.03125000204837036 ) ) ;
#2418=CARTESIAN_POINT ( 'NONE',  ( -10.00000000000102496, 5.773502691895664007, -52.75000000409673362 ) ) ;
#2420=CARTESIAN_POINT ( 'NONE',  ( 10.00000000000000000, 5.773502691896255534, -112.8749999999999858 ) ) ;
#2424=CARTESIAN_POINT ( 'NONE',  ( 10.81189881249999729, 0.000000000000000000, -12.03125000204835438 ) ) ;
#2425=VERTEX_POINT ( 'NONE', #25632 ) ;
#2426=DIRECTION ( 'NONE',  ( -0.000000000000000000, -0.000000000000000000, 1.000000000000000000 ) ) ;
#2429=CARTESIAN_POINT ( 'NONE',  ( 4.999999999999992006, -8.660254037844389075, -38.24999999999997868 ) ) ;
#2430=CARTESIAN_POINT ( 'NONE',  ( -5.000000000000003553, -8.660254037844383745, -22.37500000409675494 ) ) ;
#2431=CARTESIAN_POINT ( 'NONE',  ( 10.81189881249999729, 0.000000000000000000, -52.53125000204835970 ) ) ;
#2434=DIRECTION ( 'NONE',  ( 1.000000000000000000, 0.000000000000000000, 0.000000000000000000 ) ) ;
#2435=CARTESIAN_POINT ( 'NONE',  ( 5.405949406249999534, 9.363379034771803333, -145.2812500020483810 ) ) ;
#2436=CARTESIAN_POINT ( 'NONE',  ( -10.81189881249999907, -6.242252689847864744, -147.6562500020483810 ) ) ;
#2437=CARTESIAN_POINT ( 'NONE',  ( 9.999999999999998224, 0.000000000000000000, -64.99999999999997158 ) ) ;
#2438=CARTESIAN_POINT ( 'NONE',  ( 0.000000000000000000, 0.000000000000000000, -200.0000000000000000 ) ) ;
#2439=ORIENTED_EDGE ( 'NONE', *, *, #20097, .F. ) ;
#2440=AXIS2_PLACEMENT_3D ( 'NONE', #39241, #35600, #42257 ) ;
#2441=ORIENTED_EDGE ( 'NONE', *, *, #24077, .T. ) ;
#2442=ADVANCED_FACE ( 'NONE', ( #34927 ), #5348, .F. ) ;
#2443=EDGE_LOOP ( 'NONE', ( #16410, #16308 ) ) ;
#2444=EDGE_CURVE ( 'NONE', #6831, #23986, #28456, .T. ) ;
#2446=CARTESIAN_POINT ( 'NONE',  ( 10.81189881249999907, 6.242252689847868297, -181.2187500020484094 ) ) ;
#2447=CARTESIAN_POINT ( 'NONE',  ( 10.81189881249999729, 0.000000000000000000, -34.34375000204836681 ) ) ;
#2448=LINE ( 'NONE', #25119, #40478 ) ;
#2449=CARTESIAN_POINT ( 'NONE',  ( 7.644554776091147741E-16, 12.48450537969573659, -165.9687500020483810 ) ) ;
#2450=CARTESIAN_POINT ( 'NONE',  ( 5.405949406249999534, 9.363379034771803333, -154.0937500020483810 ) ) ;
#2453=VECTOR ( 'NONE', #31359, 1000.000000000000000 ) ;
#2455=( BOUNDED_CURVE ( )  B_SPLINE_CURVE ( 2, ( #13959, #23710, #26521, #20454, #7304, #13542, #4063 ),
 .UNSPECIFIED., .F., .F. ) 
 B_SPLINE_CURVE_WITH_KNOTS ( ( 3, 2, 2, 3 ),
 ( 0.7611940298507464675, 0.7624378109452738528, 0.7636815920398011270, 0.7649253731343285123 ),
 .UNSPECIFIED. ) 
 CURVE ( )  GEOMETRIC_REPRESENTATION_ITEM ( )  RATIONAL_B_SPLINE_CURVE ( ( 0.9999999999999761302, 0.8660254037844625774, 1.000000000000000000, 0.8660254037844387076, 1.000000000000000000, 0.8660254037844267172, 1.000000000000011990 ) ) 
 REPRESENTATION_ITEM ( '' )  );
#2456=CARTESIAN_POINT ( 'NONE',  ( -10.81189881249999907, -6.242252689847864744, -18.46875000204837036 ) ) ;
#2461=CARTESIAN_POINT ( 'NONE',  ( 7.644554776091147741E-16, 12.48450537969573659, -81.96875000204839523 ) ) ;
#2462=CARTESIAN_POINT ( 'NONE',  ( -9.183694056713487929E-15, 20.00000000000000711, 12.49999999999999112 ) ) ;
#2463=CARTESIAN_POINT ( 'NONE',  ( 10.81189881249999551, -6.242252689847874514, -49.65625000204837391 ) ) ;
#2467=ADVANCED_FACE ( 'NONE', ( #13697 ), #10263, .T. ) ;
#2468=CARTESIAN_POINT ( 'NONE',  ( 10.00000000000000000, 5.773502691896255534, -138.3750000000000000 ) ) ;
#2470=CARTESIAN_POINT ( 'NONE',  ( 10.81189881249999551, -6.242252689847874514, -144.1562500020484094 ) ) ;
#2472=CARTESIAN_POINT ( 'NONE',  ( 4.999999999999992006, -8.660254037844389075, -121.1250000040967905 ) ) ;
#2478=CARTESIAN_POINT ( 'NONE',  ( -10.81189881249999907, -6.242252689847864744, -170.1562500020483810 ) ) ;
#2479=CARTESIAN_POINT ( 'NONE',  ( -9.999999999999998224, 1.224646799147353059E-15, -46.62500000409677625 ) ) ;
#2481=CARTESIAN_POINT ( 'NONE',  ( -5.000000000000003553, -8.660254037844383745, -98.49999999999998579 ) ) ;
#2483=CARTESIAN_POINT ( 'NONE',  ( 10.00000000000025402, -5.773502691896113426, -134.5000000040967905 ) ) ;
#2484=CARTESIAN_POINT ( 'NONE',  ( 10.81189881249999729, 0.000000000000000000, -169.5312500020484094 ) ) ;
#2485=DIRECTION ( 'NONE',  ( -0.3779644730092255878, -0.6546536707079759765, 0.6546536707079793072 ) ) ;
#2486=CARTESIAN_POINT ( 'NONE',  ( -9.999999999999998224, 1.224646799147353059E-15, -178.2500000000000284 ) ) ;
#2488=CARTESIAN_POINT ( 'NONE',  ( -9.999999999999868550, 5.773502691896333694, -176.8750000000000000 ) ) ;
#2492=CARTESIAN_POINT ( 'NONE',  ( -5.405949406250003975, -9.363379034771801557, -77.03125000204838102 ) ) ;
#2495=EDGE_CURVE ( 'NONE', #14436, #20180, #26679, .T. ) ;
#2496=CARTESIAN_POINT ( 'NONE',  ( 4.999999999999992006, -8.660254037844389075, -140.2500000000000000 ) ) ;
#2498=AXIS2_PLACEMENT_3D ( 'NONE', #31974, #14726, #8283 ) ;
#2499=ORIENTED_EDGE ( 'NONE', *, *, #3935, .T. ) ;
#2501=CARTESIAN_POINT ( 'NONE',  ( 7.644554776091147741E-16, 12.48450537969573659, -27.96875000204838457 ) ) ;
#2502=CARTESIAN_POINT ( 'NONE',  ( -9.999999999999998224, 1.224646799147353059E-15, -73.62500000409677625 ) ) ;
#2503=CARTESIAN_POINT ( 'NONE',  ( -2.293366432827344421E-15, -12.48450537969573659, -4.906250002048355263 ) ) ;
#2504=CARTESIAN_POINT ( 'NONE',  ( 10.81189881249999551, -6.242252689847874514, -55.46875000204837391 ) ) ;
#2505=ORIENTED_EDGE ( 'NONE', *, *, #42040, .F. ) ;
#2506=EDGE_CURVE ( 'NONE', #41485, #10102, #8689, .T. ) ;
#2507=CARTESIAN_POINT ( 'NONE',  ( 0.000000000000000000, 0.000000000000000000, -200.0000000000000000 ) ) ;
#2509=CARTESIAN_POINT ( 'NONE',  ( 5.405949406249992428, -9.363379034771808662, -187.5937500020483810 ) ) ;
#2510=CARTESIAN_POINT ( 'NONE',  ( -10.81189881249999907, -6.242252689847864744, -174.4687500020484094 ) ) ;
#2513=DIRECTION ( 'NONE',  ( -0.000000000000000000, -0.000000000000000000, 1.000000000000000000 ) ) ;
#2514=LINE ( 'NONE', #13662, #3996 ) ;
#2516=CARTESIAN_POINT ( 'NONE',  ( -10.81189881249999907, -6.242252689847864744, -106.9687500020483668 ) ) ;
#2517=CARTESIAN_POINT ( 'NONE',  ( 9.999999999999998224, 0.000000000000000000, -84.49999999999997158 ) ) ;
#2518=CARTESIAN_POINT ( 'NONE',  ( -10.81189881249999729, 6.242252689847871849, -75.90625000204838102 ) ) ;
#2519=CARTESIAN_POINT ( 'NONE',  ( 5.405949406249999534, 9.363379034771803333, -89.59375000204838102 ) ) ;
#2521=CARTESIAN_POINT ( 'NONE',  ( -10.00000000000000000, -5.773502691896251982, -148.5000000040967905 ) ) ;
#2524=ORIENTED_EDGE ( 'NONE', *, *, #8806, .T. ) ;
#2527=CARTESIAN_POINT ( 'NONE',  ( 7.644554776091147741E-16, 12.48450537969573659, -199.1562500020484094 ) ) ;
#2528=DIRECTION ( 'NONE',  ( -0.000000000000000000, -0.000000000000000000, 1.000000000000000000 ) ) ;
#2530=ORIENTED_EDGE ( 'NONE', *, *, #4082, .F. ) ;
#2531=CARTESIAN_POINT ( 'NONE',  ( -4.999999999999996447, 8.660254037844387298, -67.49999999999997158 ) ) ;
#2533=CARTESIAN_POINT ( 'NONE',  ( -9.999999999999998224, 5.773502691896259087, -72.25000000409676204 ) ) ;
#2537=CARTESIAN_POINT ( 'NONE',  ( 10.81189881249999729, 0.000000000000000000, -64.53125000204836681 ) ) ;
#2539=DIRECTION ( 'NONE',  ( -0.000000000000000000, -0.000000000000000000, 1.000000000000000000 ) ) ;
#2542=CARTESIAN_POINT ( 'NONE',  ( -10.81189881249999729, 1.324075727343319199E-15, -192.7812500020484094 ) ) ;
#2544=CARTESIAN_POINT ( 'NONE',  ( -5.405949406249996869, 9.363379034771805109, -8.343750002048345493 ) ) ;
#2546=CARTESIAN_POINT ( 'NONE',  ( -9.999999999999479527, -5.773502691896549521, -37.50000000409674783 ) ) ;
#2547=DIRECTION ( 'NONE',  ( -0.000000000000000000, -0.000000000000000000, 1.000000000000000000 ) ) ;
#2548=CARTESIAN_POINT ( 'NONE',  ( -4.999999999999996447, 8.660254037844387298, -172.5000000000000284 ) ) ;
#2549=DIRECTION ( 'NONE',  ( -0.000000000000000000, -0.000000000000000000, 1.000000000000000000 ) ) ;
#2550=CARTESIAN_POINT ( 'NONE',  ( 10.81189881249999729, 0.000000000000000000, -99.03125000204839523 ) ) ;
#2551=ORIENTED_EDGE ( 'NONE', *, *, #34353, .F. ) ;
#2553=VERTEX_POINT ( 'NONE', #35975 ) ;
#2554=( BOUNDED_CURVE ( )  B_SPLINE_CURVE ( 2, ( #40314, #23946, #27387, #7534, #40952, #20687, #33873 ),
 .UNSPECIFIED., .F., .F. ) 
 B_SPLINE_CURVE_WITH_KNOTS ( ( 3, 2, 2, 3 ),
 ( 0.3059701492537313383, 0.3072139303482587791, 0.3084577114427861644, 0.3097014925373136052 ),
 .UNSPECIFIED. ) 
 CURVE ( )  GEOMETRIC_REPRESENTATION_ITEM ( )  RATIONAL_B_SPLINE_CURVE ( ( 1.000000000000000000, 0.8660254037844387076, 1.000000000000000000, 0.8660254037844387076, 1.000000000000000000, 0.8660254037844207220, 1.000000000000017986 ) ) 
 REPRESENTATION_ITEM ( '' )  );
#2555=ORIENTED_EDGE ( 'NONE', *, *, #33288, .F. ) ;
#2556=CARTESIAN_POINT ( 'NONE',  ( 10.81189881249999907, 6.242252689847868297, -26.90625000204838102 ) ) ;
#2559=CARTESIAN_POINT ( 'NONE',  ( -10.81189881249999729, 6.242252689847871849, -80.21875000204838102 ) ) ;
#2560=CARTESIAN_POINT ( 'NONE',  ( -9.999999999998969713, -5.773502691896847949, -4.500000004096739836 ) ) ;
#2562=CARTESIAN_POINT ( 'NONE',  ( 9.999999999999998224, 0.000000000000000000, -49.99999999999998579 ) ) ;
#2564=CARTESIAN_POINT ( 'NONE',  ( -9.999999999999998224, 5.773502691896259087, -7.750000004096748718 ) ) ;
#2565=CARTESIAN_POINT ( 'NONE',  ( 9.999999999999998224, 0.000000000000000000, -159.8750000040967905 ) ) ;
#2566=EDGE_CURVE ( 'NONE', #13495, #41596, #28008, .T. ) ;
#2567=CARTESIAN_POINT ( 'NONE',  ( 7.644554776091147741E-16, 12.48450537969573659, -126.9687500020483668 ) ) ;
#2568=CARTESIAN_POINT ( 'NONE',  ( 10.81189881249999729, 0.000000000000000000, -115.3437500020483810 ) ) ;
#2571=CARTESIAN_POINT ( 'NONE',  ( 9.999999999999996447, -5.773502691896262640, -167.5000000040968189 ) ) ;
#2575=CARTESIAN_POINT ( 'NONE',  ( 10.81189881249999729, 0.000000000000000000, -46.34375000204838102 ) ) ;
#2577=CARTESIAN_POINT ( 'NONE',  ( 10.81189881249999729, 0.000000000000000000, -3.031250002048374803 ) ) ;
#2579=CARTESIAN_POINT ( 'NONE',  ( -9.999999999999998224, 1.224646799147353059E-15, -84.12500000409677625 ) ) ;
#2581=CARTESIAN_POINT ( 'NONE',  ( 9.999999999999996447, -5.773502691896262640, -92.12499999999998579 ) ) ;
#2583=CARTESIAN_POINT ( 'NONE',  ( -2.121150477449813534E-15, -11.54700538379251284, -97.25000000409679046 ) ) ;
#2584=CARTESIAN_POINT ( 'NONE',  ( 0.000000000000000000, 0.000000000000000000, -200.0000000000000000 ) ) ;
#2586=CARTESIAN_POINT ( 'NONE',  ( 5.405949406249999534, 9.363379034771803333, -91.28125000204838102 ) ) ;
#2587=ORIENTED_EDGE ( 'NONE', *, *, #31975, .F. ) ;
#2590=CARTESIAN_POINT ( 'NONE',  ( 7.644554776091147741E-16, 12.48450537969573659, -157.1562500020484094 ) ) ;
#2592=VERTEX_POINT ( 'NONE', #20402 ) ;
#2593=CARTESIAN_POINT ( 'NONE',  ( 7.070501591499377789E-16, 11.54700538379251284, -21.12499999999997158 ) ) ;
#2594=CARTESIAN_POINT ( 'NONE',  ( -10.81189881249999729, -6.242252689847864744, -23.15625000204837747 ) ) ;
#2595=CARTESIAN_POINT ( 'NONE',  ( 4.999999999999992006, -8.660254037844389075, -155.2500000000000000 ) ) ;
#2599=CARTESIAN_POINT ( 'NONE',  ( 5.405949406249999534, 9.363379034771803333, -124.2812500020483952 ) ) ;
#2600=VERTEX_POINT ( 'NONE', #42638 ) ;
#2601=CARTESIAN_POINT ( 'NONE',  ( -9.999999999998456346, -5.773502691897145489, -13.12499999999992717 ) ) ;
#2603=CARTESIAN_POINT ( 'NONE',  ( -10.81189881249999729, 6.242252689847871849, -56.40625000204837391 ) ) ;
#2605=CARTESIAN_POINT ( 'NONE',  ( 5.405949406249999534, 9.363379034771803333, -104.5937500020483810 ) ) ;
#2606=ORIENTED_EDGE ( 'NONE', *, *, #105, .F. ) ;
#2607=ORIENTED_EDGE ( 'NONE', *, *, #22754, .T. ) ;
#2608=CARTESIAN_POINT ( 'NONE',  ( -9.999999999999998224, 1.224646799147353059E-15, -30.12500000409676204 ) ) ;
#2609=CARTESIAN_POINT ( 'NONE',  ( -10.81189881249999729, 1.324075727343319199E-15, -152.0937500020483810 ) ) ;
#2611=CARTESIAN_POINT ( 'NONE',  ( 10.81189881249999551, -6.242252689847874514, -4.468750002048369474 ) ) ;
#2612=CYLINDRICAL_SURFACE ( 'NONE', #26607, 9.999999999999998224 ) ;
#2613=CARTESIAN_POINT ( 'NONE',  ( 5.405949406249999534, 9.363379034771803333, -142.0937500020483810 ) ) ;
#2617=CARTESIAN_POINT ( 'NONE',  ( 9.999999999999996447, -5.773502691896262640, -191.5000000040968189 ) ) ;
#2619=CARTESIAN_POINT ( 'NONE',  ( -10.81189881249999729, 6.242252689847871849, -194.4062500020484094 ) ) ;
#2620=CARTESIAN_POINT ( 'NONE',  ( -10.00000000000051337, 5.773502691895962435, -148.7500000040967620 ) ) ;
#2623=CARTESIAN_POINT ( 'NONE',  ( 5.405949406249999534, 9.363379034771803333, -65.59375000204836681 ) ) ;
#2624=CARTESIAN_POINT ( 'NONE',  ( 10.81189881249999729, 0.000000000000000000, -58.34375000204835970 ) ) ;
#2626=CARTESIAN_POINT ( 'NONE',  ( 10.81189881249999551, -6.242252689847874514, -28.65625000204838813 ) ) ;
#2630=CARTESIAN_POINT ( 'NONE',  ( 7.070501591499377789E-16, 11.54700538379251284, -109.6249999999999858 ) ) ;
#2631=AXIS2_PLACEMENT_3D ( 'NONE', #16316, #39632, #20426 ) ;
#2636=CARTESIAN_POINT ( 'NONE',  ( 7.644554776091147741E-16, 12.48450537969573659, -116.6562500020483952 ) ) ;
#2637=ORIENTED_EDGE ( 'NONE', *, *, #16988, .T. ) ;
#2641=CARTESIAN_POINT ( 'NONE',  ( 9.999999999999998224, 0.000000000000000000, -37.99999999999997868 ) ) ;
#2642=CARTESIAN_POINT ( 'NONE',  ( -5.000000000000003553, -8.660254037844383745, -28.37500000409676204 ) ) ;
#2643=CARTESIAN_POINT ( 'NONE',  ( 10.81189881249999729, 6.242252689847867408, -50.90625000204838102 ) ) ;
#2646=CARTESIAN_POINT ( 'NONE',  ( -10.81189881249999729, 6.242252689847871849, -144.9062500020484094 ) ) ;
#2647=CARTESIAN_POINT ( 'NONE',  ( -5.405949406249996869, 9.363379034771805109, -152.5312500020484094 ) ) ;
#2648=CARTESIAN_POINT ( 'NONE',  ( 9.999999999999998224, 0.000000000000000000, -78.87500000409677625 ) ) ;
#2650=ORIENTED_EDGE ( 'NONE', *, *, #8291, .T. ) ;
#2653=AXIS2_PLACEMENT_3D ( 'NONE', #9552, #6531, #13193 ) ;
#2654=CARTESIAN_POINT ( 'NONE',  ( -9.999999999999998224, 1.224646799147353059E-15, -200.0000000000000000 ) ) ;
#2655=CARTESIAN_POINT ( 'NONE',  ( 10.81189881249999907, 6.242252689847868297, -182.7187500020484094 ) ) ;
#2656=CARTESIAN_POINT ( 'NONE',  ( 10.81189881249999907, 6.242252689847868297, -28.21875000204838457 ) ) ;
#2657=DIRECTION ( 'NONE',  ( -0.000000000000000000, -0.000000000000000000, 1.000000000000000000 ) ) ;
#2658=CARTESIAN_POINT ( 'NONE',  ( 10.81189881249999551, -6.242252689847874514, -163.4687500020483810 ) ) ;
#2659=CARTESIAN_POINT ( 'NONE',  ( 5.405949406249992428, -9.363379034771808662, -147.0937500020483810 ) ) ;
#2660=FACE_OUTER_BOUND ( 'NONE', #12502, .T. ) ;
#2663=CARTESIAN_POINT ( 'NONE',  ( 10.81189881249999907, 6.242252689847868297, -20.71875000204836681 ) ) ;
#2665=FACE_OUTER_BOUND ( 'NONE', #18507, .T. ) ;
#2666=CARTESIAN_POINT ( 'NONE',  ( 9.999999999999479527, 5.773502691896553074, -177.7500000040967620 ) ) ;
#2668=CARTESIAN_POINT ( 'NONE',  ( -5.405949406249996869, 9.363379034771805109, -84.84375000204836681 ) ) ;
#2670=CARTESIAN_POINT ( 'NONE',  ( -10.81189881249999729, 1.324075727343319199E-15, -53.28125000204836681 ) ) ;
#2674=CARTESIAN_POINT ( 'NONE',  ( -2.121150477449813534E-15, -11.54700538379251284, -140.3750000000000000 ) ) ;
#2675=CARTESIAN_POINT ( 'NONE',  ( -10.81189881249999729, -6.242252689847864744, -146.1562500020484094 ) ) ;
#2676=CARTESIAN_POINT ( 'NONE',  ( -9.999999999999998224, 1.224646799147353059E-15, -113.7499999999999858 ) ) ;
#2677=CARTESIAN_POINT ( 'NONE',  ( -2.121150477449813534E-15, -11.54700538379251284, -119.7500000040967905 ) ) ;
#2682=CARTESIAN_POINT ( 'NONE',  ( 10.00000000000102318, -5.773502691895667560, -48.62499999999993605 ) ) ;
#2683=CARTESIAN_POINT ( 'NONE',  ( -10.81189881249999729, 6.242252689847871849, -171.9062500020484094 ) ) ;
#2684=CARTESIAN_POINT ( 'NONE',  ( -10.00000000000000000, -5.773502691896251982, -52.50000000409676915 ) ) ;
#2687=CARTESIAN_POINT ( 'NONE',  ( 11.54700538379253416, -19.99999999999999289, 0.000000000000000000 ) ) ;
#2689=CARTESIAN_POINT ( 'NONE',  ( 9.999999999998969713, 5.773502691896851502, -84.37499999999997158 ) ) ;
#2690=CARTESIAN_POINT ( 'NONE',  ( -2.293366432827344421E-15, -12.48450537969573659, -169.9062500020483810 ) ) ;
#2692=CARTESIAN_POINT ( 'NONE',  ( -9.999999999999998224, 1.224646799147353059E-15, -200.0000000000000000 ) ) ;
#2693=EDGE_LOOP ( 'NONE', ( #37783, #7800, #33658, #3709 ) ) ;
#2694=CARTESIAN_POINT ( 'NONE',  ( 10.00000000000012257, -5.773502691896187144, -194.1250000000000568 ) ) ;
#2696=CARTESIAN_POINT ( 'NONE',  ( -5.405949406250003975, -9.363379034771801557, -80.03125000204838102 ) ) ;
#2698=CARTESIAN_POINT ( 'NONE',  ( 10.00000000000051159, -5.773502691895965988, -119.1249999999999858 ) ) ;
#2699=ORIENTED_EDGE ( 'NONE', *, *, #31320, .T. ) ;
#2700=ORIENTED_EDGE ( 'NONE', *, *, #19452, .T. ) ;
#2701=( BOUNDED_CURVE ( )  B_SPLINE_CURVE ( 2, ( #9844, #29924, #23022, #26677, #36175, #16514, #33384 ),
 .UNSPECIFIED., .F., .F. ) 
 B_SPLINE_CURVE_WITH_KNOTS ( ( 3, 2, 2, 3 ),
 ( 0.4067164179104478250, 0.4079601990049751548, 0.4092039800995025400, 0.4104477611940299253 ),
 .UNSPECIFIED. ) 
 CURVE ( )  GEOMETRIC_REPRESENTATION_ITEM ( )  RATIONAL_B_SPLINE_CURVE ( ( 0.9999999999999940048, 0.8660254037844447028, 1.000000000000000000, 0.8660254037844387076, 1.000000000000000000, 0.8660254037844327124, 1.000000000000005995 ) ) 
 REPRESENTATION_ITEM ( '' )  );
#2702=CARTESIAN_POINT ( 'NONE',  ( -10.81189881249999729, -6.242252689847864744, -25.96875000204837391 ) ) ;
#2704=CARTESIAN_POINT ( 'NONE',  ( -10.81189881249999729, 6.242252689847871849, -5.406250002048357928 ) ) ;
#2705=CARTESIAN_POINT ( 'NONE',  ( -5.405949406250003975, -9.363379034771801557, -57.34375000204835970 ) ) ;
#2706=ORIENTED_EDGE ( 'NONE', *, *, #20138, .F. ) ;
#2709=CARTESIAN_POINT ( 'NONE',  ( 5.405949406249999534, 9.363379034771803333, -190.0937500020483810 ) ) ;
#2710=CARTESIAN_POINT ( 'NONE',  ( -5.405949406250003975, -9.363379034771801557, -180.3437500020483810 ) ) ;
#2713=CARTESIAN_POINT ( 'NONE',  ( -9.999999999999998224, 1.224646799147353059E-15, -200.0000000000000000 ) ) ;
#2717=CARTESIAN_POINT ( 'NONE',  ( -2.293366432827344421E-15, -12.48450537969573659, -108.2187500020483668 ) ) ;
#2718=CARTESIAN_POINT ( 'NONE',  ( -9.999999999999998224, 1.224646799147353059E-15, -61.62500000409676204 ) ) ;
#2719=CARTESIAN_POINT ( 'NONE',  ( 7.644554776091147741E-16, 12.48450537969573659, -73.15625000204836681 ) ) ;
#2720=CARTESIAN_POINT ( 'NONE',  ( -4.999999999999996447, 8.660254037844387298, -88.87500000409677625 ) ) ;
#2721=CARTESIAN_POINT ( 'NONE',  ( -5.405949406249996869, 9.363379034771805109, -87.84375000204836681 ) ) ;
#2723=CARTESIAN_POINT ( 'NONE',  ( 7.070501591499377789E-16, 11.54700538379251284, -146.0000000040967905 ) ) ;
#2729=CARTESIAN_POINT ( 'NONE',  ( 10.81189881249999551, -6.242252689847874514, -196.6562500020484379 ) ) ;
#2734=CARTESIAN_POINT ( 'NONE',  ( 9.999999999999998224, 0.000000000000000000, -63.49999999999997158 ) ) ;
#2736=CARTESIAN_POINT ( 'NONE',  ( -9.999999999999998224, 5.773502691896259087, -70.75000000409677625 ) ) ;
#2737=ADVANCED_FACE ( 'NONE', ( #36598 ), #13279, .T. ) ;
#2740=CARTESIAN_POINT ( 'NONE',  ( 0.000000000000000000, 0.000000000000000000, -200.0000000000000000 ) ) ;
#2742=CARTESIAN_POINT ( 'NONE',  ( -5.405949406250003975, -9.363379034771801557, -65.03125000204838102 ) ) ;
#2743=EDGE_CURVE ( 'NONE', #35200, #17857, #10710, .T. ) ;
#2747=CARTESIAN_POINT ( 'NONE',  ( -2.293366432827344421E-15, -12.48450537969573659, -190.9062500020483810 ) ) ;
#2749=CARTESIAN_POINT ( 'NONE',  ( -5.405949406250003975, -9.363379034771801557, -1.843750002048366587 ) ) ;
#2750=CARTESIAN_POINT ( 'NONE',  ( 9.999999999999998224, 0.000000000000000000, -186.8750000040967905 ) ) ;
#2751=CARTESIAN_POINT ( 'NONE',  ( 10.00000000000038014, -5.773502691896040595, -180.6250000000000284 ) ) ;
#2753=LINE ( 'NONE', #26052, #5936 ) ;
#2754=CARTESIAN_POINT ( 'NONE',  ( 9.999999999999998224, 0.000000000000000000, -174.5000000000000284 ) ) ;
#2755=CARTESIAN_POINT ( 'NONE',  ( 4.999999999999992006, -8.660254037844389075, -36.74999999999997868 ) ) ;
#2756=AXIS2_PLACEMENT_3D ( 'NONE', #17575, #18008, #41089 ) ;
#2757=CARTESIAN_POINT ( 'NONE',  ( 5.405949406249999534, 9.363379034771803333, -101.7812500020483952 ) ) ;
#2759=DIRECTION ( 'NONE',  ( -0.000000000000000000, -0.000000000000000000, 1.000000000000000000 ) ) ;
#2760=ORIENTED_EDGE ( 'NONE', *, *, #35064, .F. ) ;
#2761=ORIENTED_EDGE ( 'NONE', *, *, #34676, .F. ) ;
#2762=CARTESIAN_POINT ( 'NONE',  ( -5.405949406249996869, 9.363379034771805109, -31.03125000204837036 ) ) ;
#2764=EDGE_CURVE ( 'NONE', #933, #20180, #8329, .T. ) ;
#2765=CARTESIAN_POINT ( 'NONE',  ( -2.293366432827344421E-15, -12.48450537969573659, -76.71875000204838102 ) ) ;
#2766=CARTESIAN_POINT ( 'NONE',  ( -5.000000000000003553, -8.660254037844383745, -4.375000004096768258 ) ) ;
#2767=CARTESIAN_POINT ( 'NONE',  ( -9.999999999999998224, 1.224646799147353059E-15, -148.6250000040967905 ) ) ;
#2771=CARTESIAN_POINT ( 'NONE',  ( 10.00000000000000000, 5.773502691896255534, -11.25000000409676559 ) ) ;
#2772=CARTESIAN_POINT ( 'NONE',  ( -2.121150477449813534E-15, -11.54700538379251284, -125.3749999999999858 ) ) ;
#2773=CARTESIAN_POINT ( 'NONE',  ( -2.293366432827344421E-15, -12.48450537969573659, -132.2187500020483810 ) ) ;
#2774=CARTESIAN_POINT ( 'NONE',  ( 5.405949406249992428, -9.363379034771808662, -99.28125000204839523 ) ) ;
#2775=CARTESIAN_POINT ( 'NONE',  ( -10.81189881249999729, -6.242252689847864744, -112.9687500020483810 ) ) ;
#2779=CARTESIAN_POINT ( 'NONE',  ( 5.000000000000000000, 8.660254037844385522, -171.6250000040968189 ) ) ;
#2780=CYLINDRICAL_SURFACE ( 'NONE', #37877, 9.999999999999998224 ) ;
#2784=CARTESIAN_POINT ( 'NONE',  ( 7.644554776091147741E-16, 12.48450537969573659, -4.156250002048351710 ) ) ;
#2786=CARTESIAN_POINT ( 'NONE',  ( -4.999999999999996447, 8.660254037844387298, -5.999999999999977796 ) ) ;
#2788=CARTESIAN_POINT ( 'NONE',  ( -4.999999999999996447, 8.660254037844387298, -89.99999999999998579 ) ) ;
#2790=CARTESIAN_POINT ( 'NONE',  ( 5.000000000000000000, 8.660254037844385522, -99.62500000409679046 ) ) ;
#2791=CARTESIAN_POINT ( 'NONE',  ( 5.000000000000000000, 8.660254037844385522, -150.6250000040967905 ) ) ;
#2793=CARTESIAN_POINT ( 'NONE',  ( -10.81189881249999729, 1.324075727343319199E-15, -93.78125000204838102 ) ) ;
#2794=ORIENTED_EDGE ( 'NONE', *, *, #26453, .F. ) ;
#2799=CARTESIAN_POINT ( 'NONE',  ( -4.999999999999996447, 8.660254037844387298, -19.49999999999996092 ) ) ;
#2800=PRODUCT ( 'thrust bolt', 'thrust bolt', '', ( #1706 ) ) ;
#2801=CARTESIAN_POINT ( 'NONE',  ( -9.999999999999998224, 1.224646799147353059E-15, -155.7500000000000000 ) ) ;
#2802=( BOUNDED_CURVE ( )  B_SPLINE_CURVE ( 2, ( #16105, #35577, #22400, #35366, #38586, #4998, #32132 ),
 .UNSPECIFIED., .F., .F. ) 
 B_SPLINE_CURVE_WITH_KNOTS ( ( 3, 2, 2, 3 ),
 ( 0.8358208955223882519, 0.8370646766169156372, 0.8383084577114430225, 0.8395522388059704078 ),
 .UNSPECIFIED. ) 
 CURVE ( )  GEOMETRIC_REPRESENTATION_ITEM ( )  RATIONAL_B_SPLINE_CURVE ( ( 0.9999999999999761302, 0.8660254037844625774, 1.000000000000000000, 0.8660254037844387076, 1.000000000000000000, 0.8660254037844148378, 1.000000000000023981 ) ) 
 REPRESENTATION_ITEM ( '' )  );
#2804=CARTESIAN_POINT ( 'NONE',  ( -10.00000000000000000, -5.773502691896251982, -196.1250000000000568 ) ) ;
#2805=EDGE_CURVE ( 'NONE', #4916, #2592, #4676, .T. ) ;
#2806=CARTESIAN_POINT ( 'NONE',  ( 5.405949406249992428, -9.363379034771808662, -127.7812500020483810 ) ) ;
#2807=EDGE_LOOP ( 'NONE', ( #32693, #5933, #28776, #13228 ) ) ;
#2808=CARTESIAN_POINT ( 'NONE',  ( 5.000000000000000000, 8.660254037844385522, -90.24999999999998579 ) ) ;
#2809=ORIENTED_EDGE ( 'NONE', *, *, #37458, .T. ) ;
#2810=CARTESIAN_POINT ( 'NONE',  ( -10.81189881249999907, -6.242252689847864744, -51.65625000204838102 ) ) ;
#2812=CARTESIAN_POINT ( 'NONE',  ( -10.81189881249999907, -6.242252689847864744, -103.9687500020483668 ) ) ;
#2814=ORIENTED_EDGE ( 'NONE', *, *, #14112, .F. ) ;
#2815=CARTESIAN_POINT ( 'NONE',  ( -2.121150477449813534E-15, -11.54700538379251284, -175.2500000040968189 ) ) ;
#2816=CARTESIAN_POINT ( 'NONE',  ( 7.070501591499376803E-16, 11.54700538379251284, -33.12499999999996447 ) ) ;
#2818=CARTESIAN_POINT ( 'NONE',  ( -5.405949406249996869, 9.363379034771805109, 0.6562499979516356330 ) ) ;
#2820=CARTESIAN_POINT ( 'NONE',  ( -10.81189881249999729, 1.324075727343319199E-15, -140.0937500020483810 ) ) ;
#2824=CARTESIAN_POINT ( 'NONE',  ( -9.999999999999998224, 1.224646799147353059E-15, -196.6250000040967905 ) ) ;
#2826=CARTESIAN_POINT ( 'NONE',  ( 10.81189881249999729, 0.000000000000000000, -186.0312500020484094 ) ) ;
#2827=DIRECTION ( 'NONE',  ( 1.000000000000000000, 0.000000000000000000, 0.000000000000000000 ) ) ;
#2830=CARTESIAN_POINT ( 'NONE',  ( 5.405949406249999534, 9.363379034771803333, -67.09375000204836681 ) ) ;
#2831=CARTESIAN_POINT ( 'NONE',  ( 10.81189881249999907, 6.242252689847868297, -46.21875000204837391 ) ) ;
#2833=CARTESIAN_POINT ( 'NONE',  ( 10.81189881249999551, -6.242252689847874514, -27.15625000204838102 ) ) ;
#2837=CARTESIAN_POINT ( 'NONE',  ( -4.999999999999996447, 8.660254037844387298, -110.9999999999999858 ) ) ;
#2838=CARTESIAN_POINT ( 'NONE',  ( -10.00000000000012434, 5.773502691896184480, -163.3750000000000000 ) ) ;
#2841=CARTESIAN_POINT ( 'NONE',  ( 5.405949406249999534, 9.363379034771803333, -118.2812500020483952 ) ) ;
#2842=EDGE_LOOP ( 'NONE', ( #40100, #1900, #35411, #10533 ) ) ;
#2848=CARTESIAN_POINT ( 'NONE',  ( 4.999999999999992006, -8.660254037844389075, -44.24999999999998579 ) ) ;
#2850=CARTESIAN_POINT ( 'NONE',  ( -2.121150477449813534E-15, -11.54700538379251284, -25.25000000409676559 ) ) ;
#2851=CARTESIAN_POINT ( 'NONE',  ( 5.405949406249992428, -9.363379034771808662, -40.78125000204838102 ) ) ;
#2852=CARTESIAN_POINT ( 'NONE',  ( 9.999999999999998224, 0.000000000000000000, -168.8750000040967905 ) ) ;
#2855=( BOUNDED_CURVE ( )  B_SPLINE_CURVE ( 2, ( #4115, #33482, #33051, #13799, #6713, #885, #23118 ),
 .UNSPECIFIED., .F., .F. ) 
 B_SPLINE_CURVE_WITH_KNOTS ( ( 3, 2, 2, 3 ),
 ( 0.01865671641791046345, 0.01990049751243783138, 0.02114427860696519584, 0.02238805970149256030 ),
 .UNSPECIFIED. ) 
 CURVE ( )  GEOMETRIC_REPRESENTATION_ITEM ( )  RATIONAL_B_SPLINE_CURVE ( ( 0.9999999999999981126, 0.8660254037844405950, 1.000000000000000000, 0.8660254037844387076, 1.000000000000000000, 0.8660254037844360431, 1.000000000000002665 ) ) 
 REPRESENTATION_ITEM ( '' )  );
#2857=CARTESIAN_POINT ( 'NONE',  ( -5.405949406249996869, 9.363379034771805109, -134.5312500020484094 ) ) ;
#2859=CARTESIAN_POINT ( 'NONE',  ( 10.81189881249999907, 6.242252689847868297, -148.4062500020484094 ) ) ;
#2860=LINE ( 'NONE', #3708, #10013 ) ;
#2862=ORIENTED_EDGE ( 'NONE', *, *, #7910, .F. ) ;
#2863=ORIENTED_EDGE ( 'NONE', *, *, #39892, .T. ) ;
#2865=VECTOR ( 'NONE', #1147, 1000.000000000000000 ) ;
#2867=CARTESIAN_POINT ( 'NONE',  ( 10.81189881249999907, 6.242252689847868297, -176.7187500020483810 ) ) ;
#2869=CARTESIAN_POINT ( 'NONE',  ( -2.293366432827344421E-15, -12.48450537969573659, -33.21875000204834549 ) ) ;
#2871=CARTESIAN_POINT ( 'NONE',  ( 10.81189881249999729, 6.242252689847867408, -164.7187500020483810 ) ) ;
#2872=CARTESIAN_POINT ( 'NONE',  ( 10.81189881249999551, -6.242252689847874514, -148.4687500020484094 ) ) ;
#2873=FACE_OUTER_BOUND ( 'NONE', #42621, .T. ) ;
#2876=CARTESIAN_POINT ( 'NONE',  ( -5.405949406249996869, 9.363379034771805109, -15.84375000204835082 ) ) ;
#2879=CARTESIAN_POINT ( 'NONE',  ( 7.070501591499376803E-16, 11.54700538379251284, -25.62499999999997868 ) ) ;
#2881=VECTOR ( 'NONE', #271, 1000.000000000000000 ) ;
#2882=CARTESIAN_POINT ( 'NONE',  ( -10.81189881249999907, -6.242252689847864744, -73.96875000204836681 ) ) ;
#2883=CARTESIAN_POINT ( 'NONE',  ( 7.644554776091147741E-16, 12.48450537969573659, -50.65625000204838102 ) ) ;
#2887=CARTESIAN_POINT ( 'NONE',  ( 7.070501591499377789E-16, 11.54700538379251284, -133.6250000000000000 ) ) ;
#2888=CARTESIAN_POINT ( 'NONE',  ( 10.81189881249999729, 6.242252689847867408, -146.9062500020484379 ) ) ;
#2890=CARTESIAN_POINT ( 'NONE',  ( 5.000000000000000000, 8.660254037844385522, -119.1250000040967905 ) ) ;
#2892=ORIENTED_EDGE ( 'NONE', *, *, #33101, .F. ) ;
#2895=EDGE_CURVE ( 'NONE', #2913, #27845, #40667, .T. ) ;
#2896=CARTESIAN_POINT ( 'NONE',  ( 10.81189881249999907, 6.242252689847868297, -170.9062500020484094 ) ) ;
#2897=CARTESIAN_POINT ( 'NONE',  ( -4.999999999999996447, 8.660254037844387298, -51.37500000409675494 ) ) ;
#2898=CARTESIAN_POINT ( 'NONE',  ( -9.999999999999998224, 1.224646799147353059E-15, -91.62500000409677625 ) ) ;
#2900=VECTOR ( 'NONE', #23093, 1000.000000000000000 ) ;
#2903=CARTESIAN_POINT ( 'NONE',  ( 10.81189881249999551, -6.242252689847874514, -160.6562500020484379 ) ) ;
#2904=CARTESIAN_POINT ( 'NONE',  ( -5.405949406250003975, -9.363379034771801557, -141.3437500020483810 ) ) ;
#2905=DIRECTION ( 'NONE',  ( 0.000000000000000000, 1.000000000000000000, 0.000000000000000000 ) ) ;
#2906=CARTESIAN_POINT ( 'NONE',  ( -10.00000000000051337, 5.773502691895962435, -79.75000000409677625 ) ) ;
#2909=CARTESIAN_POINT ( 'NONE',  ( 10.81189881249999551, -6.242252689847874514, -66.15625000204839523 ) ) ;
#2910=ORIENTED_EDGE ( 'NONE', *, *, #30528, .T. ) ;
#2913=VERTEX_POINT ( 'NONE', #21262 ) ;
#2916=CARTESIAN_POINT ( 'NONE',  ( 5.405949406249999534, 9.363379034771803333, -29.59375000204836326 ) ) ;
#2918=CARTESIAN_POINT ( 'NONE',  ( 5.405949406249999534, 9.363379034771803333, -1.281250002048373027 ) ) ;
#2919=CARTESIAN_POINT ( 'NONE',  ( 7.644554776091147741E-16, 12.48450537969573659, -51.96875000204836681 ) ) ;
#2923=CARTESIAN_POINT ( 'NONE',  ( 7.644554776091147741E-16, 12.48450537969573659, -188.4687500020484094 ) ) ;
#2924=CARTESIAN_POINT ( 'NONE',  ( 5.405949406249992428, -9.363379034771808662, -166.5937500020484094 ) ) ;
#2928=CARTESIAN_POINT ( 'NONE',  ( -9.999999999998969713, -5.773502691896847949, -76.12499999999998579 ) ) ;
#2929=CARTESIAN_POINT ( 'NONE',  ( -10.00000000000022027, 5.773502691896128525, -187.7500000040967620 ) ) ;
#2931=CARTESIAN_POINT ( 'NONE',  ( -10.81189881249999729, 1.324075727343319199E-15, -95.09375000204838102 ) ) ;
#2932=CARTESIAN_POINT ( 'NONE',  ( 7.070501591499376803E-16, 11.54700538379251284, -108.5000000040967763 ) ) ;
#2933=CARTESIAN_POINT ( 'NONE',  ( 10.81189881249999729, 0.000000000000000000, -73.53125000204838102 ) ) ;
#2934=CARTESIAN_POINT ( 'NONE',  ( -10.00000000000051337, 5.773502691895962435, -96.25000000409676204 ) ) ;
#2936=CARTESIAN_POINT ( 'NONE',  ( -10.81189881249999729, 1.324075727343319199E-15, -84.59375000204836681 ) ) ;
#2938=CARTESIAN_POINT ( 'NONE',  ( 9.999999999999996447, -5.773502691896262640, -145.0000000040967905 ) ) ;
#2944=CARTESIAN_POINT ( 'NONE',  ( -10.81189881249999729, 1.324075727343319199E-15, -192.7812500020484094 ) ) ;
#2945=CARTESIAN_POINT ( 'NONE',  ( 9.999999999999998224, 0.000000000000000000, -66.87500000409676204 ) ) ;
#2947=ORIENTED_EDGE ( 'NONE', *, *, #17700, .T. ) ;
#2948=CARTESIAN_POINT ( 'NONE',  ( -9.999999999999998224, 5.773502691896259087, -61.37499999999998579 ) ) ;
#2950=CARTESIAN_POINT ( 'NONE',  ( -2.121150477449813534E-15, -11.54700538379251284, -74.75000000409677625 ) ) ;
#2951=DIRECTION ( 'NONE',  ( -0.000000000000000000, -0.000000000000000000, -1.000000000000000000 ) ) ;
#2952=CARTESIAN_POINT ( 'NONE',  ( -5.000000000000003553, -8.660254037844383745, -160.3750000040967905 ) ) ;
#2954=CARTESIAN_POINT ( 'NONE',  ( 5.405949406249999534, 9.363379034771803333, -65.78125000204838102 ) ) ;
#2958=CARTESIAN_POINT ( 'NONE',  ( -10.81189881249999729, 1.324075727343319199E-15, -191.2812500020484094 ) ) ;
#2960=DIRECTION ( 'NONE',  ( 0.08682659386424779191, 0.08682659386424779191, 0.9924325091389669673 ) ) ;
#2961=PLANE ( 'NONE',  #37337 ) ;
#2962=CARTESIAN_POINT ( 'NONE',  ( 4.999999999999992006, -8.660254037844389075, -112.1250000040967763 ) ) ;
#2963=( BOUNDED_CURVE ( )  B_SPLINE_CURVE ( 2, ( #12592, #5724, #28395, #41535, #11963, #35079, #38511 ),
 .UNSPECIFIED., .F., .F. ) 
 B_SPLINE_CURVE_WITH_KNOTS ( ( 3, 2, 2, 3 ),
 ( 0.8171641791044778058, 0.8184079601990051911, 0.8196517412935324653, 0.8208955223880598506 ),
 .UNSPECIFIED. ) 
 CURVE ( )  GEOMETRIC_REPRESENTATION_ITEM ( )  RATIONAL_B_SPLINE_CURVE ( ( 0.9999999999999761302, 0.8660254037844625774, 1.000000000000000000, 0.8660254037844387076, 1.000000000000000000, 0.8660254037844267172, 1.000000000000011990 ) ) 
 REPRESENTATION_ITEM ( '' )  );
#2964=CARTESIAN_POINT ( 'NONE',  ( -2.121150477449813534E-15, -11.54700538379251284, -173.3750000000000000 ) ) ;
#2965=FACE_OUTER_BOUND ( 'NONE', #36246, .T. ) ;
#2966=CARTESIAN_POINT ( 'NONE',  ( 10.81189881249999551, -6.242252689847874514, -97.65625000204839523 ) ) ;
#2967=EDGE_LOOP ( 'NONE', ( #9119, #38047, #30125, #16707 ) ) ;
#2968=CARTESIAN_POINT ( 'NONE',  ( -9.999999999999998224, 1.224646799147353059E-15, -164.7500000000000000 ) ) ;
#2969=ORIENTED_EDGE ( 'NONE', *, *, #19490, .T. ) ;
#2970=ORIENTED_EDGE ( 'NONE', *, *, #23291, .F. ) ;
#2971=CARTESIAN_POINT ( 'NONE',  ( -10.81189881249999907, -6.242252689847864744, -37.96875000204837391 ) ) ;
#2972=CARTESIAN_POINT ( 'NONE',  ( 7.644554776091147741E-16, 12.48450537969573659, -29.65625000204835970 ) ) ;
#2974=EDGE_CURVE ( 'NONE', #18914, #15678, #38842, .T. ) ;
#2975=CARTESIAN_POINT ( 'NONE',  ( -10.81189881249999729, 6.242252689847871849, -81.71875000204838102 ) ) ;
#2977=ADVANCED_FACE ( 'NONE', ( #37026 ), #1211, .T. ) ;
#2978=CARTESIAN_POINT ( 'NONE',  ( -10.81189881249999907, -6.242252689847864744, -190.9687500020484379 ) ) ;
#2979=EDGE_CURVE ( 'NONE', #5197, #32856, #17903, .T. ) ;
#2980=LINE ( 'NONE', #15691, #23998 ) ;
#2983=CARTESIAN_POINT ( 'NONE',  ( -4.999999999999996447, 8.660254037844387298, -12.37500000409674783 ) ) ;
#2984=DIRECTION ( 'NONE',  ( 1.000000000000000000, 0.000000000000000000, 0.000000000000000000 ) ) ;
#2985=CARTESIAN_POINT ( 'NONE',  ( -10.81189881249999729, 6.242252689847871849, -128.2187500020483810 ) ) ;
#2986=CARTESIAN_POINT ( 'NONE',  ( -5.405949406249996869, 9.363379034771805109, -101.5312500020483952 ) ) ;
#2987=CARTESIAN_POINT ( 'NONE',  ( 10.81189881249999551, -6.242252689847874514, -107.9687500020483810 ) ) ;
#2990=CARTESIAN_POINT ( 'NONE',  ( -2.121150477449813534E-15, -11.54700538379251284, -173.7500000040968189 ) ) ;
#2991=CARTESIAN_POINT ( 'NONE',  ( 9.999999999999998224, 0.000000000000000000, -33.49999999999997158 ) ) ;
#2995=CARTESIAN_POINT ( 'NONE',  ( 9.999999999999998224, 0.000000000000000000, -189.5000000000000000 ) ) ;
#2999=CARTESIAN_POINT ( 'NONE',  ( 7.070501591499377789E-16, 11.54700538379251284, -79.62500000000000000 ) ) ;
#3001=CARTESIAN_POINT ( 'NONE',  ( 10.00000000000000000, 5.773502691896255534, -101.2500000040967905 ) ) ;
#3003=LINE ( 'NONE', #6452, #34136 ) ;
#3005=CARTESIAN_POINT ( 'NONE',  ( -5.405949406249996869, 9.363379034771805109, -91.03125000204838102 ) ) ;
#3008=LINE ( 'NONE', #23068, #18798 ) ;
#3010=ORIENTED_EDGE ( 'NONE', *, *, #24247, .F. ) ;
#3011=CARTESIAN_POINT ( 'NONE',  ( 9.999999999999998224, 0.000000000000000000, -15.49999999999995737 ) ) ;
#3012=CARTESIAN_POINT ( 'NONE',  ( -10.00000000000000000, -5.773502691896251982, -152.6250000000000284 ) ) ;
#3013=ADVANCED_FACE ( 'NONE', ( #15618 ), #35296, .T. ) ;
#3016=CARTESIAN_POINT ( 'NONE',  ( 5.405949406249992428, -9.363379034771808662, -124.7812500020483952 ) ) ;
#3017=ORIENTED_EDGE ( 'NONE', *, *, #28328, .F. ) ;
#3019=ORIENTED_EDGE ( 'NONE', *, *, #21343, .T. ) ;
#3020=CARTESIAN_POINT ( 'NONE',  ( 10.81189881249999729, 0.000000000000000000, -57.03125000204836681 ) ) ;
#3022=CARTESIAN_POINT ( 'NONE',  ( -2.293366432827344421E-15, -12.48450537969573659, -106.7187500020483668 ) ) ;
#3023=ORIENTED_EDGE ( 'NONE', *, *, #27774, .F. ) ;
#3025=CARTESIAN_POINT ( 'NONE',  ( 0.000000000000000000, 0.000000000000000000, -200.0000000000000000 ) ) ;
#3026=DIRECTION ( 'NONE',  ( -0.9961946980917455452, 0.000000000000000000, -0.08715574274765837404 ) ) ;
#3027=ADVANCED_FACE ( 'NONE', ( #24952 ), #38733, .T. ) ;
#3029=CARTESIAN_POINT ( 'NONE',  ( 10.81189881249999907, 6.242252689847868297, -1.218750002048353709 ) ) ;
#3032=CARTESIAN_POINT ( 'NONE',  ( 7.644554776091147741E-16, 12.48450537969573659, -131.4687500020483810 ) ) ;
#3036=CARTESIAN_POINT ( 'NONE',  ( 4.999999999999992006, -8.660254037844389075, -193.1250000040967905 ) ) ;
#3038=CARTESIAN_POINT ( 'NONE',  ( -5.405949406249996869, 9.363379034771805109, -188.5312500020484094 ) ) ;
#3039=CARTESIAN_POINT ( 'NONE',  ( -9.999999999999998224, 1.224646799147353059E-15, -148.6250000040967905 ) ) ;
#3042=CARTESIAN_POINT ( 'NONE',  ( -10.81189881249999729, 1.324075727343319199E-15, -65.09375000204836681 ) ) ;
#3043=CARTESIAN_POINT ( 'NONE',  ( 10.81189881249999551, -6.242252689847874514, -50.96875000204836681 ) ) ;
#3045=CARTESIAN_POINT ( 'NONE',  ( -10.81189881249999907, -6.242252689847864744, -20.15625000204838102 ) ) ;
#3049=CARTESIAN_POINT ( 'NONE',  ( -2.121150477449813534E-15, -11.54700538379251284, -113.3749999999999858 ) ) ;
#3050=( BOUNDED_CURVE ( )  B_SPLINE_CURVE ( 2, ( #18286, #36706, #28235, #25008, #7145, #16834, #32326 ),
 .UNSPECIFIED., .F., .F. ) 
 B_SPLINE_CURVE_WITH_KNOTS ( ( 3, 2, 2, 3 ),
 ( 0.3283582089552238847, 0.3296019900497513255, 0.3308457711442787108, 0.3320895522388061516 ),
 .UNSPECIFIED. ) 
 CURVE ( )  GEOMETRIC_REPRESENTATION_ITEM ( )  RATIONAL_B_SPLINE_CURVE ( ( 1.000000000000000000, 0.8660254037844387076, 1.000000000000000000, 0.8660254037844387076, 1.000000000000000000, 0.8660254037844207220, 1.000000000000017986 ) ) 
 REPRESENTATION_ITEM ( '' )  );
#3054=CARTESIAN_POINT ( 'NONE',  ( -10.81189881249999729, 1.324075727343319199E-15, -116.2812500020483952 ) ) ;
#3055=ADVANCED_FACE ( 'NONE', ( #25785 ), #28180, .F. ) ;
#3056=VERTEX_POINT ( 'NONE', #41538 ) ;
#3057=LINE ( 'NONE', #32209, #27242 ) ;
#3059=CARTESIAN_POINT ( 'NONE',  ( 12.99038105676667243, 7.500000000000067502, 49.99999999999998579 ) ) ;
#3061=VERTEX_POINT ( 'NONE', #22332 ) ;
#3062=CARTESIAN_POINT ( 'NONE',  ( 5.000000000000000000, 8.660254037844385522, -43.74999999999998579 ) ) ;
#3063=CARTESIAN_POINT ( 'NONE',  ( 7.070501591499377789E-16, 11.54700538379251284, -18.50000000409676559 ) ) ;
#3064=CARTESIAN_POINT ( 'NONE',  ( 10.81189881249999551, -6.242252689847874514, -40.65625000204836681 ) ) ;
#3065=CARTESIAN_POINT ( 'NONE',  ( 9.999999999999998224, 0.000000000000000000, -16.99999999999996092 ) ) ;
#3068=CARTESIAN_POINT ( 'NONE',  ( 7.423074889580975722, -12.85714285714295180, 52.14285714285716011 ) ) ;
#3069=CARTESIAN_POINT ( 'NONE',  ( -2.293366432827344421E-15, -12.48450537969573659, -139.9062500020484094 ) ) ;
#3070=CARTESIAN_POINT ( 'NONE',  ( 5.405949406249999534, 9.363379034771803333, -148.2812500020483810 ) ) ;
#3072=VERTEX_POINT ( 'NONE', #25368 ) ;
#3074=ORIENTED_EDGE ( 'NONE', *, *, #26692, .F. ) ;
#3075=LINE ( 'NONE', #29833, #24954 ) ;
#3076=CARTESIAN_POINT ( 'NONE',  ( 5.405949406249999534, 9.363379034771803333, -173.5937500020484094 ) ) ;
#3077=CARTESIAN_POINT ( 'NONE',  ( -2.293366432827344421E-15, -12.48450537969573659, -19.71875000204837747 ) ) ;
#3079=CARTESIAN_POINT ( 'NONE',  ( -10.81189881249999729, 6.242252689847871849, -155.2187500020483810 ) ) ;
#3080=CARTESIAN_POINT ( 'NONE',  ( -10.81189881249999907, -6.242252689847864744, -141.4687500020484094 ) ) ;
#3081=CARTESIAN_POINT ( 'NONE',  ( -9.999999999999998224, 1.224646799147353059E-15, -67.24999999999997158 ) ) ;
#3084=CARTESIAN_POINT ( 'NONE',  ( 5.405949406249999534, 9.363379034771803333, -14.59375000204835082 ) ) ;
#3087=( BOUNDED_CURVE ( )  B_SPLINE_CURVE ( 2, ( #41226, #2405, #5208, #1554, #8666, #24864, #18580 ),
 .UNSPECIFIED., .F., .F. ) 
 B_SPLINE_CURVE_WITH_KNOTS ( ( 3, 2, 2, 3 ),
 ( 0.7164179104477614857, 0.7176616915422888709, 0.7189054726368161452, 0.7201492537313435305 ),
 .UNSPECIFIED. ) 
 CURVE ( )  GEOMETRIC_REPRESENTATION_ITEM ( )  RATIONAL_B_SPLINE_CURVE ( ( 0.9999999999999641398, 0.8660254037844745678, 1.000000000000000000, 0.8660254037844387076, 1.000000000000000000, 0.8660254037844148378, 1.000000000000023981 ) ) 
 REPRESENTATION_ITEM ( '' )  );
#3090=CARTESIAN_POINT ( 'NONE',  ( 9.999999999999479527, 5.773502691896553074, -99.75000000409679046 ) ) ;
#3091=EDGE_CURVE ( 'NONE', #900, #22125, #533, .T. ) ;
#3092=CARTESIAN_POINT ( 'NONE',  ( 10.81189881249999907, 6.242252689847868297, -70.21875000204840944 ) ) ;
#3093=CARTESIAN_POINT ( 'NONE',  ( 5.405949406249999534, 9.363379034771803333, -49.28125000204838813 ) ) ;
#3096=CARTESIAN_POINT ( 'NONE',  ( -10.00000000000000000, -5.773502691896251982, -137.6250000000000000 ) ) ;
#3097=CARTESIAN_POINT ( 'NONE',  ( 5.405949406249999534, 9.363379034771803333, -139.2812500020483810 ) ) ;
#3098=CARTESIAN_POINT ( 'NONE',  ( 4.999999999999992006, -8.660254037844389075, -98.62500000409677625 ) ) ;
#3099=CARTESIAN_POINT ( 'NONE',  ( 4.999999999999992006, -8.660254037844389075, -116.6250000040967905 ) ) ;
#3105=CARTESIAN_POINT ( 'NONE',  ( -2.121150477449813534E-15, -11.54700538379251284, -140.7500000040967905 ) ) ;
#3106=CARTESIAN_POINT ( 'NONE',  ( -2.293366432827344421E-15, -12.48450537969573659, -175.9062500020483810 ) ) ;
#3107=CARTESIAN_POINT ( 'NONE',  ( 4.999999999999992006, -8.660254037844389075, -41.62500000409677625 ) ) ;
#3109=EDGE_CURVE ( 'NONE', #17742, #4273, #23718, .T. ) ;
#3111=CARTESIAN_POINT ( 'NONE',  ( 9.999999999999479527, 5.773502691896553074, -45.37499999999995737 ) ) ;
#3112=CARTESIAN_POINT ( 'NONE',  ( 5.405949406249999534, 9.363379034771803333, -160.2812500020484094 ) ) ;
#3113=CARTESIAN_POINT ( 'NONE',  ( -5.405949406249996869, 9.363379034771805109, -146.3437500020483810 ) ) ;
#3117=CARTESIAN_POINT ( 'NONE',  ( 9.999999999999998224, 0.000000000000000000, -30.49999999999997158 ) ) ;
#3118=CARTESIAN_POINT ( 'NONE',  ( 10.81189881249999551, -6.242252689847874514, -73.65625000204836681 ) ) ;
#3121=CARTESIAN_POINT ( 'NONE',  ( -5.405949406249996869, 9.363379034771805109, -120.8437500020483952 ) ) ;
#3122=ORIENTED_EDGE ( 'NONE', *, *, #36245, .F. ) ;
#3123=ORIENTED_EDGE ( 'NONE', *, *, #3935, .F. ) ;
#3125=CARTESIAN_POINT ( 'NONE',  ( -10.81189881249999729, 6.242252689847871849, -21.71875000204837036 ) ) ;
#3126=CARTESIAN_POINT ( 'NONE',  ( -5.405949406249996869, 9.363379034771805109, -1.031250002048372805 ) ) ;
#3127=CARTESIAN_POINT ( 'NONE',  ( -5.405949406250003975, -9.363379034771801557, -49.84375000204838102 ) ) ;
#3128=CARTESIAN_POINT ( 'NONE',  ( -5.000000000000003553, -8.660254037844383745, -71.87500000409677625 ) ) ;
#3130=CARTESIAN_POINT ( 'NONE',  ( -10.81189881249999729, 6.242252689847871849, -185.2187500020484379 ) ) ;
#3131=CARTESIAN_POINT ( 'NONE',  ( 5.405949406249999534, 9.363379034771803333, -166.0937500020484094 ) ) ;
#3137=CARTESIAN_POINT ( 'NONE',  ( -9.999999999999998224, 1.224646799147353059E-15, -19.62500000409675494 ) ) ;
#3139=CARTESIAN_POINT ( 'NONE',  ( 10.81189881249999551, -6.242252689847874514, -97.46875000204838102 ) ) ;
#3140=CARTESIAN_POINT ( 'NONE',  ( -9.999999999999998224, 1.224646799147353059E-15, -85.24999999999997158 ) ) ;
#3141=CARTESIAN_POINT ( 'NONE',  ( -10.81189881249999907, -6.242252689847864744, -75.65625000204839523 ) ) ;
#3142=DIRECTION ( 'NONE',  ( -0.000000000000000000, -0.000000000000000000, 1.000000000000000000 ) ) ;
#3144=CARTESIAN_POINT ( 'NONE',  ( -10.81189881249999729, 6.242252689847871849, -164.4062500020483810 ) ) ;
#3146=CARTESIAN_POINT ( 'NONE',  ( 5.000000000000000000, 8.660254037844385522, -140.1250000040967905 ) ) ;
#3151=CARTESIAN_POINT ( 'NONE',  ( 5.405949406249992428, -9.363379034771808662, -196.7812500020484094 ) ) ;
#3154=ORIENTED_EDGE ( 'NONE', *, *, #16310, .T. ) ;
#3155=CARTESIAN_POINT ( 'NONE',  ( 7.070501591499377789E-16, 11.54700538379251284, -54.12499999999997158 ) ) ;
#3157=CARTESIAN_POINT ( 'NONE',  ( 9.999999999999998224, 0.000000000000000000, -72.87500000409677625 ) ) ;
#3158=EDGE_CURVE ( 'NONE', #18128, #20886, #15127, .T. ) ;
#3159=CARTESIAN_POINT ( 'NONE',  ( 9.999999999998969713, 5.773502691896851502, -66.37499999999997158 ) ) ;
#3162=AXIS2_PLACEMENT_3D ( 'NONE', #7151, #10168, #4128 ) ;
#3163=CARTESIAN_POINT ( 'NONE',  ( 10.81189881249999551, -6.242252689847874514, -69.15625000204840944 ) ) ;
#3164=AXIS2_PLACEMENT_3D ( 'NONE', #18503, #2125, #15256 ) ;
#3168=CARTESIAN_POINT ( 'NONE',  ( -5.405949406249996869, 9.363379034771805109, -188.5312500020484094 ) ) ;
#3170=CARTESIAN_POINT ( 'NONE',  ( -5.405949406249996869, 9.363379034771805109, -0.8437500020483656993 ) ) ;
#3171=CARTESIAN_POINT ( 'NONE',  ( 9.999999999999998224, 0.000000000000000000, -110.3750000040967763 ) ) ;
#3174=CARTESIAN_POINT ( 'NONE',  ( -9.999999999999479527, -5.773502691896549521, -46.12499999999995026 ) ) ;
#3176=CARTESIAN_POINT ( 'NONE',  ( -2.121150477449813534E-15, -11.54700538379251284, -168.8750000000000000 ) ) ;
#3177=CARTESIAN_POINT ( 'NONE',  ( 5.000000000000000000, 8.660254037844385522, -166.7500000000000000 ) ) ;
#3178=CARTESIAN_POINT ( 'NONE',  ( 5.405949406249992428, -9.363379034771808662, -97.78125000204839523 ) ) ;
#3179=EDGE_LOOP ( 'NONE', ( #26005, #32252, #14720, #39877 ) ) ;
#3180=CARTESIAN_POINT ( 'NONE',  ( 9.999999999999998224, 0.000000000000000000, -162.5000000000000000 ) ) ;
#3182=ORIENTED_EDGE ( 'NONE', *, *, #26935, .F. ) ;
#3184=CARTESIAN_POINT ( 'NONE',  ( 7.644554776091147741E-16, 12.48450537969573659, -32.46875000204835970 ) ) ;
#3185=CARTESIAN_POINT ( 'NONE',  ( -2.293366432827344421E-15, -12.48450537969573659, -24.40625000204838457 ) ) ;
#3186=CARTESIAN_POINT ( 'NONE',  ( -10.81189881249999729, 1.324075727343319199E-15, -75.59375000204838102 ) ) ;
#3187=CARTESIAN_POINT ( 'NONE',  ( -5.000000000000003553, -8.660254037844383745, -83.87500000409677625 ) ) ;
#3188=CARTESIAN_POINT ( 'NONE',  ( -5.405949406249996869, 9.363379034771805109, -192.8437500020484094 ) ) ;
#3190=CARTESIAN_POINT ( 'NONE',  ( -4.999999999999996447, 8.660254037844387298, -72.37500000409677625 ) ) ;
#3193=CARTESIAN_POINT ( 'NONE',  ( 7.070501591499377789E-16, 11.54700538379251284, -5.000000004096767370 ) ) ;
#3194=CARTESIAN_POINT ( 'NONE',  ( -9.999999999999998224, 1.224646799147353059E-15, -130.2499999999999716 ) ) ;
#3195=CARTESIAN_POINT ( 'NONE',  ( -2.293366432827344421E-15, -12.48450537969573659, -124.7187500020483668 ) ) ;
#3196=CARTESIAN_POINT ( 'NONE',  ( 10.81189881249999907, 6.242252689847868297, -97.40625000204839523 ) ) ;
#3197=CARTESIAN_POINT ( 'NONE',  ( 5.405949406249992428, -9.363379034771808662, -111.0937500020483810 ) ) ;
#3200=CARTESIAN_POINT ( 'NONE',  ( 7.070501591499377789E-16, 11.54700538379251284, -165.5000000040967905 ) ) ;
#3201=DIRECTION ( 'NONE',  ( 1.000000000000000000, 0.000000000000000000, 0.000000000000000000 ) ) ;
#3207=CARTESIAN_POINT ( 'NONE',  ( -9.999999999999998224, 1.224646799147353059E-15, -127.2499999999999716 ) ) ;
#3209=CARTESIAN_POINT ( 'NONE',  ( 7.070501591499377789E-16, 11.54700538379251284, -82.62500000000000000 ) ) ;
#3211=CARTESIAN_POINT ( 'NONE',  ( -9.999999999999998224, 5.773502691896259087, -94.75000000409677625 ) ) ;
#3212=DIRECTION ( 'NONE',  ( -0.000000000000000000, -0.000000000000000000, 1.000000000000000000 ) ) ;
#3214=CARTESIAN_POINT ( 'NONE',  ( -5.405949406249996869, 9.363379034771805109, -92.53125000204838102 ) ) ;
#3215=ORIENTED_EDGE ( 'NONE', *, *, #6620, .F. ) ;
#3216=( BOUNDED_CURVE ( )  B_SPLINE_CURVE ( 2, ( #11619, #11839, #4521, #25040, #24827, #8417, #8626 ),
 .UNSPECIFIED., .F., .F. ) 
 B_SPLINE_CURVE_WITH_KNOTS ( ( 3, 2, 2, 3 ),
 ( 0.1679104477611940427, 0.1691542288557214002, 0.1703980099502487855, 0.1716417910447761430 ),
 .UNSPECIFIED. ) 
 CURVE ( )  GEOMETRIC_REPRESENTATION_ITEM ( )  RATIONAL_B_SPLINE_CURVE ( ( 1.000000000000000000, 0.8660254037844387076, 1.000000000000000000, 0.8660254037844387076, 1.000000000000000000, 0.8660254037844357100, 1.000000000000003109 ) ) 
 REPRESENTATION_ITEM ( '' )  );
#3220=ORIENTED_EDGE ( 'NONE', *, *, #29989, .F. ) ;
#3221=CARTESIAN_POINT ( 'NONE',  ( 9.999999999999996447, -5.773502691896262640, -12.62499999999996270 ) ) ;
#3222=EDGE_CURVE ( 'NONE', #38687, #3910, #19288, .T. ) ;
#3223=CARTESIAN_POINT ( 'NONE',  ( 10.00000000000000000, 5.773502691896255534, -144.3750000000000284 ) ) ;
#3226=CARTESIAN_POINT ( 'NONE',  ( 9.999999999999996447, -5.773502691896262640, -188.1250000000000284 ) ) ;
#3227=CARTESIAN_POINT ( 'NONE',  ( -5.405949406250003975, -9.363379034771801557, -116.0312500020483952 ) ) ;
#3230=ORIENTED_EDGE ( 'NONE', *, *, #36245, .T. ) ;
#3231=CARTESIAN_POINT ( 'NONE',  ( -5.405949406250003975, -9.363379034771801557, -42.53125000204838102 ) ) ;
#3233=CARTESIAN_POINT ( 'NONE',  ( 5.405949406249999534, 9.363379034771803333, -106.0937500020483810 ) ) ;
#3234=CARTESIAN_POINT ( 'NONE',  ( -10.81189881249999729, 6.242252689847871849, -125.4062500020483810 ) ) ;
#3235=ORIENTED_EDGE ( 'NONE', *, *, #33571, .T. ) ;
#3237=CARTESIAN_POINT ( 'NONE',  ( -9.999999999999998224, 1.224646799147353059E-15, -126.1250000040967620 ) ) ;
#3239=LINE ( 'NONE', #29147, #41974 ) ;
#3241=CARTESIAN_POINT ( 'NONE',  ( 10.81189881249999729, 6.242252689847867408, -133.2187500020483810 ) ) ;
#3243=CARTESIAN_POINT ( 'NONE',  ( -2.121150477449813534E-15, -11.54700538379251284, -158.3750000000000000 ) ) ;
#3245=CARTESIAN_POINT ( 'NONE',  ( -10.00000000000000000, -5.773502691896251982, -195.0000000040967905 ) ) ;
#3247=CARTESIAN_POINT ( 'NONE',  ( 5.405949406249999534, 9.363379034771803333, -185.7812500020484094 ) ) ;
#3248=CARTESIAN_POINT ( 'NONE',  ( -5.000000000000003553, -8.660254037844383745, -185.8750000040967905 ) ) ;
#3251=CARTESIAN_POINT ( 'NONE',  ( -10.81189881249999729, 1.324075727343319199E-15, -60.59375000204836681 ) ) ;
#3252=CARTESIAN_POINT ( 'NONE',  ( 10.81189881249999551, -6.242252689847874514, -47.96875000204836681 ) ) ;
#3255=CARTESIAN_POINT ( 'NONE',  ( 7.644554776091147741E-16, 12.48450537969573659, -22.15625000204837391 ) ) ;
#3259=CARTESIAN_POINT ( 'NONE',  ( -9.999999999999998224, 5.773502691896259087, -106.3749999999999858 ) ) ;
#3261=CYLINDRICAL_SURFACE ( 'NONE', #18288, 9.999999999999998224 ) ;
#3264=CARTESIAN_POINT ( 'NONE',  ( 10.81189881249999729, 6.242252689847867408, -118.4062500020483810 ) ) ;
#3265=EDGE_LOOP ( 'NONE', ( #20993, #9522, #25953, #23706 ) ) ;
#3266=CYLINDRICAL_SURFACE ( 'NONE', #20331, 9.999999999999998224 ) ;
#3269=ORIENTED_EDGE ( 'NONE', *, *, #15533, .F. ) ;
#3270=CARTESIAN_POINT ( 'NONE',  ( -4.999999999999996447, 8.660254037844387298, -44.99999999999998579 ) ) ;
#3271=CARTESIAN_POINT ( 'NONE',  ( -4.999999999999996447, 8.660254037844387298, -15.37500000409675138 ) ) ;
#3273=CARTESIAN_POINT ( 'NONE',  ( -10.81189881249999729, -6.242252689847864744, -42.65625000204837391 ) ) ;
#3278=CARTESIAN_POINT ( 'NONE',  ( -10.81189881249999907, -6.242252689847864744, -137.1562500020483810 ) ) ;
#3279=EDGE_CURVE ( 'NONE', #795, #25379, #31162, .T. ) ;
#3280=CARTESIAN_POINT ( 'NONE',  ( 5.405949406249992428, -9.363379034771808662, -139.7812500020483810 ) ) ;
#3283=ORIENTED_EDGE ( 'NONE', *, *, #35723, .T. ) ;
#3284=VERTEX_POINT ( 'NONE', #16460 ) ;
#3285=ORIENTED_EDGE ( 'NONE', *, *, #12511, .F. ) ;
#3286=CARTESIAN_POINT ( 'NONE',  ( 4.999999999999992006, -8.660254037844389075, -129.7499999999999716 ) ) ;
#3287=CARTESIAN_POINT ( 'NONE',  ( -2.293366432827344421E-15, -12.48450537969573659, -172.7187500020484094 ) ) ;
#3288=EDGE_CURVE ( 'NONE', #2291, #8915, #19541, .T. ) ;
#3289=CARTESIAN_POINT ( 'NONE',  ( 5.405949406249992428, -9.363379034771808662, -25.59375000204835970 ) ) ;
#3292=CARTESIAN_POINT ( 'NONE',  ( -5.405949406250003975, -9.363379034771801557, -153.3437500020483810 ) ) ;
#3293=CARTESIAN_POINT ( 'NONE',  ( 10.81189881249999551, -6.242252689847874514, -142.4687500020483810 ) ) ;
#3295=CARTESIAN_POINT ( 'NONE',  ( -9.999999999998456346, -5.773502691897145489, -10.12499999999994671 ) ) ;
#3298=CARTESIAN_POINT ( 'NONE',  ( -2.293366432827344421E-15, -12.48450537969573659, -21.21875000204837036 ) ) ;
#3300=FACE_OUTER_BOUND ( 'NONE', #20729, .T. ) ;
#3302=CARTESIAN_POINT ( 'NONE',  ( -10.00000000000051337, 5.773502691895962435, -99.25000000409679046 ) ) ;
#3303=CARTESIAN_POINT ( 'NONE',  ( 5.405949406249992428, -9.363379034771808662, -76.59375000204838102 ) ) ;
#3304=CARTESIAN_POINT ( 'NONE',  ( -10.81189881249999907, -6.242252689847864744, -42.65625000204837391 ) ) ;
#3306=DIRECTION ( 'NONE',  ( -0.000000000000000000, -0.000000000000000000, 1.000000000000000000 ) ) ;
#3308=CARTESIAN_POINT ( 'NONE',  ( 9.999999999999998224, 0.000000000000000000, -128.0000000000000000 ) ) ;
#3309=CARTESIAN_POINT ( 'NONE',  ( 7.644554776091147741E-16, 12.48450537969573659, -134.6562500020483810 ) ) ;
#3310=CARTESIAN_POINT ( 'NONE',  ( -9.999999999999998224, 1.224646799147353059E-15, -151.2500000000000000 ) ) ;
#3311=CARTESIAN_POINT ( 'NONE',  ( -9.999999999999998224, 5.773502691896259087, -115.7500000040967763 ) ) ;
#3313=VERTEX_POINT ( 'NONE', #26204 ) ;
#3316=CARTESIAN_POINT ( 'NONE',  ( -10.81189881249999729, 6.242252689847871849, -170.4062500020484094 ) ) ;
#3317=CARTESIAN_POINT ( 'NONE',  ( 7.070501591499377789E-16, 11.54700538379251284, -42.50000000409675494 ) ) ;
#3320=CARTESIAN_POINT ( 'NONE',  ( -9.999999999999998224, 1.224646799147353059E-15, -124.2500000000000000 ) ) ;
#3321=CARTESIAN_POINT ( 'NONE',  ( 5.405949406249999534, 9.363379034771803333, -157.2812500020484094 ) ) ;
#3322=CARTESIAN_POINT ( 'NONE',  ( 10.81189881249999729, 0.000000000000000000, -139.3437500020484094 ) ) ;
#3324=DIRECTION ( 'NONE',  ( 1.000000000000000000, 0.000000000000000000, 0.000000000000000000 ) ) ;
#3325=CARTESIAN_POINT ( 'NONE',  ( -9.999999999999998224, 1.224646799147353059E-15, -79.24999999999998579 ) ) ;
#3326=AXIS2_PLACEMENT_3D ( 'NONE', #16008, #16214, #36518 ) ;
#3327=ORIENTED_EDGE ( 'NONE', *, *, #4709, .T. ) ;
#3329=ADVANCED_FACE ( 'NONE', ( #6357 ), #20144, .T. ) ;
#3330=CARTESIAN_POINT ( 'NONE',  ( -10.81189881249999907, -6.242252689847864744, -69.65625000204839523 ) ) ;
#3331=ORIENTED_EDGE ( 'NONE', *, *, #19158, .T. ) ;
#3333=CARTESIAN_POINT ( 'NONE',  ( -10.81189881249999907, -6.242252689847864744, -115.9687500020483810 ) ) ;
#3336=CARTESIAN_POINT ( 'NONE',  ( -2.293366432827344421E-15, -12.48450537969573659, -24.21875000204836326 ) ) ;
#3337=( BOUNDED_CURVE ( )  B_SPLINE_CURVE ( 2, ( #37639, #33985, #27931, #1392, #37853, #27500, #2038 ),
 .UNSPECIFIED., .F., .F. ) 
 B_SPLINE_CURVE_WITH_KNOTS ( ( 3, 2, 2, 3 ),
 ( 0.4291044776119404269, 0.4303482587064677567, 0.4315920398009951975, 0.4328358208955225273 ),
 .UNSPECIFIED. ) 
 CURVE ( )  GEOMETRIC_REPRESENTATION_ITEM ( )  RATIONAL_B_SPLINE_CURVE ( ( 0.9999999999999880096, 0.8660254037844506980, 1.000000000000000000, 0.8660254037844387076, 1.000000000000000000, 0.8660254037844207220, 1.000000000000017986 ) ) 
 REPRESENTATION_ITEM ( '' )  );
#3338=CARTESIAN_POINT ( 'NONE',  ( -10.81189881249999907, -6.242252689847864744, -0.6562500020483670315 ) ) ;
#3339=CARTESIAN_POINT ( 'NONE',  ( 10.81189881249999729, 0.000000000000000000, -44.84375000204837391 ) ) ;
#3340=CARTESIAN_POINT ( 'NONE',  ( 9.999999999999998224, 0.000000000000000000, -200.0000000000000000 ) ) ;
#3342=CARTESIAN_POINT ( 'NONE',  ( -2.293366432827344421E-15, -12.48450537969573659, -183.2187500020484094 ) ) ;
#3343=CARTESIAN_POINT ( 'NONE',  ( 10.81189881249999551, -6.242252689847874514, -169.4687500020483810 ) ) ;
#3347=( BOUNDED_CURVE ( )  B_SPLINE_CURVE ( 2, ( #30566, #24513, #33589, #14553, #27102, #37666, #4224 ),
 .UNSPECIFIED., .F., .F. ) 
 B_SPLINE_CURVE_WITH_KNOTS ( ( 3, 2, 2, 3 ),
 ( 0.6231343283582090331, 0.6243781094527364184, 0.6256218905472638037, 0.6268656716417911889 ),
 .UNSPECIFIED. ) 
 CURVE ( )  GEOMETRIC_REPRESENTATION_ITEM ( )  RATIONAL_B_SPLINE_CURVE ( ( 0.9999999999999880096, 0.8660254037844506980, 1.000000000000000000, 0.8660254037844387076, 1.000000000000000000, 0.8660254037844267172, 1.000000000000011990 ) ) 
 REPRESENTATION_ITEM ( '' )  );
#3349=CARTESIAN_POINT ( 'NONE',  ( -10.81189881249999907, -6.242252689847864744, -93.46875000204836681 ) ) ;
#3350=CARTESIAN_POINT ( 'NONE',  ( 5.000000000000000000, 8.660254037844385522, -198.6250000040967905 ) ) ;
#3351=CARTESIAN_POINT ( 'NONE',  ( 5.405949406249999534, 9.363379034771803333, -62.78125000204837391 ) ) ;
#3352=CARTESIAN_POINT ( 'NONE',  ( 9.999999999999994671, -5.773502691896262640, -131.5000000040967905 ) ) ;
#3354=AXIS2_PLACEMENT_3D ( 'NONE', #14912, #21622, #11677 ) ;
#3355=CARTESIAN_POINT ( 'NONE',  ( 5.405949406249992428, -9.363379034771808662, -163.7812500020484094 ) ) ;
#3357=CARTESIAN_POINT ( 'NONE',  ( -9.999999999999998224, 1.224646799147353059E-15, -138.1250000040967620 ) ) ;
#3359=ORIENTED_EDGE ( 'NONE', *, *, #11801, .F. ) ;
#3362=CARTESIAN_POINT ( 'NONE',  ( -5.405949406249996869, 9.363379034771805109, -196.0312500020484094 ) ) ;
#3365=ORIENTED_EDGE ( 'NONE', *, *, #14669, .T. ) ;
#3366=CARTESIAN_POINT ( 'NONE',  ( 4.999999999999992006, -8.660254037844389075, -56.24999999999996447 ) ) ;
#3368=CARTESIAN_POINT ( 'NONE',  ( -9.999999999999998224, 1.224646799147353059E-15, -67.62500000409676204 ) ) ;
#3369=CARTESIAN_POINT ( 'NONE',  ( -10.00000000000154188, 5.773502691895366468, -12.25000000409673184 ) ) ;
#3371=CARTESIAN_POINT ( 'NONE',  ( -5.405949406250003975, -9.363379034771801557, -63.53125000204837391 ) ) ;
#3374=CYLINDRICAL_SURFACE ( 'NONE', #18662, 9.999999999999998224 ) ;
#3375=CARTESIAN_POINT ( 'NONE',  ( -10.81189881249999907, -6.242252689847864744, -186.6562500020484094 ) ) ;
#3377=CARTESIAN_POINT ( 'NONE',  ( -10.00000000000051337, 5.773502691895962435, -40.37499999999996447 ) ) ;
#3378=FACE_OUTER_BOUND ( 'NONE', #6460, .T. ) ;
#3381=CARTESIAN_POINT ( 'NONE',  ( 7.070501591499377789E-16, 11.54700538379251284, -169.6250000000000000 ) ) ;
#3382=CARTESIAN_POINT ( 'NONE',  ( -5.000000000000003553, -8.660254037844383745, -62.49999999999997158 ) ) ;
#3383=CARTESIAN_POINT ( 'NONE',  ( -10.81189881249999729, 6.242252689847871849, -90.90625000204838102 ) ) ;
#3384=ORIENTED_EDGE ( 'NONE', *, *, #5674, .F. ) ;
#3385=CARTESIAN_POINT ( 'NONE',  ( 0.000000000000000000, 0.000000000000000000, -200.0000000000000000 ) ) ;
#3386=AXIS2_PLACEMENT_3D ( 'NONE', #25176, #5097, #29038 ) ;
#3387=EDGE_LOOP ( 'NONE', ( #39891, #19721, #3869, #2794 ) ) ;
#3388=EDGE_LOOP ( 'NONE', ( #29268, #29544, #38794, #1702 ) ) ;
#3389=CARTESIAN_POINT ( 'NONE',  ( -5.405949406249996869, 9.363379034771805109, -30.84375000204836326 ) ) ;
#3390=CARTESIAN_POINT ( 'NONE',  ( 10.81189881249999551, -6.242252689847874514, -25.65625000204839168 ) ) ;
#3392=CARTESIAN_POINT ( 'NONE',  ( 5.405949406249999534, 9.363379034771803333, -73.09375000204838102 ) ) ;
#3393=DIRECTION ( 'NONE',  ( -0.000000000000000000, -0.000000000000000000, 1.000000000000000000 ) ) ;
#3394=CARTESIAN_POINT ( 'NONE',  ( -10.81189881249999729, 6.242252689847871849, -189.7187500020484379 ) ) ;
#3395=CARTESIAN_POINT ( 'NONE',  ( -2.293366432827344421E-15, -12.48450537969573659, -153.2187500020483810 ) ) ;
#3396=EDGE_CURVE ( 'NONE', #3609, #16045, #19502, .T. ) ;
#3397=CARTESIAN_POINT ( 'NONE',  ( -5.000000000000003553, -8.660254037844383745, -79.37500000409677625 ) ) ;
#3401=CARTESIAN_POINT ( 'NONE',  ( -2.121150477449813534E-15, -11.54700538379251284, -1.250000004096749828 ) ) ;
#3403=CARTESIAN_POINT ( 'NONE',  ( -5.405949406249996869, 9.363379034771805109, -119.3437500020483810 ) ) ;
#3404=CARTESIAN_POINT ( 'NONE',  ( 7.644554776091147741E-16, 12.48450537969573659, -95.65625000204838102 ) ) ;
#3405=CARTESIAN_POINT ( 'NONE',  ( 10.81189881249999729, 0.000000000000000000, -106.3437500020483810 ) ) ;
#3408=CARTESIAN_POINT ( 'NONE',  ( 9.999999999999998224, 0.000000000000000000, -161.3750000040967905 ) ) ;
#3409=CARTESIAN_POINT ( 'NONE',  ( 7.070501591499376803E-16, 11.54700538379251284, -81.50000000409677625 ) ) ;
#3417=CARTESIAN_POINT ( 'NONE',  ( -9.999999999999998224, 1.224646799147353059E-15, -77.74999999999998579 ) ) ;
#3419=CARTESIAN_POINT ( 'NONE',  ( 4.999999999999992006, -8.660254037844389075, -91.12500000409677625 ) ) ;
#3420=( BOUNDED_CURVE ( )  B_SPLINE_CURVE ( 2, ( #38062, #15165, #15379, #28363, #8929, #33080, #13405 ),
 .UNSPECIFIED., .F., .F. ) 
 B_SPLINE_CURVE_WITH_KNOTS ( ( 3, 2, 2, 3 ),
 ( 0.08208955223880604057, 0.08333333333333339810, 0.08457711442786078337, 0.08582089552238814090 ),
 .UNSPECIFIED. ) 
 CURVE ( )  GEOMETRIC_REPRESENTATION_ITEM ( )  RATIONAL_B_SPLINE_CURVE ( ( 0.9999999999999924505, 0.8660254037844461461, 1.000000000000000000, 0.8660254037844387076, 1.000000000000000000, 0.8660254037844297148, 1.000000000000008882 ) ) 
 REPRESENTATION_ITEM ( '' )  );
#3422=CARTESIAN_POINT ( 'NONE',  ( 5.405949406249992428, -9.363379034771808662, -88.78125000204838102 ) ) ;
#3423=ORIENTED_EDGE ( 'NONE', *, *, #31811, .T. ) ;
#3427=ORIENTED_EDGE ( 'NONE', *, *, #18315, .F. ) ;
#3428=CARTESIAN_POINT ( 'NONE',  ( -9.999999999999998224, 1.224646799147353059E-15, -11.74999999999995559 ) ) ;
#3429=EDGE_CURVE ( 'NONE', #32487, #7438, #6080, .T. ) ;
#3430=CARTESIAN_POINT ( 'NONE',  ( 5.000000000000000000, 8.660254037844385522, -142.7500000000000000 ) ) ;
#3431=CARTESIAN_POINT ( 'NONE',  ( 0.000000000000000000, 0.000000000000000000, -200.0000000000000000 ) ) ;
#3434=CARTESIAN_POINT ( 'NONE',  ( -10.00000000000000000, -5.773502691896251982, -187.1250000000000284 ) ) ;
#3435=CARTESIAN_POINT ( 'NONE',  ( 10.81189881249999551, -6.242252689847874514, -120.1562500020483810 ) ) ;
#3436=ORIENTED_EDGE ( 'NONE', *, *, #39059, .T. ) ;
#3437=CARTESIAN_POINT ( 'NONE',  ( 9.999999999999998224, 0.000000000000000000, -74.37500000409677625 ) ) ;
#3438=ORIENTED_EDGE ( 'NONE', *, *, #32558, .T. ) ;
#3439=CARTESIAN_POINT ( 'NONE',  ( 10.81189881249999907, 6.242252689847868297, -43.40625000204837391 ) ) ;
#3441=CARTESIAN_POINT ( 'NONE',  ( -10.81189881249999729, 1.324075727343319199E-15, -93.59375000204838102 ) ) ;
#3442=CARTESIAN_POINT ( 'NONE',  ( -5.405949406249996869, 9.363379034771805109, -127.0312500020483952 ) ) ;
#3443=ORIENTED_EDGE ( 'NONE', *, *, #13647, .T. ) ;
#3444=CARTESIAN_POINT ( 'NONE',  ( 9.999999999999998224, 0.000000000000000000, -200.0000000000000000 ) ) ;
#3445=CARTESIAN_POINT ( 'NONE',  ( 10.00000000000025402, -5.773502691896113426, -125.5000000040967763 ) ) ;
#3449=CARTESIAN_POINT ( 'NONE',  ( -5.405949406249996869, 9.363379034771805109, -132.8437500020484094 ) ) ;
#3453=CARTESIAN_POINT ( 'NONE',  ( -2.121150477449813534E-15, -11.54700538379251284, -182.7500000040967905 ) ) ;
#3455=CARTESIAN_POINT ( 'NONE',  ( 5.405949406249999534, 9.363379034771803333, -187.2812500020484094 ) ) ;
#3457=CARTESIAN_POINT ( 'NONE',  ( -10.00000000000051337, 5.773502691895962435, -6.250000004096728290 ) ) ;
#3461=CARTESIAN_POINT ( 'NONE',  ( 7.644554776091147741E-16, 12.48450537969573659, -56.46875000204837391 ) ) ;
#3462=CARTESIAN_POINT ( 'NONE',  ( 5.405949406249999534, 9.363379034771803333, -47.59375000204838102 ) ) ;
#3464=CARTESIAN_POINT ( 'NONE',  ( -10.81189881249999729, 1.324075727343319199E-15, -20.28125000204836326 ) ) ;
#3466=CARTESIAN_POINT ( 'NONE',  ( -9.999999999999998224, 1.224646799147353059E-15, -145.2500000000000000 ) ) ;
#3468=CARTESIAN_POINT ( 'NONE',  ( 10.00000000000000000, 5.773502691896255534, -102.3749999999999858 ) ) ;
#3470=FACE_OUTER_BOUND ( 'NONE', #14717, .T. ) ;
#3473=CARTESIAN_POINT ( 'NONE',  ( -10.81189881249999729, 1.324075727343319199E-15, -113.2812500020483952 ) ) ;
#3474=ORIENTED_EDGE ( 'NONE', *, *, #8536, .F. ) ;
#3480=CARTESIAN_POINT ( 'NONE',  ( -10.00000000000000000, -5.773502691896251982, -31.12499999999995381 ) ) ;
#3481=CARTESIAN_POINT ( 'NONE',  ( -9.999999999999998224, 5.773502691896259087, -21.25000000409676204 ) ) ;
#3482=CARTESIAN_POINT ( 'NONE',  ( 5.405949406249999534, 9.363379034771803333, -40.28125000204838102 ) ) ;
#3483=CARTESIAN_POINT ( 'NONE',  ( 10.00000000000102318, -5.773502691895667560, -2.124999999999920064 ) ) ;
#3486=AXIS2_PLACEMENT_3D ( 'NONE', #5561, #22176, #6410 ) ;
#3487=CARTESIAN_POINT ( 'NONE',  ( 5.405949406249999534, 9.363379034771803333, -145.2812500020483810 ) ) ;
#3488=CARTESIAN_POINT ( 'NONE',  ( -9.999999999999998224, 1.224646799147353059E-15, -16.24999999999995737 ) ) ;
#3490=VERTEX_POINT ( 'NONE', #23395 ) ;
#3491=ORIENTED_EDGE ( 'NONE', *, *, #5970, .T. ) ;
#3492=CARTESIAN_POINT ( 'NONE',  ( 9.999999999999998224, 0.000000000000000000, -200.0000000000000000 ) ) ;
#3493=CARTESIAN_POINT ( 'NONE',  ( -5.405949406250003975, -9.363379034771801557, -171.3437500020484094 ) ) ;
#3494=CARTESIAN_POINT ( 'NONE',  ( 10.81189881249999907, 6.242252689847868297, -23.71875000204836326 ) ) ;
#3496=ADVANCED_FACE ( 'NONE', ( #16037 ), #29232, .T. ) ;
#3497=CARTESIAN_POINT ( 'NONE',  ( 10.81189881249999729, 6.242252689847867408, -152.7187500020483810 ) ) ;
#3498=CARTESIAN_POINT ( 'NONE',  ( 10.81189881249999729, 0.000000000000000000, -148.3437500020483810 ) ) ;
#3499=EDGE_CURVE ( 'NONE', #107, #10156, #14500, .T. ) ;
#3500=CARTESIAN_POINT ( 'NONE',  ( -5.000000000000003553, -8.660254037844383745, -88.37500000409677625 ) ) ;
#3503=CARTESIAN_POINT ( 'NONE',  ( 5.405949406249992428, -9.363379034771808662, -7.593750002048343717 ) ) ;
#3507=CARTESIAN_POINT ( 'NONE',  ( -9.999999999999998224, 1.224646799147353059E-15, -200.0000000000000000 ) ) ;
#3509=CARTESIAN_POINT ( 'NONE',  ( -4.999999999999996447, 8.660254037844387298, -99.37500000409679046 ) ) ;
#3511=CARTESIAN_POINT ( 'NONE',  ( 10.81189881249999729, 0.000000000000000000, -73.34375000204838102 ) ) ;
#3512=CARTESIAN_POINT ( 'NONE',  ( 10.81189881249999907, 6.242252689847868297, -44.90625000204836681 ) ) ;
#3514=LINE ( 'NONE', #290, #32334 ) ;
#3516=CARTESIAN_POINT ( 'NONE',  ( 4.999999999999992006, -8.660254037844389075, -126.7499999999999716 ) ) ;
#3517=CARTESIAN_POINT ( 'NONE',  ( -10.81189881249999729, 6.242252689847871849, -137.4062500020484094 ) ) ;
#3519=DIRECTION ( 'NONE',  ( -0.000000000000000000, -0.000000000000000000, 1.000000000000000000 ) ) ;
#3520=CARTESIAN_POINT ( 'NONE',  ( 10.00000000000000000, 5.773502691896255534, -117.7500000040967905 ) ) ;
#3522=ORIENTED_EDGE ( 'NONE', *, *, #4036, .T. ) ;
#3525=CARTESIAN_POINT ( 'NONE',  ( 9.999999999999998224, 0.000000000000000000, -185.0000000000000000 ) ) ;
#3526=CARTESIAN_POINT ( 'NONE',  ( 5.405949406249999534, 9.363379034771803333, -166.2812500020484094 ) ) ;
#3527=CARTESIAN_POINT ( 'NONE',  ( -5.000000000000003553, -8.660254037844383745, -44.87500000409677625 ) ) ;
#3528=EDGE_CURVE ( 'NONE', #6885, #20093, #7452, .T. ) ;
#3529=CYLINDRICAL_SURFACE ( 'NONE', #2176, 9.999999999999998224 ) ;
#3531=DIRECTION ( 'NONE',  ( -0.000000000000000000, -0.000000000000000000, 1.000000000000000000 ) ) ;
#3532=CARTESIAN_POINT ( 'NONE',  ( 10.81189881249999551, -6.242252689847874514, -162.1562500020484379 ) ) ;
#3534=CARTESIAN_POINT ( 'NONE',  ( 10.81189881249999907, 6.242252689847868297, -137.7187500020484094 ) ) ;
#3535=CARTESIAN_POINT ( 'NONE',  ( 9.999999999999998224, 0.000000000000000000, -158.0000000000000000 ) ) ;
#3536=CARTESIAN_POINT ( 'NONE',  ( 9.999999999999998224, 0.000000000000000000, -150.5000000000000000 ) ) ;
#3537=ADVANCED_FACE ( 'NONE', ( #36971 ), #945, .T. ) ;
#3538=ORIENTED_EDGE ( 'NONE', *, *, #35604, .F. ) ;
#3539=CARTESIAN_POINT ( 'NONE',  ( -10.00000000000076916, 5.773502691895813221, -114.2500000040967905 ) ) ;
#3541=CARTESIAN_POINT ( 'NONE',  ( -10.81189881249999729, 1.324075727343319199E-15, -66.78125000204838102 ) ) ;
#3544=CARTESIAN_POINT ( 'NONE',  ( -10.81189881249999729, 6.242252689847871849, -122.2187500020483810 ) ) ;
#3545=VERTEX_POINT ( 'NONE', #21206 ) ;
#3546=EDGE_CURVE ( 'NONE', #34431, #19091, #738, .T. ) ;
#3547=( BOUNDED_CURVE ( )  B_SPLINE_CURVE ( 2, ( #22379, #36806, #13691 ),
 .UNSPECIFIED., .F., .F. ) 
 B_SPLINE_CURVE_WITH_KNOTS ( ( 3, 3 ),
 ( 0.9888059701492539766, 0.9894244334336458335 ),
 .UNSPECIFIED. ) 
 CURVE ( )  GEOMETRIC_REPRESENTATION_ITEM ( )  RATIONAL_B_SPLINE_CURVE ( ( 0.9999999999999761302, 0.9333818714843358233, 0.9330147364001334376 ) ) 
 REPRESENTATION_ITEM ( '' )  );
#3548=ORIENTED_EDGE ( 'NONE', *, *, #31857, .F. ) ;
#3549=CARTESIAN_POINT ( 'NONE',  ( 5.405949406249992428, -9.363379034771808662, -19.59375000204835615 ) ) ;
#3550=CARTESIAN_POINT ( 'NONE',  ( -5.405949406250003975, -9.363379034771801557, -0.5312500020483723606 ) ) ;
#3551=AXIS2_PLACEMENT_3D ( 'NONE', #18996, #32180, #28298 ) ;
#3552=CARTESIAN_POINT ( 'NONE',  ( -10.81189881249999907, -6.242252689847864744, -43.96875000204835970 ) ) ;
#3553=CARTESIAN_POINT ( 'NONE',  ( -9.999999999999998224, 1.224646799147353059E-15, -89.74999999999998579 ) ) ;
#3555=CARTESIAN_POINT ( 'NONE',  ( 7.644554776091147741E-16, 12.48450537969573659, -182.4687500020484094 ) ) ;
#3556=CARTESIAN_POINT ( 'NONE',  ( -10.81189881249999729, 1.324075727343319199E-15, -167.0937500020484094 ) ) ;
#3559=ADVANCED_FACE ( 'NONE', ( #24685 ), #24468, .T. ) ;
#3561=CARTESIAN_POINT ( 'NONE',  ( 9.999999999999884537, 5.773502691896319483, -194.2500000040968189 ) ) ;
#3563=CARTESIAN_POINT ( 'NONE',  ( -2.293366432827344421E-15, -12.48450537969573659, -93.21875000204838102 ) ) ;
#3565=CARTESIAN_POINT ( 'NONE',  ( 10.81189881249999729, 0.000000000000000000, -69.03125000204838102 ) ) ;
#3568=CARTESIAN_POINT ( 'NONE',  ( 10.81189881249999551, -6.242252689847874514, -121.6562500020483952 ) ) ;
#3569=CARTESIAN_POINT ( 'NONE',  ( -10.81189881249999729, 6.242252689847871849, -161.4062500020483810 ) ) ;
#3571=CARTESIAN_POINT ( 'NONE',  ( 5.000000000000000000, 8.660254037844385522, -141.6250000040967905 ) ) ;
#3573=VECTOR ( 'NONE', #36462, 1000.000000000000000 ) ;
#3578=CARTESIAN_POINT ( 'NONE',  ( 5.405949406249999534, 9.363379034771803333, -185.7812500020484094 ) ) ;
#3579=CARTESIAN_POINT ( 'NONE',  ( 5.000000000000000000, 8.660254037844385522, -131.1250000040967620 ) ) ;
#3581=ORIENTED_EDGE ( 'NONE', *, *, #17700, .F. ) ;
#3582=CARTESIAN_POINT ( 'NONE',  ( -4.999999999999996447, 8.660254037844387298, -59.99999999999997158 ) ) ;
#3584=CARTESIAN_POINT ( 'NONE',  ( 9.999999999999996447, -5.773502691896262640, -70.00000000409679046 ) ) ;
#3586=FACE_OUTER_BOUND ( 'NONE', #2443, .T. ) ;
#3588=CARTESIAN_POINT ( 'NONE',  ( 5.405949406249999534, 9.363379034771803333, -62.78125000204837391 ) ) ;
#3590=EDGE_CURVE ( 'NONE', #19091, #33541, #1590, .T. ) ;
#3594=CARTESIAN_POINT ( 'NONE',  ( 10.81189881249999551, -6.242252689847874514, -184.6562500020484094 ) ) ;
#3595=VECTOR ( 'NONE', #2485, 1000.000000000000000 ) ;
#3597=CARTESIAN_POINT ( 'NONE',  ( -4.999999999999996447, 8.660254037844387298, -40.49999999999997868 ) ) ;
#3602=CARTESIAN_POINT ( 'NONE',  ( 4.999999999999992006, -8.660254037844389075, -168.7500000000000000 ) ) ;
#3603=CARTESIAN_POINT ( 'NONE',  ( -9.999999999999998224, 1.224646799147353059E-15, -138.1250000040967620 ) ) ;
#3604=CARTESIAN_POINT ( 'NONE',  ( 5.405949406249999534, 9.363379034771803333, -92.78125000204838102 ) ) ;
#3605=VERTEX_POINT ( 'NONE', #30519 ) ;
#3606=CARTESIAN_POINT ( 'NONE',  ( 9.999999999999998224, 0.000000000000000000, -83.37500000409677625 ) ) ;
#3607=CARTESIAN_POINT ( 'NONE',  ( -9.999999999999479527, -5.773502691896549521, -70.12499999999998579 ) ) ;
#3608=ORIENTED_EDGE ( 'NONE', *, *, #2495, .T. ) ;
#3609=VERTEX_POINT ( 'NONE', #11483 ) ;
#3610=CARTESIAN_POINT ( 'NONE',  ( 10.81189881249999907, 6.242252689847868297, -34.21875000204835260 ) ) ;
#3611=CARTESIAN_POINT ( 'NONE',  ( -10.81189881249999729, 1.324075727343319199E-15, -18.78125000204835970 ) ) ;
#3612=( BOUNDED_CURVE ( )  B_SPLINE_CURVE ( 2, ( #27385, #11768, #27169, #33870, #30212, #8344, #21705, #38111, #38321, #26954, #10541, #28197, #17014, #20263, #1872, #40521, #24969, #31436, #41330, #8555, #33451, #4084, #40109, #5311, #18463, #23727, #30631, #30426, #31651, #36878, #14186, #7322, #18245, #2085, #7532, #37089, #28414, #15215, #857, #41552, #11983, #20472, #25179, #10965, #24754, #3879, #40312, #4296, #648, #21495, #33660, #13974, #10752, #23944, #20685, #37901, #34677, #5099, #32495, #29041, #12820, #26011, #31870, #41756, #39163, #35311, #28625, #35930, #22770, #2301, #5953, #5741, #29244, #12191, #2709, #15427, #25382, #38529, #32285, #9595, #18894, #32074, #22137, #38748, #25800, #6161, #22555, #2923, #8971, #16053, #19103, #32699, #35731, #6371, #2509, #15633, #28835, #19301, #41966, #19515, #15841, #16259, #12400, #9177, #42179, #12606, #25593, #22348, #26220, #35524, #42388, #38956, #9390, #3130, #29458, #42601, #13027, #8762, #21918, #35098, #5523, #18673, #36558, #36771, #958, #39369, #6784, #325, #29673, #3342, #7208, #20360, #33550, #16474, #17328, #3555, #117, #19728, #13239, #33128, #3975, #17115, #30531, #36351, #40210, #30315, #9805, #13658, #40004, #16899, #26426, #750, #19939, #30101, #3766, #16689, #23626, #13872, #36985, #39577, #27067, #10642, #10012, #23833, #23190, #7004, #14076, #29885, #7421, #13444, #26640, #20571, #22984, #33761, #32909, #4184, #39789, #36141, #20155, #10222, #23409, #6572, #33345, #540, #26849, #10435, #27491, #7856, #8068, #20787, #34403, #31595, #8496, #4612, #14727, #27273, #34830, #18188, #34194, #7637, #4822, #30737, #31380, #11067, #21218, #17536, #41274, #5043, #28141, #11494, #1814, #14941, #2028, #27919, #21649, #11282, #10856, #11710, #37843, #24909, #38056, #8285, #24268, #21432, #5254, #17969, #18406, #1598, #37188, #24477, #31169, #37628, #40411, #33976, #24047, #41050, #40625, #4397, #40843, #37414, #1168, #24697, #21005, #34617, #14291, #17753, #30948, #1381, #14511, #27705, #35044, #42336, #29196, #8711, #12345, #12139, #35679, #5471, #9128, #21865, #31817, #39108, #18621, #19466, #11927, #41701, #28571, #2449, #32232, #12559, #28988, #38906, #2251, #9335, #25544, #9545, #42127, #2871, #25332, #15371, #38477, #22504, #8921, #28783, #25753, #6107, #22083, #2658, #5692, #35470, #35258, #15792, #18841, #12766, #25960, #32022, #15582, #19254, #41914, #38694, #22298, #32444, #16001, #22719, #5894, #35884, #19050, #6319, #38264, #32651, #15157, #28355, #41493, #25120, #36719, #29618, #39739, #36089, #17064, #23572, #3927, #9755, #7158, #26379, #36511, #10174, #23139, #30047, #494, #701, #33071, #19888, #10591, #13608, #61, #26801, #40160, #26588, #30262, #20103, #12972, #20310, #9961, #16636, #26169, #33294, #13820, #33503, #20521, #39316, #6524, #10383, #42548, #3079, #39951, #23359, #27013, #23778, #36931, #7375, #16206, #13186, #22936, #29408, #19674, #32861, #275, #39530, #3292, #16420, #6948, #36303, #6733, #3497, #3720, #29838, #13396, #16849, #24859, #30895, #4772, #31117, #17920, #14683, #7586, #27870, #1332, #14896, #1550, #21385, #17491, #20739, #37138, #41004, #27442, #18140, #27653, #34568, #11448, #33926, #24648, #40794, #4350, #14240, #8454, #30684, #4560, #37791, #8236, #1115, #21166, #24214, #11235, #40364, #34354, #37365, #31336, #1767, #7808, #40579, #4999, #20956, #23997, #10805, #28095, #41222, #11660, #11020, #38009, #34142, #17701, #14024, #14463, #24434, #33709, #37577, #8022, #4134, #17275, #30480, #909, #27219, #22249, #41862, #28303, #25705, #2194, #12300, #28736, #41657, #5845, #19001, #19208, #8873, #38431, #29150, #32186, #5426, #2613, #15952, #2403, #15743, #18787, #25497, #12512, #28525, #35209, #31549, #25074, #15328, #22037, #32397, #5639, #21817, #2820, #35419, #15534, #34998, #28943, #38646, #38856, #9282, #34784, #31976, #12093, #31766, #42080, #1982, #22454, #18578, #42289, #9081, #15108, #25908, #35631, #6058, #12710, #41441, #39060, #18360, #25286, #21605, #5205, #11878, #38219, #8664, #17017, #3669, #32810, #443, #6479, #29355, #19625, #36253, #13560, #13772, #6896, #7112, #12922, #26751, #30215, #39271, #33243, #16159, #19835, #26957, #9705, #36460, #42494, #3241, #20266, #23305, #3449, #22884, #10127, #16585, #39903, #32607, #26116, #10334, #36043, #36671, #23522, #3032, #6683, #16367, #29997, #29566, #29787, #12, #13135, #26331, #33019, #33454, #39482, #3882, #652, #228, #20049, #9915, #16798, #9498, #23091, #22666, #13350, #35838, #6270, #19416, #26541, #39690, #860, #7966, #33875, #24591, #34084, #27820, #17868, #27173, #21115, #4088, #7756, #20689, #14841, #13976, #4719, #23948, #10968, #37525, #24383, #40315, #27604, #30634, #17649, #17228, #40744, #1066, #37740, #8184, #14189, #10756, #31064, #27388, #30430, #37092, #34303, #1497, #14632, #7535, #18090, #4299, #17438, #20476, #40525, #24164, #40953, #37310, #20901, #11397, #4506, #30844, #1281, #14410, #11186, #21331, #34520, #4943, #31284, #1714, #40112, #10545, #23730, #36881, #7326, #33663, #2143, #35583, #38591, #11825, #9032, #22406, #8822, #22196, #25235, #35157, #18950, #34945, #41607, #37958, #42030, #12041, #38381, #15278, #21554, #18307, #35371, #5798, #28252, #8612, #21978, #34734, #5583, #32137, #5156, #6012, #5370, #31496, #8403, #1928, #21767, #25446, #25025, #15055, #2568, #38168, #18736, #41390, #12460, #15697, #28896, #12253, #25653, #18523, #31928, #2356, #31712, #38809, #9237, #19161, #28476, #15483, #32351, #2775, #28687, #28038, #41166, #41815, #11605, #24813, #25862, #42664, #39438, #29522, #39017, #29955, #13088, #26288, #3197, #9454, #6226, #23257, #12667, #33410, #39641, #36202, #20004, #26495, #10081, #33196, #29106, #9871, #22837, #395, #13515, #22620, #23045, #12880, #36417, #19371, #6639, #35795, #32559, #2987, #19789, #3627, #26075, #16754, #7071, #32976, #29739, #16323, #6851, #26703, #16111, #39855, #3405, #10289, #186, #23476, #42453, #29307, #39226, #36624, #9664, #20220, #16540, #15902, #42242, #35999, #6434, #19577, #13306, #32760, #21286, #20432, #11136, #30381, #17394, #1237, #30800, #4037, #34041, #37051, #24119, #10500, #4461, #7488, #1449, #14584, #20640, #33617, #37256, #37478, #34260, #3835, #17604, #40909, #30591, #30167, #7922, #14362, #21069, #4674, #23906, #607, #27772, #23688, #1022, #40069, #40694, #14142, #10925, #27343, #40477, #11351, #17824, #7278, #27129, #33828, #24544, #7707, #17183, #37695, #27560, #20857, #813, #24337, #31019, #8137, #26912, #36835, #16971, #10709, #13935, #13722, #40272, #4252, #18256, #12410, #18475, #1663, #38761, #5534, #8773, #15644, #27989, #9187, #31238, #31446, #5108, #21716, #21929, #18683, #15438, #8355, #28636, #31662, #28844, #31881, #22148, #1881, #21506, #37911, #2311, #28207, #18904, #28425, #35322, #12201, #34688, #41767, #41119, #15009, #41341, #34472, #11778, #25393, #24980, #5321, #38540, #8981, #38121, #35109, #8566, #11994, #11558, #5751, #34898, #32085, #2519, #2096, #15226, #41561, #25189, #24767, #38330, #41979, #25603, #4894, #18042, #14794, #29257, #25811, #2721, #38967, #16065, #20322, #6172, #9402, #13833, #19313, #16860, #35534, #39965, #23585, #40375, #3939, #505, #27027, #33516, #17077, #40172, #5962, #6960, #42401, #32506, #36732, #15853, #10603, #2936, #921, #20117, #30063, #29052, #22566, #42191, #3730, #23790, #12832, #36945, #14036, #33305, #7170, #22782, #30275, #26023, #30494, #714, #39175, #7387, #9609, #12618, #35943, #35744, #13621, #20534, #26813, #33723, #10395, #4146, #17290, #27232, #22358, #19114, #32297, #28314, #11033, #37803, #30697, #20968, #14907, #10817, #8249, #24227, #41016, #1345, #31131, #17502, #11460, #14474, #8466, #21617, #27669, #40591, #18152, #37378, #34154, #34368, #4363, #17932, #15119, #34796, #31561, #17714, #14252, #33941, #27455, #4572, #21396, #7821, #30909, #1777, #40807, #4784, #1129, #24872, #31347, #11672, #34581, #28106, #41234, #24010, #1564, #11247, #5011, #38022, #5216, #24445, #37590, #18372, #1994, #8034, #37152, #7598, #14694, #20753, #27883, #21178, #24661, #22260, #38656, #22678, #12721, #12310, #25508, #28747, #35008, #31776, #6069, #38230, #5438, #42090, #2413, #39070, #9509, #15545, #28535, #19218, #41667, #22047, #35429, #18590, #9294, #35641, #2206, #19427, #5651, #15338, #21829, #12102, #35220, #38865, #25297, #38440, #32408, #8884, #5857, #18799, #25919, #2830, #42300, #25716, #15964, #31987, #32196, #19011, #41873, #22464, #29160, #35848, #9093, #2623, #6281, #32617, #15755, #3042, #16170, #28953, #41455, #12523, #8675, #11890, #25085, #239, #39282, #664, #13361, #26553, #16596, #22897, #19637, #36682, #26127, #4097, #10344, #6906, #33465, #39914, #23532, #3891, #42505, #39701, #6489, #13783, #26966, #36053, #10137, #26341, #7122, #32821, #23317, #3251, #16378, #9715, #36471, #17026, #39493, #30225, #20486, #20060, #454, #29799, #13570, #20277, #29578, #40124, #33255, #10554, #26761, #23740, #13146, #23, #9924, #36893, #23103, #7337, #3681, #33672, #29365, #36265, #12932, #6696, #19847, #33031, #3461, #16809, #30008, #21341, #34745, #40964, #40327, #34529, #1075, #27832, #37968, #1292, #27183, #21564, #31076, #34315, #41176, #10769, #14200, #4953, #8413, #14421, #1509, #17660, #11407, #27400, #24823, #24601, #40536, #8194, #10979, #37102, #24175, #27615, #18100, #17239, #14643, #14853, #11197, #31295, #37750, #4309, #1726, #23958, #40755, #30439, #17448, #28050, #7545, #37322, #11615, #870, #13986, #20699, #33887, #7769, #30644, #24395, #17879, #20912, #34095, #4516, #30854, #37536, #7976, #21126, #4731, #5592, #28263, #18745, #6019, #38816, #15287, #41823, #5166, #22413, #32145, #28484, #9040, #5381, #38178, #2575, #18532, #31937, #8622, #42038, #15704, #28903, #38600, #12467, #25661, #18318, #25455, #35591, #2364, #15064, #9243, #35380, #38391, #19169, #5805, #31722, #18958, #31508, #15491, #1938, #22205, #21778, #28696, #12260, #41401, #11835, #25036, #12050, #34957, #2152, #41616, #25246, #8832, #21989, #35166, #24747, #21269, #5092, #11541, #37893, #18238, #14125, #27754, #7905, #11116, #14776, #24100, #31428, #27543, #24318, #27972, #37239, #40890, #40677, #21486, #34024, #37677, #7686, #17587, #20841, #24527, #1865, #37462, #14992, #34880, #11333, #41099, #1432, #8337, #21053, #8547, #34669, #8117, #24962, #28189, #41323, #34243, #30786, #4446, #11761, #4657, #38103, #34455, #21698, #5303, #1220, #18455, #14345, #4876, #1007, #17807, #27327, #40461, #31003, #14565, #10909, #18024, #31219, #1646, #22129, #9170, #38314, #32277, #35304, #29239, #42381, #5735, #18666, #38949, #31863, #12184, #12391, #42172, #12599, #25793, #8755, #9589, #38522, #35090, #11975, #5515, #25375, #29033, #15419, #2295, #22549, #28617, #25587, #21910, #2916, #9383, #32489, #41749, #35724, #8965, #22341, #38741, #18887, #15833, #6154, #12813, #32067, #2501, #39158, #19295, #15626, #16046, #26006, #35517, #22764, #5946, #41545, #35926, #28828, #41959, #25170, #6365, #19094, #2702, #31644, #2077, #15208, #28407, #16253, #36979, #534, #39783, #23621, #30096, #13653, #36766, #32694, #3336, #39363, #110, #19509, #36135, #26844, #16469, #33122, #16894, #3761, #19723, #6997, #10005, #10217, #26213, #20150, #23185, #17110, #30310, #36346, #3125, #29667, #6777, #9800, #22979, #39995, #10428, #7203, #6567, #40207, #26421, #32903, #42596, #13233, #39572, #20356, #19934, #3549, #33545, #16684, #29880, #3970, #744, #13866, #27062, #10637, #23827, #29453, #33339, #13021, #319, #13439, #26634, #23402, #36552, #17629, #24571, #40503, #37719, #8380, #7515, #8161, #11161, #21095, #4919, #20879, #27583, #23928, #28015, #40721, #24360, #1262, #20664, #4276, #21309, #10736, #31470, #34498, #34283, #18067, #31264, #37072, #17418, #1689, #10948, #33852, #41144, #11582, #30615, #37502, #24145, #14818, #1043, #7945, #14168, #27367, #37284, #4698, #24790, #7731, #34066, #4487, #14386, #31044, #11373, #27799, #37935, #30824, #21530, #17847, #34712, #40931, #5134, #1475, #14610, #18280, #13958, #27152, #40294, #38564, #9427, #34922, #2335, #9006, #22175, #2121, #15251, #2544, #35347, #19138, #25005, #5344, #32323, #28452, #21743, #29078, #15876, #38147, #41792, #41586, #28662, #11803, #6197, #15670, #18929, #25835, #8590, #19342, #41366, #12018, #25214, #31905, #32112, #42005, #28871, #25629, #18499, #38787, #12227, #38990, #31688, #38358, #25419, #35560, #1903, #12433, #42215, #8796, #5987, #22592, #21954, #15463, #5775, #9211, #35135, #5560, #15033, #18712, #22382, #2749, #28231, #12643, #35769, #7043, #16297, #365, #155, #3170, #9843, #40041, #29711, #29923, #36809, #32532, #42635, #36174 ),
 .UNSPECIFIED., .F., .F. ) 
 B_SPLINE_CURVE_WITH_KNOTS ( ( 3, 2, 2, 2, 2, 2, 2, 2, 2, 2, 2, 2, 2, 2, 2, 2, 2, 2, 2, 2, 2, 2, 2, 2, 2, 2, 2, 2, 2, 2, 2, 2, 2, 2, 2, 2, 2, 2, 2, 2, 2, 2, 2, 2, 2, 2, 2, 2, 2, 2, 2, 2, 2, 2, 2, 2, 2, 2, 2, 2, 2, 2, 2, 2, 2, 2, 2, 2, 2, 2, 2, 2, 2, 2, 2, 2, 2, 2, 2, 2, 2, 2, 2, 2, 2, 2, 2, 2, 2, 2, 2, 2, 2, 2, 2, 2, 2, 2, 2, 2, 2, 2, 2, 2, 2, 2, 2, 2, 2, 2, 2, 2, 2, 2, 2, 2, 2, 2, 2, 2, 2, 2, 2, 2, 2, 2, 2, 2, 2, 2, 2, 2, 2, 2, 2, 2, 2, 2, 2, 2, 2, 2, 2, 2, 2, 2, 2, 2, 2, 2, 2, 2, 2, 2, 2, 2, 2, 2, 2, 2, 2, 2, 2, 2, 2, 2, 2, 2, 2, 2, 2, 2, 2, 2, 2, 2, 2, 2, 2, 2, 2, 2, 2, 2, 2, 2, 2, 2, 2, 2, 2, 2, 2, 2, 2, 2, 2, 2, 2, 2, 2, 2, 2, 2, 2, 2, 2, 2, 2, 2, 2, 2, 2, 2, 2, 2, 2, 2, 2, 2, 2, 2, 2, 2, 2, 2, 2, 2, 2, 2, 2, 2, 2, 2, 2, 2, 2, 2, 2, 2, 2, 2, 2, 2, 2, 2, 2, 2, 2, 2, 2, 2, 2, 2, 2, 2, 2, 2, 2, 2, 2, 2, 2, 2, 2, 2, 2, 2, 2, 2, 2, 2, 2, 2, 2, 2, 2, 2, 2, 2, 2, 2, 2, 2, 2, 2, 2, 2, 2, 2, 2, 2, 2, 2, 2, 2, 2, 2, 2, 2, 2, 2, 2, 2, 2, 2, 2, 2, 2, 2, 2, 2, 2, 2, 2, 2, 2, 2, 2, 2, 2, 2, 2, 2, 2, 2, 2, 2, 2, 2, 2, 2, 2, 2, 2, 2, 2, 2, 2, 2, 2, 2, 2, 2, 2, 2, 2, 2, 2, 2, 2, 2, 2, 2, 2, 2, 2, 2, 2, 2, 2, 2, 2, 2, 2, 2, 2, 2, 2, 2, 2, 2, 2, 2, 2, 2, 2, 2, 2, 2, 2, 2, 2, 2, 2, 2, 2, 2, 2, 2, 2, 2, 2, 2, 2, 2, 2, 2, 2, 2, 2, 2, 2, 2, 2, 2, 2, 2, 2, 2, 2, 2, 2, 2, 2, 2, 2, 2, 2, 2, 2, 2, 2, 2, 2, 2, 2, 2, 2, 2, 2, 2, 2, 2, 2, 2, 2, 2, 2, 2, 2, 2, 2, 2, 2, 2, 2, 2, 2, 2, 2, 2, 2, 2, 2, 2, 2, 2, 2, 2, 2, 2, 2, 2, 2, 2, 2, 2, 2, 2, 2, 2, 2, 2, 2, 2, 2, 2, 2, 2, 2, 2, 2, 2, 2, 2, 2, 2, 2, 2, 2, 2, 2, 2, 2, 2, 2, 2, 2, 2, 2, 2, 2, 2, 2, 2, 2, 2, 2, 2, 2, 2, 2, 2, 2, 2, 2, 2, 2, 2, 2, 2, 2, 2, 2, 2, 2, 2, 2, 2, 2, 2, 2, 2, 2, 2, 2, 2, 2, 2, 2, 2, 2, 2, 2, 2, 2, 2, 2, 2, 2, 2, 2, 2, 2, 2, 2, 2, 2, 2, 2, 2, 2, 2, 2, 2, 2, 2, 2, 2, 2, 2, 2, 2, 2, 2, 2, 2, 2, 2, 2, 2, 2, 2, 2, 2, 2, 2, 2, 2, 2, 2, 2, 2, 2, 2, 2, 2, 2, 2, 2, 2, 2, 2, 2, 2, 2, 2, 2, 2, 2, 2, 2, 2, 2, 2, 2, 2, 2, 2, 2, 2, 2, 2, 2, 2, 2, 2, 2, 2, 2, 2, 2, 2, 2, 2, 2, 2, 2, 2, 2, 2, 2, 2, 2, 2, 2, 2, 2, 2, 2, 2, 2, 2, 2, 2, 2, 2, 2, 2, 2, 2, 2, 2, 2, 2, 2, 2, 2, 2, 2, 2, 2, 2, 2, 2, 2, 2, 2, 2, 2, 2, 2, 2, 2, 2, 2, 2, 2, 2, 2, 2, 2, 2, 2, 2, 2, 2, 2, 2, 2, 2, 2, 2, 2, 2, 2, 2, 2, 2, 2, 2, 2, 2, 2, 2, 2, 2, 2, 2, 2, 2, 2, 2, 2, 2, 2, 2, 2, 2, 2, 2, 2, 2, 2, 2, 2, 2, 2, 2, 2, 2, 2, 2, 2, 2, 2, 2, 2, 2, 2, 2, 2, 2, 2, 2, 2, 2, 2, 2, 2, 2, 2, 2, 2, 2, 2, 2, 2, 2, 2, 2, 2, 2, 2, 2, 2, 2, 2, 2, 2, 2, 2, 2, 2, 2, 2, 2, 2, 2, 2, 2, 2, 2, 2, 2, 2, 2, 3 ),
 ( 0.000000000000000000, 0.001243781094527363160, 0.002487562189054726321, 0.003731343283582089481, 0.004975124378109452641, 0.006218905472636816235, 0.007462686567164178962, 0.008706467661691542556, 0.009950248756218905283, 0.01119402985074626801, 0.01243781094527363247, 0.01368159203980099520, 0.01492537313432835792, 0.01616915422885572065, 0.01741293532338308511, 0.01865671641791044610, 0.01990049751243781057, 0.02114427860696517503, 0.02238805970149253602, 0.02363184079601990048, 0.02487562189054726494, 0.02611940298507462593, 0.02736318407960199039, 0.02860696517412935486, 0.02985074626865671585, 0.03109452736318408031, 0.03233830845771144130, 0.03358208955223880576, 0.03482587064676617022, 0.03606965174129353469, 0.03731343283582089221, 0.03855721393034825667, 0.03980099502487562113, 0.04104477611940298559, 0.04228855721393035005, 0.04353233830845771452, 0.04477611940298507204, 0.04601990049751243650, 0.04726368159203980096, 0.04850746268656716542, 0.04975124378109452988, 0.05099502487562188741, 0.05223880597014925187, 0.05348258706467661633, 0.05472636815920398079, 0.05597014925373134525, 0.05721393034825870971, 0.05845771144278606724, 0.05970149253731343170, 0.06094527363184079616, 0.06218905472636816062, 0.06343283582089552508, 0.06467661691542288260, 0.06592039800995025400, 0.06716417910447761153, 0.06840796019900496905, 0.06965174129353234045, 0.07089552238805969797, 0.07213930348258706937, 0.07338308457711442689, 0.07462686567164178442, 0.07587064676616915582, 0.07711442786069651334, 0.07835820895522388474, 0.07960199004975124226, 0.08084577114427861366, 0.08208955223880597118, 0.08333333333333332871, 0.08457711442786070011, 0.08582089552238805763, 0.08706467661691542903, 0.08830845771144278655, 0.08955223880597014408, 0.09079601990049751548, 0.09203980099502487300, 0.09328358208955224440, 0.09452736318407960192, 0.09577114427860695944, 0.09701492537313433084, 0.09825870646766168837, 0.09950248756218905977, 0.1007462686567164173, 0.1019900497512437748, 0.1032338308457711462, 0.1044776119402985037, 0.1057213930348258751, 0.1069651741293532327, 0.1082089552238805902, 0.1094527363184079616, 0.1106965174129353191, 0.1119402985074626905, 0.1131840796019900480, 0.1144278606965174194, 0.1156716417910447769, 0.1169154228855721345, 0.1181592039800995059, 0.1194029850746268634, 0.1206467661691542348, 0.1218905472636815923, 0.1231343283582089498, 0.1243781094527363212, 0.1256218905472636926, 0.1268656716417910502, 0.1281094527363184077, 0.1293532338308457652, 0.1305970149253731227, 0.1318407960199005080, 0.1330845771144278655, 0.1343283582089552231, 0.1355721393034825806, 0.1368159203980099381, 0.1380597014925373234, 0.1393034825870646809, 0.1405472636815920384, 0.1417910447761193959, 0.1430348258706467535, 0.1442786069651741387, 0.1455223880597014963, 0.1467661691542288538, 0.1480099502487562113, 0.1492537313432835688, 0.1504975124378109541, 0.1517412935323383116, 0.1529850746268656692, 0.1542288557213930267, 0.1554726368159203842, 0.1567164179104477695, 0.1579601990049751270, 0.1592039800995024845, 0.1604477611940298420, 0.1616915422885572273, 0.1629353233830845848, 0.1641791044776119424, 0.1654228855721392999, 0.1666666666666666574, 0.1679104477611940427, 0.1691542288557214002, 0.1703980099502487577, 0.1716417910447761153, 0.1728855721393034728, 0.1741293532338308581, 0.1753731343283582156, 0.1766169154228855731, 0.1778606965174129306, 0.1791044776119402882, 0.1803482587064676734, 0.1815920398009950310, 0.1828358208955223885, 0.1840796019900497460, 0.1853233830845771035, 0.1865671641791044888, 0.1878109452736318463, 0.1890547263681592038, 0.1902985074626865614, 0.1915422885572139189, 0.1927860696517413042, 0.1940298507462686617, 0.1952736318407960192, 0.1965174129353233767, 0.1977611940298507343, 0.1990049751243781195, 0.2002487562189054771, 0.2014925373134328346, 0.2027363184079601921, 0.2039800995024875496, 0.2052238805970149349, 0.2064676616915422924, 0.2077114427860696499, 0.2089552238805970075, 0.2101990049751243650, 0.2114427860696517503, 0.2126865671641791078, 0.2139303482587064653, 0.2151741293532338228, 0.2164179104477611804, 0.2176616915422885656, 0.2189054726368159232, 0.2201492537313432807, 0.2213930348258706382, 0.2226368159203980235, 0.2238805970149253810, 0.2251243781094527385, 0.2263681592039800961, 0.2276119402985074536, 0.2288557213930348389, 0.2300995024875621964, 0.2313432835820895539, 0.2325870646766169114, 0.2338308457711442689, 0.2350746268656716542, 0.2363184079601990117, 0.2375621890547263693, 0.2388059701492537268, 0.2400497512437810843, 0.2412935323383084696, 0.2425373134328358271, 0.2437810945273631846, 0.2450248756218905422, 0.2462686567164178997, 0.2475124378109452850, 0.2487562189054726425, 0.2500000000000000000, 0.2512437810945273853, 0.2524875621890547150, 0.2537313432835821003, 0.2549751243781094301, 0.2562189054726368154, 0.2574626865671642006, 0.2587064676616915304, 0.2599502487562189157, 0.2611940298507462455, 0.2624378109452736307, 0.2636815920398010160, 0.2649253731343283458, 0.2661691542288557311, 0.2674129353233830608, 0.2686567164179104461, 0.2699004975124378314, 0.2711442786069651611, 0.2723880597014925464, 0.2736318407960198762, 0.2748756218905472615, 0.2761194029850746468, 0.2773631840796019765, 0.2786069651741293618, 0.2798507462686566916, 0.2810945273631840768, 0.2823383084577114621, 0.2835820895522387919, 0.2848258706467661772, 0.2860696517412935069, 0.2873134328358208922, 0.2885572139303482775, 0.2898009950248756073, 0.2910447761194029925, 0.2922885572139303223, 0.2935323383084577076, 0.2947761194029850929, 0.2960199004975124226, 0.2972636815920398079, 0.2985074626865671377, 0.2997512437810945229, 0.3009950248756219082, 0.3022388059701492380, 0.3034825870646766233, 0.3047263681592039530, 0.3059701492537313383, 0.3072139303482587236, 0.3084577114427860534, 0.3097014925373134386, 0.3109452736318407684, 0.3121890547263681537, 0.3134328358208955390, 0.3146766169154228687, 0.3159203980099502540, 0.3171641791044776393, 0.3184079601990049690, 0.3196517412935323543, 0.3208955223880596841, 0.3221393034825870694, 0.3233830845771144546, 0.3246268656716417844, 0.3258706467661691697, 0.3271144278606964995, 0.3283582089552238847, 0.3296019900497512700, 0.3308457711442785998, 0.3320895522388059851, 0.3333333333333333148, 0.3345771144278607001, 0.3358208955223880854, 0.3370646766169154152, 0.3383084577114428004, 0.3395522388059701302, 0.3407960199004975155, 0.3420398009950249008, 0.3432835820895522305, 0.3445273631840796158, 0.3457711442786069456, 0.3470149253731343308, 0.3482587064676617161, 0.3495024875621890459, 0.3507462686567164312, 0.3519900497512437609, 0.3532338308457711462, 0.3544776119402985315, 0.3557213930348258613, 0.3569651741293532465, 0.3582089552238805763, 0.3594527363184079616, 0.3606965174129353469, 0.3619402985074626766, 0.3631840796019900619, 0.3644278606965173917, 0.3656716417910447769, 0.3669154228855721622, 0.3681592039800994920, 0.3694029850746268773, 0.3706467661691542070, 0.3718905472636815923, 0.3731343283582089776, 0.3743781094527363074, 0.3756218905472636926, 0.3768656716417910224, 0.3781094527363184077, 0.3793532338308457930, 0.3805970149253731227, 0.3818407960199005080, 0.3830845771144278378, 0.3843283582089552231, 0.3855721393034826083, 0.3868159203980099381, 0.3880597014925373234, 0.3893034825870646531, 0.3905472636815920384, 0.3917910447761194237, 0.3930348258706467535, 0.3942786069651741387, 0.3955223880597014685, 0.3967661691542288538, 0.3980099502487562391, 0.3992537313432835688, 0.4004975124378109541, 0.4017412935323382839, 0.4029850746268656692, 0.4042288557213930544, 0.4054726368159203842, 0.4067164179104477695, 0.4079601990049750992, 0.4092039800995024845, 0.4104477611940298698, 0.4116915422885571996, 0.4129353233830845848, 0.4141791044776119146, 0.4154228855721392999, 0.4166666666666666297, 0.4179104477611940149, 0.4191542288557214002, 0.4203980099502487300, 0.4216417910447761153, 0.4228855721393035005, 0.4241293532338308303, 0.4253731343283582156, 0.4266169154228855454, 0.4278606965174129306, 0.4291044776119403159, 0.4303482587064676457, 0.4315920398009950310, 0.4328358208955223607, 0.4340796019900497460, 0.4353233830845771313, 0.4365671641791044610, 0.4378109452736318463, 0.4390547263681592316, 0.4402985074626865614, 0.4415422885572139466, 0.4427860696517412764, 0.4440298507462686617, 0.4452736318407960470, 0.4465174129353233767, 0.4477611940298507620, 0.4490049751243780918, 0.4502487562189054771, 0.4514925373134328623, 0.4527363184079601921, 0.4539800995024875774, 0.4552238805970149071, 0.4564676616915422924, 0.4577114427860696777, 0.4589552238805970075, 0.4601990049751243927, 0.4614427860696517225, 0.4626865671641791078, 0.4639303482587064931, 0.4651741293532338228, 0.4664179104477612081, 0.4676616915422885379, 0.4689054726368159232, 0.4701492537313433084, 0.4713930348258706382, 0.4726368159203980235, 0.4738805970149253532, 0.4751243781094527385, 0.4763681592039801238, 0.4776119402985074536, 0.4788557213930348389, 0.4800995024875621686, 0.4813432835820895539, 0.4825870646766169392, 0.4838308457711442689, 0.4850746268656716542, 0.4863184079601989840, 0.4875621890547263693, 0.4888059701492537545, 0.4900497512437810843, 0.4912935323383084696, 0.4925373134328357994, 0.4937810945273631846, 0.4950248756218905699, 0.4962686567164178997, 0.4975124378109452850, 0.4987562189054726147, 0.5000000000000000000, 0.5012437810945273853, 0.5024875621890547706, 0.5037313432835820448, 0.5049751243781094301, 0.5062189054726368154, 0.5074626865671642006, 0.5087064676616915859, 0.5099502487562188602, 0.5111940298507462455, 0.5124378109452736307, 0.5136815920398010160, 0.5149253731343284013, 0.5161691542288556755, 0.5174129353233830608, 0.5186567164179104461, 0.5199004975124378314, 0.5211442786069652167, 0.5223880597014924909, 0.5236318407960198762, 0.5248756218905472615, 0.5261194029850746468, 0.5273631840796020320, 0.5286069651741293063, 0.5298507462686566916, 0.5310945273631840768, 0.5323383084577114621, 0.5335820895522388474, 0.5348258706467661217, 0.5360696517412935069, 0.5373134328358208922, 0.5385572139303482775, 0.5398009950248756628, 0.5410447761194029370, 0.5422885572139303223, 0.5435323383084577076, 0.5447761194029850929, 0.5460199004975124781, 0.5472636815920397524, 0.5485074626865671377, 0.5497512437810945229, 0.5509950248756219082, 0.5522388059701492935, 0.5534825870646765678, 0.5547263681592039530, 0.5559701492537313383, 0.5572139303482587236, 0.5584577114427861089, 0.5597014925373133831, 0.5609452736318407684, 0.5621890547263681537, 0.5634328358208955390, 0.5646766169154229242, 0.5659203980099501985, 0.5671641791044775838, 0.5684079601990049690, 0.5696517412935323543, 0.5708955223880597396, 0.5721393034825870139, 0.5733830845771143991, 0.5746268656716417844, 0.5758706467661691697, 0.5771144278606965550, 0.5783582089552238292, 0.5796019900497512145, 0.5808457711442785998, 0.5820895522388059851, 0.5833333333333333703, 0.5845771144278606446, 0.5858208955223880299, 0.5870646766169154152, 0.5883084577114428004, 0.5895522388059701857, 0.5907960199004974600, 0.5920398009950248452, 0.5932835820895522305, 0.5945273631840796158, 0.5957711442786070011, 0.5970149253731342753, 0.5982587064676616606, 0.5995024875621890459, 0.6007462686567164312, 0.6019900497512438164, 0.6032338308457710907, 0.6044776119402984760, 0.6057213930348258613, 0.6069651741293532465, 0.6082089552238806318, 0.6094527363184079061, 0.6106965174129352913, 0.6119402985074626766, 0.6131840796019900619, 0.6144278606965174472, 0.6156716417910447214, 0.6169154228855721067, 0.6181592039800994920, 0.6194029850746268773, 0.6206467661691542625, 0.6218905472636815368, 0.6231343283582089221, 0.6243781094527363074, 0.6256218905472636926, 0.6268656716417910779, 0.6281094527363184632, 0.6293532338308457375, 0.6305970149253731227, 0.6318407960199005080, 0.6330845771144278933, 0.6343283582089552786, 0.6355721393034825528, 0.6368159203980099381, 0.6380597014925373234, 0.6393034825870647087, 0.6405472636815920939, 0.6417910447761193682, 0.6430348258706467535, 0.6442786069651741387, 0.6455223880597015240, 0.6467661691542289093, 0.6480099502487561836, 0.6492537313432835688, 0.6504975124378109541, 0.6517412935323383394, 0.6529850746268657247, 0.6542288557213929989, 0.6554726368159203842, 0.6567164179104477695, 0.6579601990049751548, 0.6592039800995025400, 0.6604477611940298143, 0.6616915422885571996, 0.6629353233830845848, 0.6641791044776119701, 0.6654228855721393554, 0.6666666666666666297, 0.6679104477611940149, 0.6691542288557214002, 0.6703980099502487855, 0.6716417910447761708, 0.6728855721393034450, 0.6741293532338308303, 0.6753731343283582156, 0.6766169154228856009, 0.6778606965174129861, 0.6791044776119402604, 0.6803482587064676457, 0.6815920398009950310, 0.6828358208955224162, 0.6840796019900498015, 0.6853233830845770758, 0.6865671641791044610, 0.6878109452736318463, 0.6890547263681592316, 0.6902985074626866169, 0.6915422885572138911, 0.6927860696517412764, 0.6940298507462686617, 0.6952736318407960470, 0.6965174129353234322, 0.6977611940298507065, 0.6990049751243780918, 0.7002487562189054771, 0.7014925373134328623, 0.7027363184079602476, 0.7039800995024875219, 0.7052238805970149071, 0.7064676616915422924, 0.7077114427860696777, 0.7089552238805970630, 0.7101990049751243372, 0.7114427860696517225, 0.7126865671641791078, 0.7139303482587064931, 0.7151741293532338783, 0.7164179104477611526, 0.7176616915422885379, 0.7189054726368159232, 0.7201492537313433084, 0.7213930348258706937, 0.7226368159203979680, 0.7238805970149253532, 0.7251243781094527385, 0.7263681592039801238, 0.7276119402985075091, 0.7288557213930347833, 0.7300995024875621686, 0.7313432835820895539, 0.7325870646766169392, 0.7338308457711443245, 0.7350746268656715987, 0.7363184079601989840, 0.7375621890547263693, 0.7388059701492537545, 0.7400497512437811398, 0.7412935323383084141, 0.7425373134328357994, 0.7437810945273631846, 0.7450248756218905699, 0.7462686567164179552, 0.7475124378109452294, 0.7487562189054726147, 0.7500000000000000000, 0.7512437810945273853, 0.7524875621890547706, 0.7537313432835820448, 0.7549751243781094301, 0.7562189054726368154, 0.7574626865671642006, 0.7587064676616915859, 0.7599502487562188602, 0.7611940298507462455, 0.7624378109452736307, 0.7636815920398010160, 0.7649253731343284013, 0.7661691542288556755, 0.7674129353233830608, 0.7686567164179104461, 0.7699004975124378314, 0.7711442786069652167, 0.7723880597014924909, 0.7736318407960198762, 0.7748756218905472615, 0.7761194029850746468, 0.7773631840796020320, 0.7786069651741293063, 0.7798507462686566916, 0.7810945273631840768, 0.7823383084577114621, 0.7835820895522388474, 0.7848258706467661217, 0.7860696517412935069, 0.7873134328358208922, 0.7885572139303482775, 0.7898009950248756628, 0.7910447761194029370, 0.7922885572139303223, 0.7935323383084577076, 0.7947761194029850929, 0.7960199004975124781, 0.7972636815920397524, 0.7985074626865671377, 0.7997512437810945229, 0.8009950248756219082, 0.8022388059701492935, 0.8034825870646765678, 0.8047263681592039530, 0.8059701492537313383, 0.8072139303482587236, 0.8084577114427861089, 0.8097014925373133831, 0.8109452736318407684, 0.8121890547263681537, 0.8134328358208955390, 0.8146766169154229242, 0.8159203980099501985, 0.8171641791044775838, 0.8184079601990049690, 0.8196517412935323543, 0.8208955223880597396, 0.8221393034825870139, 0.8233830845771143991, 0.8246268656716417844, 0.8258706467661691697, 0.8271144278606965550, 0.8283582089552238292, 0.8296019900497512145, 0.8308457711442785998, 0.8320895522388059851, 0.8333333333333332593, 0.8345771144278606446, 0.8358208955223880299, 0.8370646766169154152, 0.8383084577114428004, 0.8395522388059701857, 0.8407960199004974600, 0.8420398009950248452, 0.8432835820895522305, 0.8445273631840796158, 0.8457711442786070011, 0.8470149253731342753, 0.8482587064676616606, 0.8495024875621890459, 0.8507462686567164312, 0.8519900497512438164, 0.8532338308457710907, 0.8544776119402984760, 0.8557213930348258613, 0.8569651741293532465, 0.8582089552238806318, 0.8594527363184079061, 0.8606965174129352913, 0.8619402985074626766, 0.8631840796019900619, 0.8644278606965174472, 0.8656716417910447214, 0.8669154228855721067, 0.8681592039800994920, 0.8694029850746268773, 0.8706467661691542625, 0.8718905472636815368, 0.8731343283582089221, 0.8743781094527363074, 0.8756218905472636926, 0.8768656716417910779, 0.8781094527363184632, 0.8793532338308457375, 0.8805970149253731227, 0.8818407960199005080, 0.8830845771144278933, 0.8843283582089552786, 0.8855721393034825528, 0.8868159203980099381, 0.8880597014925373234, 0.8893034825870647087, 0.8905472636815920939, 0.8917910447761193682, 0.8930348258706467535, 0.8942786069651741387, 0.8955223880597015240, 0.8967661691542289093, 0.8980099502487561836, 0.8992537313432835688, 0.9004975124378109541, 0.9017412935323383394, 0.9029850746268657247, 0.9042288557213929989, 0.9054726368159203842, 0.9067164179104477695, 0.9079601990049751548, 0.9092039800995025400, 0.9104477611940298143, 0.9116915422885571996, 0.9129353233830845848, 0.9141791044776120811, 0.9154228855721393554, 0.9166666666666666297, 0.9179104477611940149, 0.9191542288557214002, 0.9203980099502487855, 0.9216417910447761708, 0.9228855721393034450, 0.9241293532338308303, 0.9253731343283582156, 0.9266169154228856009, 0.9278606965174129861, 0.9291044776119402604, 0.9303482587064676457, 0.9315920398009950310, 0.9328358208955224162, 0.9340796019900498015, 0.9353233830845770758, 0.9365671641791044610, 0.9378109452736318463, 0.9390547263681592316, 0.9402985074626866169, 0.9415422885572138911, 0.9427860696517412764, 0.9440298507462686617, 0.9452736318407960470, 0.9465174129353234322, 0.9477611940298507065, 0.9490049751243780918, 0.9502487562189054771, 0.9514925373134328623, 0.9527363184079602476, 0.9539800995024875219, 0.9552238805970149071, 0.9564676616915422924, 0.9577114427860696777, 0.9589552238805970630, 0.9601990049751243372, 0.9614427860696517225, 0.9626865671641791078, 0.9639303482587064931, 0.9651741293532338783, 0.9664179104477611526, 0.9676616915422885379, 0.9689054726368159232, 0.9701492537313433084, 0.9713930348258706937, 0.9726368159203979680, 0.9738805970149253532, 0.9751243781094527385, 0.9763681592039801238, 0.9776119402985075091, 0.9788557213930347833, 0.9800995024875621686, 0.9813432835820895539, 0.9825870646766169392, 0.9838308457711443245, 0.9850746268656715987, 0.9863184079601989840, 0.9875621890547263693, 0.9888059701492537545, 0.9900497512437811398, 0.9912935323383084141, 0.9917697938471236041 ),
 .UNSPECIFIED. ) 
 CURVE ( )  GEOMETRIC_REPRESENTATION_ITEM ( )  RATIONAL_B_SPLINE_CURVE ( ( 1.000000000000000000, 0.8660254037844387076, 1.000000000000000000, 0.8660254037844387076, 1.000000000000000000, 0.8660254037844387076, 1.000000000000000000, 0.8660254037844387076, 1.000000000000000000, 0.8660254037844387076, 1.000000000000000000, 0.8660254037844387076, 1.000000000000000000, 0.8660254037844387076, 1.000000000000000000, 0.8660254037844387076, 1.000000000000000000, 0.8660254037844387076, 1.000000000000000000, 0.8660254037844387076, 1.000000000000000000, 0.8660254037844387076, 1.000000000000000000, 0.8660254037844387076, 1.000000000000000000, 0.8660254037844387076, 1.000000000000000000, 0.8660254037844387076, 1.000000000000000000, 0.8660254037844387076, 1.000000000000000000, 0.8660254037844387076, 1.000000000000000000, 0.8660254037844387076, 1.000000000000000000, 0.8660254037844387076, 1.000000000000000000, 0.8660254037844387076, 1.000000000000000000, 0.8660254037844387076, 1.000000000000000000, 0.8660254037844387076, 1.000000000000000000, 0.8660254037844387076, 1.000000000000000000, 0.8660254037844387076, 1.000000000000000000, 0.8660254037844387076, 1.000000000000000000, 0.8660254037844387076, 1.000000000000000000, 0.8660254037844387076, 1.000000000000000000, 0.8660254037844387076, 1.000000000000000000, 0.8660254037844387076, 1.000000000000000000, 0.8660254037844387076, 1.000000000000000000, 0.8660254037844387076, 1.000000000000000000, 0.8660254037844387076, 1.000000000000000000, 0.8660254037844387076, 1.000000000000000000, 0.8660254037844387076, 1.000000000000000000, 0.8660254037844387076, 1.000000000000000000, 0.8660254037844387076, 1.000000000000000000, 0.8660254037844387076, 1.000000000000000000, 0.8660254037844387076, 1.000000000000000000, 0.8660254037844387076, 1.000000000000000000, 0.8660254037844387076, 1.000000000000000000, 0.8660254037844387076, 1.000000000000000000, 0.8660254037844387076, 1.000000000000000000, 0.8660254037844387076, 1.000000000000000000, 0.8660254037844387076, 1.000000000000000000, 0.8660254037844387076, 1.000000000000000000, 0.8660254037844387076, 1.000000000000000000, 0.8660254037844387076, 1.000000000000000000, 0.8660254037844387076, 1.000000000000000000, 0.8660254037844387076, 1.000000000000000000, 0.8660254037844387076, 1.000000000000000000, 0.8660254037844387076, 1.000000000000000000, 0.8660254037844387076, 1.000000000000000000, 0.8660254037844387076, 1.000000000000000000, 0.8660254037844387076, 1.000000000000000000, 0.8660254037844387076, 1.000000000000000000, 0.8660254037844387076, 1.000000000000000000, 0.8660254037844387076, 1.000000000000000000, 0.8660254037844387076, 1.000000000000000000, 0.8660254037844387076, 1.000000000000000000, 0.8660254037844387076, 1.000000000000000000, 0.8660254037844387076, 1.000000000000000000, 0.8660254037844387076, 1.000000000000000000, 0.8660254037844387076, 1.000000000000000000, 0.8660254037844387076, 1.000000000000000000, 0.8660254037844387076, 1.000000000000000000, 0.8660254037844387076, 1.000000000000000000, 0.8660254037844387076, 1.000000000000000000, 0.8660254037844387076, 1.000000000000000000, 0.8660254037844387076, 1.000000000000000000, 0.8660254037844387076, 1.000000000000000000, 0.8660254037844387076, 1.000000000000000000, 0.8660254037844387076, 1.000000000000000000, 0.8660254037844387076, 1.000000000000000000, 0.8660254037844387076, 1.000000000000000000, 0.8660254037844387076, 1.000000000000000000, 0.8660254037844387076, 1.000000000000000000, 0.8660254037844387076, 1.000000000000000000, 0.8660254037844387076, 1.000000000000000000, 0.8660254037844387076, 1.000000000000000000, 0.8660254037844387076, 1.000000000000000000, 0.8660254037844387076, 1.000000000000000000, 0.8660254037844387076, 1.000000000000000000, 0.8660254037844387076, 1.000000000000000000, 0.8660254037844387076, 1.000000000000000000, 0.8660254037844387076, 1.000000000000000000, 0.8660254037844387076, 1.000000000000000000, 0.8660254037844387076, 1.000000000000000000, 0.8660254037844387076, 1.000000000000000000, 0.8660254037844387076, 1.000000000000000000, 0.8660254037844387076, 1.000000000000000000, 0.8660254037844387076, 1.000000000000000000, 0.8660254037844387076, 1.000000000000000000, 0.8660254037844387076, 1.000000000000000000, 0.8660254037844387076, 1.000000000000000000, 0.8660254037844387076, 1.000000000000000000, 0.8660254037844387076, 1.000000000000000000, 0.8660254037844387076, 1.000000000000000000, 0.8660254037844387076, 1.000000000000000000, 0.8660254037844387076, 1.000000000000000000, 0.8660254037844387076, 1.000000000000000000, 0.8660254037844387076, 1.000000000000000000, 0.8660254037844387076, 1.000000000000000000, 0.8660254037844387076, 1.000000000000000000, 0.8660254037844387076, 1.000000000000000000, 0.8660254037844387076, 1.000000000000000000, 0.8660254037844387076, 1.000000000000000000, 0.8660254037844387076, 1.000000000000000000, 0.8660254037844387076, 1.000000000000000000, 0.8660254037844387076, 1.000000000000000000, 0.8660254037844387076, 1.000000000000000000, 0.8660254037844387076, 1.000000000000000000, 0.8660254037844387076, 1.000000000000000000, 0.8660254037844387076, 1.000000000000000000, 0.8660254037844387076, 1.000000000000000000, 0.8660254037844387076, 1.000000000000000000, 0.8660254037844387076, 1.000000000000000000, 0.8660254037844387076, 1.000000000000000000, 0.8660254037844387076, 1.000000000000000000, 0.8660254037844387076, 1.000000000000000000, 0.8660254037844387076, 1.000000000000000000, 0.8660254037844387076, 1.000000000000000000, 0.8660254037844387076, 1.000000000000000000, 0.8660254037844387076, 1.000000000000000000, 0.8660254037844387076, 1.000000000000000000, 0.8660254037844387076, 1.000000000000000000, 0.8660254037844387076, 1.000000000000000000, 0.8660254037844387076, 1.000000000000000000, 0.8660254037844387076, 1.000000000000000000, 0.8660254037844387076, 1.000000000000000000, 0.8660254037844387076, 1.000000000000000000, 0.8660254037844387076, 1.000000000000000000, 0.8660254037844387076, 1.000000000000000000, 0.8660254037844387076, 1.000000000000000000, 0.8660254037844387076, 1.000000000000000000, 0.8660254037844387076, 1.000000000000000000, 0.8660254037844387076, 1.000000000000000000, 0.8660254037844387076, 1.000000000000000000, 0.8660254037844387076, 1.000000000000000000, 0.8660254037844387076, 1.000000000000000000, 0.8660254037844387076, 1.000000000000000000, 0.8660254037844387076, 1.000000000000000000, 0.8660254037844387076, 1.000000000000000000, 0.8660254037844387076, 1.000000000000000000, 0.8660254037844387076, 1.000000000000000000, 0.8660254037844387076, 1.000000000000000000, 0.8660254037844387076, 1.000000000000000000, 0.8660254037844387076, 1.000000000000000000, 0.8660254037844387076, 1.000000000000000000, 0.8660254037844387076, 1.000000000000000000, 0.8660254037844387076, 1.000000000000000000, 0.8660254037844387076, 1.000000000000000000, 0.8660254037844387076, 1.000000000000000000, 0.8660254037844387076, 1.000000000000000000, 0.8660254037844387076, 1.000000000000000000, 0.8660254037844387076, 1.000000000000000000, 0.8660254037844387076, 1.000000000000000000, 0.8660254037844387076, 1.000000000000000000, 0.8660254037844387076, 1.000000000000000000, 0.8660254037844387076, 1.000000000000000000, 0.8660254037844387076, 1.000000000000000000, 0.8660254037844387076, 1.000000000000000000, 0.8660254037844387076, 1.000000000000000000, 0.8660254037844387076, 1.000000000000000000, 0.8660254037844387076, 1.000000000000000000, 0.8660254037844387076, 1.000000000000000000, 0.8660254037844387076, 1.000000000000000000, 0.8660254037844387076, 1.000000000000000000, 0.8660254037844387076, 1.000000000000000000, 0.8660254037844387076, 1.000000000000000000, 0.8660254037844387076, 1.000000000000000000, 0.8660254037844387076, 1.000000000000000000, 0.8660254037844387076, 1.000000000000000000, 0.8660254037844387076, 1.000000000000000000, 0.8660254037844387076, 1.000000000000000000, 0.8660254037844387076, 1.000000000000000000, 0.8660254037844387076, 1.000000000000000000, 0.8660254037844387076, 1.000000000000000000, 0.8660254037844387076, 1.000000000000000000, 0.8660254037844387076, 1.000000000000000000, 0.8660254037844387076, 1.000000000000000000, 0.8660254037844387076, 1.000000000000000000, 0.8660254037844387076, 1.000000000000000000, 0.8660254037844387076, 1.000000000000000000, 0.8660254037844387076, 1.000000000000000000, 0.8660254037844387076, 1.000000000000000000, 0.8660254037844387076, 1.000000000000000000, 0.8660254037844387076, 1.000000000000000000, 0.8660254037844387076, 1.000000000000000000, 0.8660254037844387076, 1.000000000000000000, 0.8660254037844387076, 1.000000000000000000, 0.8660254037844387076, 1.000000000000000000, 0.8660254037844387076, 1.000000000000000000, 0.8660254037844387076, 1.000000000000000000, 0.8660254037844387076, 1.000000000000000000, 0.8660254037844387076, 1.000000000000000000, 0.8660254037844387076, 1.000000000000000000, 0.8660254037844387076, 1.000000000000000000, 0.8660254037844387076, 1.000000000000000000, 0.8660254037844387076, 1.000000000000000000, 0.8660254037844387076, 1.000000000000000000, 0.8660254037844387076, 1.000000000000000000, 0.8660254037844387076, 1.000000000000000000, 0.8660254037844387076, 1.000000000000000000, 0.8660254037844387076, 1.000000000000000000, 0.8660254037844387076, 1.000000000000000000, 0.8660254037844387076, 1.000000000000000000, 0.8660254037844387076, 1.000000000000000000, 0.8660254037844387076, 1.000000000000000000, 0.8660254037844387076, 1.000000000000000000, 0.8660254037844387076, 1.000000000000000000, 0.8660254037844387076, 1.000000000000000000, 0.8660254037844387076, 1.000000000000000000, 0.8660254037844387076, 1.000000000000000000, 0.8660254037844387076, 1.000000000000000000, 0.8660254037844387076, 1.000000000000000000, 0.8660254037844387076, 1.000000000000000000, 0.8660254037844387076, 1.000000000000000000, 0.8660254037844387076, 1.000000000000000000, 0.8660254037844387076, 1.000000000000000000, 0.8660254037844387076, 1.000000000000000000, 0.8660254037844387076, 1.000000000000000000, 0.8660254037844387076, 1.000000000000000000, 0.8660254037844387076, 1.000000000000000000, 0.8660254037844387076, 1.000000000000000000, 0.8660254037844387076, 1.000000000000000000, 0.8660254037844387076, 1.000000000000000000, 0.8660254037844387076, 1.000000000000000000, 0.8660254037844387076, 1.000000000000000000, 0.8660254037844387076, 1.000000000000000000, 0.8660254037844387076, 1.000000000000000000, 0.8660254037844387076, 1.000000000000000000, 0.8660254037844387076, 1.000000000000000000, 0.8660254037844387076, 1.000000000000000000, 0.8660254037844387076, 1.000000000000000000, 0.8660254037844387076, 1.000000000000000000, 0.8660254037844387076, 1.000000000000000000, 0.8660254037844387076, 1.000000000000000000, 0.8660254037844387076, 1.000000000000000000, 0.8660254037844387076, 1.000000000000000000, 0.8660254037844387076, 1.000000000000000000, 0.8660254037844387076, 1.000000000000000000, 0.8660254037844387076, 1.000000000000000000, 0.8660254037844387076, 1.000000000000000000, 0.8660254037844387076, 1.000000000000000000, 0.8660254037844387076, 1.000000000000000000, 0.8660254037844387076, 1.000000000000000000, 0.8660254037844387076, 1.000000000000000000, 0.8660254037844387076, 1.000000000000000000, 0.8660254037844387076, 1.000000000000000000, 0.8660254037844387076, 1.000000000000000000, 0.8660254037844387076, 1.000000000000000000, 0.8660254037844387076, 1.000000000000000000, 0.8660254037844387076, 1.000000000000000000, 0.8660254037844387076, 1.000000000000000000, 0.8660254037844387076, 1.000000000000000000, 0.8660254037844387076, 1.000000000000000000, 0.8660254037844387076, 1.000000000000000000, 0.8660254037844387076, 1.000000000000000000, 0.8660254037844387076, 1.000000000000000000, 0.8660254037844387076, 1.000000000000000000, 0.8660254037844387076, 1.000000000000000000, 0.8660254037844387076, 1.000000000000000000, 0.8660254037844387076, 1.000000000000000000, 0.8660254037844387076, 1.000000000000000000, 0.8660254037844387076, 1.000000000000000000, 0.8660254037844387076, 1.000000000000000000, 0.8660254037844387076, 1.000000000000000000, 0.8660254037844387076, 1.000000000000000000, 0.8660254037844387076, 1.000000000000000000, 0.8660254037844387076, 1.000000000000000000, 0.8660254037844387076, 1.000000000000000000, 0.8660254037844387076, 1.000000000000000000, 0.8660254037844387076, 1.000000000000000000, 0.8660254037844387076, 1.000000000000000000, 0.8660254037844387076, 1.000000000000000000, 0.8660254037844387076, 1.000000000000000000, 0.8660254037844387076, 1.000000000000000000, 0.8660254037844387076, 1.000000000000000000, 0.8660254037844387076, 1.000000000000000000, 0.8660254037844387076, 1.000000000000000000, 0.8660254037844387076, 1.000000000000000000, 0.8660254037844387076, 1.000000000000000000, 0.8660254037844387076, 1.000000000000000000, 0.8660254037844387076, 1.000000000000000000, 0.8660254037844387076, 1.000000000000000000, 0.8660254037844387076, 1.000000000000000000, 0.8660254037844387076, 1.000000000000000000, 0.8660254037844387076, 1.000000000000000000, 0.8660254037844387076, 1.000000000000000000, 0.8660254037844387076, 1.000000000000000000, 0.8660254037844387076, 1.000000000000000000, 0.8660254037844387076, 1.000000000000000000, 0.8660254037844387076, 1.000000000000000000, 0.8660254037844387076, 1.000000000000000000, 0.8660254037844387076, 1.000000000000000000, 0.8660254037844387076, 1.000000000000000000, 0.8660254037844387076, 1.000000000000000000, 0.8660254037844387076, 1.000000000000000000, 0.8660254037844387076, 1.000000000000000000, 0.8660254037844387076, 1.000000000000000000, 0.8660254037844387076, 1.000000000000000000, 0.8660254037844387076, 1.000000000000000000, 0.8660254037844387076, 1.000000000000000000, 0.8660254037844387076, 1.000000000000000000, 0.8660254037844387076, 1.000000000000000000, 0.8660254037844387076, 1.000000000000000000, 0.8660254037844387076, 1.000000000000000000, 0.8660254037844387076, 1.000000000000000000, 0.8660254037844387076, 1.000000000000000000, 0.8660254037844387076, 1.000000000000000000, 0.8660254037844387076, 1.000000000000000000, 0.8660254037844387076, 1.000000000000000000, 0.8660254037844387076, 1.000000000000000000, 0.8660254037844387076, 1.000000000000000000, 0.8660254037844387076, 1.000000000000000000, 0.8660254037844387076, 1.000000000000000000, 0.8660254037844387076, 1.000000000000000000, 0.8660254037844387076, 1.000000000000000000, 0.8660254037844387076, 1.000000000000000000, 0.8660254037844387076, 1.000000000000000000, 0.8660254037844387076, 1.000000000000000000, 0.8660254037844387076, 1.000000000000000000, 0.8660254037844387076, 1.000000000000000000, 0.8660254037844387076, 1.000000000000000000, 0.8660254037844387076, 1.000000000000000000, 0.8660254037844387076, 1.000000000000000000, 0.8660254037844387076, 1.000000000000000000, 0.8660254037844387076, 1.000000000000000000, 0.8660254037844387076, 1.000000000000000000, 0.8660254037844387076, 1.000000000000000000, 0.8660254037844387076, 1.000000000000000000, 0.8660254037844387076, 1.000000000000000000, 0.8660254037844387076, 1.000000000000000000, 0.8660254037844387076, 1.000000000000000000, 0.8660254037844387076, 1.000000000000000000, 0.8660254037844387076, 1.000000000000000000, 0.8660254037844387076, 1.000000000000000000, 0.8660254037844387076, 1.000000000000000000, 0.8660254037844387076, 1.000000000000000000, 0.8660254037844387076, 1.000000000000000000, 0.8660254037844387076, 1.000000000000000000, 0.8660254037844387076, 1.000000000000000000, 0.8660254037844387076, 1.000000000000000000, 0.8660254037844387076, 1.000000000000000000, 0.8660254037844387076, 1.000000000000000000, 0.8660254037844387076, 1.000000000000000000, 0.8660254037844387076, 1.000000000000000000, 0.8660254037844387076, 1.000000000000000000, 0.8660254037844387076, 1.000000000000000000, 0.8660254037844387076, 1.000000000000000000, 0.8660254037844387076, 1.000000000000000000, 0.8660254037844387076, 1.000000000000000000, 0.8660254037844387076, 1.000000000000000000, 0.8660254037844387076, 1.000000000000000000, 0.8660254037844387076, 1.000000000000000000, 0.8660254037844387076, 1.000000000000000000, 0.8660254037844387076, 1.000000000000000000, 0.8660254037844387076, 1.000000000000000000, 0.8660254037844387076, 1.000000000000000000, 0.8660254037844387076, 1.000000000000000000, 0.8660254037844387076, 1.000000000000000000, 0.8660254037844387076, 1.000000000000000000, 0.8660254037844387076, 1.000000000000000000, 0.8660254037844387076, 1.000000000000000000, 0.8660254037844387076, 1.000000000000000000, 0.8660254037844387076, 1.000000000000000000, 0.8660254037844387076, 1.000000000000000000, 0.8660254037844387076, 1.000000000000000000, 0.8660254037844387076, 1.000000000000000000, 0.8660254037844387076, 1.000000000000000000, 0.8660254037844387076, 1.000000000000000000, 0.8660254037844387076, 1.000000000000000000, 0.8660254037844387076, 1.000000000000000000, 0.8660254037844387076, 1.000000000000000000, 0.8660254037844387076, 1.000000000000000000, 0.8660254037844387076, 1.000000000000000000, 0.8660254037844387076, 1.000000000000000000, 0.8660254037844387076, 1.000000000000000000, 0.8660254037844387076, 1.000000000000000000, 0.8660254037844387076, 1.000000000000000000, 0.8660254037844387076, 1.000000000000000000, 0.8660254037844387076, 1.000000000000000000, 0.8660254037844387076, 1.000000000000000000, 0.8660254037844387076, 1.000000000000000000, 0.8660254037844387076, 1.000000000000000000, 0.8660254037844387076, 1.000000000000000000, 0.8660254037844387076, 1.000000000000000000, 0.8660254037844387076, 1.000000000000000000, 0.8660254037844387076, 1.000000000000000000, 0.8660254037844387076, 1.000000000000000000, 0.8660254037844387076, 1.000000000000000000, 0.8660254037844387076, 1.000000000000000000, 0.8660254037844387076, 1.000000000000000000, 0.8660254037844387076, 1.000000000000000000, 0.8660254037844387076, 1.000000000000000000, 0.8660254037844387076, 1.000000000000000000, 0.8660254037844387076, 1.000000000000000000, 0.8660254037844387076, 1.000000000000000000, 0.8660254037844387076, 1.000000000000000000, 0.8660254037844387076, 1.000000000000000000, 0.8660254037844387076, 1.000000000000000000, 0.8660254037844387076, 1.000000000000000000, 0.8660254037844387076, 1.000000000000000000, 0.8660254037844387076, 1.000000000000000000, 0.8660254037844387076, 1.000000000000000000, 0.8660254037844387076, 1.000000000000000000, 0.8660254037844387076, 1.000000000000000000, 0.8660254037844387076, 1.000000000000000000, 0.8660254037844387076, 1.000000000000000000, 0.8660254037844387076, 1.000000000000000000, 0.8660254037844387076, 1.000000000000000000, 0.8660254037844387076, 1.000000000000000000, 0.8660254037844387076, 1.000000000000000000, 0.8660254037844387076, 1.000000000000000000, 0.8660254037844387076, 1.000000000000000000, 0.8660254037844387076, 1.000000000000000000, 0.8660254037844387076, 1.000000000000000000, 0.8660254037844387076, 1.000000000000000000, 0.8660254037844387076, 1.000000000000000000, 0.8660254037844387076, 1.000000000000000000, 0.8660254037844387076, 1.000000000000000000, 0.8660254037844387076, 1.000000000000000000, 0.8660254037844387076, 1.000000000000000000, 0.8660254037844387076, 1.000000000000000000, 0.8660254037844387076, 1.000000000000000000, 0.8660254037844387076, 1.000000000000000000, 0.8660254037844387076, 1.000000000000000000, 0.8660254037844387076, 1.000000000000000000, 0.8660254037844387076, 1.000000000000000000, 0.8660254037844387076, 1.000000000000000000, 0.8660254037844387076, 1.000000000000000000, 0.8660254037844387076, 1.000000000000000000, 0.8660254037844387076, 1.000000000000000000, 0.8660254037844387076, 1.000000000000000000, 0.8660254037844387076, 1.000000000000000000, 0.8660254037844387076, 1.000000000000000000, 0.8660254037844387076, 1.000000000000000000, 0.8660254037844387076, 1.000000000000000000, 0.8660254037844387076, 1.000000000000000000, 0.8660254037844387076, 1.000000000000000000, 0.8660254037844387076, 1.000000000000000000, 0.8660254037844387076, 1.000000000000000000, 0.8660254037844387076, 1.000000000000000000, 0.8660254037844387076, 1.000000000000000000, 0.8660254037844387076, 1.000000000000000000, 0.8660254037844387076, 1.000000000000000000, 0.8660254037844387076, 1.000000000000000000, 0.8660254037844387076, 1.000000000000000000, 0.8660254037844387076, 1.000000000000000000, 0.8660254037844387076, 1.000000000000000000, 0.8660254037844387076, 1.000000000000000000, 0.8660254037844387076, 1.000000000000000000, 0.8660254037844387076, 1.000000000000000000, 0.8660254037844387076, 1.000000000000000000, 0.8660254037844387076, 1.000000000000000000, 0.8660254037844387076, 1.000000000000000000, 0.8660254037844387076, 1.000000000000000000, 0.8660254037844387076, 1.000000000000000000, 0.8660254037844387076, 1.000000000000000000, 0.8660254037844387076, 1.000000000000000000, 0.8660254037844387076, 1.000000000000000000, 0.8660254037844387076, 1.000000000000000000, 0.8660254037844387076, 1.000000000000000000, 0.8660254037844387076, 1.000000000000000000, 0.8660254037844387076, 1.000000000000000000, 0.8660254037844387076, 1.000000000000000000, 0.8660254037844387076, 1.000000000000000000, 0.8660254037844387076, 1.000000000000000000, 0.8660254037844387076, 1.000000000000000000, 0.8660254037844387076, 1.000000000000000000, 0.8660254037844387076, 1.000000000000000000, 0.8660254037844387076, 1.000000000000000000, 0.8660254037844387076, 1.000000000000000000, 0.8660254037844387076, 1.000000000000000000, 0.8660254037844387076, 1.000000000000000000, 0.8660254037844387076, 1.000000000000000000, 0.8660254037844387076, 1.000000000000000000, 0.8660254037844387076, 1.000000000000000000, 0.8660254037844387076, 1.000000000000000000, 0.8660254037844387076, 1.000000000000000000, 0.8660254037844387076, 1.000000000000000000, 0.8660254037844387076, 1.000000000000000000, 0.8660254037844387076, 1.000000000000000000, 0.8660254037844387076, 1.000000000000000000, 0.8660254037844387076, 1.000000000000000000, 0.8660254037844387076, 1.000000000000000000, 0.8660254037844387076, 1.000000000000000000, 0.8660254037844387076, 1.000000000000000000, 0.8660254037844387076, 1.000000000000000000, 0.8660254037844387076, 1.000000000000000000, 0.8660254037844387076, 1.000000000000000000, 0.8660254037844387076, 1.000000000000000000, 0.8660254037844387076, 1.000000000000000000, 0.8660254037844387076, 1.000000000000000000, 0.8660254037844387076, 1.000000000000000000, 0.8660254037844387076, 1.000000000000000000, 0.8660254037844387076, 1.000000000000000000, 0.8660254037844387076, 1.000000000000000000, 0.8660254037844387076, 1.000000000000000000, 0.8660254037844387076, 1.000000000000000000, 0.8660254037844387076, 1.000000000000000000, 0.8660254037844387076, 1.000000000000000000, 0.8660254037844387076, 1.000000000000000000, 0.8660254037844387076, 1.000000000000000000, 0.8660254037844387076, 1.000000000000000000, 0.8660254037844387076, 1.000000000000000000, 0.8660254037844387076, 1.000000000000000000, 0.8660254037844387076, 1.000000000000000000, 0.8660254037844387076, 1.000000000000000000, 0.8660254037844387076, 1.000000000000000000, 0.8660254037844387076, 1.000000000000000000, 0.8660254037844387076, 1.000000000000000000, 0.8660254037844387076, 1.000000000000000000, 0.8660254037844387076, 1.000000000000000000, 0.8660254037844387076, 1.000000000000000000, 0.8660254037844387076, 1.000000000000000000, 0.8660254037844387076, 1.000000000000000000, 0.8660254037844387076, 1.000000000000000000, 0.8660254037844387076, 1.000000000000000000, 0.8660254037844387076, 1.000000000000000000, 0.8660254037844387076, 1.000000000000000000, 0.8660254037844387076, 1.000000000000000000, 0.8660254037844387076, 1.000000000000000000, 0.8660254037844387076, 1.000000000000000000, 0.8660254037844387076, 1.000000000000000000, 0.8660254037844387076, 1.000000000000000000, 0.8660254037844387076, 1.000000000000000000, 0.8660254037844387076, 1.000000000000000000, 0.8660254037844387076, 1.000000000000000000, 0.8660254037844387076, 1.000000000000000000, 0.8660254037844387076, 1.000000000000000000, 0.8660254037844387076, 1.000000000000000000, 0.8660254037844387076, 1.000000000000000000, 0.8660254037844387076, 1.000000000000000000, 0.8660254037844387076, 1.000000000000000000, 0.8660254037844387076, 1.000000000000000000, 0.8660254037844387076, 1.000000000000000000, 0.8660254037844387076, 1.000000000000000000, 0.8660254037844387076, 1.000000000000000000, 0.8660254037844387076, 1.000000000000000000, 0.8660254037844387076, 1.000000000000000000, 0.8660254037844387076, 1.000000000000000000, 0.8660254037844387076, 1.000000000000000000, 0.8660254037844387076, 1.000000000000000000, 0.8660254037844387076, 1.000000000000000000, 0.8660254037844387076, 1.000000000000000000, 0.8660254037844387076, 1.000000000000000000, 0.8660254037844387076, 1.000000000000000000, 0.8660254037844387076, 1.000000000000000000, 0.8660254037844387076, 1.000000000000000000, 0.8660254037844387076, 1.000000000000000000, 0.8660254037844387076, 1.000000000000000000, 0.8660254037844387076, 1.000000000000000000, 0.8660254037844387076, 1.000000000000000000, 0.8660254037844387076, 1.000000000000000000, 0.8660254037844387076, 1.000000000000000000, 0.8660254037844387076, 1.000000000000000000, 0.8660254037844387076, 1.000000000000000000, 0.8660254037844387076, 1.000000000000000000, 0.8660254037844387076, 1.000000000000000000, 0.8660254037844387076, 1.000000000000000000, 0.8660254037844387076, 1.000000000000000000, 0.8660254037844387076, 1.000000000000000000, 0.8660254037844387076, 1.000000000000000000, 0.8660254037844387076, 1.000000000000000000, 0.8660254037844387076, 1.000000000000000000, 0.8660254037844387076, 1.000000000000000000, 0.8660254037844387076, 1.000000000000000000, 0.8660254037844387076, 1.000000000000000000, 0.8660254037844387076, 1.000000000000000000, 0.8660254037844387076, 1.000000000000000000, 0.8660254037844387076, 1.000000000000000000, 0.8660254037844387076, 1.000000000000000000, 0.8660254037844387076, 1.000000000000000000, 0.8660254037844387076, 1.000000000000000000, 0.8660254037844387076, 1.000000000000000000, 0.8660254037844387076, 1.000000000000000000, 0.8660254037844387076, 1.000000000000000000, 0.8660254037844387076, 1.000000000000000000, 0.8660254037844387076, 1.000000000000000000, 0.8660254037844387076, 1.000000000000000000, 0.8660254037844387076, 1.000000000000000000, 0.8660254037844387076, 1.000000000000000000, 0.8660254037844387076, 1.000000000000000000, 0.8660254037844387076, 1.000000000000000000, 0.8660254037844387076, 1.000000000000000000, 0.8660254037844387076, 1.000000000000000000, 0.8660254037844387076, 1.000000000000000000, 0.8660254037844387076, 1.000000000000000000, 0.8660254037844387076, 1.000000000000000000, 0.8660254037844387076, 1.000000000000000000, 0.8660254037844387076, 1.000000000000000000, 0.8660254037844387076, 1.000000000000000000, 0.8660254037844387076, 1.000000000000000000, 0.8660254037844387076, 1.000000000000000000, 0.8660254037844387076, 1.000000000000000000, 0.8660254037844387076, 1.000000000000000000, 0.8660254037844387076, 1.000000000000000000, 0.8660254037844387076, 1.000000000000000000, 0.8660254037844387076, 1.000000000000000000, 0.8660254037844387076, 1.000000000000000000, 0.8660254037844387076, 1.000000000000000000, 0.8660254037844387076, 1.000000000000000000, 0.8660254037844387076, 1.000000000000000000, 0.8660254037844387076, 1.000000000000000000, 0.8660254037844387076, 1.000000000000000000, 0.8660254037844387076, 1.000000000000000000, 0.8660254037844387076, 1.000000000000000000, 0.8660254037844387076, 1.000000000000000000, 0.8660254037844387076, 1.000000000000000000, 0.8660254037844387076, 1.000000000000000000, 0.8660254037844387076, 1.000000000000000000, 0.8660254037844387076, 1.000000000000000000, 0.8660254037844387076, 1.000000000000000000, 0.8660254037844387076, 1.000000000000000000, 0.8660254037844387076, 1.000000000000000000, 0.8660254037844387076, 1.000000000000000000, 0.8660254037844387076, 1.000000000000000000, 0.8660254037844387076, 1.000000000000000000, 0.8660254037844387076, 1.000000000000000000, 0.8660254037844387076, 1.000000000000000000, 0.8660254037844387076, 1.000000000000000000, 0.8660254037844387076, 1.000000000000000000, 0.8660254037844387076, 1.000000000000000000, 0.8660254037844387076, 1.000000000000000000, 0.8660254037844387076, 1.000000000000000000, 0.8660254037844387076, 1.000000000000000000, 0.8660254037844387076, 1.000000000000000000, 0.8660254037844387076, 1.000000000000000000, 0.8660254037844387076, 1.000000000000000000, 0.8660254037844387076, 1.000000000000000000, 0.8660254037844387076, 1.000000000000000000, 0.8660254037844387076, 1.000000000000000000, 0.8660254037844387076, 1.000000000000000000, 0.8660254037844387076, 1.000000000000000000, 0.8660254037844387076, 1.000000000000000000, 0.8660254037844387076, 1.000000000000000000, 0.8660254037844387076, 1.000000000000000000, 0.8660254037844387076, 1.000000000000000000, 0.8660254037844387076, 1.000000000000000000, 0.8660254037844387076, 1.000000000000000000, 0.8660254037844387076, 1.000000000000000000, 0.8660254037844387076, 1.000000000000000000, 0.8660254037844387076, 1.000000000000000000, 0.8660254037844387076, 1.000000000000000000, 0.8660254037844387076, 1.000000000000000000, 0.8660254037844387076, 1.000000000000000000, 0.8660254037844387076, 1.000000000000000000, 0.8660254037844387076, 1.000000000000000000, 0.8660254037844387076, 1.000000000000000000, 0.8660254037844387076, 1.000000000000000000, 0.8660254037844387076, 1.000000000000000000, 0.8660254037844387076, 1.000000000000000000, 0.8660254037844387076, 1.000000000000000000, 0.8660254037844387076, 1.000000000000000000, 0.8660254037844387076, 1.000000000000000000, 0.8660254037844387076, 1.000000000000000000, 0.8660254037844387076, 1.000000000000000000, 0.8660254037844387076, 1.000000000000000000, 0.8660254037844387076, 1.000000000000000000, 0.8660254037844387076, 1.000000000000000000, 0.8660254037844387076, 1.000000000000000000, 0.8660254037844387076, 1.000000000000000000, 0.8660254037844387076, 1.000000000000000000, 0.8660254037844387076, 1.000000000000000000, 0.8660254037844387076, 1.000000000000000000, 0.8660254037844387076, 1.000000000000000000, 0.8660254037844387076, 1.000000000000000000, 0.8660254037844387076, 1.000000000000000000, 0.8660254037844387076, 1.000000000000000000, 0.8660254037844387076, 1.000000000000000000, 0.8660254037844387076, 1.000000000000000000, 0.8660254037844387076, 1.000000000000000000, 0.8660254037844387076, 1.000000000000000000, 0.8660254037844387076, 1.000000000000000000, 0.8660254037844387076, 1.000000000000000000, 0.8660254037844387076, 1.000000000000000000, 0.8660254037844387076, 1.000000000000000000, 0.8660254037844387076, 1.000000000000000000, 0.8660254037844387076, 1.000000000000000000, 0.8660254037844387076, 1.000000000000000000, 0.8660254037844387076, 1.000000000000000000, 0.8660254037844387076, 1.000000000000000000, 0.8660254037844387076, 1.000000000000000000, 0.8660254037844387076, 1.000000000000000000, 0.8660254037844387076, 1.000000000000000000, 0.8660254037844387076, 1.000000000000000000, 0.8660254037844387076, 1.000000000000000000, 0.8660254037844387076, 1.000000000000000000, 0.8660254037844387076, 1.000000000000000000, 0.8660254037844387076, 1.000000000000000000, 0.8660254037844387076, 1.000000000000000000, 0.8660254037844387076, 1.000000000000000000, 0.8660254037844387076, 1.000000000000000000, 0.8660254037844387076, 1.000000000000000000, 0.8660254037844387076, 1.000000000000000000, 0.8660254037844387076, 1.000000000000000000, 0.8660254037844387076, 1.000000000000000000, 0.8660254037844387076, 1.000000000000000000, 0.8660254037844387076, 1.000000000000000000, 0.8660254037844387076, 1.000000000000000000, 0.8660254037844387076, 1.000000000000000000, 0.8660254037844387076, 1.000000000000000000, 0.8660254037844387076, 1.000000000000000000, 0.8660254037844387076, 1.000000000000000000, 0.8660254037844387076, 1.000000000000000000, 0.8660254037844387076, 1.000000000000000000, 0.8660254037844387076, 1.000000000000000000, 0.8660254037844387076, 1.000000000000000000, 0.8660254037844387076, 1.000000000000000000, 0.8660254037844387076, 1.000000000000000000, 0.8660254037844387076, 1.000000000000000000, 0.8660254037844387076, 1.000000000000000000, 0.8660254037844387076, 1.000000000000000000, 0.8660254037844387076, 1.000000000000000000, 0.8660254037844387076, 1.000000000000000000, 0.8660254037844387076, 1.000000000000000000, 0.8660254037844387076, 1.000000000000000000, 0.8660254037844387076, 1.000000000000000000, 0.8660254037844387076, 1.000000000000000000, 0.8660254037844387076, 1.000000000000000000, 0.8660254037844387076, 1.000000000000000000, 0.8660254037844387076, 1.000000000000000000, 0.8660254037844387076, 1.000000000000000000, 0.8660254037844387076, 1.000000000000000000, 0.8660254037844387076, 1.000000000000000000, 0.8660254037844387076, 1.000000000000000000, 0.8660254037844387076, 1.000000000000000000, 0.8660254037844387076, 1.000000000000000000, 0.8660254037844387076, 1.000000000000000000, 0.8660254037844387076, 1.000000000000000000, 0.8660254037844387076, 1.000000000000000000, 0.8660254037844387076, 1.000000000000000000, 0.8660254037844387076, 1.000000000000000000, 0.8660254037844387076, 1.000000000000000000, 0.8660254037844387076, 1.000000000000000000, 0.8660254037844387076, 1.000000000000000000, 0.8660254037844387076, 1.000000000000000000, 0.8660254037844387076, 1.000000000000000000, 0.8660254037844387076, 1.000000000000000000, 0.8660254037844387076, 1.000000000000000000, 0.8660254037844387076, 1.000000000000000000, 0.8660254037844387076, 1.000000000000000000, 0.8660254037844387076, 1.000000000000000000, 0.8660254037844387076, 1.000000000000000000, 0.8660254037844387076, 1.000000000000000000, 0.8660254037844387076, 1.000000000000000000, 0.8660254037844387076, 1.000000000000000000, 0.8660254037844387076, 1.000000000000000000, 0.8660254037844387076, 1.000000000000000000, 0.8660254037844387076, 1.000000000000000000, 0.8660254037844387076, 1.000000000000000000, 0.8660254037844387076, 1.000000000000000000, 0.8660254037844387076, 1.000000000000000000, 0.8660254037844387076, 1.000000000000000000, 0.8660254037844387076, 1.000000000000000000, 0.8660254037844387076, 1.000000000000000000, 0.8660254037844387076, 1.000000000000000000, 0.8660254037844387076, 1.000000000000000000, 0.8660254037844387076, 1.000000000000000000, 0.8660254037844387076, 1.000000000000000000, 0.8660254037844387076, 1.000000000000000000, 0.8660254037844387076, 1.000000000000000000, 0.8660254037844387076, 1.000000000000000000, 0.8660254037844387076, 1.000000000000000000, 0.8660254037844387076, 1.000000000000000000, 0.8660254037844387076, 1.000000000000000000, 0.8660254037844387076, 1.000000000000000000, 0.8660254037844387076, 1.000000000000000000, 0.8660254037844387076, 1.000000000000000000, 0.8660254037844387076, 1.000000000000000000, 0.8660254037844387076, 1.000000000000000000, 0.8660254037844387076, 1.000000000000000000, 0.8660254037844387076, 1.000000000000000000, 0.8660254037844387076, 1.000000000000000000, 0.8660254037844387076, 1.000000000000000000, 0.8660254037844387076, 1.000000000000000000, 0.8660254037844387076, 1.000000000000000000, 0.8660254037844387076, 1.000000000000000000, 0.8660254037844387076, 1.000000000000000000, 0.8660254037844387076, 1.000000000000000000, 0.8660254037844387076, 1.000000000000000000, 0.8660254037844387076, 1.000000000000000000, 0.8660254037844387076, 1.000000000000000000, 0.8660254037844387076, 1.000000000000000000, 0.8660254037844387076, 1.000000000000000000, 0.8660254037844387076, 1.000000000000000000, 0.8660254037844387076, 1.000000000000000000, 0.8660254037844387076, 1.000000000000000000, 0.8660254037844387076, 1.000000000000000000, 0.8660254037844387076, 1.000000000000000000, 0.8660254037844387076, 1.000000000000000000, 0.8660254037844387076, 1.000000000000000000, 0.8660254037844387076, 1.000000000000000000, 0.8660254037844387076, 1.000000000000000000, 0.8660254037844387076, 1.000000000000000000, 0.8660254037844387076, 1.000000000000000000, 0.8660254037844387076, 1.000000000000000000, 0.9486992175574315844, 0.9366860366984544051 ) ) 
 REPRESENTATION_ITEM ( '' )  );
#3614=CARTESIAN_POINT ( 'NONE',  ( 10.81189881249999551, -6.242252689847874514, -73.46875000204835260 ) ) ;
#3615=CARTESIAN_POINT ( 'NONE',  ( -10.00000000000076916, 5.773502691895813221, -104.8749999999999716 ) ) ;
#3616=CARTESIAN_POINT ( 'NONE',  ( -10.81189881249999729, 6.242252689847871849, -194.2187500020483810 ) ) ;
#3617=CARTESIAN_POINT ( 'NONE',  ( -2.293366432827344421E-15, -12.48450537969573659, -151.7187500020483810 ) ) ;
#3618=DIRECTION ( 'NONE',  ( -0.000000000000000000, -0.000000000000000000, 1.000000000000000000 ) ) ;
#3619=CARTESIAN_POINT ( 'NONE',  ( -9.999999999999998224, 1.224646799147353059E-15, -189.1250000040967905 ) ) ;
#3621=CARTESIAN_POINT ( 'NONE',  ( -9.999999999999998224, 5.773502691896259087, -4.750000004096766482 ) ) ;
#3622=AXIS2_PLACEMENT_3D ( 'NONE', #34855, #7285, #27729 ) ;
#3623=DIRECTION ( 'NONE',  ( 1.000000000000000000, 0.000000000000000000, 0.000000000000000000 ) ) ;
#3624=CARTESIAN_POINT ( 'NONE',  ( -10.81189881249999729, 1.324075727343319199E-15, -119.0937500020483810 ) ) ;
#3626=CARTESIAN_POINT ( 'NONE',  ( -10.81189881249999729, 6.242252689847871849, -92.40625000204838102 ) ) ;
#3627=CARTESIAN_POINT ( 'NONE',  ( 10.81189881249999729, 6.242252689847867408, -107.7187500020483810 ) ) ;
#3630=CARTESIAN_POINT ( 'NONE',  ( 10.00000000000000000, 5.773502691896255534, -159.7500000040967905 ) ) ;
#3634=EDGE_CURVE ( 'NONE', #33917, #3910, #37833, .T. ) ;
#3639=CARTESIAN_POINT ( 'NONE',  ( -10.00000000000000000, -5.773502691896251982, -77.62499999999998579 ) ) ;
#3641=CARTESIAN_POINT ( 'NONE',  ( 10.00000000000000000, 5.773502691896255534, -93.75000000409677625 ) ) ;
#3644=CARTESIAN_POINT ( 'NONE',  ( 10.81189881249999729, 0.000000000000000000, -87.03125000204838102 ) ) ;
#3645=ORIENTED_EDGE ( 'NONE', *, *, #22928, .T. ) ;
#3650=CARTESIAN_POINT ( 'NONE',  ( -9.999999999999998224, 1.224646799147353059E-15, -10.24999999999995381 ) ) ;
#3651=CARTESIAN_POINT ( 'NONE',  ( 9.999999999999996447, -5.773502691896262640, -144.6250000000000000 ) ) ;
#3652=CARTESIAN_POINT ( 'NONE',  ( 0.000000000000000000, 0.000000000000000000, -200.0000000000000000 ) ) ;
#3655=CARTESIAN_POINT ( 'NONE',  ( 7.070501591499377789E-16, 11.54700538379251284, -189.1250000000000000 ) ) ;
#3656=CARTESIAN_POINT ( 'NONE',  ( 9.999999999999998224, 0.000000000000000000, -96.49999999999998579 ) ) ;
#3657=CARTESIAN_POINT ( 'NONE',  ( 10.81189881249999729, 0.000000000000000000, -117.0312500020483952 ) ) ;
#3659=VERTEX_POINT ( 'NONE', #33966 ) ;
#3660=CARTESIAN_POINT ( 'NONE',  ( -5.405949406250003975, -9.363379034771801557, -47.03125000204838813 ) ) ;
#3662=CARTESIAN_POINT ( 'NONE',  ( 7.644554776091147741E-16, 12.48450537969573659, -95.46875000204839523 ) ) ;
#3663=CARTESIAN_POINT ( 'NONE',  ( -5.405949406249996869, 9.363379034771805109, -124.0312500020483952 ) ) ;
#3665=DIRECTION ( 'NONE',  ( 1.000000000000000000, 0.000000000000000000, 0.000000000000000000 ) ) ;
#3668=CARTESIAN_POINT ( 'NONE',  ( 9.999999999999998224, 0.000000000000000000, -159.5000000000000000 ) ) ;
#3669=CARTESIAN_POINT ( 'NONE',  ( 7.644554776091147741E-16, 12.48450537969573659, -135.9687500020483810 ) ) ;
#3670=( BOUNDED_CURVE ( )  B_SPLINE_CURVE ( 2, ( #710, #40588, #33936, #1342, #17929, #503, #13618 ),
 .UNSPECIFIED., .F., .F. ) 
 B_SPLINE_CURVE_WITH_KNOTS ( ( 3, 2, 2, 3 ),
 ( 0.1007462686567163757, 0.1019900497512437887, 0.1032338308457712017, 0.1044776119402986148 ),
 .UNSPECIFIED. ) 
 CURVE ( )  GEOMETRIC_REPRESENTATION_ITEM ( )  RATIONAL_B_SPLINE_CURVE ( ( 1.000000000000004441, 0.8660254037844342667, 1.000000000000000000, 0.8660254037844387076, 1.000000000000000000, 0.8660254037844267172, 1.000000000000011990 ) ) 
 REPRESENTATION_ITEM ( '' )  );
#3672=CARTESIAN_POINT ( 'NONE',  ( 10.00000000000051159, -5.773502691895965988, -44.12499999999996447 ) ) ;
#3674=CARTESIAN_POINT ( 'NONE',  ( -2.121150477449813534E-15, -11.54700538379251284, -184.2500000040967905 ) ) ;
#3676=CARTESIAN_POINT ( 'NONE',  ( 7.644554776091147741E-16, 12.48450537969573659, -182.6562500020484094 ) ) ;
#3677=EDGE_CURVE ( 'NONE', #16045, #795, #18788, .T. ) ;
#3678=FACE_OUTER_BOUND ( 'NONE', #38998, .T. ) ;
#3679=CARTESIAN_POINT ( 'NONE',  ( -9.999999999999998224, 1.224646799147353059E-15, -184.6250000040967905 ) ) ;
#3681=CARTESIAN_POINT ( 'NONE',  ( -10.81189881249999729, -6.242252689847864744, -57.46875000204836681 ) ) ;
#3682=CARTESIAN_POINT ( 'NONE',  ( -10.81189881249999907, -6.242252689847864744, -40.96875000204834549 ) ) ;
#3684=CARTESIAN_POINT ( 'NONE',  ( 10.81189881249999729, 0.000000000000000000, -21.03125000204836326 ) ) ;
#3688=CARTESIAN_POINT ( 'NONE',  ( -9.999999999999998224, 5.773502691896259087, -109.3750000000000000 ) ) ;
#3693=CARTESIAN_POINT ( 'NONE',  ( -10.81189881249999729, 6.242252689847871849, -105.9062500020483810 ) ) ;
#3694=ORIENTED_EDGE ( 'NONE', *, *, #5638, .T. ) ;
#3697=CARTESIAN_POINT ( 'NONE',  ( 9.999999999999998224, 0.000000000000000000, -200.0000000000000000 ) ) ;
#3700=CARTESIAN_POINT ( 'NONE',  ( -2.121150477449813534E-15, -11.54700538379251284, -30.87499999999995381 ) ) ;
#3701=CARTESIAN_POINT ( 'NONE',  ( -4.999999999999996447, 8.660254037844387298, -21.37500000409675494 ) ) ;
#3702=CARTESIAN_POINT ( 'NONE',  ( 5.405949406249992428, -9.363379034771808662, -45.28125000204838102 ) ) ;
#3703=CARTESIAN_POINT ( 'NONE',  ( 9.999999999999998224, 0.000000000000000000, -200.0000000000000000 ) ) ;
#3706=CARTESIAN_POINT ( 'NONE',  ( -10.81189881249999729, 6.242252689847871849, -140.4062500020484094 ) ) ;
#3708=CARTESIAN_POINT ( 'NONE',  ( 9.999999999999998224, 0.000000000000000000, -200.0000000000000000 ) ) ;
#3709=ORIENTED_EDGE ( 'NONE', *, *, #5480, .F. ) ;
#3710=EDGE_LOOP ( 'NONE', ( #40304, #16626, #8914, #34396 ) ) ;
#3711=VERTEX_POINT ( 'NONE', #18397 ) ;
#3713=FACE_OUTER_BOUND ( 'NONE', #41486, .T. ) ;
#3714=( BOUNDED_CURVE ( )  B_SPLINE_CURVE ( 2, ( #9803, #32493, #3128, #39575, #33126, #13442, #6158 ),
 .UNSPECIFIED., .F., .F. ) 
 B_SPLINE_CURVE_WITH_KNOTS ( ( 3, 2, 2, 3 ),
 ( 0.6305970149253732338, 0.6318407960199006190, 0.6330845771144280043, 0.6343283582089553896 ),
 .UNSPECIFIED. ) 
 CURVE ( )  GEOMETRIC_REPRESENTATION_ITEM ( )  RATIONAL_B_SPLINE_CURVE ( ( 0.9999999999999880096, 0.8660254037844506980, 1.000000000000000000, 0.8660254037844387076, 1.000000000000000000, 0.8660254037844267172, 1.000000000000011990 ) ) 
 REPRESENTATION_ITEM ( '' )  );
#3715=CARTESIAN_POINT ( 'NONE',  ( 5.405949406249992428, -9.363379034771808662, -171.0937500020484094 ) ) ;
#3717=CARTESIAN_POINT ( 'NONE',  ( 10.81189881249999907, 6.242252689847868297, -25.21875000204837036 ) ) ;
#3719=CARTESIAN_POINT ( 'NONE',  ( 0.000000000000000000, 0.000000000000000000, -200.0000000000000000 ) ) ;
#3720=CARTESIAN_POINT ( 'NONE',  ( 5.405949406249999534, 9.363379034771803333, -152.5937500020483810 ) ) ;
#3721=CARTESIAN_POINT ( 'NONE',  ( 10.81189881249999551, -6.242252689847874514, -136.4687500020483810 ) ) ;
#3724=CARTESIAN_POINT ( 'NONE',  ( -10.81189881249999729, 1.324075727343319199E-15, -14.09375000204834905 ) ) ;
#3727=CYLINDRICAL_SURFACE ( 'NONE', #28925, 9.999999999999998224 ) ;
#3729=CARTESIAN_POINT ( 'NONE',  ( 9.999999999998969713, 5.773502691896851502, -56.25000000409675494 ) ) ;
#3730=CARTESIAN_POINT ( 'NONE',  ( 10.81189881249999729, 6.242252689847867408, -83.71875000204836681 ) ) ;
#3731=CARTESIAN_POINT ( 'NONE',  ( -2.293366432827344421E-15, -12.48450537969573659, -75.21875000204839523 ) ) ;
#3732=CARTESIAN_POINT ( 'NONE',  ( -5.405949406249996869, 9.363379034771805109, -43.03125000204838102 ) ) ;
#3734=CARTESIAN_POINT ( 'NONE',  ( -9.999999999999479527, -5.773502691896549521, -139.5000000040967620 ) ) ;
#3736=CARTESIAN_POINT ( 'NONE',  ( 9.999999999999998224, 0.000000000000000000, -131.0000000000000000 ) ) ;
#3737=CARTESIAN_POINT ( 'NONE',  ( -5.405949406249996869, 9.363379034771805109, -140.5312500020484094 ) ) ;
#3743=CARTESIAN_POINT ( 'NONE',  ( -9.999999999999998224, 1.224646799147353059E-15, -200.0000000000000000 ) ) ;
#3744=CARTESIAN_POINT ( 'NONE',  ( 5.405949406249999534, 9.363379034771803333, -167.7812500020484094 ) ) ;
#3745=CARTESIAN_POINT ( 'NONE',  ( 9.999999999999998224, 0.000000000000000000, -44.37500000409677625 ) ) ;
#3746=DIRECTION ( 'NONE',  ( 1.000000000000000000, 0.000000000000000000, 0.000000000000000000 ) ) ;
#3748=CARTESIAN_POINT ( 'NONE',  ( 10.81189881249999551, -6.242252689847874514, -159.1562500020484094 ) ) ;
#3749=CARTESIAN_POINT ( 'NONE',  ( 5.405949406249992428, -9.363379034771808662, -138.0937500020483810 ) ) ;
#3750=CARTESIAN_POINT ( 'NONE',  ( -9.999999999999998224, 1.224646799147353059E-15, -200.0000000000000000 ) ) ;
#3751=CARTESIAN_POINT ( 'NONE',  ( 5.000000000000000000, 8.660254037844385522, -150.2500000000000000 ) ) ;
#3753=EDGE_LOOP ( 'NONE', ( #37343, #15976, #39421, #31216 ) ) ;
#3754=EDGE_CURVE ( 'NONE', #16498, #28563, #32224, .T. ) ;
#3756=CARTESIAN_POINT ( 'NONE',  ( -10.81189881249999729, 6.242252689847871849, -72.90625000204838102 ) ) ;
#3757=VERTEX_POINT ( 'NONE', #8489 ) ;
#3759=CARTESIAN_POINT ( 'NONE',  ( -10.81189881249999729, 1.324075727343319199E-15, -116.0937500020483810 ) ) ;
#3760=ORIENTED_EDGE ( 'NONE', *, *, #6144, .F. ) ;
#3761=CARTESIAN_POINT ( 'NONE',  ( -10.81189881249999729, 1.324075727343319199E-15, -23.09375000204835615 ) ) ;
#3762=CARTESIAN_POINT ( 'NONE',  ( 10.81189881249999729, 0.000000000000000000, -1.531250002048373249 ) ) ;
#3763=CARTESIAN_POINT ( 'NONE',  ( -5.405949406249996869, 9.363379034771805109, -50.34375000204835260 ) ) ;
#3765=FACE_OUTER_BOUND ( 'NONE', #29723, .T. ) ;
#3766=CARTESIAN_POINT ( 'NONE',  ( 5.405949406249992428, -9.363379034771808662, -180.0937500020484094 ) ) ;
#3767=CARTESIAN_POINT ( 'NONE',  ( 7.644554776091147741E-16, 12.48450537969573659, -170.4687500020483810 ) ) ;
#3770=CARTESIAN_POINT ( 'NONE',  ( 9.999999999999998224, 0.000000000000000000, -146.3750000040967905 ) ) ;
#3771=CARTESIAN_POINT ( 'NONE',  ( 9.999999999999872102, 5.773502691896329253, -193.8750000000000284 ) ) ;
#3773=CARTESIAN_POINT ( 'NONE',  ( -10.81189881249999907, -6.242252689847864744, -97.96875000204838102 ) ) ;
#3774=CARTESIAN_POINT ( 'NONE',  ( -10.00000000000102496, 5.773502691895664007, -34.37499999999994316 ) ) ;
#3775=CARTESIAN_POINT ( 'NONE',  ( 10.81189881249999551, -6.242252689847874514, -63.15625000204837391 ) ) ;
#3777=ADVANCED_FACE ( 'NONE', ( #12131 ), #31370, .T. ) ;
#3778=CARTESIAN_POINT ( 'NONE',  ( -10.81189881249999729, 1.324075727343319199E-15, -123.7812500020483952 ) ) ;
#3779=CARTESIAN_POINT ( 'NONE',  ( -5.405949406250003975, -9.363379034771801557, -159.5312500020484094 ) ) ;
#3781=CARTESIAN_POINT ( 'NONE',  ( 4.999999999999992006, -8.660254037844389075, -137.6250000040967620 ) ) ;
#3783=ORIENTED_EDGE ( 'NONE', *, *, #13665, .T. ) ;
#3784=VECTOR ( 'NONE', #4002, 1000.000000000000000 ) ;
#3787=CARTESIAN_POINT ( 'NONE',  ( -10.81189881249999729, 6.242252689847871849, -191.4062500020484094 ) ) ;
#3791=CARTESIAN_POINT ( 'NONE',  ( 9.999999999999996447, -5.773502691896262640, -54.62499999999996447 ) ) ;
#3793=CARTESIAN_POINT ( 'NONE',  ( -5.000000000000003553, -8.660254037844383745, -68.87500000409677625 ) ) ;
#3797=CARTESIAN_POINT ( 'NONE',  ( 10.81189881249999551, -6.242252689847874514, -57.15625000204837391 ) ) ;
#3800=CARTESIAN_POINT ( 'NONE',  ( 10.81189881249999907, 6.242252689847868297, -182.9062500020484094 ) ) ;
#3802=CARTESIAN_POINT ( 'NONE',  ( -9.999999999999998224, 1.224646799147353059E-15, -40.24999999999997868 ) ) ;
#3803=CARTESIAN_POINT ( 'NONE',  ( 0.000000000000000000, 0.000000000000000000, -200.0000000000000000 ) ) ;
#3804=EDGE_CURVE ( 'NONE', #17414, #18914, #11916, .T. ) ;
#3805=CARTESIAN_POINT ( 'NONE',  ( -9.999999999999998224, 1.224646799147353059E-15, -116.7499999999999858 ) ) ;
#3806=CARTESIAN_POINT ( 'NONE',  ( -9.885120488223384072, 1.745261150048159848, -0.000000000000000000 ) ) ;
#3808=ADVANCED_FACE ( 'NONE', ( #21641 ), #22074, .T. ) ;
#3809=CYLINDRICAL_SURFACE ( 'NONE', #33768, 9.999999999999998224 ) ;
#3811=CARTESIAN_POINT ( 'NONE',  ( -2.293366432827344421E-15, -12.48450537969573659, -96.40625000204839523 ) ) ;
#3815=ORIENTED_EDGE ( 'NONE', *, *, #21256, .T. ) ;
#3816=VERTEX_POINT ( 'NONE', #28345 ) ;
#3817=CARTESIAN_POINT ( 'NONE',  ( -10.81189881249999907, -6.242252689847864744, -30.46875000204834549 ) ) ;
#3818=VECTOR ( 'NONE', #15763, 1000.000000000000000 ) ;
#3819=CARTESIAN_POINT ( 'NONE',  ( 10.81189881249999907, 6.242252689847868297, -23.90625000204838102 ) ) ;
#3820=CARTESIAN_POINT ( 'NONE',  ( 10.81189881249999551, -6.242252689847874514, -68.96875000204839523 ) ) ;
#3823=EDGE_CURVE ( 'NONE', #32468, #18020, #32051, .T. ) ;
#3824=CARTESIAN_POINT ( 'NONE',  ( -10.81189881249999907, -6.242252689847864744, -196.9687500020484379 ) ) ;
#3825=CARTESIAN_POINT ( 'NONE',  ( -5.405949406249996869, 9.363379034771805109, -153.8437500020483810 ) ) ;
#3827=CARTESIAN_POINT ( 'NONE',  ( 9.999999999999998224, 0.000000000000000000, -174.8750000040967905 ) ) ;
#3830=CARTESIAN_POINT ( 'NONE',  ( 9.999999999999996447, -5.773502691896262640, -5.500000004096770034 ) ) ;
#3831=FACE_OUTER_BOUND ( 'NONE', #7684, .T. ) ;
#3832=CARTESIAN_POINT ( 'NONE',  ( 10.81189881249999551, -6.242252689847874514, -122.9687500020483810 ) ) ;
#3834=CARTESIAN_POINT ( 'NONE',  ( 7.644554776091147741E-16, 12.48450537969573659, -89.65625000204839523 ) ) ;
#3835=CARTESIAN_POINT ( 'NONE',  ( 7.644554776091147741E-16, 12.48450537969573659, -101.4687500020483668 ) ) ;
#3837=VECTOR ( 'NONE', #20697, 1000.000000000000000 ) ;
#3839=CARTESIAN_POINT ( 'NONE',  ( 10.00000000000000000, 5.773502691896255534, -158.2500000040967905 ) ) ;
#3840=( BOUNDED_CURVE ( )  B_SPLINE_CURVE ( 2, ( #21959, #18505, #27588, #8387, #25011, #11169, #38153 ),
 .UNSPECIFIED., .F., .F. ) 
 B_SPLINE_CURVE_WITH_KNOTS ( ( 3, 2, 2, 3 ),
 ( 0.4626865671641792743, 0.4639303482587066596, 0.4651741293532339339, 0.4664179104477613191 ),
 .UNSPECIFIED. ) 
 CURVE ( )  GEOMETRIC_REPRESENTATION_ITEM ( )  RATIONAL_B_SPLINE_CURVE ( ( 0.9999999999999820144, 0.8660254037844566932, 1.000000000000000000, 0.8660254037844387076, 1.000000000000000000, 0.8660254037844267172, 1.000000000000011990 ) ) 
 REPRESENTATION_ITEM ( '' )  );
#3844=CARTESIAN_POINT ( 'NONE',  ( 4.999999999999992006, -8.660254037844389075, -53.62500000409675494 ) ) ;
#3846=CARTESIAN_POINT ( 'NONE',  ( -9.999999999999998224, 5.773502691896259087, -83.87499999999998579 ) ) ;
#3848=CARTESIAN_POINT ( 'NONE',  ( -5.000000000000003553, -8.660254037844383745, -88.37500000409677625 ) ) ;
#3849=AXIS2_PLACEMENT_3D ( 'NONE', #1319, #24205, #10796 ) ;
#3852=CARTESIAN_POINT ( 'NONE',  ( -10.81189881249999729, 1.324075727343319199E-15, -84.78125000204838102 ) ) ;
#3853=ORIENTED_EDGE ( 'NONE', *, *, #24630, .F. ) ;
#3858=CARTESIAN_POINT ( 'NONE',  ( 4.999999999999992006, -8.660254037844389075, -12.74999999999995559 ) ) ;
#3860=CARTESIAN_POINT ( 'NONE',  ( -9.999999999999998224, 1.224646799147353059E-15, -148.2500000000000000 ) ) ;
#3863=CARTESIAN_POINT ( 'NONE',  ( 5.000000000000000000, 8.660254037844385522, -187.7500000000000000 ) ) ;
#3864=DIRECTION ( 'NONE',  ( -0.000000000000000000, -0.000000000000000000, 1.000000000000000000 ) ) ;
#3866=CARTESIAN_POINT ( 'NONE',  ( 7.644554776091147741E-16, 12.48450537969573659, -119.6562500020484094 ) ) ;
#3867=VERTEX_POINT ( 'NONE', #8911 ) ;
#3868=CARTESIAN_POINT ( 'NONE',  ( 5.000000000000000000, 8.660254037844385522, -36.62500000409676915 ) ) ;
#3869=ORIENTED_EDGE ( 'NONE', *, *, #4709, .F. ) ;
#3871=CARTESIAN_POINT ( 'NONE',  ( 10.81189881249999729, 0.000000000000000000, -43.53125000204838102 ) ) ;
#3873=EDGE_CURVE ( 'NONE', #31913, #1269, #5826, .T. ) ;
#3874=CARTESIAN_POINT ( 'NONE',  ( 5.405949406249992428, -9.363379034771808662, -93.09375000204838102 ) ) ;
#3875=CARTESIAN_POINT ( 'NONE',  ( -10.81189881249999729, -6.242252689847864744, -125.1562500020483810 ) ) ;
#3877=VECTOR ( 'NONE', #964, 1000.000000000000000 ) ;
#3878=CARTESIAN_POINT ( 'NONE',  ( 5.000000000000000000, 8.660254037844385522, -51.62500000409675494 ) ) ;
#3879=CARTESIAN_POINT ( 'NONE',  ( -2.293366432827344421E-15, -12.48450537969573659, -193.7187500020484094 ) ) ;
#3882=CARTESIAN_POINT ( 'NONE',  ( 7.644554776091147741E-16, 12.48450537969573659, -129.9687500020483810 ) ) ;
#3885=CARTESIAN_POINT ( 'NONE',  ( 7.070501591499377789E-16, 11.54700538379251284, -189.5000000040968189 ) ) ;
#3887=CARTESIAN_POINT ( 'NONE',  ( -10.81189881249999729, 1.324075727343319199E-15, -176.2812500020484094 ) ) ;
#3888=DIRECTION ( 'NONE',  ( -0.3779644730092261984, 0.6546536707079756434, -0.6546536707079793072 ) ) ;
#3891=CARTESIAN_POINT ( 'NONE',  ( -10.81189881249999729, 1.324075727343319199E-15, -62.09375000204836681 ) ) ;
#3892=CARTESIAN_POINT ( 'NONE',  ( 5.405949406249992428, -9.363379034771808662, -45.09375000204837391 ) ) ;
#3894=CARTESIAN_POINT ( 'NONE',  ( 10.81189881249999907, 6.242252689847868297, -17.90625000204837036 ) ) ;
#3898=CARTESIAN_POINT ( 'NONE',  ( 5.000000000000000000, 8.660254037844385522, -106.7499999999999858 ) ) ;
#3900=CARTESIAN_POINT ( 'NONE',  ( 10.00000000000051159, -5.773502691895965988, -49.00000000409676204 ) ) ;
#3904=CARTESIAN_POINT ( 'NONE',  ( -5.405949406249996869, 9.363379034771805109, -107.5312500020483810 ) ) ;
#3908=DIRECTION ( 'NONE',  ( -0.000000000000000000, -0.000000000000000000, 1.000000000000000000 ) ) ;
#3910=VERTEX_POINT ( 'NONE', #23131 ) ;
#3911=CARTESIAN_POINT ( 'NONE',  ( 4.999999999999992006, -8.660254037844389075, -32.24999999999997158 ) ) ;
#3912=CARTESIAN_POINT ( 'NONE',  ( -10.81189881249999729, -6.242252689847864744, -35.15625000204836681 ) ) ;
#3915=CARTESIAN_POINT ( 'NONE',  ( 5.000000000000000000, 8.660254037844385522, -57.62500000409676204 ) ) ;
#3916=CARTESIAN_POINT ( 'NONE',  ( -10.81189881249999907, -6.242252689847864744, -140.1562500020484094 ) ) ;
#3917=CARTESIAN_POINT ( 'NONE',  ( -9.999999999999998224, 1.224646799147353059E-15, -97.62500000409677625 ) ) ;
#3918=ORIENTED_EDGE ( 'NONE', *, *, #9375, .T. ) ;
#3919=ORIENTED_EDGE ( 'NONE', *, *, #30488, .F. ) ;
#3920=( BOUNDED_CURVE ( )  B_SPLINE_CURVE ( 2, ( #39230, #29110, #32980, #3409, #25867, #25658, #16327 ),
 .UNSPECIFIED., .F., .F. ) 
 B_SPLINE_CURVE_WITH_KNOTS ( ( 3, 2, 2, 3 ),
 ( 0.5820895522388062071, 0.5833333333333335924, 0.5845771144278607556, 0.5858208955223881409 ),
 .UNSPECIFIED. ) 
 CURVE ( )  GEOMETRIC_REPRESENTATION_ITEM ( )  RATIONAL_B_SPLINE_CURVE ( ( 0.9999999999999761302, 0.8660254037844625774, 1.000000000000000000, 0.8660254037844387076, 1.000000000000000000, 0.8660254037844267172, 1.000000000000011990 ) ) 
 REPRESENTATION_ITEM ( '' )  );
#3921=CARTESIAN_POINT ( 'NONE',  ( 5.000000000000000000, 8.660254037844385522, -159.2500000000000000 ) ) ;
#3922=LINE ( 'NONE', #9957, #4940 ) ;
#3923=CARTESIAN_POINT ( 'NONE',  ( 5.405949406249999534, 9.363379034771803333, -169.0937500020484094 ) ) ;
#3925=CARTESIAN_POINT ( 'NONE',  ( -5.405949406249996869, 9.363379034771805109, -20.34375000204835615 ) ) ;
#3927=CARTESIAN_POINT ( 'NONE',  ( -5.405949406250003975, -9.363379034771801557, -159.3437500020484094 ) ) ;
#3928=CARTESIAN_POINT ( 'NONE',  ( 5.405949406249999534, 9.363379034771803333, -137.5937500020483810 ) ) ;
#3929=DIRECTION ( 'NONE',  ( -0.000000000000000000, -0.000000000000000000, 1.000000000000000000 ) ) ;
#3933=CARTESIAN_POINT ( 'NONE',  ( 7.644554776091147741E-16, 12.48450537969573659, -9.968750002048363257 ) ) ;
#3935=EDGE_CURVE ( 'NONE', #26035, #1967, #2860, .T. ) ;
#3936=CARTESIAN_POINT ( 'NONE',  ( 5.000000000000000000, 8.660254037844385522, -5.125000004096769146 ) ) ;
#3939=CARTESIAN_POINT ( 'NONE',  ( -10.81189881249999729, 6.242252689847871849, -86.21875000204836681 ) ) ;
#3940=CARTESIAN_POINT ( 'NONE',  ( 10.81189881249999907, 6.242252689847868297, -64.21875000204838102 ) ) ;
#3941=CARTESIAN_POINT ( 'NONE',  ( -5.405949406249996869, 9.363379034771805109, -40.03125000204838102 ) ) ;
#3943=LINE ( 'NONE', #17507, #22667 ) ;
#3945=CARTESIAN_POINT ( 'NONE',  ( -4.999999999999996447, 8.660254037844387298, -127.5000000000000000 ) ) ;
#3946=CARTESIAN_POINT ( 'NONE',  ( 5.405949406249992428, -9.363379034771808662, -139.7812500020483810 ) ) ;
#3947=CARTESIAN_POINT ( 'NONE',  ( 10.00000000000025402, -5.773502691896113426, -187.0000000040967905 ) ) ;
#3949=CARTESIAN_POINT ( 'NONE',  ( 10.81189881249999551, -6.242252689847874514, -18.15625000204837036 ) ) ;
#3950=VERTEX_POINT ( 'NONE', #26157 ) ;
#3953=CARTESIAN_POINT ( 'NONE',  ( 7.070501591499376803E-16, 11.54700538379251284, -39.12499999999995737 ) ) ;
#3954=CARTESIAN_POINT ( 'NONE',  ( -5.000000000000003553, -8.660254037844383745, -38.87500000409676915 ) ) ;
#3955=CARTESIAN_POINT ( 'NONE',  ( -5.000000000000003553, -8.660254037844383745, -58.37500000409676204 ) ) ;
#3957=CARTESIAN_POINT ( 'NONE',  ( 7.070501591499376803E-16, 11.54700538379251284, -147.1250000000000000 ) ) ;
#3958=CARTESIAN_POINT ( 'NONE',  ( 5.405949406249992428, -9.363379034771808662, -150.2812500020483810 ) ) ;
#3959=CARTESIAN_POINT ( 'NONE',  ( 10.81189881249999729, 0.000000000000000000, -133.3437500020484094 ) ) ;
#3960=CARTESIAN_POINT ( 'NONE',  ( 10.00000000000051159, -5.773502691895965988, -115.0000000040967905 ) ) ;
#3961=ORIENTED_EDGE ( 'NONE', *, *, #22665, .T. ) ;
#3962=DIRECTION ( 'NONE',  ( 1.000000000000000000, 0.000000000000000000, 0.000000000000000000 ) ) ;
#3964=CARTESIAN_POINT ( 'NONE',  ( -10.81189881249999907, -6.242252689847864744, -63.65625000204836681 ) ) ;
#3965=ORIENTED_EDGE ( 'NONE', *, *, #14049, .F. ) ;
#3967=VECTOR ( 'NONE', #4032, 1000.000000000000000 ) ;
#3968=CARTESIAN_POINT ( 'NONE',  ( 10.81189881249999907, 6.242252689847868297, -112.2187500020483810 ) ) ;
#3969=VERTEX_POINT ( 'NONE', #6724 ) ;
#3970=CARTESIAN_POINT ( 'NONE',  ( 5.405949406249999534, 9.363379034771803333, -19.09375000204835260 ) ) ;
#3971=CARTESIAN_POINT ( 'NONE',  ( -5.405949406250003975, -9.363379034771801557, -190.8437500020484094 ) ) ;
#3972=CARTESIAN_POINT ( 'NONE',  ( -2.293366432827344421E-15, -12.48450537969573659, -49.71875000204835970 ) ) ;
#3973=CARTESIAN_POINT ( 'NONE',  ( 8.069781934609757457, -7.195427280628551969, 1.661355961043940754E-14 ) ) ;
#3974=CARTESIAN_POINT ( 'NONE',  ( 9.999999999998969713, 5.773502691896851502, -0.3749999999999439892 ) ) ;
#3975=CARTESIAN_POINT ( 'NONE',  ( -5.405949406250003975, -9.363379034771801557, -181.8437500020483810 ) ) ;
#3976=CARTESIAN_POINT ( 'NONE',  ( 5.405949406249992428, -9.363379034771808662, -160.5937500020484094 ) ) ;
#3979=CARTESIAN_POINT ( 'NONE',  ( -9.999999999999998224, 1.224646799147353059E-15, -128.7499999999999716 ) ) ;
#3981=CARTESIAN_POINT ( 'NONE',  ( -2.293366432827344421E-15, -12.48450537969573659, -85.71875000204838102 ) ) ;
#3982=CARTESIAN_POINT ( 'NONE',  ( 10.81189881249999907, 6.242252689847868297, -67.40625000204839523 ) ) ;
#3984=ADVANCED_FACE ( 'NONE', ( #42327 ), #33062, .T. ) ;
#3986=CARTESIAN_POINT ( 'NONE',  ( 5.405949406249999534, 9.363379034771803333, -125.7812500020483668 ) ) ;
#3987=CARTESIAN_POINT ( 'NONE',  ( -10.81189881249999729, -6.242252689847864744, -165.6562500020483810 ) ) ;
#3989=CARTESIAN_POINT ( 'NONE',  ( 9.999999999999998224, 0.000000000000000000, -137.3750000040967905 ) ) ;
#3991=ORIENTED_EDGE ( 'NONE', *, *, #36775, .F. ) ;
#3994=CARTESIAN_POINT ( 'NONE',  ( 10.81189881249999729, 0.000000000000000000, -190.5312500020484094 ) ) ;
#3996=VECTOR ( 'NONE', #6789, 1000.000000000000000 ) ;
#3998=CARTESIAN_POINT ( 'NONE',  ( 7.070501591499377789E-16, 11.54700538379251284, -51.12499999999998579 ) ) ;
#4000=CARTESIAN_POINT ( 'NONE',  ( -4.999999999999996447, 8.660254037844387298, -63.37500000409676204 ) ) ;
#4002=DIRECTION ( 'NONE',  ( -0.000000000000000000, -0.000000000000000000, 1.000000000000000000 ) ) ;
#4004=CARTESIAN_POINT ( 'NONE',  ( 10.81189881249999729, 6.242252689847867408, -58.40625000204838102 ) ) ;
#4008=CARTESIAN_POINT ( 'NONE',  ( 7.644554776091147741E-16, 12.48450537969573659, -188.6562500020484379 ) ) ;
#4010=LINE ( 'NONE', #23874, #23559 ) ;
#4012=CARTESIAN_POINT ( 'NONE',  ( 10.00000000000102318, -5.773502691895667560, -89.12499999999994316 ) ) ;
#4013=DIRECTION ( 'NONE',  ( 1.000000000000000000, 0.000000000000000000, 0.000000000000000000 ) ) ;
#4014=CARTESIAN_POINT ( 'NONE',  ( 4.999999999999992006, -8.660254037844389075, -122.2500000000000000 ) ) ;
#4015=CARTESIAN_POINT ( 'NONE',  ( -5.405949406250003975, -9.363379034771801557, -89.03125000204838102 ) ) ;
#4016=ORIENTED_EDGE ( 'NONE', *, *, #38610, .F. ) ;
#4018=ORIENTED_EDGE ( 'NONE', *, *, #16822, .T. ) ;
#4019=ORIENTED_EDGE ( 'NONE', *, *, #11969, .F. ) ;
#4020=CARTESIAN_POINT ( 'NONE',  ( -5.405949406250003975, -9.363379034771801557, -28.84375000204836326 ) ) ;
#4021=CARTESIAN_POINT ( 'NONE',  ( 5.405949406249992428, -9.363379034771808662, -24.28125000204836681 ) ) ;
#4023=CARTESIAN_POINT ( 'NONE',  ( 10.81189881249999551, -6.242252689847874514, -71.96875000204838102 ) ) ;
#4024=DIRECTION ( 'NONE',  ( 1.000000000000000000, 0.000000000000000000, 0.000000000000000000 ) ) ;
#4026=CARTESIAN_POINT ( 'NONE',  ( 10.81189881249999729, 0.000000000000000000, -182.8437500020483810 ) ) ;
#4027=CARTESIAN_POINT ( 'NONE',  ( -5.405949406249996869, 9.363379034771805109, -152.3437500020483810 ) ) ;
#4028=CARTESIAN_POINT ( 'NONE',  ( 10.81189881249999729, 0.000000000000000000, -1.343750002048366143 ) ) ;
#4029=CARTESIAN_POINT ( 'NONE',  ( -9.999999999999998224, 1.224646799147353059E-15, -200.0000000000000000 ) ) ;
#4030=CARTESIAN_POINT ( 'NONE',  ( -9.999999999999998224, 1.224646799147353059E-15, -200.0000000000000000 ) ) ;
#4031=CARTESIAN_POINT ( 'NONE',  ( -9.999999999999998224, 5.773502691896259087, -6.250000004096741613 ) ) ;
#4032=DIRECTION ( 'NONE',  ( -0.000000000000000000, -0.000000000000000000, 1.000000000000000000 ) ) ;
#4033=CARTESIAN_POINT ( 'NONE',  ( 5.405949406249999534, 9.363379034771803333, -119.5937500020483810 ) ) ;
#4035=CARTESIAN_POINT ( 'NONE',  ( 10.81189881249999907, 6.242252689847868297, -86.90625000204836681 ) ) ;
#4036=EDGE_CURVE ( 'NONE', #1094, #2019, #33435, .T. ) ;
#4037=CARTESIAN_POINT ( 'NONE',  ( 10.81189881249999729, 6.242252689847867408, -103.2187500020483810 ) ) ;
#4039=EDGE_CURVE ( 'NONE', #318, #26657, #20170, .T. ) ;
#4041=CARTESIAN_POINT ( 'NONE',  ( 7.070501591499377789E-16, 11.54700538379251284, -162.5000000040967905 ) ) ;
#4042=EDGE_CURVE ( 'NONE', #6810, #30574, #37832, .T. ) ;
#4049=CARTESIAN_POINT ( 'NONE',  ( -5.000000000000003553, -8.660254037844383745, -75.99999999999998579 ) ) ;
#4051=CARTESIAN_POINT ( 'NONE',  ( -2.121150477449813534E-15, -11.54700538379251284, -91.25000000409677625 ) ) ;
#4052=CARTESIAN_POINT ( 'NONE',  ( -9.999999999999998224, 1.224646799147353059E-15, -96.12500000409677625 ) ) ;
#4055=CARTESIAN_POINT ( 'NONE',  ( -5.405949406250003975, -9.363379034771801557, -83.03125000204838102 ) ) ;
#4057=CARTESIAN_POINT ( 'NONE',  ( -4.999999999999996447, 8.660254037844387298, -20.99999999999996447 ) ) ;
#4060=CARTESIAN_POINT ( 'NONE',  ( -10.00000000000000000, -5.773502691896251982, -8.624999999999976907 ) ) ;
#4062=CARTESIAN_POINT ( 'NONE',  ( -2.121150477449813534E-15, -11.54700538379251284, -143.3750000000000000 ) ) ;
#4063=CARTESIAN_POINT ( 'NONE',  ( -9.999999999999998224, 1.224646799147353059E-15, -45.12500000409677625 ) ) ;
#4066=CARTESIAN_POINT ( 'NONE',  ( -10.81189881249999729, 6.242252689847871849, -135.9062500020484094 ) ) ;
#4068=CARTESIAN_POINT ( 'NONE',  ( -9.999999999999998224, 1.224646799147353059E-15, -188.7500000000000000 ) ) ;
#4069=CARTESIAN_POINT ( 'NONE',  ( 4.999999999999992006, -8.660254037844389075, -184.1250000040967905 ) ) ;
#4070=VECTOR ( 'NONE', #12003, 1000.000000000000000 ) ;
#4071=CARTESIAN_POINT ( 'NONE',  ( 5.405949406249999534, 9.363379034771803333, -116.7812500020483952 ) ) ;
#4072=ORIENTED_EDGE ( 'NONE', *, *, #37286, .T. ) ;
#4073=CARTESIAN_POINT ( 'NONE',  ( -9.999999999999998224, 1.224646799147353059E-15, -13.24999999999995559 ) ) ;
#4074=ORIENTED_EDGE ( 'NONE', *, *, #12921, .F. ) ;
#4075=EDGE_LOOP ( 'NONE', ( #23803, #42412, #28178, #952 ) ) ;
#4077=CARTESIAN_POINT ( 'NONE',  ( 10.81189881249999907, 6.242252689847868297, -46.40625000204835970 ) ) ;
#4079=CARTESIAN_POINT ( 'NONE',  ( 10.81189881249999551, -6.242252689847874514, -97.46875000204838102 ) ) ;
#4080=CARTESIAN_POINT ( 'NONE',  ( -10.81189881249999729, -6.242252689847864744, -126.6562500020483810 ) ) ;
#4081=ORIENTED_EDGE ( 'NONE', *, *, #7202, .F. ) ;
#4082=EDGE_CURVE ( 'NONE', #10102, #41485, #6612, .T. ) ;
#4083=CARTESIAN_POINT ( 'NONE',  ( 7.070501591499376803E-16, 11.54700538379251284, -51.50000000409676204 ) ) ;
#4084=CARTESIAN_POINT ( 'NONE',  ( -2.293366432827344421E-15, -12.48450537969573659, -196.7187500020484094 ) ) ;
#4087=FACE_OUTER_BOUND ( 'NONE', #33392, .T. ) ;
#4088=CARTESIAN_POINT ( 'NONE',  ( 7.644554776091147741E-16, 12.48450537969573659, -126.9687500020483952 ) ) ;
#4091=CARTESIAN_POINT ( 'NONE',  ( 9.999999999999996447, -5.773502691896262640, -185.5000000040967905 ) ) ;
#4093=CARTESIAN_POINT ( 'NONE',  ( 7.644554776091147741E-16, 12.48450537969573659, -178.1562500020484094 ) ) ;
#4095=CARTESIAN_POINT ( 'NONE',  ( -4.999999999999996447, 8.660254037844387298, -121.8750000040967905 ) ) ;
#4097=CARTESIAN_POINT ( 'NONE',  ( 10.81189881249999729, 0.000000000000000000, -62.84375000204836681 ) ) ;
#4098=VECTOR ( 'NONE', #18235, 1000.000000000000000 ) ;
#4099=CARTESIAN_POINT ( 'NONE',  ( 10.81189881249999907, 6.242252689847868297, -38.71875000204835260 ) ) ;
#4101=CARTESIAN_POINT ( 'NONE',  ( -2.293366432827344421E-15, -12.48450537969573659, -13.90625000204836503 ) ) ;
#4105=CARTESIAN_POINT ( 'NONE',  ( 10.00000000000000000, 5.773502691896255534, -105.3749999999999858 ) ) ;
#4107=CARTESIAN_POINT ( 'NONE',  ( -5.321294541346989426, -5.321294541346989426, -220.0000000000000000 ) ) ;
#4110=CARTESIAN_POINT ( 'NONE',  ( 10.81189881249999729, 6.242252689847867408, -106.4062500020483952 ) ) ;
#4111=ORIENTED_EDGE ( 'NONE', *, *, #18175, .F. ) ;
#4113=CARTESIAN_POINT ( 'NONE',  ( -9.999999999998456346, -5.773502691897145489, -12.00000000409673184 ) ) ;
#4115=CARTESIAN_POINT ( 'NONE',  ( -9.999999999999998224, 1.224646799147353059E-15, -195.1250000040967905 ) ) ;
#4118=CARTESIAN_POINT ( 'NONE',  ( -9.999999999999998224, 1.224646799147353059E-15, -34.24999999999997158 ) ) ;
#4120=CARTESIAN_POINT ( 'NONE',  ( -10.81189881249999729, -6.242252689847864744, -36.65625000204835970 ) ) ;
#4121=CARTESIAN_POINT ( 'NONE',  ( -9.999999999999998224, 1.224646799147353059E-15, -91.24999999999998579 ) ) ;
#4123=CARTESIAN_POINT ( 'NONE',  ( 10.81189881249999551, -6.242252689847874514, -139.6562500020484094 ) ) ;
#4125=ORIENTED_EDGE ( 'NONE', *, *, #4837, .T. ) ;
#4127=ORIENTED_EDGE ( 'NONE', *, *, #26163, .T. ) ;
#4128=DIRECTION ( 'NONE',  ( 1.000000000000000000, 0.000000000000000000, 0.000000000000000000 ) ) ;
#4129=FACE_OUTER_BOUND ( 'NONE', #33448, .T. ) ;
#4130=CARTESIAN_POINT ( 'NONE',  ( 10.81189881249999729, 0.000000000000000000, -169.3437500020484094 ) ) ;
#4132=CARTESIAN_POINT ( 'NONE',  ( 10.81189881249999729, 0.000000000000000000, -17.84375000204835260 ) ) ;
#4133=DIRECTION ( 'NONE',  ( 0.4999999999999998335, 0.8660254037844387076, 0.000000000000000000 ) ) ;
#4134=CARTESIAN_POINT ( 'NONE',  ( -10.81189881249999729, 6.242252689847871849, -144.7187500020484094 ) ) ;
#4135=CARTESIAN_POINT ( 'NONE',  ( 10.81189881249999551, -6.242252689847874514, -137.9687500020483810 ) ) ;
#4136=CARTESIAN_POINT ( 'NONE',  ( 5.405949406249999534, 9.363379034771803333, -103.2812500020483952 ) ) ;
#4140=CARTESIAN_POINT ( 'NONE',  ( 10.81189881249999729, 0.000000000000000000, -7.343750002048343717 ) ) ;
#4143=CARTESIAN_POINT ( 'NONE',  ( -2.121150477449813534E-15, -11.54700538379251284, -96.87500000000000000 ) ) ;
#4146=CARTESIAN_POINT ( 'NONE',  ( 10.81189881249999729, 0.000000000000000000, -80.84375000204838102 ) ) ;
#4147=CARTESIAN_POINT ( 'NONE',  ( -10.81189881249999907, -6.242252689847864744, -63.46875000204838102 ) ) ;
#4149=CARTESIAN_POINT ( 'NONE',  ( -2.293366432827344421E-15, -12.48450537969573659, -39.40625000204835260 ) ) ;
#4153=CARTESIAN_POINT ( 'NONE',  ( -9.999999999999998224, 5.773502691896259087, -133.3750000000000000 ) ) ;
#4154=CARTESIAN_POINT ( 'NONE',  ( -2.293366432827344421E-15, -12.48450537969573659, -133.9062500020483810 ) ) ;
#4156=CARTESIAN_POINT ( 'NONE',  ( -10.81189881249999729, 1.324075727343319199E-15, -17.28125000204835970 ) ) ;
#4157=VERTEX_POINT ( 'NONE', #42538 ) ;
#4162=CARTESIAN_POINT ( 'NONE',  ( -10.00000000000000000, -5.773502691896251982, -36.00000000409675494 ) ) ;
#4163=CARTESIAN_POINT ( 'NONE',  ( 9.999999999999998224, 0.000000000000000000, -57.87500000409676204 ) ) ;
#4165=CARTESIAN_POINT ( 'NONE',  ( -4.999999999999996447, 8.660254037844387298, -147.0000000000000000 ) ) ;
#4166=CARTESIAN_POINT ( 'NONE',  ( 5.405949406249992428, -9.363379034771808662, -154.7812500020484094 ) ) ;
#4167=CARTESIAN_POINT ( 'NONE',  ( -5.405949406249996869, 9.363379034771805109, -132.8437500020484094 ) ) ;
#4169=ORIENTED_EDGE ( 'NONE', *, *, #4814, .F. ) ;
#4171=CARTESIAN_POINT ( 'NONE',  ( 5.000000000000000000, 8.660254037844385522, -22.74999999999996447 ) ) ;
#4173=EDGE_CURVE ( 'NONE', #35132, #24959, #17640, .T. ) ;
#4174=ORIENTED_EDGE ( 'NONE', *, *, #41905, .T. ) ;
#4176=CARTESIAN_POINT ( 'NONE',  ( 7.644554776091147741E-16, 12.48450537969573659, -113.4687500020483952 ) ) ;
#4178=LINE ( 'NONE', #14722, #5179 ) ;
#4179=CARTESIAN_POINT ( 'NONE',  ( -5.405949406250003975, -9.363379034771801557, -192.3437500020484094 ) ) ;
#4180=CARTESIAN_POINT ( 'NONE',  ( 10.81189881249999729, 0.000000000000000000, -35.84375000204836681 ) ) ;
#4181=CARTESIAN_POINT ( 'NONE',  ( -9.999999999999998224, 1.224646799147353059E-15, -61.62500000409676204 ) ) ;
#4182=CARTESIAN_POINT ( 'NONE',  ( -9.999999999999998224, 1.224646799147353059E-15, -151.6250000040967905 ) ) ;
#4184=CARTESIAN_POINT ( 'NONE',  ( -10.81189881249999729, -6.242252689847864744, -177.4687500020484094 ) ) ;
#4185=CARTESIAN_POINT ( 'NONE',  ( -5.405949406250003975, -9.363379034771801557, -159.3437500020484094 ) ) ;
#4189=DIRECTION ( 'NONE',  ( 0.08682659386424779191, -0.08682659386424779191, 0.9924325091389669673 ) ) ;
#4191=CARTESIAN_POINT ( 'NONE',  ( -10.81189881249999907, -6.242252689847864744, -91.96875000204838102 ) ) ;
#4193=CARTESIAN_POINT ( 'NONE',  ( 5.405949406249992428, -9.363379034771808662, -64.78125000204838102 ) ) ;
#4194=CARTESIAN_POINT ( 'NONE',  ( -5.000000000000003553, -8.660254037844383745, -97.37500000409677625 ) ) ;
#4196=CARTESIAN_POINT ( 'NONE',  ( 5.405949406249999534, 9.363379034771803333, -121.2812500020483952 ) ) ;
#4197=CARTESIAN_POINT ( 'NONE',  ( -5.405949406249996869, 9.363379034771805109, -151.0312500020483810 ) ) ;
#4199=CARTESIAN_POINT ( 'NONE',  ( 10.00000000000000000, 5.773502691896255534, -129.7500000040967905 ) ) ;
#4201=ADVANCED_FACE ( 'NONE', ( #17479 ), #40565, .T. ) ;
#4206=CARTESIAN_POINT ( 'NONE',  ( -5.405949406250003975, -9.363379034771801557, -191.0312500020484094 ) ) ;
#4208=ORIENTED_EDGE ( 'NONE', *, *, #37566, .T. ) ;
#4209=CARTESIAN_POINT ( 'NONE',  ( -5.000000000000003553, -8.660254037844383745, -47.49999999999998579 ) ) ;
#4211=CARTESIAN_POINT ( 'NONE',  ( -10.00000000000000000, -5.773502691896251982, -66.00000000409679046 ) ) ;
#4212=CARTESIAN_POINT ( 'NONE',  ( -9.999999999999998224, 1.224646799147353059E-15, -21.12500000409675494 ) ) ;
#4215=CARTESIAN_POINT ( 'NONE',  ( -10.81189881249999729, -6.242252689847864744, -60.65625000204840234 ) ) ;
#4217=( BOUNDED_CURVE ( )  B_SPLINE_CURVE ( 2, ( #8696, #14711, #27686, #15139, #34385, #11050, #28337 ),
 .UNSPECIFIED., .F., .F. ) 
 B_SPLINE_CURVE_WITH_KNOTS ( ( 3, 2, 2, 3 ),
 ( 0.6194029850746269883, 0.6206467661691543736, 0.6218905472636816478, 0.6231343283582090331 ),
 .UNSPECIFIED. ) 
 CURVE ( )  GEOMETRIC_REPRESENTATION_ITEM ( )  RATIONAL_B_SPLINE_CURVE ( ( 0.9999999999999880096, 0.8660254037844506980, 1.000000000000000000, 0.8660254037844387076, 1.000000000000000000, 0.8660254037844267172, 1.000000000000011990 ) ) 
 REPRESENTATION_ITEM ( '' )  );
#4220=CARTESIAN_POINT ( 'NONE',  ( -5.000000000000003553, -8.660254037844383745, -35.49999999999997868 ) ) ;
#4221=CARTESIAN_POINT ( 'NONE',  ( -5.405949406249996869, 9.363379034771805109, -173.5312500020484094 ) ) ;
#4224=CARTESIAN_POINT ( 'NONE',  ( 9.999999999999998224, 0.000000000000000000, -72.87500000409677625 ) ) ;
#4225=CARTESIAN_POINT ( 'NONE',  ( -5.000000000000003553, -8.660254037844383745, -81.99999999999998579 ) ) ;
#4227=( BOUNDED_CURVE ( )  B_SPLINE_CURVE ( 2, ( #11797, #8585, #25414, #38559, #34707, #25624, #28227 ),
 .UNSPECIFIED., .F., .F. ) 
 B_SPLINE_CURVE_WITH_KNOTS ( ( 3, 2, 2, 3 ),
 ( 0.6007462686567165422, 0.6019900497512439275, 0.6032338308457712017, 0.6044776119402985870 ),
 .UNSPECIFIED. ) 
 CURVE ( )  GEOMETRIC_REPRESENTATION_ITEM ( )  RATIONAL_B_SPLINE_CURVE ( ( 0.9999999999999880096, 0.8660254037844506980, 1.000000000000000000, 0.8660254037844387076, 1.000000000000000000, 0.8660254037844267172, 1.000000000000011990 ) ) 
 REPRESENTATION_ITEM ( '' )  );
#4228=LINE ( 'NONE', #26889, #26193 ) ;
#4229=CARTESIAN_POINT ( 'NONE',  ( -2.293366432827344421E-15, -12.48450537969573659, -85.90625000204839523 ) ) ;
#4231=EDGE_CURVE ( 'NONE', #22494, #22182, #33698, .T. ) ;
#4232=CARTESIAN_POINT ( 'NONE',  ( 10.00000000000102318, -5.773502691895667560, -69.62499999999995737 ) ) ;
#4233=ORIENTED_EDGE ( 'NONE', *, *, #17475, .F. ) ;
#4234=ORIENTED_EDGE ( 'NONE', *, *, #24415, .T. ) ;
#4235=CARTESIAN_POINT ( 'NONE',  ( -2.293366432827344421E-15, -12.48450537969573659, -22.71875000204837747 ) ) ;
#4236=CARTESIAN_POINT ( 'NONE',  ( 5.405949406249999534, 9.363379034771803333, -10.28125000204835260 ) ) ;
#4237=CARTESIAN_POINT ( 'NONE',  ( 10.81189881249999729, 0.000000000000000000, -71.84375000204836681 ) ) ;
#4238=CARTESIAN_POINT ( 'NONE',  ( 7.070501591499376803E-16, 11.54700538379251284, -164.0000000040967905 ) ) ;
#4240=CARTESIAN_POINT ( 'NONE',  ( 10.81189881249999551, -6.242252689847874514, -185.9687500020484094 ) ) ;
#4243=DIRECTION ( 'NONE',  ( -0.000000000000000000, -0.000000000000000000, 1.000000000000000000 ) ) ;
#4245=CARTESIAN_POINT ( 'NONE',  ( 5.000000000000000000, 8.660254037844385522, -141.2500000000000000 ) ) ;
#4246=CARTESIAN_POINT ( 'NONE',  ( 7.070501591499377789E-16, 11.54700538379251284, 0.9999999959032610519 ) ) ;
#4247=CARTESIAN_POINT ( 'NONE',  ( 5.000000000000000000, 8.660254037844385522, -60.62500000409676204 ) ) ;
#4249=CARTESIAN_POINT ( 'NONE',  ( -10.81189881249999729, 6.242252689847871849, -116.2187500020483810 ) ) ;
#4251=CARTESIAN_POINT ( 'NONE',  ( 10.81189881249999907, 6.242252689847868297, -92.90625000204839523 ) ) ;
#4252=CARTESIAN_POINT ( 'NONE',  ( -2.293366432827344421E-15, -12.48450537969573659, -96.21875000204838102 ) ) ;
#4255=CARTESIAN_POINT ( 'NONE',  ( -2.121150477449813534E-15, -11.54700538379251284, -152.7500000040967620 ) ) ;
#4264=CARTESIAN_POINT ( 'NONE',  ( -9.999999999999998224, 5.773502691896259087, -76.37499999999998579 ) ) ;
#4266=CARTESIAN_POINT ( 'NONE',  ( -2.121150477449813534E-15, -11.54700538379251284, -88.25000000409677625 ) ) ;
#4267=CARTESIAN_POINT ( 'NONE',  ( 9.999999999999998224, 0.000000000000000000, -171.5000000000000000 ) ) ;
#4269=CARTESIAN_POINT ( 'NONE',  ( -10.81189881249999729, -6.242252689847864744, -83.15625000204836681 ) ) ;
#4271=CARTESIAN_POINT ( 'NONE',  ( 9.999999999999998224, 0.000000000000000000, -168.5000000000000000 ) ) ;
#4273=VERTEX_POINT ( 'NONE', #14229 ) ;
#4274=CARTESIAN_POINT ( 'NONE',  ( -10.81189881249999729, 1.324075727343319199E-15, -197.2812500020484094 ) ) ;
#4276=CARTESIAN_POINT ( 'NONE',  ( 5.405949406249992428, -9.363379034771808662, -15.09375000204835082 ) ) ;
#4277=DIRECTION ( 'NONE',  ( -0.000000000000000000, -0.000000000000000000, 1.000000000000000000 ) ) ;
#4279=CARTESIAN_POINT ( 'NONE',  ( -5.405949406250003975, -9.363379034771801557, -138.5312500020484094 ) ) ;
#4280=CARTESIAN_POINT ( 'NONE',  ( 5.000000000000000000, 8.660254037844385522, -186.2500000000000000 ) ) ;
#4283=CARTESIAN_POINT ( 'NONE',  ( 5.405949406249992428, -9.363379034771808662, -109.7812500020483810 ) ) ;
#4286=EDGE_CURVE ( 'NONE', #31643, #5198, #23206, .T. ) ;
#4287=VERTEX_POINT ( 'NONE', #3917 ) ;
#4288=EDGE_CURVE ( 'NONE', #37390, #33430, #36691, .T. ) ;
#4289=EDGE_LOOP ( 'NONE', ( #3235, #27590, #39153, #22336 ) ) ;
#4290=CARTESIAN_POINT ( 'NONE',  ( -10.81189881249999729, 1.324075727343319199E-15, -41.28125000204838102 ) ) ;
#4292=CARTESIAN_POINT ( 'NONE',  ( 10.81189881249999729, 0.000000000000000000, -92.84375000204838102 ) ) ;
#4293=FACE_OUTER_BOUND ( 'NONE', #32853, .T. ) ;
#4294=( BOUNDED_CURVE ( )  B_SPLINE_CURVE ( 2, ( #40816, #20761, #4793, #11256, #11468, #17298, #21189 ),
 .UNSPECIFIED., .F., .F. ) 
 B_SPLINE_CURVE_WITH_KNOTS ( ( 3, 2, 2, 3 ),
 ( 0.6529850746268659467, 0.6542288557213932210, 0.6554726368159206062, 0.6567164179104479915 ),
 .UNSPECIFIED. ) 
 CURVE ( )  GEOMETRIC_REPRESENTATION_ITEM ( )  RATIONAL_B_SPLINE_CURVE ( ( 0.9999999999999761302, 0.8660254037844625774, 1.000000000000000000, 0.8660254037844387076, 1.000000000000000000, 0.8660254037844148378, 1.000000000000023981 ) ) 
 REPRESENTATION_ITEM ( '' )  );
#4295=CARTESIAN_POINT ( 'NONE',  ( -9.999999999999998224, 1.224646799147353059E-15, -173.7500000000000284 ) ) ;
#4296=CARTESIAN_POINT ( 'NONE',  ( 10.81189881249999551, -6.242252689847874514, -193.4687500020484094 ) ) ;
#4299=CARTESIAN_POINT ( 'NONE',  ( -2.293366432827344421E-15, -12.48450537969573659, -123.2187500020483952 ) ) ;
#4303=CARTESIAN_POINT ( 'NONE',  ( 7.070501591499377789E-16, 11.54700538379251284, -185.0000000040967905 ) ) ;
#4305=CARTESIAN_POINT ( 'NONE',  ( -2.293366432827344421E-15, -12.48450537969573659, -175.9062500020484379 ) ) ;
#4306=CARTESIAN_POINT ( 'NONE',  ( 9.999999999999998224, 0.000000000000000000, -180.5000000000000000 ) ) ;
#4307=CARTESIAN_POINT ( 'NONE',  ( 7.070501591499376803E-16, 11.54700538379251284, -122.0000000040967905 ) ) ;
#4309=CARTESIAN_POINT ( 'NONE',  ( -5.405949406250003975, -9.363379034771801557, -51.34375000204835260 ) ) ;
#4310=CARTESIAN_POINT ( 'NONE',  ( 10.81189881249999729, 0.000000000000000000, -43.34375000204837391 ) ) ;
#4312=CARTESIAN_POINT ( 'NONE',  ( 5.405949406249992428, -9.363379034771808662, -9.281250002048352599 ) ) ;
#4314=CARTESIAN_POINT ( 'NONE',  ( -9.999999999999479527, -5.773502691896549521, -93.00000000409676204 ) ) ;
#4316=CARTESIAN_POINT ( 'NONE',  ( 9.999999999999996447, -5.773502691896262640, -93.62499999999998579 ) ) ;
#4318=CARTESIAN_POINT ( 'NONE',  ( -5.000000000000003553, -8.660254037844383745, -112.3750000040967763 ) ) ;
#4319=EDGE_CURVE ( 'NONE', #40567, #29474, #21818, .T. ) ;
#4323=CARTESIAN_POINT ( 'NONE',  ( -2.293366432827344421E-15, -12.48450537969573659, -108.4062500020483810 ) ) ;
#4324=EDGE_LOOP ( 'NONE', ( #25882, #24799, #9220, #28023 ) ) ;
#4325=CARTESIAN_POINT ( 'NONE',  ( 9.999999999999998224, 0.000000000000000000, -8.375000004096744277 ) ) ;
#4327=CARTESIAN_POINT ( 'NONE',  ( -9.999999999999998224, 1.224646799147353059E-15, -166.6250000040967905 ) ) ;
#4330=CARTESIAN_POINT ( 'NONE',  ( 5.000000000000000000, 8.660254037844385522, -27.24999999999996803 ) ) ;
#4331=CARTESIAN_POINT ( 'NONE',  ( 7.644554776091147741E-16, 12.48450537969573659, -32.65625000204835970 ) ) ;
#4332=CARTESIAN_POINT ( 'NONE',  ( -9.999999999999998224, 5.773502691896259087, -160.3749999999999716 ) ) ;
#4334=CARTESIAN_POINT ( 'NONE',  ( 10.81189881249999729, 0.000000000000000000, -133.5312500020484094 ) ) ;
#4337=ORIENTED_EDGE ( 'NONE', *, *, #2216, .F. ) ;
#4338=( BOUNDED_CURVE ( )  B_SPLINE_CURVE ( 2, ( #38895, #32012, #28559, #9323, #35667, #41691, #41260 ),
 .UNSPECIFIED., .F., .F. ) 
 B_SPLINE_CURVE_WITH_KNOTS ( ( 3, 2, 2, 3 ),
 ( 0.6940298507462688837, 0.6952736318407962690, 0.6965174129353237653, 0.6977611940298510396 ),
 .UNSPECIFIED. ) 
 CURVE ( )  GEOMETRIC_REPRESENTATION_ITEM ( )  RATIONAL_B_SPLINE_CURVE ( ( 0.9999999999999761302, 0.8660254037844625774, 1.000000000000000000, 0.8660254037844387076, 1.000000000000000000, 0.8660254037844028474, 1.000000000000035971 ) ) 
 REPRESENTATION_ITEM ( '' )  );
#4339=EDGE_CURVE ( 'NONE', #32487, #3490, #1538, .T. ) ;
#4341=VERTEX_POINT ( 'NONE', #15094 ) ;
#4343=CARTESIAN_POINT ( 'NONE',  ( -9.999999999999742428, -5.773502691896402084, -121.1250000000000000 ) ) ;
#4345=CARTESIAN_POINT ( 'NONE',  ( 4.999999999999992006, -8.660254037844389075, -134.2499999999999716 ) ) ;
#4346=CARTESIAN_POINT ( 'NONE',  ( -2.293366432827344421E-15, -12.48450537969573659, -163.7187500020483810 ) ) ;
#4348=CARTESIAN_POINT ( 'NONE',  ( -2.293366432827344421E-15, -12.48450537969573659, -18.21875000204837036 ) ) ;
#4349=DIRECTION ( 'NONE',  ( 1.000000000000000000, 0.000000000000000000, 0.000000000000000000 ) ) ;
#4350=CARTESIAN_POINT ( 'NONE',  ( -10.81189881249999729, 1.324075727343319199E-15, -149.0937500020483810 ) ) ;
#4351=CARTESIAN_POINT ( 'NONE',  ( -10.81189881249999729, 6.242252689847871849, -135.7187500020483810 ) ) ;
#4352=CARTESIAN_POINT ( 'NONE',  ( 5.405949406249999534, 9.363379034771803333, -109.2812500020483810 ) ) ;
#4356=CARTESIAN_POINT ( 'NONE',  ( -5.405949406249996869, 9.363379034771805109, -12.84375000204834905 ) ) ;
#4360=CARTESIAN_POINT ( 'NONE',  ( 9.999999999999998224, 0.000000000000000000, -96.49999999999998579 ) ) ;
#4363=CARTESIAN_POINT ( 'NONE',  ( -10.81189881249999729, 6.242252689847871849, -77.21875000204838102 ) ) ;
#4364=CARTESIAN_POINT ( 'NONE',  ( 10.81189881249999729, 0.000000000000000000, -68.84375000204836681 ) ) ;
#4365=CARTESIAN_POINT ( 'NONE',  ( -9.999999999999998224, 1.224646799147353059E-15, -167.7500000000000000 ) ) ;
#4366=CARTESIAN_POINT ( 'NONE',  ( -10.81189881249999729, 1.324075727343319199E-15, -35.28125000204837391 ) ) ;
#4370=CARTESIAN_POINT ( 'NONE',  ( -9.999999999999998224, 5.773502691896259087, -118.3750000000000000 ) ) ;
#4371=CARTESIAN_POINT ( 'NONE',  ( -10.81189881249999729, 1.324075727343319199E-15, -134.2812500020483810 ) ) ;
#4372=DIRECTION ( 'NONE',  ( 0.000000000000000000, -0.000000000000000000, 1.000000000000000000 ) ) ;
#4374=CARTESIAN_POINT ( 'NONE',  ( -10.81189881249999729, -6.242252689847864744, -15.65625000204837569 ) ) ;
#4376=LINE ( 'NONE', #5024, #2453 ) ;
#4378=CARTESIAN_POINT ( 'NONE',  ( 5.000000000000000000, 8.660254037844385522, -9.249999999999952038 ) ) ;
#4379=CARTESIAN_POINT ( 'NONE',  ( 7.070501591499377789E-16, 11.54700538379251284, -35.00000000409674783 ) ) ;
#4383=CARTESIAN_POINT ( 'NONE',  ( 10.81189881249999551, -6.242252689847874514, -150.1562500020484094 ) ) ;
#4384=CARTESIAN_POINT ( 'NONE',  ( 5.405949406249992428, -9.363379034771808662, -132.0937500020483810 ) ) ;
#4386=ORIENTED_EDGE ( 'NONE', *, *, #20247, .F. ) ;
#4387=VERTEX_POINT ( 'NONE', #31752 ) ;
#4388=VERTEX_POINT ( 'NONE', #41429 ) ;
#4389=CARTESIAN_POINT ( 'NONE',  ( -10.81189881249999907, -6.242252689847864744, -109.9687500020483668 ) ) ;
#4390=EDGE_LOOP ( 'NONE', ( #40997, #15151, #31808, #25816 ) ) ;
#4392=CARTESIAN_POINT ( 'NONE',  ( 10.81189881249999551, -6.242252689847874514, -187.4687500020484094 ) ) ;
#4393=CARTESIAN_POINT ( 'NONE',  ( -10.81189881249999907, -6.242252689847864744, -42.46875000204835260 ) ) ;
#4396=CARTESIAN_POINT ( 'NONE',  ( -5.000000000000003553, -8.660254037844383745, -10.37500000409674605 ) ) ;
#4397=CARTESIAN_POINT ( 'NONE',  ( -2.293366432827344421E-15, -12.48450537969573659, -169.7187500020483810 ) ) ;
#4398=CARTESIAN_POINT ( 'NONE',  ( -5.405949406250003975, -9.363379034771801557, -157.8437500020483810 ) ) ;
#4399=CARTESIAN_POINT ( 'NONE',  ( -2.121150477449813534E-15, -11.54700538379251284, -25.25000000409676559 ) ) ;
#4402=CARTESIAN_POINT ( 'NONE',  ( -2.121150477449813534E-15, -11.54700538379251284, -42.87499999999997868 ) ) ;
#4405=CARTESIAN_POINT ( 'NONE',  ( 5.405949406249992428, -9.363379034771808662, -85.59375000204836681 ) ) ;
#4407=CARTESIAN_POINT ( 'NONE',  ( 10.81189881249999907, 6.242252689847868297, -55.40625000204837391 ) ) ;
#4408=CARTESIAN_POINT ( 'NONE',  ( -4.999999999999996447, 8.660254037844387298, -87.37500000409677625 ) ) ;
#4410=CARTESIAN_POINT ( 'NONE',  ( 10.81189881249999729, 0.000000000000000000, -120.0312500020483952 ) ) ;
#4411=CARTESIAN_POINT ( 'NONE',  ( -2.293366432827344421E-15, -12.48450537969573659, -156.4062500020484379 ) ) ;
#4414=CARTESIAN_POINT ( 'NONE',  ( 10.00000000000000000, 5.773502691896255534, -131.2500000040967905 ) ) ;
#4416=ORIENTED_EDGE ( 'NONE', *, *, #19816, .F. ) ;
#4420=CARTESIAN_POINT ( 'NONE',  ( 5.405949406249992428, -9.363379034771808662, -189.2812500020484094 ) ) ;
#4421=ORIENTED_EDGE ( 'NONE', *, *, #40051, .T. ) ;
#4422=CARTESIAN_POINT ( 'NONE',  ( 7.070501591499377789E-16, 11.54700538379251284, -52.62499999999997868 ) ) ;
#4424=CARTESIAN_POINT ( 'NONE',  ( -4.999999999999996447, 8.660254037844387298, -55.87500000409676204 ) ) ;
#4425=CARTESIAN_POINT ( 'NONE',  ( 9.999999999999998224, 0.000000000000000000, -108.8750000040967763 ) ) ;
#4427=CARTESIAN_POINT ( 'NONE',  ( -11.54700538379250574, -20.00000000000000355, 45.00000000000009237 ) ) ;
#4429=CARTESIAN_POINT ( 'NONE',  ( 5.405949406249999534, 9.363379034771803333, -53.78125000204836681 ) ) ;
#4432=DIRECTION ( 'NONE',  ( -0.000000000000000000, -0.000000000000000000, 1.000000000000000000 ) ) ;
#4433=CARTESIAN_POINT ( 'NONE',  ( 10.81189881249999729, 0.000000000000000000, -175.5312500020483810 ) ) ;
#4435=CARTESIAN_POINT ( 'NONE',  ( -9.999999999999998224, 1.224646799147353059E-15, -200.0000000000000000 ) ) ;
#4437=CARTESIAN_POINT ( 'NONE',  ( -2.121150477449813534E-15, -11.54700538379251284, -89.37499999999997158 ) ) ;
#4438=CARTESIAN_POINT ( 'NONE',  ( -10.00000000000051337, 5.773502691895962435, -105.2500000040967620 ) ) ;
#4439=CARTESIAN_POINT ( 'NONE',  ( 7.070501591499376803E-16, 11.54700538379251284, -39.50000000409675494 ) ) ;
#4440=CARTESIAN_POINT ( 'NONE',  ( -5.405949406250003975, -9.363379034771801557, -83.03125000204838102 ) ) ;
#4443=ORIENTED_EDGE ( 'NONE', *, *, #8828, .T. ) ;
#4445=EDGE_CURVE ( 'NONE', #6420, #18833, #38084, .T. ) ;
#4446=CARTESIAN_POINT ( 'NONE',  ( 10.81189881249999551, -6.242252689847874514, -35.96875000204835260 ) ) ;
#4447=CARTESIAN_POINT ( 'NONE',  ( 10.81189881249999551, -6.242252689847874514, -25.46875000204837391 ) ) ;
#4448=CARTESIAN_POINT ( 'NONE',  ( -2.293366432827344421E-15, -12.48450537969573659, -15.40625000204837391 ) ) ;
#4449=CARTESIAN_POINT ( 'NONE',  ( -10.81189881249999729, 6.242252689847871849, -66.71875000204838102 ) ) ;
#4451=CARTESIAN_POINT ( 'NONE',  ( 5.405949406249992428, -9.363379034771808662, -181.5937500020483810 ) ) ;
#4453=LINE ( 'NONE', #15001, #32376 ) ;
#4454=DIRECTION ( 'NONE',  ( -0.000000000000000000, -0.000000000000000000, 1.000000000000000000 ) ) ;
#4455=CARTESIAN_POINT ( 'NONE',  ( -9.999999999999998224, 1.224646799147353059E-15, -65.74999999999997158 ) ) ;
#4457=CARTESIAN_POINT ( 'NONE',  ( 0.000000000000000000, 0.000000000000000000, -200.0000000000000000 ) ) ;
#4458=CARTESIAN_POINT ( 'NONE',  ( -10.81189881249999729, 6.242252689847871849, -110.2187500020483810 ) ) ;
#4459=LINE ( 'NONE', #20218, #28719 ) ;
#4460=CARTESIAN_POINT ( 'NONE',  ( 5.405949406249992428, -9.363379034771808662, -93.28125000204838102 ) ) ;
#4461=CARTESIAN_POINT ( 'NONE',  ( -10.81189881249999729, 1.324075727343319199E-15, -102.5937500020483810 ) ) ;
#4465=CARTESIAN_POINT ( 'NONE',  ( 9.999999999999996447, -5.773502691896262640, -152.5000000040967905 ) ) ;
#4467=( BOUNDED_CURVE ( )  B_SPLINE_CURVE ( 2, ( #20196, #3174, #9845, #29926, #367, #19766, #15878 ),
 .UNSPECIFIED., .F., .F. ) 
 B_SPLINE_CURVE_WITH_KNOTS ( ( 3, 2, 2, 3 ),
 ( 0.7649253731343285123, 0.7661691542288557866, 0.7674129353233831718, 0.7686567164179105571 ),
 .UNSPECIFIED. ) 
 CURVE ( )  GEOMETRIC_REPRESENTATION_ITEM ( )  RATIONAL_B_SPLINE_CURVE ( ( 0.9999999999999880096, 0.8660254037844506980, 1.000000000000000000, 0.8660254037844387076, 1.000000000000000000, 0.8660254037844267172, 1.000000000000011990 ) ) 
 REPRESENTATION_ITEM ( '' )  );
#4470=CARTESIAN_POINT ( 'NONE',  ( -4.999999999999996447, 8.660254037844387298, -153.3750000040967905 ) ) ;
#4474=CARTESIAN_POINT ( 'NONE',  ( -4.999999999999996447, 8.660254037844387298, -73.49999999999998579 ) ) ;
#4476=CARTESIAN_POINT ( 'NONE',  ( -5.000000000000003553, -8.660254037844383745, -80.87500000409677625 ) ) ;
#4477=CARTESIAN_POINT ( 'NONE',  ( 10.00000000000051159, -5.773502691895965988, -95.50000000409676204 ) ) ;
#4479=CARTESIAN_POINT ( 'NONE',  ( -10.81189881249999729, 1.324075727343319199E-15, -80.28125000204838102 ) ) ;
#4480=( BOUNDED_CURVE ( )  B_SPLINE_CURVE ( 2, ( #4327, #40343, #14658, #11423, #37766, #17465, #1742 ),
 .UNSPECIFIED., .F., .F. ) 
 B_SPLINE_CURVE_WITH_KNOTS ( ( 3, 2, 2, 3 ),
 ( 0.1604477611940298698, 0.1616915422885572551, 0.1629353233830845848, 0.1641791044776119424 ),
 .UNSPECIFIED. ) 
 CURVE ( )  GEOMETRIC_REPRESENTATION_ITEM ( )  RATIONAL_B_SPLINE_CURVE ( ( 0.9999999999999970024, 0.8660254037844417052, 1.000000000000000000, 0.8660254037844387076, 1.000000000000000000, 0.8660254037844387076, 1.000000000000000000 ) ) 
 REPRESENTATION_ITEM ( '' )  );
#4482=CARTESIAN_POINT ( 'NONE',  ( -9.999999999999998224, 1.224646799147353059E-15, -167.7500000000000000 ) ) ;
#4485=CARTESIAN_POINT ( 'NONE',  ( -5.000000000000003553, -8.660254037844383745, -2.499999999999974243 ) ) ;
#4487=CARTESIAN_POINT ( 'NONE',  ( 5.405949406249999534, 9.363379034771803333, -11.59375000204834727 ) ) ;
#4488=CARTESIAN_POINT ( 'NONE',  ( -5.000000000000003553, -8.660254037844383745, -176.8750000040967905 ) ) ;
#4490=CARTESIAN_POINT ( 'NONE',  ( 10.81189881249999907, 6.242252689847868297, -128.9062500020483810 ) ) ;
#4491=CARTESIAN_POINT ( 'NONE',  ( -4.999999999999996447, 8.660254037844387298, -181.5000000000000000 ) ) ;
#4492=CARTESIAN_POINT ( 'NONE',  ( 0.000000000000000000, 0.000000000000000000, -200.0000000000000000 ) ) ;
#4493=CARTESIAN_POINT ( 'NONE',  ( 10.81189881249999551, -6.242252689847874514, -108.1562500020483810 ) ) ;
#4494=ORIENTED_EDGE ( 'NONE', *, *, #38620, .F. ) ;
#4495=CARTESIAN_POINT ( 'NONE',  ( -4.999999999999996447, 8.660254037844387298, -138.3750000040967905 ) ) ;
#4496=ORIENTED_EDGE ( 'NONE', *, *, #2895, .F. ) ;
#4497=ORIENTED_EDGE ( 'NONE', *, *, #37845, .F. ) ;
#4498=CARTESIAN_POINT ( 'NONE',  ( 5.405949406249992428, -9.363379034771808662, -37.78125000204838102 ) ) ;
#4500=CARTESIAN_POINT ( 'NONE',  ( 10.81189881249999551, -6.242252689847874514, -89.96875000204838102 ) ) ;
#4501=CARTESIAN_POINT ( 'NONE',  ( 9.999999999999998224, 0.000000000000000000, -167.0000000000000000 ) ) ;
#4502=CARTESIAN_POINT ( 'NONE',  ( 0.000000000000000000, 0.000000000000000000, -200.0000000000000000 ) ) ;
#4503=AXIS2_PLACEMENT_3D ( 'NONE', #31678, #8996, #7561 ) ;
#4506=CARTESIAN_POINT ( 'NONE',  ( -10.81189881249999729, 1.324075727343319199E-15, -122.0937500020483952 ) ) ;
#4508=CARTESIAN_POINT ( 'NONE',  ( 10.81189881249999551, -6.242252689847874514, -0.1562500020483646446 ) ) ;
#4511=CARTESIAN_POINT ( 'NONE',  ( -9.999999999999998224, 5.773502691896259087, -178.7500000040967905 ) ) ;
#4513=CARTESIAN_POINT ( 'NONE',  ( -5.405949406250003975, -9.363379034771801557, -177.5312500020483810 ) ) ;
#4516=CARTESIAN_POINT ( 'NONE',  ( -5.405949406249996869, 9.363379034771805109, -48.84375000204838102 ) ) ;
#4517=CARTESIAN_POINT ( 'NONE',  ( -10.81189881249999907, -6.242252689847864744, -43.96875000204835970 ) ) ;
#4519=CARTESIAN_POINT ( 'NONE',  ( -10.81189881249999907, -6.242252689847864744, -12.65625000204835970 ) ) ;
#4521=CARTESIAN_POINT ( 'NONE',  ( -5.000000000000003553, -8.660254037844383745, -164.8750000040967905 ) ) ;
#4523=EDGE_CURVE ( 'NONE', #10167, #38258, #24610, .T. ) ;
#4524=CARTESIAN_POINT ( 'NONE',  ( 4.999999999999992006, -8.660254037844389075, -96.74999999999998579 ) ) ;
#4526=CARTESIAN_POINT ( 'NONE',  ( 9.999999999999998224, 0.000000000000000000, -102.8750000040967763 ) ) ;
#4527=CARTESIAN_POINT ( 'NONE',  ( -5.000000000000003553, -8.660254037844383745, -169.0000000000000000 ) ) ;
#4530=CARTESIAN_POINT ( 'NONE',  ( 10.81189881249999551, -6.242252689847874514, -111.1562500020483952 ) ) ;
#4531=ORIENTED_EDGE ( 'NONE', *, *, #30417, .F. ) ;
#4535=CARTESIAN_POINT ( 'NONE',  ( -5.405949406250003975, -9.363379034771801557, -168.5312500020484094 ) ) ;
#4538=CARTESIAN_POINT ( 'NONE',  ( 9.999999999999996447, -5.773502691896262640, -24.62499999999998934 ) ) ;
#4539=CARTESIAN_POINT ( 'NONE',  ( -5.405949406249996869, 9.363379034771805109, -37.03125000204837391 ) ) ;
#4540=CARTESIAN_POINT ( 'NONE',  ( 4.999999999999992006, -8.660254037844389075, -162.7500000000000000 ) ) ;
#4541=LINE ( 'NONE', #1098, #26277 ) ;
#4543=VECTOR ( 'NONE', #28297, 1000.000000000000000 ) ;
#4544=AXIS2_PLACEMENT_3D ( 'NONE', #28875, #16090, #9215 ) ;
#4545=CARTESIAN_POINT ( 'NONE',  ( -9.999999999999998224, 1.224646799147353059E-15, -34.24999999999997158 ) ) ;
#4546=CARTESIAN_POINT ( 'NONE',  ( -10.81189881249999729, 1.324075727343319199E-15, -137.2812500020483810 ) ) ;
#4547=CARTESIAN_POINT ( 'NONE',  ( -1.880502898556992042, 9.996614838207573683, 4.524943085473207639E-15 ) ) ;
#4549=( BOUNDED_CURVE ( )  B_SPLINE_CURVE ( 2, ( #18402, #41487, #11923, #21860, #18616, #12135, #31813 ),
 .UNSPECIFIED., .F., .F. ) 
 B_SPLINE_CURVE_WITH_KNOTS ( ( 3, 2, 2, 3 ),
 ( 0.9514925373134331954, 0.9527363184079605807, 0.9539800995024879660, 0.9552238805970153512 ),
 .UNSPECIFIED. ) 
 CURVE ( )  GEOMETRIC_REPRESENTATION_ITEM ( )  RATIONAL_B_SPLINE_CURVE ( ( 0.9999999999999641398, 0.8660254037844745678, 1.000000000000000000, 0.8660254037844387076, 1.000000000000000000, 0.8660254037843908570, 1.000000000000047740 ) ) 
 REPRESENTATION_ITEM ( '' )  );
#4550=CARTESIAN_POINT ( 'NONE',  ( 5.000000000000000000, 8.660254037844385522, -167.1250000040967905 ) ) ;
#4551=ORIENTED_EDGE ( 'NONE', *, *, #36139, .T. ) ;
#4552=ORIENTED_EDGE ( 'NONE', *, *, #6442, .F. ) ;
#4554=CARTESIAN_POINT ( 'NONE',  ( 7.070501591499376803E-16, 11.54700538379251284, -182.0000000040967905 ) ) ;
#4555=CARTESIAN_POINT ( 'NONE',  ( -2.121150477449813534E-15, -11.54700538379251284, -146.7500000040967905 ) ) ;
#4556=CARTESIAN_POINT ( 'NONE',  ( -10.81189881249999729, 1.324075727343319199E-15, -168.5937500020484094 ) ) ;
#4558=CARTESIAN_POINT ( 'NONE',  ( 10.81189881249999729, 0.000000000000000000, -14.84375000204835082 ) ) ;
#4559=FACE_OUTER_BOUND ( 'NONE', #30726, .T. ) ;
#4560=CARTESIAN_POINT ( 'NONE',  ( 5.405949406249992428, -9.363379034771808662, -148.5937500020483810 ) ) ;
#4561=CARTESIAN_POINT ( 'NONE',  ( -5.405949406249996869, 9.363379034771805109, -140.3437500020484094 ) ) ;
#4562=CARTESIAN_POINT ( 'NONE',  ( -5.405949406249996869, 9.363379034771805109, -107.5312500020483810 ) ) ;
#4566=CARTESIAN_POINT ( 'NONE',  ( -5.405949406250003975, -9.363379034771801557, -3.343750002048367698 ) ) ;
#4568=CARTESIAN_POINT ( 'NONE',  ( -9.999999999999998224, 1.224646799147353059E-15, -152.7500000000000000 ) ) ;
#4569=CARTESIAN_POINT ( 'NONE',  ( -4.999999999999996447, 8.660254037844387298, -4.875000004096769146 ) ) ;
#4572=CARTESIAN_POINT ( 'NONE',  ( 5.405949406249999534, 9.363379034771803333, -76.09375000204838102 ) ) ;
#4573=CARTESIAN_POINT ( 'NONE',  ( -10.81189881249999907, -6.242252689847864744, -64.96875000204838102 ) ) ;
#4575=CARTESIAN_POINT ( 'NONE',  ( -5.405949406249996869, 9.363379034771805109, -35.53125000204837391 ) ) ;
#4577=CARTESIAN_POINT ( 'NONE',  ( 0.000000000000000000, 0.000000000000000000, -200.0000000000000000 ) ) ;
#4580=EDGE_CURVE ( 'NONE', #19402, #25691, #27872, .T. ) ;
#4581=CARTESIAN_POINT ( 'NONE',  ( -9.999999999999998224, 1.224646799147353059E-15, -124.2500000000000000 ) ) ;
#4582=CARTESIAN_POINT ( 'NONE',  ( 10.81189881249999729, 6.242252689847867408, -131.9062500020483810 ) ) ;
#4585=CARTESIAN_POINT ( 'NONE',  ( -10.81189881249999729, 1.324075727343319199E-15, -14.28125000204835615 ) ) ;
#4587=ORIENTED_EDGE ( 'NONE', *, *, #42588, .F. ) ;
#4590=CARTESIAN_POINT ( 'NONE',  ( 7.070501591499377789E-16, 11.54700538379251284, -38.00000000409676204 ) ) ;
#4591=CARTESIAN_POINT ( 'NONE',  ( -10.00000000000051337, 5.773502691895962435, -148.3749999999999716 ) ) ;
#4594=( BOUNDED_CURVE ( )  B_SPLINE_CURVE ( 2, ( #8254, #37808, #18157, #15124, #34801, #35014, #12107 ),
 .UNSPECIFIED., .F., .F. ) 
 B_SPLINE_CURVE_WITH_KNOTS ( ( 3, 2, 2, 3 ),
 ( 0.3134328358208955390, 0.3146766169154229242, 0.3159203980099503650, 0.3171641791044778058 ),
 .UNSPECIFIED. ) 
 CURVE ( )  GEOMETRIC_REPRESENTATION_ITEM ( )  RATIONAL_B_SPLINE_CURVE ( ( 1.000000000000000000, 0.8660254037844387076, 1.000000000000000000, 0.8660254037844387076, 1.000000000000000000, 0.8660254037844207220, 1.000000000000017986 ) ) 
 REPRESENTATION_ITEM ( '' )  );
#4595=CARTESIAN_POINT ( 'NONE',  ( -9.999999999999998224, 1.224646799147353059E-15, -191.7500000000000000 ) ) ;
#4596=CARTESIAN_POINT ( 'NONE',  ( -2.293366432827344421E-15, -12.48450537969573659, -156.4062500020483810 ) ) ;
#4597=CARTESIAN_POINT ( 'NONE',  ( 5.405949406249992428, -9.363379034771808662, -126.0937500020483668 ) ) ;
#4598=CARTESIAN_POINT ( 'NONE',  ( 5.000000000000000000, 8.660254037844385522, -190.7500000000000000 ) ) ;
#4600=CARTESIAN_POINT ( 'NONE',  ( 7.070501591499376803E-16, 11.54700538379251284, -22.62499999999997868 ) ) ;
#4601=ORIENTED_EDGE ( 'NONE', *, *, #32446, .F. ) ;
#4605=CARTESIAN_POINT ( 'NONE',  ( -5.405949406250003975, -9.363379034771801557, -109.8437500020483810 ) ) ;
#4606=VERTEX_POINT ( 'NONE', #34270 ) ;
#4608=CARTESIAN_POINT ( 'NONE',  ( 10.81189881249999551, -6.242252689847874514, -185.9687500020484094 ) ) ;
#4609=CARTESIAN_POINT ( 'NONE',  ( -5.405949406249996869, 9.363379034771805109, -41.34375000204837391 ) ) ;
#4610=CARTESIAN_POINT ( 'NONE',  ( 0.3998884125188737482, -10.45061954883015254, 8.157905031340238759E-16 ) ) ;
#4611=CARTESIAN_POINT ( 'NONE',  ( -9.999999999999998224, 1.224646799147353059E-15, -174.1250000040968189 ) ) ;
#4612=CARTESIAN_POINT ( 'NONE',  ( 10.81189881249999729, 6.242252689847867408, -175.2187500020484094 ) ) ;
#4613=CARTESIAN_POINT ( 'NONE',  ( -10.81189881249999907, -6.242252689847864744, -163.9687500020484094 ) ) ;
#4617=CARTESIAN_POINT ( 'NONE',  ( 9.999999999999998224, 0.000000000000000000, -74.37500000409677625 ) ) ;
#4619=CARTESIAN_POINT ( 'NONE',  ( -5.405949406249996869, 9.363379034771805109, -87.84375000204836681 ) ) ;
#4620=CARTESIAN_POINT ( 'NONE',  ( 10.00000000000025402, -5.773502691896113426, -135.6250000000000000 ) ) ;
#4621=CARTESIAN_POINT ( 'NONE',  ( 5.405949406249999534, 9.363379034771803333, -61.28125000204837391 ) ) ;
#4624=CARTESIAN_POINT ( 'NONE',  ( 5.405949406249999534, 9.363379034771803333, -112.2812500020483952 ) ) ;
#4625=CARTESIAN_POINT ( 'NONE',  ( -10.81189881249999729, 1.324075727343319199E-15, -150.7812500020483810 ) ) ;
#4628=CARTESIAN_POINT ( 'NONE',  ( 7.070501591499377789E-16, 11.54700538379251284, -126.5000000040967905 ) ) ;
#4634=CARTESIAN_POINT ( 'NONE',  ( 5.405949406249999534, 9.363379034771803333, -184.2812500020484094 ) ) ;
#4636=CARTESIAN_POINT ( 'NONE',  ( -4.999999999999996447, 8.660254037844387298, -52.49999999999996447 ) ) ;
#4638=CARTESIAN_POINT ( 'NONE',  ( -10.00000000000000000, -5.773502691896251982, -55.50000000409678336 ) ) ;
#4639=CARTESIAN_POINT ( 'NONE',  ( -9.999999999999998224, 1.224646799147353059E-15, -49.62500000409675494 ) ) ;
#4640=CARTESIAN_POINT ( 'NONE',  ( 9.999999999999998224, 0.000000000000000000, -171.8750000040968189 ) ) ;
#4642=CARTESIAN_POINT ( 'NONE',  ( -10.81189881249999729, 1.324075727343319199E-15, -53.28125000204836681 ) ) ;
#4645=CARTESIAN_POINT ( 'NONE',  ( 7.070501591499376803E-16, 11.54700538379251284, -158.0000000040968189 ) ) ;
#4646=CARTESIAN_POINT ( 'NONE',  ( -10.81189881249999729, 1.324075727343319199E-15, -180.7812500020484094 ) ) ;
#4647=ADVANCED_FACE ( 'NONE', ( #37488 ), #40281, .T. ) ;
#4651=CARTESIAN_POINT ( 'NONE',  ( 9.999999999999998224, 0.000000000000000000, -162.8750000040967905 ) ) ;
#4652=CARTESIAN_POINT ( 'NONE',  ( 10.81189881249999907, 6.242252689847868297, -88.40625000204839523 ) ) ;
#4653=ORIENTED_EDGE ( 'NONE', *, *, #41203, .T. ) ;
#4655=VERTEX_POINT ( 'NONE', #14154 ) ;
#4656=ORIENTED_EDGE ( 'NONE', *, *, #17738, .F. ) ;
#4657=CARTESIAN_POINT ( 'NONE',  ( 10.81189881249999729, 6.242252689847867408, -35.71875000204835260 ) ) ;
#4658=CARTESIAN_POINT ( 'NONE',  ( -5.405949406250003975, -9.363379034771801557, -24.34375000204835970 ) ) ;
#4659=CARTESIAN_POINT ( 'NONE',  ( 7.644554776091147741E-16, 12.48450537969573659, -16.15625000204837747 ) ) ;
#4660=CARTESIAN_POINT ( 'NONE',  ( 5.405949406249999534, 9.363379034771803333, -65.59375000204836681 ) ) ;
#4661=DIRECTION ( 'NONE',  ( -0.000000000000000000, -0.000000000000000000, 1.000000000000000000 ) ) ;
#4663=CARTESIAN_POINT ( 'NONE',  ( 10.81189881249999907, 6.242252689847868297, -185.7187500020483810 ) ) ;
#4666=CARTESIAN_POINT ( 'NONE',  ( 5.000000000000000000, 8.660254037844385522, -199.7500000000000000 ) ) ;
#4667=CYLINDRICAL_SURFACE ( 'NONE', #25390, 9.999999999999998224 ) ;
#4668=FACE_OUTER_BOUND ( 'NONE', #38926, .T. ) ;
#4670=CARTESIAN_POINT ( 'NONE',  ( 5.405949406249999534, 9.363379034771803333, -113.5937500020483810 ) ) ;
#4671=CARTESIAN_POINT ( 'NONE',  ( 9.999999999999998224, 0.000000000000000000, -18.87500000409675494 ) ) ;
#4672=VECTOR ( 'NONE', #37576, 1000.000000000000114 ) ;
#4673=CARTESIAN_POINT ( 'NONE',  ( -10.81189881249999729, 1.324075727343319199E-15, -86.28125000204838102 ) ) ;
#4674=CARTESIAN_POINT ( 'NONE',  ( 10.81189881249999551, -6.242252689847874514, -100.4687500020483952 ) ) ;
#4675=VECTOR ( 'NONE', #26378, 1000.000000000000000 ) ;
#4676=( BOUNDED_CURVE ( )  B_SPLINE_CURVE ( 2, ( #18230, #37670, #17798, #17368, #27319, #4438, #21475 ),
 .UNSPECIFIED., .F., .F. ) 
 B_SPLINE_CURVE_WITH_KNOTS ( ( 3, 2, 2, 3 ),
 ( 0.4626865671641792743, 0.4639303482587066596, 0.4651741293532339339, 0.4664179104477613191 ),
 .UNSPECIFIED. ) 
 CURVE ( )  GEOMETRIC_REPRESENTATION_ITEM ( )  RATIONAL_B_SPLINE_CURVE ( ( 0.9999999999999820144, 0.8660254037844566932, 1.000000000000000000, 0.8660254037844387076, 1.000000000000000000, 0.8660254037844267172, 1.000000000000011990 ) ) 
 REPRESENTATION_ITEM ( '' )  );
#4679=CARTESIAN_POINT ( 'NONE',  ( 5.000000000000000000, 8.660254037844385522, -150.6250000040967905 ) ) ;
#4684=CARTESIAN_POINT ( 'NONE',  ( -4.999999999999996447, 8.660254037844387298, -172.5000000000000284 ) ) ;
#4686=CARTESIAN_POINT ( 'NONE',  ( 4.999999999999992006, -8.660254037844389075, -77.24999999999998579 ) ) ;
#4688=CARTESIAN_POINT ( 'NONE',  ( -9.999999999999998224, 5.773502691896259087, -81.25000000409677625 ) ) ;
#4691=CARTESIAN_POINT ( 'NONE',  ( -2.293366432827344421E-15, -12.48450537969573659, -78.40625000204838102 ) ) ;
#4695=VERTEX_POINT ( 'NONE', #23915 ) ;
#4696=CARTESIAN_POINT ( 'NONE',  ( 5.000000000000000000, 8.660254037844385522, -1.749999999999973799 ) ) ;
#4698=CARTESIAN_POINT ( 'NONE',  ( 5.405949406249992428, -9.363379034771808662, -12.09375000204834727 ) ) ;
#4700=CARTESIAN_POINT ( 'NONE',  ( 10.81189881249999907, 6.242252689847868297, -131.9062500020484094 ) ) ;
#4701=CARTESIAN_POINT ( 'NONE',  ( 9.999999999999996447, -5.773502691896262640, -182.1250000000000000 ) ) ;
#4702=DIRECTION ( 'NONE',  ( -0.000000000000000000, -0.000000000000000000, 1.000000000000000000 ) ) ;
#4703=CARTESIAN_POINT ( 'NONE',  ( -5.405949406250003975, -9.363379034771801557, -108.5312500020483810 ) ) ;
#4704=ORIENTED_EDGE ( 'NONE', *, *, #10791, .T. ) ;
#4705=CARTESIAN_POINT ( 'NONE',  ( 5.000000000000000000, 8.660254037844385522, -138.6250000040967905 ) ) ;
#4707=ORIENTED_EDGE ( 'NONE', *, *, #1065, .F. ) ;
#4709=EDGE_CURVE ( 'NONE', #22217, #29348, #22078, .T. ) ;
#4710=CARTESIAN_POINT ( 'NONE',  ( 5.405949406249992428, -9.363379034771808662, -36.28125000204837391 ) ) ;
#4712=CARTESIAN_POINT ( 'NONE',  ( -5.405949406250003975, -9.363379034771801557, -84.34375000204836681 ) ) ;
#4713=DIRECTION ( 'NONE',  ( -0.000000000000000000, -0.000000000000000000, 1.000000000000000000 ) ) ;
#4714=CYLINDRICAL_SURFACE ( 'NONE', #464, 9.999999999999998224 ) ;
#4715=( BOUNDED_CURVE ( )  B_SPLINE_CURVE ( 2, ( #31853, #8328, #28606, #35082, #38094, #14766, #27962 ),
 .UNSPECIFIED., .F., .F. ) 
 B_SPLINE_CURVE_WITH_KNOTS ( ( 3, 2, 2, 3 ),
 ( 0.9029850746268659467, 0.9042288557213932210, 0.9054726368159207173, 0.9067164179104481025 ),
 .UNSPECIFIED. ) 
 CURVE ( )  GEOMETRIC_REPRESENTATION_ITEM ( )  RATIONAL_B_SPLINE_CURVE ( ( 0.9999999999999761302, 0.8660254037844625774, 1.000000000000000000, 0.8660254037844387076, 1.000000000000000000, 0.8660254037844028474, 1.000000000000035971 ) ) 
 REPRESENTATION_ITEM ( '' )  );
#4716=CARTESIAN_POINT ( 'NONE',  ( -9.999999999999998224, 1.224646799147353059E-15, -167.7500000000000000 ) ) ;
#4718=CARTESIAN_POINT ( 'NONE',  ( 10.00000000000102318, -5.773502691895667560, -68.12499999999995737 ) ) ;
#4719=CARTESIAN_POINT ( 'NONE',  ( -5.405949406250003975, -9.363379034771801557, -126.3437500020483952 ) ) ;
#4721=CARTESIAN_POINT ( 'NONE',  ( -2.293366432827344421E-15, -12.48450537969573659, -0.4062500020483658103 ) ) ;
#4724=CARTESIAN_POINT ( 'NONE',  ( -2.121150477449813534E-15, -11.54700538379251284, -176.7500000040967620 ) ) ;
#4726=CARTESIAN_POINT ( 'NONE',  ( -10.81189881249999729, -6.242252689847864744, -179.1562500020484094 ) ) ;
#4728=CARTESIAN_POINT ( 'NONE',  ( -9.999999999999998224, 1.224646799147353059E-15, -70.62500000409677625 ) ) ;
#4731=CARTESIAN_POINT ( 'NONE',  ( -2.293366432827344421E-15, -12.48450537969573659, -48.21875000204836681 ) ) ;
#4732=EDGE_CURVE ( 'NONE', #35021, #13374, #8855, .T. ) ;
#4734=CARTESIAN_POINT ( 'NONE',  ( 5.405949406249999534, 9.363379034771803333, -13.28125000204835615 ) ) ;
#4736=CARTESIAN_POINT ( 'NONE',  ( 9.999999999999998224, 0.000000000000000000, -192.8750000040967905 ) ) ;
#4738=CARTESIAN_POINT ( 'NONE',  ( 9.999999999999998224, 0.000000000000000000, -97.99999999999998579 ) ) ;
#4740=CARTESIAN_POINT ( 'NONE',  ( -9.999999999999998224, 1.224646799147353059E-15, -109.6250000040967763 ) ) ;
#4741=FACE_OUTER_BOUND ( 'NONE', #36183, .T. ) ;
#4744=CARTESIAN_POINT ( 'NONE',  ( -5.405949406249996869, 9.363379034771805109, -103.0312500020483952 ) ) ;
#4745=VERTEX_POINT ( 'NONE', #30602 ) ;
#4748=CARTESIAN_POINT ( 'NONE',  ( -10.81189881249999907, -6.242252689847864744, -165.6562500020483810 ) ) ;
#4750=VERTEX_POINT ( 'NONE', #7719 ) ;
#4751=CARTESIAN_POINT ( 'NONE',  ( 7.070501591499377789E-16, 11.54700538379251284, -22.62499999999997868 ) ) ;
#4752=CARTESIAN_POINT ( 'NONE',  ( -5.405949406250003975, -9.363379034771801557, -35.03125000204837391 ) ) ;
#4753=CARTESIAN_POINT ( 'NONE',  ( 9.999999999999998224, 0.000000000000000000, -165.5000000000000000 ) ) ;
#4754=DIRECTION ( 'NONE',  ( -0.000000000000000000, -0.000000000000000000, 1.000000000000000000 ) ) ;
#4757=CARTESIAN_POINT ( 'NONE',  ( 7.644554776091147741E-16, 12.48450537969573659, -130.1562500020483810 ) ) ;
#4758=CARTESIAN_POINT ( 'NONE',  ( 5.000000000000000000, 8.660254037844385522, -46.74999999999998579 ) ) ;
#4759=CARTESIAN_POINT ( 'NONE',  ( -5.000000000000003553, -8.660254037844383745, -119.8750000040967905 ) ) ;
#4760=VERTEX_POINT ( 'NONE', #17615 ) ;
#4761=CARTESIAN_POINT ( 'NONE',  ( 10.81189881249999729, 0.000000000000000000, -61.53125000204837391 ) ) ;
#4762=EDGE_CURVE ( 'NONE', #24456, #35132, #10210, .T. ) ;
#4763=ORIENTED_EDGE ( 'NONE', *, *, #9324, .F. ) ;
#4767=CARTESIAN_POINT ( 'NONE',  ( 7.644554776091147741E-16, 12.48450537969573659, -168.9687500020483810 ) ) ;
#4769=CARTESIAN_POINT ( 'NONE',  ( 5.405949406249999534, 9.363379034771803333, -11.59375000204834727 ) ) ;
#4770=AXIS2_PLACEMENT_3D ( 'NONE', #7078, #13730, #17401 ) ;
#4772=CARTESIAN_POINT ( 'NONE',  ( -5.405949406250003975, -9.363379034771801557, -151.8437500020483810 ) ) ;
#4773=CARTESIAN_POINT ( 'NONE',  ( -5.405949406249996869, 9.363379034771805109, -125.3437500020483952 ) ) ;
#4774=CARTESIAN_POINT ( 'NONE',  ( 5.405949406249999534, 9.363379034771803333, -107.7812500020483810 ) ) ;
#4778=CARTESIAN_POINT ( 'NONE',  ( 10.81189881249999551, -6.242252689847874514, 0.03124999795165228286 ) ) ;
#4781=CARTESIAN_POINT ( 'NONE',  ( 10.00000000000006040, -5.773502691896226224, -196.0000000040968473 ) ) ;
#4784=CARTESIAN_POINT ( 'NONE',  ( -5.405949406250003975, -9.363379034771801557, -75.34375000204838102 ) ) ;
#4785=CARTESIAN_POINT ( 'NONE',  ( -10.81189881249999729, 6.242252689847871849, -65.21875000204838102 ) ) ;
#4787=CARTESIAN_POINT ( 'NONE',  ( -10.81189881249999907, -6.242252689847864744, -32.15625000204835970 ) ) ;
#4791=CARTESIAN_POINT ( 'NONE',  ( 10.00000000000000000, 5.773502691896255534, -123.3749999999999858 ) ) ;
#4792=CARTESIAN_POINT ( 'NONE',  ( 10.81189881249999729, 6.242252689847867408, -130.4062500020483810 ) ) ;
#4793=CARTESIAN_POINT ( 'NONE',  ( -5.000000000000003553, -8.660254037844383745, -67.37500000409676204 ) ) ;
#4795=CARTESIAN_POINT ( 'NONE',  ( 10.81189881249999551, -6.242252689847874514, -21.15625000204836681 ) ) ;
#4800=CARTESIAN_POINT ( 'NONE',  ( -5.000000000000003553, -8.660254037844383745, -34.37500000409676915 ) ) ;
#4801=( BOUNDED_CURVE ( )  B_SPLINE_CURVE ( 2, ( #14104, #23437, #7451, #7237, #10250, #16929, #4425 ),
 .UNSPECIFIED., .F., .F. ) 
 B_SPLINE_CURVE_WITH_KNOTS ( ( 3, 2, 2, 3 ),
 ( 0.4440298507462688282, 0.4452736318407962135, 0.4465174129353234878, 0.4477611940298508730 ),
 .UNSPECIFIED. ) 
 CURVE ( )  GEOMETRIC_REPRESENTATION_ITEM ( )  RATIONAL_B_SPLINE_CURVE ( ( 0.9999999999999820144, 0.8660254037844566932, 1.000000000000000000, 0.8660254037844387076, 1.000000000000000000, 0.8660254037844267172, 1.000000000000011990 ) ) 
 REPRESENTATION_ITEM ( '' )  );
#4802=CARTESIAN_POINT ( 'NONE',  ( 9.999999999999998224, 0.000000000000000000, -149.0000000000000000 ) ) ;
#4804=CARTESIAN_POINT ( 'NONE',  ( 9.999999999999998224, 0.000000000000000000, -191.0000000000000000 ) ) ;
#4805=CARTESIAN_POINT ( 'NONE',  ( -10.81189881249999907, -6.242252689847864744, -153.6562500020484094 ) ) ;
#4806=AXIS2_PLACEMENT_3D ( 'NONE', #42161, #19286, #18654 ) ;
#4807=CARTESIAN_POINT ( 'NONE',  ( -5.405949406250003975, -9.363379034771801557, -126.3437500020483952 ) ) ;
#4809=ORIENTED_EDGE ( 'NONE', *, *, #22059, .T. ) ;
#4810=DIRECTION ( 'NONE',  ( -0.000000000000000000, -0.000000000000000000, 1.000000000000000000 ) ) ;
#4811=ORIENTED_EDGE ( 'NONE', *, *, #24808, .T. ) ;
#4813=ORIENTED_EDGE ( 'NONE', *, *, #14906, .T. ) ;
#4814=EDGE_CURVE ( 'NONE', #6986, #3969, #27624, .T. ) ;
#4815=ORIENTED_EDGE ( 'NONE', *, *, #26459, .T. ) ;
#4817=ADVANCED_FACE ( 'NONE', ( #36770 ), #7003, .T. ) ;
#4818=CARTESIAN_POINT ( 'NONE',  ( -10.81189881249999907, -6.242252689847864744, -190.9687500020484379 ) ) ;
#4819=CARTESIAN_POINT ( 'NONE',  ( -10.81189881249999729, 6.242252689847871849, -38.21875000204836681 ) ) ;
#4820=CARTESIAN_POINT ( 'NONE',  ( 4.168882320602625313, -9.758565647681585631, 6.544024882825217862E-15 ) ) ;
#4821=CARTESIAN_POINT ( 'NONE',  ( 7.070501591499376803E-16, 11.54700538379251284, -139.6250000000000000 ) ) ;
#4822=CARTESIAN_POINT ( 'NONE',  ( -5.405949406250003975, -9.363379034771801557, -174.3437500020484094 ) ) ;
#4823=CARTESIAN_POINT ( 'NONE',  ( 10.81189881249999907, 6.242252689847868297, -164.7187500020483810 ) ) ;
#4829=CARTESIAN_POINT ( 'NONE',  ( 5.000000000000000000, 8.660254037844385522, -87.24999999999998579 ) ) ;
#4832=CARTESIAN_POINT ( 'NONE',  ( -5.405949406250003975, -9.363379034771801557, -91.84375000204838102 ) ) ;
#4833=CARTESIAN_POINT ( 'NONE',  ( 4.999999999999992006, -8.660254037844389075, -82.12500000409676204 ) ) ;
#4834=CARTESIAN_POINT ( 'NONE',  ( -10.81189881249999907, -6.242252689847864744, -56.15625000204837391 ) ) ;
#4837=EDGE_CURVE ( 'NONE', #33095, #42590, #11595, .T. ) ;
#4838=CARTESIAN_POINT ( 'NONE',  ( 7.644554776091147741E-16, 12.48450537969573659, -112.1562500020483810 ) ) ;
#4839=CARTESIAN_POINT ( 'NONE',  ( 10.81189881249999729, 0.000000000000000000, -153.0312500020484094 ) ) ;
#4840=DIRECTION ( 'NONE',  ( -0.000000000000000000, -0.000000000000000000, 1.000000000000000000 ) ) ;
#4842=CARTESIAN_POINT ( 'NONE',  ( -4.999999999999996447, 8.660254037844387298, -130.8750000040967905 ) ) ;
#4844=( BOUNDED_CURVE ( )  B_SPLINE_CURVE ( 2, ( #28752, #36059, #28958, #29370, #9515, #15760, #16175 ),
 .UNSPECIFIED., .F., .F. ) 
 B_SPLINE_CURVE_WITH_KNOTS ( ( 3, 2, 2, 3 ),
 ( 0.9514925373134331954, 0.9527363184079605807, 0.9539800995024879660, 0.9552238805970153512 ),
 .UNSPECIFIED. ) 
 CURVE ( )  GEOMETRIC_REPRESENTATION_ITEM ( )  RATIONAL_B_SPLINE_CURVE ( ( 0.9999999999999641398, 0.8660254037844745678, 1.000000000000000000, 0.8660254037844387076, 1.000000000000000000, 0.8660254037843908570, 1.000000000000047740 ) ) 
 REPRESENTATION_ITEM ( '' )  );
#4845=VERTEX_POINT ( 'NONE', #16898 ) ;
#4850=CARTESIAN_POINT ( 'NONE',  ( 7.644554776091147741E-16, 12.48450537969573659, -184.1562500020484094 ) ) ;
#4851=ORIENTED_EDGE ( 'NONE', *, *, #29617, .T. ) ;
#4853=CARTESIAN_POINT ( 'NONE',  ( 9.999999999999996447, -5.773502691896262640, -59.50000000409676915 ) ) ;
#4854=EDGE_CURVE ( 'NONE', #38736, #35715, #39464, .T. ) ;
#4856=CARTESIAN_POINT ( 'NONE',  ( 10.00000000000012790, 5.773502691896179151, -171.7500000040967620 ) ) ;
#4858=CARTESIAN_POINT ( 'NONE',  ( 10.81189881249999729, 6.242252689847867408, -49.40625000204837391 ) ) ;
#4862=CARTESIAN_POINT ( 'NONE',  ( 5.405949406249992428, -9.363379034771808662, -175.7812500020484094 ) ) ;
#4863=CARTESIAN_POINT ( 'NONE',  ( 9.999999999999479527, 5.773502691896553074, -147.7500000040967620 ) ) ;
#4865=ORIENTED_EDGE ( 'NONE', *, *, #21422, .T. ) ;
#4867=CARTESIAN_POINT ( 'NONE',  ( -9.999999999999998224, 1.224646799147353059E-15, -154.2500000000000000 ) ) ;
#4868=CARTESIAN_POINT ( 'NONE',  ( -9.999999999999998224, 1.224646799147353059E-15, -1.249999999999973355 ) ) ;
#4869=CARTESIAN_POINT ( 'NONE',  ( -5.405949406250003975, -9.363379034771801557, -86.03125000204838102 ) ) ;
#4870=ORIENTED_EDGE ( 'NONE', *, *, #929, .F. ) ;
#4871=AXIS2_PLACEMENT_3D ( 'NONE', #37827, #8698, #2434 ) ;
#4872=DIRECTION ( 'NONE',  ( -0.000000000000000000, -0.000000000000000000, 1.000000000000000000 ) ) ;
#4873=VERTEX_POINT ( 'NONE', #1166 ) ;
#4875=EDGE_CURVE ( 'NONE', #39779, #4966, #14621, .T. ) ;
#4876=CARTESIAN_POINT ( 'NONE',  ( -2.293366432827344421E-15, -12.48450537969573659, -34.71875000204835260 ) ) ;
#4877=CARTESIAN_POINT ( 'NONE',  ( 10.81189881249999729, 0.000000000000000000, -23.84375000204835970 ) ) ;
#4878=CARTESIAN_POINT ( 'NONE',  ( 10.81189881249999907, 6.242252689847868297, -14.90625000204837036 ) ) ;
#4879=CARTESIAN_POINT ( 'NONE',  ( -5.405949406250003975, -9.363379034771801557, -63.34375000204836681 ) ) ;
#4880=VERTEX_POINT ( 'NONE', #24267 ) ;
#4881=ADVANCED_FACE ( 'NONE', ( #3765 ), #40002, .T. ) ;
#4882=CARTESIAN_POINT ( 'NONE',  ( -9.999999999998969713, -5.773502691896847949, -131.6250000000000000 ) ) ;
#4884=CARTESIAN_POINT ( 'NONE',  ( 5.405949406249992428, -9.363379034771808662, -184.5937500020483810 ) ) ;
#4887=CARTESIAN_POINT ( 'NONE',  ( 9.999999999999998224, 0.000000000000000000, -182.3750000040967905 ) ) ;
#4890=CARTESIAN_POINT ( 'NONE',  ( 0.000000000000000000, 0.000000000000000000, -200.0000000000000000 ) ) ;
#4891=CARTESIAN_POINT ( 'NONE',  ( -10.81189881249999907, -6.242252689847864744, -115.9687500020483810 ) ) ;
#4892=DIRECTION ( 'NONE',  ( -0.000000000000000000, -0.000000000000000000, 1.000000000000000000 ) ) ;
#4893=CARTESIAN_POINT ( 'NONE',  ( -2.293366432827344421E-15, -12.48450537969573659, -84.40625000204838102 ) ) ;
#4894=CARTESIAN_POINT ( 'NONE',  ( 10.81189881249999551, -6.242252689847874514, -88.46875000204836681 ) ) ;
#4897=CARTESIAN_POINT ( 'NONE',  ( 9.999999999999998224, 0.000000000000000000, -156.8750000040967905 ) ) ;
#4899=ADVANCED_FACE ( 'NONE', ( #37413 ), #14075, .T. ) ;
#4906=CARTESIAN_POINT ( 'NONE',  ( -9.999999999999998224, 1.224646799147353059E-15, -10.24999999999995381 ) ) ;
#4907=CARTESIAN_POINT ( 'NONE',  ( 4.999999999999992006, -8.660254037844389075, -72.74999999999998579 ) ) ;
#4909=CARTESIAN_POINT ( 'NONE',  ( -9.999999999999998224, 1.224646799147353059E-15, -85.62500000409677625 ) ) ;
#4912=CARTESIAN_POINT ( 'NONE',  ( 7.644554776091147741E-16, 12.48450537969573659, -79.15625000204838102 ) ) ;
#4916=VERTEX_POINT ( 'NONE', #33549 ) ;
#4917=CARTESIAN_POINT ( 'NONE',  ( 9.999999999999998224, 0.000000000000000000, -3.499999999999975131 ) ) ;
#4919=CARTESIAN_POINT ( 'NONE',  ( 10.81189881249999729, 6.242252689847867408, -16.21875000204836326 ) ) ;
#4923=CARTESIAN_POINT ( 'NONE',  ( -5.405949406250003975, -9.363379034771801557, -131.0312500020484094 ) ) ;
#4924=CARTESIAN_POINT ( 'NONE',  ( 5.000000000000000000, 8.660254037844385522, -184.7500000000000000 ) ) ;
#4925=CARTESIAN_POINT ( 'NONE',  ( 9.999999999999998224, 0.000000000000000000, -200.0000000000000000 ) ) ;
#4926=CARTESIAN_POINT ( 'NONE',  ( 7.644554776091147741E-16, 12.48450537969573659, -112.1562500020483810 ) ) ;
#4927=ORIENTED_EDGE ( 'NONE', *, *, #11221, .F. ) ;
#4929=ORIENTED_EDGE ( 'NONE', *, *, #1611, .T. ) ;
#4930=ORIENTED_EDGE ( 'NONE', *, *, #40243, .F. ) ;
#4931=CARTESIAN_POINT ( 'NONE',  ( 10.81189881249999729, 0.000000000000000000, -36.03125000204837391 ) ) ;
#4934=CARTESIAN_POINT ( 'NONE',  ( 10.81189881249999551, -6.242252689847874514, -86.96875000204838102 ) ) ;
#4936=DIRECTION ( 'NONE',  ( -0.000000000000000000, -0.000000000000000000, 1.000000000000000000 ) ) ;
#4940=VECTOR ( 'NONE', #20305, 1000.000000000000000 ) ;
#4943=CARTESIAN_POINT ( 'NONE',  ( 10.81189881249999729, 6.242252689847867408, -121.2187500020483952 ) ) ;
#4948=CARTESIAN_POINT ( 'NONE',  ( -4.999999999999996447, 8.660254037844387298, -178.8750000040967905 ) ) ;
#4949=CARTESIAN_POINT ( 'NONE',  ( 7.644554776091147741E-16, 12.48450537969573659, -169.1562500020484094 ) ) ;
#4950=CARTESIAN_POINT ( 'NONE',  ( 9.999999999999998224, 0.000000000000000000, -103.9999999999999858 ) ) ;
#4953=CARTESIAN_POINT ( 'NONE',  ( 5.405949406249992428, -9.363379034771808662, -54.09375000204835970 ) ) ;
#4955=CARTESIAN_POINT ( 'NONE',  ( -10.81189881249999907, -6.242252689847864744, -9.656250002048379244 ) ) ;
#4957=DIRECTION ( 'NONE',  ( -0.000000000000000000, -0.000000000000000000, 1.000000000000000000 ) ) ;
#4959=CARTESIAN_POINT ( 'NONE',  ( -2.121150477449813534E-15, -11.54700538379251284, -101.3750000000000000 ) ) ;
#4961=CARTESIAN_POINT ( 'NONE',  ( 9.999999999999998224, 0.000000000000000000, -108.8750000040967763 ) ) ;
#4964=CARTESIAN_POINT ( 'NONE',  ( -10.81189881249999729, 6.242252689847871849, -102.9062500020483952 ) ) ;
#4965=EDGE_CURVE ( 'NONE', #3711, #41596, #38331, .T. ) ;
#4966=VERTEX_POINT ( 'NONE', #4182 ) ;
#4969=CARTESIAN_POINT ( 'NONE',  ( 5.000000000000000000, 8.660254037844385522, -141.6250000040967905 ) ) ;
#4970=CARTESIAN_POINT ( 'NONE',  ( 5.405949406249999534, 9.363379034771803333, -161.7812500020484094 ) ) ;
#4972=ORIENTED_EDGE ( 'NONE', *, *, #30168, .F. ) ;
#4973=CARTESIAN_POINT ( 'NONE',  ( 4.999999999999992006, -8.660254037844389075, -21.74999999999996447 ) ) ;
#4974=CARTESIAN_POINT ( 'NONE',  ( -10.81189881249999729, -6.242252689847864744, -26.15625000204837391 ) ) ;
#4975=CARTESIAN_POINT ( 'NONE',  ( 10.00000000000000000, 5.773502691896255534, -165.3749999999999716 ) ) ;
#4976=CARTESIAN_POINT ( 'NONE',  ( -5.000000000000003553, -8.660254037844383745, -103.0000000000000000 ) ) ;
#4978=( BOUNDED_CURVE ( )  B_SPLINE_CURVE ( 2, ( #40932, #14387, #1904, #34499, #31689, #11374, #28016 ),
 .UNSPECIFIED., .F., .F. ) 
 B_SPLINE_CURVE_WITH_KNOTS ( ( 3, 2, 2, 3 ),
 ( 0.6679104477611942370, 0.6691542288557216223, 0.6703980099502490075, 0.6716417910447763928 ),
 .UNSPECIFIED. ) 
 CURVE ( )  GEOMETRIC_REPRESENTATION_ITEM ( )  RATIONAL_B_SPLINE_CURVE ( ( 0.9999999999999761302, 0.8660254037844625774, 1.000000000000000000, 0.8660254037844387076, 1.000000000000000000, 0.8660254037844148378, 1.000000000000023981 ) ) 
 REPRESENTATION_ITEM ( '' )  );
#4979=AXIS2_PLACEMENT_3D ( 'NONE', #16034, #39562, #42584 ) ;
#4980=DIRECTION ( 'NONE',  ( 0.000000000000000000, 0.000000000000000000, 1.000000000000000000 ) ) ;
#4981=CARTESIAN_POINT ( 'NONE',  ( 10.81189881249999729, 0.000000000000000000, -135.0312500020484094 ) ) ;
#4982=CARTESIAN_POINT ( 'NONE',  ( 7.547620300323909959, 7.372587587660208719, -7.434655202704447971E-15 ) ) ;
#4984=ORIENTED_EDGE ( 'NONE', *, *, #20639, .F. ) ;
#4985=( BOUNDED_SURFACE ( )  B_SPLINE_SURFACE ( 1, 2, ( 
 ( #8815, #35151, #29096, #38163, #12659, #5575, #9446, #15477, #18729, #35786, #39008, #12246, #22611, #25438, #35363, #5791, #18944, #32128, #39630, #3824, #22827, #26484, #7060, #35991, #13504, #16531, #596, #10278, #10070, #26693, #12871, #10489, #30156, #23465, #39845, #13295, #20210, #36612, #6425, #33399, #23247, #3616, #16315, #19568, #16743, #39217, #29513, #16960, #36825, #386, #42444, #13713, #3188, #29943, #29728, #32752, #39429, #26902, #174, #40058, #23678, #19363, #42655, #23037, #9655, #26067, #32548, #2978, #32967, #16103, #13080, #26276, #9864, #36193, #6630, #19781, #29297, #3394, #36407, #6840, #19993, #33184, #20628, #21277, #27761, #8124, #34250, #40898, #37684, #24755, #37468, #33817, #1226, #20420, #11547, #10699, #11340, #14783, #40262, #24535, #24325, #7267, #10915, #30582, #33608, #23893, #14572, #4240, #20847, #4663, #17814, #7479, #7912, #40467, #27550, #13926, #21059, #24108, #4884, #18031, #37246, #37041, #34462, #17382, #1012, #30792, #802, #27979, #7693, #31009, #1438, #31228, #4026, #41107, #1653, #14132, #30372, #14352, #17171, #27333, #27121, #34031, #4451, #17593, #40684, #11122, #15428, #1873, #41967, #18464, #28626, #28415, #2710, #19104, #35312, #8972, #31652, #2302, #41553, #22349, #25180, #21496, #41757, #2086, #38530, #14999, #15842, #18674, #11984, #34888, #32286, #38322, #41331, #8763, #5312, #35525, #21919, #38112, #5954, #22138, #31871, #8556, #5742, #35099, #12192, #15216, #5524, #25594, #21706, #28198, #29042, #9178, #31437, #25383, #18895, #15634, #11769, #32075, #24970, #2510, #28836, #42180, #12401, #38749, #12607, #37902, #8345, #34678, #5100, #18246, #16054, #33346, #19940, #6372, #16690, #35931, #30102, #26012, #23410, #38957, #9806, #39164, #10223, #20156, #39790, #42602, #29245, #32910, #36142, #326, #16901, #3767, #36352, #19302, #42389, #33129, #22556, #541, #6785, #3343, #29886, #6162, #16475, #26427, #12821, #22985, #32700, #19516, #39578, #32496, #13446, #9596, #25801, #6573, #35732, #9391, #10014, #13028, #3556, #19729, #26641, #29674, #2924, #22771, #118, #36559, #3131, #13240, #7005, #16260, #29459, #23191, #26221, #39370, #20788, #7857, #7209, #4823, #24478, #17754, #34195, #7638, #1382, #4613, #751, #14512, #33977, #40626, #10643, #13873, #11068, #33551, #23835, #30949, #31170, #37415, #36772, #27706, #40211, #24269, #24048, #27068, #33762, #21219, #10857, #21006, #17970, #13659, #36986, #17329, #3976, #20362, #40844, #8069, #27275, #26850, #7422, #20572, #17116, #30316, #4185, #30532, #11283, #959, #14077, #40412, #37630, #23627, #37189, #34404, #40005, #10436, #4398, #17537, #30739, #1169, #14292, #27492, #38265, #14728, #1816, #18189, #14942, #12140, #41702, #31381, #21433, #28356, #22084, #31596, #41494, #25545, #35259, #8712, #38478, #37844, #35471, #12346, #5693, #18842, #21866, #32023, #2450, #28142, #15583, #35045, #28572, #41275, #11711, #25333, #34618, #24910, #28784, #19051, #8922, #24698, #41915, #38057, #38695, #11928, #8497, #21650, #9129, #25121, #22299, #5895, #1599, #34831, #5255, #5044, #8286, #27920, #41052, #15158, #11495, #18407, #2029, #5472, #18622, #31818, #2252, #15372, #16002, #35680, #9336, #13187, #42128, #2872, #3498, #9962, #33072, #16421, #23140, #19889, #6949, #19675, #29197, #26170, #2659, #32445, #6108, #42337, #62, #29619, #19255, #22505, #16207, #36304, #19467, #16637, #26589, #29839, #6320, #12767, #39317, #42549, #6735, #23360, #39740, #26380, #25754, #25961, #39531, #28989, #32233, #276, #9756, #13397, #12560, #22937, #32862, #39109, #29409, #9546, #22720, #3293, #38907, #10175, #35885, #36512, #12973, #32652, #15793, #3080, #36090, #6525, #910, #11021, #27220, #39952, #36720, #40365, #4561, #23573, #10806, #7809, #7159, #14241, #17066, #13821, #24215, #10384, #27654, #27444, #702, #37366, #30263, #24435, #20311, #17702, #33295, #4135, #33504, #37578, #3928, #20957, #40795, #27014, #40580, #37139, #20104, #23779, #40161, #3721, #10592, #34143, #36932, #33710, #17492, #4351, #7376, #7587, #20522, #23999, #26802, #20740, #17276, #30897, #1333, #30481, #14025, #14464, #33927, #30685, #1116, #13610, #11236, #16850, #30048, #495, #38808, #8023, #16109, #42240, #15482, #31118, #15696, #2773, #24649, #14684, #22195, #29305, #21167, #25652, #9235, #28895, #27871, #12665, #31927, #42028, #41814, #42451, #32556, #6010, #22404, #2355, #12459, #12252, #35793, #38590, #34356, #35581, #28686, #19159, #41005, #12878, #32136, #25444, #5581, #2985, #9031, #11449, #35370, #18735, #6224, #5797, #8820, #19369, #32349, #2567, #21977, #15899, #18949, #29104, #25860, #39015, #9452, #35156, #37792, #26073, #22618, #1551, #4773, #17921, #16968, #29520, #33193, #3195, #392, #20217, #7275, #30163, #604, #26700, #13719, #26909, #13932, #183, #19787, #39224, #13086, #3832, #23042, #10078, #36621, #23473, #39436, #39852, #29737, #16751, #16321, #10286, #13303, #36832, #20429, #26492, #26286, #40066, #9869, #32974, #20001, #32758, #17180, #39637, #13511, #7068, #33407, #9662, #4033, #10497, #3403, #19575, #3624, #22835, #42662, #23685, #6431, #36200, #33615, #30378, #810, #35997, #6637, #16538, #23255, #36414, #6848, #29952, #40269, #27340, #1019, #40474, #37692, #24541, #14139, #4249, #11132, #4891, #14359, #11554, #21503, #41115, #1233, #30588, #34257, #37475, #1659, #18252, #34685, #8133, #20636, #17391, #34469, #23903, #1878, #21283, #4670, #31235, #7485, #17821, #27768, #10922, #24334, #34038, #37252, #40906, #33825, #14791, #24116, #5105, #7919, #37048, #31443, #11348, #27557, #18039, #21066, #27986, #31016, #7704, #20854, #1446, #24764, #4458, #14581, #37908, #17601, #8352, #27126, #10706, #30797, #40691, #9184, #8563, #6168, #25807, #19110, #35531, #8978, #2717, #5960, #2093, #15848, #35319, #29048, #41975, #32293, #42187, #32501, #2516, #28422, #22145, #28204, #15223, #31659, #41558, #25600, #12407, #11991, #34894, #41765, #12614, #2309, #38964, #9398, #22562, #31878, #18471, #5748, #25388, #35740, #19308, #15006, #38758, #21713, #5318, #22355, #11775, #41338, #24977, #18901, #38118, #25187, #32082, #15641, #38327, #12198, #21925, #8769, #28841, #35106, #5531, #18680, #15435, #38537, #28633, #7216, #16697, #32916, #23417, #26433, #36565, #10020, #22777, #19522, #23198, #30108, #6379, #36358, #33353, #32706, #39796, #125, #26858, #7011, #6791, #10229, #39170, #36780, #13664, #20163, #3773, #39584, #16907, #547, #3139, #40012, #19947, #29893, #42607, #16266, #333, #35938, #13035, #10442, #20368, #26647, #26018, #23634, #29465, #13452, #13246, #26228, #22990, #2931, #33135, #16060, #29252, #42396, #39376, #6579, #9812, #9604, #12827, #36147, #16482, #19736, #3349, #29681, #3563, #13878, #36993, #14084, #7428, #14737, #8297, #10651, #14521, #757, #4191, #4832, #11291, #23843, #17544, #24486, #20796, #17978, #27930, #31178, #7645, #20579, #40634, #1178, #8077, #24706, #41060, #1391, #27074, #33769, #40852, #30324, #33557, #27714, #11074, #37638, #40217, #24277, #34203, #17336, #30746, #40420, #966, #4619, #30539, #21228, #27284, #11504, #14299, #10864, #37852, #17765, #33984, #34414, #27499, #1607, #37422, #24055, #37197, #7865, #3981, #4405, #21013, #17122, #30959, #15592, #18631, #2668, #12356, #28580, #28793, #14951, #12570, #32241, #25554, #41924, #15382, #9139, #38705, #8505, #22307, #41710, #5702, #18415, #21659, #18853, #41283, #31605, #35480, #38916, #2461, #1824, #5907, #5263, #32033, #31825, #34839, #41504, #28998, #2261, #19060, #25763, #21441, #2037, #25128, #11722, #28149, #15802, #42139, #35053, #34625, #15168, #28365, #24920, #38064, #11936, #38274, #8720, #5052, #18198, #21875, #31389, #5481, #12148, #25340, #38487, #8931, #22095, #35269, #39751, #26814, #39541, #22730, #3303, #22516, #9556, #25971, #35896, #19899, #6746, #39122, #29849, #39327, #36521, #3731, #23371, #26180, #12779, #16431, #19688, #26601, #506, #16861, #33083, #2882, #42347, #16648, #6118, #9347, #3511, #29630, #13408, #32456, #73, #9972, #6333, #36101, #16219, #19476, #23152, #16012, #10186, #32662, #30064, #6535, #19263, #13622, #36314, #9767, #287, #32872, #6961, #13197, #29208, #3092, #26390, #20118, #29419, #33306, #35689, #42559, #12983, #22947, #21179, #30910, #4364, #34155, #33517, #31132, #8035, #1346, #17715, #33942, #27670, #14475, #27028, #40808, #17503, #24228, #36946, #40173, #37379, #17078, #7388, #11248, #14695, #20969, #20323, #24446, #23791, #7822, #7599, #10604, #17291, #4785, #37153, #4573, #1565, #39966, #20535, #922, #30276, #3940, #37591, #34369, #10818, #10396, #33724, #4147, #715, #13834, #30495, #14037, #27233, #17933, #23586, #40376, #36733, #7171, #24011, #20754, #30698, #1130, #14253, #27456, #40592, #11034, #15339, #41235, #21830, #41017, #28107, #1778, #11673, #38441, #25298, #14908, #5012, #11891, #11461, #25086, #24873, #32197, #31348, #31988, #35430, #18153, #5652, #2207, #2624, #31562, #8467, #27884, #38023, #35221, #21618, #41456, #8885, #12103, #34797, #28536, #18373, #5439, #34582, #41668, #1995, #25509, #38657, #15120, #5217, #18800, #28315, #38231, #8676, #21397, #5858, #35009, #22048, #2414, #15546, #24662, #19012, #28748, #37804, #41874, #12311, #18591, #31777, #9094, #22261, #8250, #28954, #32822, #16379, #36054, #22465, #19848, #39071, #6490, #6282, #23318, #39702, #13147, #29580, #9510, #22898, #19428, #240, #3043, #42091, #19638, #22680, #24, #35642, #36473, #39283, #32618, #12722, #10138, #16171, #19219, #29366, #25920, #13362, #42506, #15965, #26554, #26342, #9716, #29161, #39494, #12933, #3252, #35849, #26129, #3462, #42301, #6070, #6907, #29800, #9295, #9925, #23104, #36266, #32409, #6697, #2831, #33033, #16597, #20061, #33256, #15756, #12524, #25717, #38866, #3892, #666, #30645, #23533, #20913, #33888, #30226, #17449, #17027, #4517, #20278, #10981, #1076, #30440, #4310, #26762, #34096, #24176, #14201, #27401, #17240, #40537, #37323, #7123, #7770, #871, #23959, #13784, #33466, #37103, #10345, #26967, #17661, #3682, #16810, #39915, #30009, #40125, #455, #13987, #10555, #36894, #13571, #10770, #36683, #23741, #7338, #20487, #33673, #7547, #27184, #4099, #40328, #20700, #12655, #22822, #6421, #2971, #22604, #16099, #35985, #29291, #23460, #16952, #19357, #23242, #9439, #12866, #13500, #19988, #379, #26478, #33179, #29939, #42229, #29724, #26061, #36186, #25848, #42439, #39212, #9649, #10064, #39625, #19561, #32543, #26271, #3610, #29506, #26688, #36607, #39841, #16311, #32747, #6624, #9857, #16739, #33394, #7055, #36401, #35780, #3184, #6834, #39003, #6212, #10273, #19776, #20205, #42649, #32961, #169, #13076, #39424, #23033, #3389, #13291, #16526, #3817, #13920, #8118, #14126, #40052, #34456, #1221, #17377, #7906, #10910, #21054, #37240, #7261, #4020, #7687, #14566, #33601, #20842, #17808, #17164, #24319, #27328, #11334, #1008, #30366, #40891, #14346, #24101, #796, #30787, #30577, #34025, #27114, #40462, #31004, #40256, #20413, #27755, #1433, #23673, #4447, #10692, #34244, #23888, #17588, #36820, #27544, #11117, #24528, #4658, #37678, #40678, #21270, #4877, #37036, #7472, #30150, #20621, #588, #37463, #33811, #13706, #4235, #26897, #10483, #29413, #36308, #13191, #6529, #22941, #39115, #32866, #36095, #32237, #3298, #22724, #42553, #42133, #2663, #12977, #22303, #12564, #19680, #19893, #26174, #25549, #16425, #28993, #39320, #12772, #15797, #22510, #9966, #42341, #9760, #6739, #2456, #25758, #6112, #35475, #9133, #29623, #39536, #16006, #15587, #38911, #9342, #5901, #38699, #19055, #35684, #19259, #26384, #28788, #32450, #66, #12351, #2876, #23145, #41919, #29201, #25965, #9550, #35889, #6326, #32656, #19471, #3084, #16212, #33299, #6953, #3724, #915, #30486, #20109, #10179, #17071, #10811, #20316, #17497, #27449, #4356, #7164, #36516, #40166, #707, #7592, #24220, #40585, #14030, #37371, #16854, #37144, #11026, #23364, #24004, #7381, #7814, #36725, #13615, #33077, #30056, #40370, #500, #3933, #27226, #17281, #26807, #20527, #23578, #10598, #39744, #33715, #33510, #30690, #1123, #30268, #39958, #20746, #10389, #13826, #27020, #26594, #3503, #23784, #4140, #33933, #14246, #16641, #29843, #281, #13402, #36939, #34789, #21390, #37583, #27659, #34573, #41661, #34148, #38014, #21610, #41228, #40800, #25079, #1556, #11665, #11454, #28529, #2198, #18366, #5210, #14688, #28100, #24654, #5431, #8242, #4566, #24866, #27877, #31554, #11241, #12097, #1771, #37797, #17926, #15332, #5004, #24440, #18145, #31123, #18582, #31341, #21172, #31770, #1987, #14901, #34362, #15113, #8459, #28308, #41009, #41447, #8668, #4778, #8028, #25290, #35002, #14469, #11883 ),
 ( #38224, #21822, #38435, #20962, #17708, #30903, #1338, #18792, #22253, #22888, #29359, #9709, #35842, #42498, #39275, #26334, #39064, #35423, #2824, #22041, #9085, #25501, #5850, #19420, #6274, #38650, #28740, #35635, #12926, #38859, #36047, #3245, #6483, #25709, #12304, #15957, #19212, #26121, #16, #16371, #32611, #2407, #41866, #16163, #5643, #8878, #3036, #29154, #19630, #31981, #42293, #9502, #19005, #6062, #15748, #32190, #22671, #15538, #32814, #2617, #29571, #32401, #28947, #13139, #35213, #9286, #42084, #12715, #12516, #25912, #22458, #13354, #17020, #23952, #232, #3885, #27177, #26545, #33667, #36675, #20693, #23095, #30219, #20053, #23734, #30638, #7539, #864, #17233, #33458, #40320, #30434, #39694, #10761, #658, #36885, #36464, #10130, #7331, #16589, #6900, #13980, #14194, #20480, #19839, #37096, #23309, #4091, #7116, #33247, #16802, #4303, #20270, #33881, #13776, #39486, #447, #3674, #9919, #30001, #17442, #13564, #10338, #1070, #36258, #26755, #26960, #39907, #40116, #3453, #10549, #23526, #6688, #33024, #29791, #14415, #34739, #27609, #7971, #8189, #20906, #5376, #1503, #1719, #14848, #28044, #27393, #34951, #18313, #18527, #41171, #11610, #27825, #1286, #34088, #40959, #31716, #40530, #24818, #37963, #4948, #4511, #31503, #21120, #18095, #17873, #2147, #8617, #8408, #21559, #34309, #34525, #31069, #11830, #14637, #10973, #31290, #4724, #5161, #17654, #24169, #21336, #11402, #24389, #21773, #24596, #30849, #37745, #37530, #25030, #1933, #40749, #38173, #15060, #28258, #11191, #41395, #37316, #7762, #12256, #15700, #2990, #41818, #35161, #42456, #29311, #8826, #12463, #25449, #35798, #5587, #9240, #21983, #19165, #39021, #26078, #6229, #19375, #2779, #32562, #16115, #38595, #9035, #12883, #18740, #22840, #9457, #22200, #39229, #35374, #35587, #32141, #9667, #28480, #42033, #28691, #19580, #31932, #36003, #6437, #2359, #22409, #32764, #15282, #15486, #41611, #6015, #42245, #5801, #18953, #12670, #2571, #28899, #12045, #25241, #22623, #38385, #25656, #38812, #25866, #32354, #15905, #29109, #10714, #398, #610, #7491, #3200, #13309, #6854, #36206, #9875, #13726, #40275, #16758, #16326, #26499, #10084, #6642, #26291, #19792, #39644, #32979, #27132, #20644, #23048, #26915, #13091, #16543, #17186, #23691, #4041, #30171, #36838, #33620, #29525, #33413, #29742, #39858, #42667, #3408, #189, #23260, #40073, #10503, #36420, #20007, #29958, #7282, #33199, #30384, #23909, #816, #3630, #13518, #10292, #26706, #20435, #37054, #39441, #13939, #23479, #36627, #7074, #20223, #3839, #16974, #11354, #37914, #14146, #40912, #34475, #7711, #17827, #40697, #1241, #4897, #27346, #21509, #17607, #11780, #31022, #1025, #38123, #18045, #21074, #11562, #14587, #24770, #24548, #10928, #20860, #37699, #18260, #37261, #8141, #34691, #34044, #27993, #1452, #15012, #17397, #21289, #14365, #31241, #24982, #1883, #8358, #5111, #4255, #27776, #4465, #8568, #30803, #31449, #41344, #24122, #28209, #1668, #33831, #37481, #27563, #30595, #11140, #41122, #24340, #4679, #14797, #40481, #7925, #34263, #12203, #41982, #28427, #22360, #25396, #19315, #32509, #38542, #8776, #29054, #21932, #2313, #2521, #15228, #42403, #8983, #38763, #9189, #35536, #21718, #29260, #12620, #12835, #5965, #19116, #22150, #38333, #41563, #35325, #26025, #34901, #32302, #2723, #12412, #11996, #25813, #15440, #25605, #5753, #39178, #2938, #15856, #42193, #28638, #28847, #18906, #6175, #32087, #5323, #38969, #41771, #9405, #25192, #18477, #15647, #22568, #18685, #16067, #35747, #35111, #31664, #31883, #2098, #5536, #9818, #20376, #23424, #3571, #22999, #10237, #10027, #29902, #6587, #23208, #40020, #36154, #29472, #36788, #23642, #3146, #6801, #19743, #30117, #42614, #16705, #16273, #13462, #33361, #33565, #554, #13674, #39805, #26866, #10450, #32923, #3357, #7225, #13041, #17132, #3781, #16489, #3989, #29688, #340, #26441, #30333, #763, #131, #26236, #13886, #27082, #39385, #19955, #13254, #9611, #39593, #26655, #36366, #36573, #16915, #22785, #35945, #6388, #7019, #19529, #32713, #33143, #20172, #31187, #30546, #5061, #34423, #20805, #1617, #33993, #17774, #14309, #17987, #10659, #24286, #10872, #1832, #974, #14746, #18208, #14092, #27939, #14530, #14960, #1187, #4414, #40225, #27293, #4842, #24065, #11085, #37647, #24494, #40429, #27724, #30754, #30970, #4199, #40860, #27509, #37861, #8306, #40643, #37207, #41068, #7654, #17553, #21021, #33777, #31398, #37431, #11300, #8087, #21237, #23852, #37001, #11513, #7436, #24715, #21451, #7874, #34212, #17343, #4628, #20589, #1400, #34634, #28803, #5711, #34849, #32250, #8730, #18862, #18640, #35698, #9355, #25564, #41935, #21884, #35278, #31834, #12578, #15392, #11731, #32043, #35062, #12366, #5272, #6126, #8940, #2270, #25137, #22525, #28589, #31614, #41720, #38283, #25771, #12157, #28374, #38924, #38716, #22104, #41514, #9149, #25350, #2472, #5490, #38496, #15601, #22317, #5918, #41292, #35490, #11946, #32465, #2047, #2677, #19270, #18424, #19069, #15811, #2890, #29007, #42147, #28158, #15177, #24930, #38074, #8514, #21667, #295, #16228, #3520, #6543, #36322, #22738, #16656, #19697, #14210, #27409, #32880, #3099, #23379, #29427, #39336, #39549, #9564, #37331, #3311, #33092, #29857, #13416, #16020, #24184, #7555, #7778, #26611, #39759, #16440, #32671, #35904, #29639, #20921, #29216, #10194, #36529, #6753, #6341, #20708, #9775, #19907, #82, #34103, #40545, #33896, #4318, #22955, #23159, #13205, #1084, #26398, #42355, #17457, #36109, #30654, #19484, #12788, #9980, #10989, #12992, #25979, #39131, #42568, #26188, #1517, #2161, #18108, #4740, #15295, #18327, #41184, #17886, #5173, #4961, #24831, #14651, #31303, #34966, #31084, #24403, #31731, #18540, #40763, #1735, #27840, #25044, #37544, #11624, #11205, #8421, #28273, #28492, #38186, #8630, #34753, #21786, #5389, #40972, #11415, #41624, #7984, #12058, #41409, #24609, #25254, #37758, #17669, #8202, #21351, #21135, #27623, #34323, #34537, #14861, #38399, #21997, #28058, #11843, #14430, #37977, #8841, #4526, #30863, #31516, #1299, #21572, #1946, #15071, #5813, #29120, #5600, #35389, #9048, #18966, #3001, #32575, #22213, #12268, #19177, #12895, #22421, #19592, #29536, #6450, #9252, #38609, #42256, #2790, #9678, #26303, #42678, #16126, #28704, #25464, #42467, #31944, #9887, #29323, #12681, #39240, #15498, #25878, #35809, #32153, #32366, #42048, #2583, #6241, #41831, #22851, #15712, #13104, #15919, #2372, #39452, #19385, #35599, #26089, #39032, #36013, #9467, #28911, #12474, #22636, #32775, #25669, #3211, #16338, #38823, #35175, #18754, #6027, #6653, #619, #3641, #7292, #14157, #33840, #27141, #827, #16983, #10725, #13948, #10093, #23918, #13735, #20444, #20017, #23271, #33629, #199, #33210, #40284, #40492, #4051, #3419, #37062, #6866, #17195, #33422, #36430, #408, #30605, #20233, #30394, #27357, #23061, #16768, #26716, #13320, #29754, #7501, #17407, #36637, #36849, #10302, #20653, #3848, #4266, #30181, #26509, #39656, #26924, #1034, #29968, #40082, #36217, #13529, #19803, #10513, #32991, #16556, #23700, #39868, #23489, #7083, #21728, #15022, #31459, #4909, #41354, #1893, #40708, #11791, #31251, #37924, #7935, #11151, #8370, #30813, #21085, #28221, #28439, #34701, #34054, #24993, #37491, #21520, #21299, #24350, #31032, #18488, #8151, #5121, #15241, #10938, #34273, #14597, #1252, #17618, #18270, #5333, #24559, #24131, #4688, #17837, #14376, #4476, #27573, #1464, #27787, #34911, #37273, #40921, #38135, #20870, #11364, #8578, #31676, #2110, #7722, #37709, #34487, #18056, #41133, #1679, #14807, #28003, #11573, #24779, #41780, #9416, #38980, #15452, #18699, #25617, #19326, #28858, #26038, #35958, #12846, #15658, #2323, #5977, #9201, #16078, #32724, #6399, #22581, #35123, #31895, #6187, #38344, #16286, #35759, #19128, #2950, #21943, #32313, #42205, #28650, #38775, #5764, #8994, #12631, #5547, #29271, #25407, #19540, #22370, #8786, #3157, #12214, #32521, #15866, #41575, #2533, #22162, #12008, #38553, #42415, #35337, #12423, #39190, #25825, #18917, #29067, #32100, #2736, #41994, #9624, #35547, #22796, #25203, #3584, #16501, #36798, #29699, #10038, #10248, #23011, #7448, #16718, #3793, #16927, #30128, #29484, #37012, #20386, #20601, #565, #13685, #29913, #3368, #36165, #352, #33788, #42624, #26876, #40031, #7031, #6598, #33577, #23220, #20183, #19968, #4211, #10670, #10461, #23652, #36378, #36584, #33154, #13899, #13474, #13054, #33373, #6813, #7236, #19754, #26248, #23436, #26666, #26452, #23864, #39816, #32936, #4000, #39604, #27092, #17143, #145, #40235, #30344, #773, #13266, #39397, #9829, #37656, #14321, #17784, #5070, #1197, #37217, #1843, #31408, #10884, #14540, #27520, #37870, #7664, #11311, #24076, #21247, #41077, #28167, #8315, #21460, #4853, #34644, #18218, #40652, #11094, #14969, #20817, #24939, #11522, #24297, #41302, #37441, #8096, #34222, #11740, #30558, #1410, #30764, #21676, #34003, #38082, #8523, #34859, #17996, #17354, #985, #7884, #21032, #14103, #4424, #27304, #24724, #4638, #40440, #30981, #34433, #27734, #17564, #40870, #24504, #31196, #1626, #14755, #27950, #12795, #38293, #25778, #22324, #22745, #8948, #28597, #5281, #21893, #12585, #31842, #18870, #2684, #32257, #5498, #35499, #38505, #25571, #11955, #5925, #22111, #2897, #16027, #35285, #35071, #38931, #18648, #41728, #28810, #41525, #25988, #5718, #19076, #15819, #29015, #18434, #39139, #9363, #9571, #42154, #22532, #32050, #2279, #25146, #35705, #38723, #19277, #6134, #32473, #29223, #42362, #31623, #2057, #15187, #15400, #41942, #28384, #12165, #25357, #2479, #8739, #15608, #12375, #9156, #19914, #13635, #23166, #20339, #30292, #7185, #9987, #39343, #302, #3527, #10411, #27045, #731, #3745, #29435, #26195, #521, #32678, #10619, #16875, #13422, #39981, #16235, #26618, #36537, #9782, #33103, #90, #3317, #6978, #42577, #23604, #19704, #13849, #16663, #3107, #40190, #20132, #36329, #26827, #29864, #39556, #16449, #35911, #22962, #36748, #32887, #6760, #33320, #30080, #36117, #23387, #26406, #39767, #12998, #33531, #10201, #3954, #17092, #6348, #6550, #19492, #29647, #13212, #4590, #17306, #1795, #40605, #40823, #11264, #24460, #23807, #31363, #14710, #14924, #37607, #8049, #24244, #10833, #24027, #4162, #41033, #36961, #21197, #34384, #1360, #30510, #27901, #4379, #14491, #14269, #28123, #5028, #4800, #17949, #17518, #30925, #27470, #8265, #11049, #7403, #27685, #30718, #31148, #937, #41251, #17730, #37395, #20769, #18169, #7837, #27248, #20985, #33957, #21412, #34171, #37167, #34598, #1580, #11476, #7615, #24677, #37823, #20551, #1145, #33740, #14055, #40389, #31578, #38884, #25734, #5236, #8902, #8694, #32214, #2010, #5669, #18389, #15565, #35450, #22483, #2642, #15773, #41894, #28970, #42109, #21847, #5456, #12543, #15137, #19237, #5876, #35027, #9315, #18606, #32005, #28553, #35659, #24890, #38460, #25102, #15984, #28335, #6090, #32425, #41473, #2850, #28766, #29179, #11693, #38676, #38039, #8481, #21635, #12328, #38249, #18821, #34813, #11907, #31795, #2228, #22278, #9110, #15355, #41685, #22066, #12123, #25315, #35239, #2430, #25527, #19030, #19445, #26362, #29601, #39723, #475, #3701, #3481, #22699, #6301, #260, #39090, #13591, #16617, #39514, #26573, #9529, #9943, #6717, #32637, #16401, #9737, #12953, #19869, #35868, #10158, #29385, #30029, #44, #3063, #42318, #33055, #32843, #13381, #13168, #23340, #23123, #16188, #42528, #36287, #6928, #26148, #29820, #36491, #39299, #20082, #33276, #16830, #25941, #12741, #22918, #36072, #6509, #19658, #3271, #15896, #32134, #25858, #29101, #25233, #39013, #15694, #22402, #35154, #38379, #35579, #15275, #5579, #42238, #12876, #19156, #18521, #12663, #21975, #6008, #5795, #8818, #15480, #2983, #35368, #32347, #42449, #38165, #18732, #41812, #28474, #2140, #2771, #32553, #9028, #8611, #31925, #2353, #41605, #31710, #12038, #28683, #12250, #19367, #21765, #25442, #34943, #9233, #28893, #9450, #22616, #16107, #35790, #38588, #22194, #6222, #5368, #18948, #29303, #42026, #2564, #12456, #25649, #38806, #42660, #10077, #32972, #36198, #39850, #6429, #13717, #9867, #4031, #23253, #35995, #30376, #10284, #13301, #3830, #6846, #16966, #33190, #3193, #13084, #3621, #10495, #29518, #16748, #26907, #26282, #20216, #36412, #7272, #9659, #29950, #6635, #23471, #17178, #36830, #30161, #602, #19999, #40063, #23683, #39434, #20427, #391, #36618, #23040, #19785, #7065, #16319, #3401, #33613, #807, #33404, #19573, #26071, #16536, #39222, #13509, #29734, #179, #22832, #26699, #32756, #26490, #39635, #24114, #17599, #4246, #20634 ) ),
 .UNSPECIFIED., .F., .F., .F. ) 
 B_SPLINE_SURFACE_WITH_KNOTS ( ( 2, 2 ),
 ( 3, 2, 2, 2, 2, 2, 2, 2, 2, 2, 2, 2, 2, 2, 2, 2, 2, 2, 2, 2, 2, 2, 2, 2, 2, 2, 2, 2, 2, 2, 2, 2, 2, 2, 2, 2, 2, 2, 2, 2, 2, 2, 2, 2, 2, 2, 2, 2, 2, 2, 2, 2, 2, 2, 2, 2, 2, 2, 2, 2, 2, 2, 2, 2, 2, 2, 2, 2, 2, 2, 2, 2, 2, 2, 2, 2, 2, 2, 2, 2, 2, 2, 2, 2, 2, 2, 2, 2, 2, 2, 2, 2, 2, 2, 2, 2, 2, 2, 2, 2, 2, 2, 2, 2, 2, 2, 2, 2, 2, 2, 2, 2, 2, 2, 2, 2, 2, 2, 2, 2, 2, 2, 2, 2, 2, 2, 2, 2, 2, 2, 2, 2, 2, 2, 2, 2, 2, 2, 2, 2, 2, 2, 2, 2, 2, 2, 2, 2, 2, 2, 2, 2, 2, 2, 2, 2, 2, 2, 2, 2, 2, 2, 2, 2, 2, 2, 2, 2, 2, 2, 2, 2, 2, 2, 2, 2, 2, 2, 2, 2, 2, 2, 2, 2, 2, 2, 2, 2, 2, 2, 2, 2, 2, 2, 2, 2, 2, 2, 2, 2, 2, 2, 2, 2, 2, 2, 2, 2, 2, 2, 2, 2, 2, 2, 2, 2, 2, 2, 2, 2, 2, 2, 2, 2, 2, 2, 2, 2, 2, 2, 2, 2, 2, 2, 2, 2, 2, 2, 2, 2, 2, 2, 2, 2, 2, 2, 2, 2, 2, 2, 2, 2, 2, 2, 2, 2, 2, 2, 2, 2, 2, 2, 2, 2, 2, 2, 2, 2, 2, 2, 2, 2, 2, 2, 2, 2, 2, 2, 2, 2, 2, 2, 2, 2, 2, 2, 2, 2, 2, 2, 2, 2, 2, 2, 2, 2, 2, 2, 2, 2, 2, 2, 2, 2, 2, 2, 2, 2, 2, 2, 2, 2, 2, 2, 2, 2, 2, 2, 2, 2, 2, 2, 2, 2, 2, 2, 2, 2, 2, 2, 2, 2, 2, 2, 2, 2, 2, 2, 2, 2, 2, 2, 2, 2, 2, 2, 2, 2, 2, 2, 2, 2, 2, 2, 2, 2, 2, 2, 2, 2, 2, 2, 2, 2, 2, 2, 2, 2, 2, 2, 2, 2, 2, 2, 2, 2, 2, 2, 2, 2, 2, 2, 2, 2, 2, 2, 2, 2, 2, 2, 2, 2, 2, 2, 2, 2, 2, 2, 2, 2, 2, 2, 2, 2, 2, 2, 2, 2, 2, 2, 2, 2, 2, 2, 2, 2, 2, 2, 2, 2, 2, 2, 2, 2, 2, 2, 2, 2, 2, 2, 2, 2, 2, 2, 2, 2, 2, 2, 2, 2, 2, 2, 2, 2, 2, 2, 2, 2, 2, 2, 2, 2, 2, 2, 2, 2, 2, 2, 2, 2, 2, 2, 2, 2, 2, 2, 2, 2, 2, 2, 2, 2, 2, 2, 2, 2, 2, 2, 2, 2, 2, 2, 2, 2, 2, 2, 2, 2, 2, 2, 2, 2, 2, 2, 2, 2, 2, 2, 2, 2, 2, 2, 2, 2, 2, 2, 2, 2, 2, 2, 2, 2, 2, 2, 2, 2, 2, 2, 2, 2, 2, 2, 2, 2, 2, 2, 2, 2, 2, 2, 2, 2, 2, 2, 2, 2, 2, 2, 2, 2, 2, 2, 2, 2, 2, 2, 2, 2, 2, 2, 2, 2, 2, 2, 2, 2, 2, 2, 2, 2, 2, 2, 2, 2, 2, 2, 2, 2, 2, 2, 2, 2, 2, 2, 2, 2, 2, 2, 2, 2, 2, 2, 2, 2, 2, 2, 2, 2, 2, 2, 2, 2, 2, 2, 2, 2, 2, 2, 2, 2, 2, 2, 2, 2, 2, 2, 2, 2, 2, 2, 2, 2, 2, 2, 2, 2, 2, 2, 2, 2, 2, 2, 2, 2, 2, 2, 2, 2, 2, 2, 2, 2, 2, 2, 2, 2, 2, 2, 2, 2, 2, 2, 2, 2, 2, 2, 2, 2, 2, 2, 2, 2, 2, 2, 2, 2, 2, 2, 2, 2, 2, 2, 2, 2, 2, 2, 2, 2, 2, 2, 2, 2, 2, 2, 2, 2, 2, 2, 2, 2, 2, 2, 2, 2, 2, 2, 2, 2, 2, 2, 2, 2, 2, 2, 2, 2, 2, 2, 2, 2, 2, 2, 2, 2, 2, 2, 2, 2, 2, 2, 2, 2, 2, 2, 2, 2, 2, 2, 2, 2, 2, 2, 2, 2, 2, 2, 2, 2, 2, 2, 2, 2, 2, 2, 2, 2, 2, 2, 2, 2, 2, 2, 2, 2, 2, 2, 2, 2, 2, 2, 2, 2, 2, 2, 2, 2, 2, 2, 2, 2, 2, 2, 2, 2, 2, 2, 2, 2, 2, 2, 2, 2, 2, 2, 2, 2, 2, 2, 2, 2, 2, 2, 2, 2, 2, 2, 2, 2, 2, 2, 2, 2, 2, 2, 2, 2, 2, 2, 2, 2, 3 ),
 ( 0.000000000000000000, 1.000000000000000000 ),
 ( 0.000000000000000000, 0.001243781094527363160, 0.002487562189054726321, 0.003731343283582089481, 0.004975124378109452641, 0.006218905472636816235, 0.007462686567164178962, 0.008706467661691542556, 0.009950248756218905283, 0.01119402985074626801, 0.01243781094527363247, 0.01368159203980099520, 0.01492537313432835792, 0.01616915422885572065, 0.01741293532338308511, 0.01865671641791044610, 0.01990049751243781057, 0.02114427860696517503, 0.02238805970149253602, 0.02363184079601990048, 0.02487562189054726494, 0.02611940298507462593, 0.02736318407960199039, 0.02860696517412935486, 0.02985074626865671585, 0.03109452736318408031, 0.03233830845771144130, 0.03358208955223880576, 0.03482587064676617022, 0.03606965174129353469, 0.03731343283582089221, 0.03855721393034825667, 0.03980099502487562113, 0.04104477611940298559, 0.04228855721393035005, 0.04353233830845771452, 0.04477611940298507204, 0.04601990049751243650, 0.04726368159203980096, 0.04850746268656716542, 0.04975124378109452988, 0.05099502487562188741, 0.05223880597014925187, 0.05348258706467661633, 0.05472636815920398079, 0.05597014925373134525, 0.05721393034825870971, 0.05845771144278606724, 0.05970149253731343170, 0.06094527363184079616, 0.06218905472636816062, 0.06343283582089552508, 0.06467661691542288260, 0.06592039800995025400, 0.06716417910447761153, 0.06840796019900496905, 0.06965174129353234045, 0.07089552238805969797, 0.07213930348258706937, 0.07338308457711442689, 0.07462686567164178442, 0.07587064676616915582, 0.07711442786069651334, 0.07835820895522388474, 0.07960199004975124226, 0.08084577114427861366, 0.08208955223880597118, 0.08333333333333332871, 0.08457711442786070011, 0.08582089552238805763, 0.08706467661691542903, 0.08830845771144278655, 0.08955223880597014408, 0.09079601990049751548, 0.09203980099502487300, 0.09328358208955224440, 0.09452736318407960192, 0.09577114427860695944, 0.09701492537313433084, 0.09825870646766168837, 0.09950248756218905977, 0.1007462686567164173, 0.1019900497512437748, 0.1032338308457711462, 0.1044776119402985037, 0.1057213930348258751, 0.1069651741293532327, 0.1082089552238805902, 0.1094527363184079616, 0.1106965174129353191, 0.1119402985074626905, 0.1131840796019900480, 0.1144278606965174194, 0.1156716417910447769, 0.1169154228855721345, 0.1181592039800995059, 0.1194029850746268634, 0.1206467661691542348, 0.1218905472636815923, 0.1231343283582089498, 0.1243781094527363212, 0.1256218905472636926, 0.1268656716417910502, 0.1281094527363184077, 0.1293532338308457652, 0.1305970149253731227, 0.1318407960199005080, 0.1330845771144278655, 0.1343283582089552231, 0.1355721393034825806, 0.1368159203980099381, 0.1380597014925373234, 0.1393034825870646809, 0.1405472636815920384, 0.1417910447761193959, 0.1430348258706467535, 0.1442786069651741387, 0.1455223880597014963, 0.1467661691542288538, 0.1480099502487562113, 0.1492537313432835688, 0.1504975124378109541, 0.1517412935323383116, 0.1529850746268656692, 0.1542288557213930267, 0.1554726368159203842, 0.1567164179104477695, 0.1579601990049751270, 0.1592039800995024845, 0.1604477611940298420, 0.1616915422885572273, 0.1629353233830845848, 0.1641791044776119424, 0.1654228855721392999, 0.1666666666666666574, 0.1679104477611940427, 0.1691542288557214002, 0.1703980099502487577, 0.1716417910447761153, 0.1728855721393034728, 0.1741293532338308581, 0.1753731343283582156, 0.1766169154228855731, 0.1778606965174129306, 0.1791044776119402882, 0.1803482587064676734, 0.1815920398009950310, 0.1828358208955223885, 0.1840796019900497460, 0.1853233830845771035, 0.1865671641791044888, 0.1878109452736318463, 0.1890547263681592038, 0.1902985074626865614, 0.1915422885572139189, 0.1927860696517413042, 0.1940298507462686617, 0.1952736318407960192, 0.1965174129353233767, 0.1977611940298507343, 0.1990049751243781195, 0.2002487562189054771, 0.2014925373134328346, 0.2027363184079601921, 0.2039800995024875496, 0.2052238805970149349, 0.2064676616915422924, 0.2077114427860696499, 0.2089552238805970075, 0.2101990049751243650, 0.2114427860696517503, 0.2126865671641791078, 0.2139303482587064653, 0.2151741293532338228, 0.2164179104477611804, 0.2176616915422885656, 0.2189054726368159232, 0.2201492537313432807, 0.2213930348258706382, 0.2226368159203980235, 0.2238805970149253810, 0.2251243781094527385, 0.2263681592039800961, 0.2276119402985074536, 0.2288557213930348389, 0.2300995024875621964, 0.2313432835820895539, 0.2325870646766169114, 0.2338308457711442689, 0.2350746268656716542, 0.2363184079601990117, 0.2375621890547263693, 0.2388059701492537268, 0.2400497512437810843, 0.2412935323383084696, 0.2425373134328358271, 0.2437810945273631846, 0.2450248756218905422, 0.2462686567164178997, 0.2475124378109452850, 0.2487562189054726425, 0.2500000000000000000, 0.2512437810945273853, 0.2524875621890547150, 0.2537313432835821003, 0.2549751243781094301, 0.2562189054726368154, 0.2574626865671642006, 0.2587064676616915304, 0.2599502487562189157, 0.2611940298507462455, 0.2624378109452736307, 0.2636815920398010160, 0.2649253731343283458, 0.2661691542288557311, 0.2674129353233830608, 0.2686567164179104461, 0.2699004975124378314, 0.2711442786069651611, 0.2723880597014925464, 0.2736318407960198762, 0.2748756218905472615, 0.2761194029850746468, 0.2773631840796019765, 0.2786069651741293618, 0.2798507462686566916, 0.2810945273631840768, 0.2823383084577114621, 0.2835820895522387919, 0.2848258706467661772, 0.2860696517412935069, 0.2873134328358208922, 0.2885572139303482775, 0.2898009950248756073, 0.2910447761194029925, 0.2922885572139303223, 0.2935323383084577076, 0.2947761194029850929, 0.2960199004975124226, 0.2972636815920398079, 0.2985074626865671377, 0.2997512437810945229, 0.3009950248756219082, 0.3022388059701492380, 0.3034825870646766233, 0.3047263681592039530, 0.3059701492537313383, 0.3072139303482587236, 0.3084577114427860534, 0.3097014925373134386, 0.3109452736318407684, 0.3121890547263681537, 0.3134328358208955390, 0.3146766169154228687, 0.3159203980099502540, 0.3171641791044776393, 0.3184079601990049690, 0.3196517412935323543, 0.3208955223880596841, 0.3221393034825870694, 0.3233830845771144546, 0.3246268656716417844, 0.3258706467661691697, 0.3271144278606964995, 0.3283582089552238847, 0.3296019900497512700, 0.3308457711442785998, 0.3320895522388059851, 0.3333333333333333148, 0.3345771144278607001, 0.3358208955223880854, 0.3370646766169154152, 0.3383084577114428004, 0.3395522388059701302, 0.3407960199004975155, 0.3420398009950249008, 0.3432835820895522305, 0.3445273631840796158, 0.3457711442786069456, 0.3470149253731343308, 0.3482587064676617161, 0.3495024875621890459, 0.3507462686567164312, 0.3519900497512437609, 0.3532338308457711462, 0.3544776119402985315, 0.3557213930348258613, 0.3569651741293532465, 0.3582089552238805763, 0.3594527363184079616, 0.3606965174129353469, 0.3619402985074626766, 0.3631840796019900619, 0.3644278606965173917, 0.3656716417910447769, 0.3669154228855721622, 0.3681592039800994920, 0.3694029850746268773, 0.3706467661691542070, 0.3718905472636815923, 0.3731343283582089776, 0.3743781094527363074, 0.3756218905472636926, 0.3768656716417910224, 0.3781094527363184077, 0.3793532338308457930, 0.3805970149253731227, 0.3818407960199005080, 0.3830845771144278378, 0.3843283582089552231, 0.3855721393034826083, 0.3868159203980099381, 0.3880597014925373234, 0.3893034825870646531, 0.3905472636815920384, 0.3917910447761194237, 0.3930348258706467535, 0.3942786069651741387, 0.3955223880597014685, 0.3967661691542288538, 0.3980099502487562391, 0.3992537313432835688, 0.4004975124378109541, 0.4017412935323382839, 0.4029850746268656692, 0.4042288557213930544, 0.4054726368159203842, 0.4067164179104477695, 0.4079601990049750992, 0.4092039800995024845, 0.4104477611940298698, 0.4116915422885571996, 0.4129353233830845848, 0.4141791044776119146, 0.4154228855721392999, 0.4166666666666666852, 0.4179104477611940149, 0.4191542288557214002, 0.4203980099502487300, 0.4216417910447761153, 0.4228855721393035005, 0.4241293532338308303, 0.4253731343283582156, 0.4266169154228855454, 0.4278606965174129306, 0.4291044776119403159, 0.4303482587064676457, 0.4315920398009950310, 0.4328358208955223607, 0.4340796019900497460, 0.4353233830845771313, 0.4365671641791044610, 0.4378109452736318463, 0.4390547263681592316, 0.4402985074626865614, 0.4415422885572139466, 0.4427860696517412764, 0.4440298507462686617, 0.4452736318407960470, 0.4465174129353233767, 0.4477611940298507620, 0.4490049751243780918, 0.4502487562189054771, 0.4514925373134328623, 0.4527363184079601921, 0.4539800995024875774, 0.4552238805970149071, 0.4564676616915422924, 0.4577114427860696777, 0.4589552238805970075, 0.4601990049751243927, 0.4614427860696517225, 0.4626865671641791078, 0.4639303482587064931, 0.4651741293532338228, 0.4664179104477612081, 0.4676616915422885379, 0.4689054726368159232, 0.4701492537313433084, 0.4713930348258706382, 0.4726368159203980235, 0.4738805970149253532, 0.4751243781094527385, 0.4763681592039801238, 0.4776119402985074536, 0.4788557213930348389, 0.4800995024875621686, 0.4813432835820895539, 0.4825870646766169392, 0.4838308457711442689, 0.4850746268656716542, 0.4863184079601989840, 0.4875621890547263693, 0.4888059701492537545, 0.4900497512437810843, 0.4912935323383084696, 0.4925373134328357994, 0.4937810945273631846, 0.4950248756218905699, 0.4962686567164178997, 0.4975124378109452850, 0.4987562189054726147, 0.5000000000000000000, 0.5012437810945273853, 0.5024875621890547706, 0.5037313432835820448, 0.5049751243781094301, 0.5062189054726368154, 0.5074626865671642006, 0.5087064676616915859, 0.5099502487562188602, 0.5111940298507462455, 0.5124378109452736307, 0.5136815920398010160, 0.5149253731343284013, 0.5161691542288556755, 0.5174129353233830608, 0.5186567164179104461, 0.5199004975124378314, 0.5211442786069652167, 0.5223880597014924909, 0.5236318407960198762, 0.5248756218905472615, 0.5261194029850746468, 0.5273631840796020320, 0.5286069651741293063, 0.5298507462686566916, 0.5310945273631840768, 0.5323383084577114621, 0.5335820895522388474, 0.5348258706467661217, 0.5360696517412935069, 0.5373134328358208922, 0.5385572139303482775, 0.5398009950248756628, 0.5410447761194029370, 0.5422885572139303223, 0.5435323383084577076, 0.5447761194029850929, 0.5460199004975124781, 0.5472636815920397524, 0.5485074626865671377, 0.5497512437810945229, 0.5509950248756219082, 0.5522388059701492935, 0.5534825870646765678, 0.5547263681592039530, 0.5559701492537313383, 0.5572139303482587236, 0.5584577114427861089, 0.5597014925373133831, 0.5609452736318407684, 0.5621890547263681537, 0.5634328358208955390, 0.5646766169154229242, 0.5659203980099501985, 0.5671641791044775838, 0.5684079601990049690, 0.5696517412935323543, 0.5708955223880597396, 0.5721393034825870139, 0.5733830845771143991, 0.5746268656716417844, 0.5758706467661691697, 0.5771144278606965550, 0.5783582089552238292, 0.5796019900497512145, 0.5808457711442785998, 0.5820895522388059851, 0.5833333333333333703, 0.5845771144278606446, 0.5858208955223880299, 0.5870646766169154152, 0.5883084577114428004, 0.5895522388059701857, 0.5907960199004974600, 0.5920398009950248452, 0.5932835820895522305, 0.5945273631840796158, 0.5957711442786070011, 0.5970149253731342753, 0.5982587064676616606, 0.5995024875621890459, 0.6007462686567164312, 0.6019900497512438164, 0.6032338308457710907, 0.6044776119402984760, 0.6057213930348258613, 0.6069651741293532465, 0.6082089552238806318, 0.6094527363184079061, 0.6106965174129352913, 0.6119402985074626766, 0.6131840796019900619, 0.6144278606965174472, 0.6156716417910447214, 0.6169154228855721067, 0.6181592039800994920, 0.6194029850746268773, 0.6206467661691542625, 0.6218905472636815368, 0.6231343283582089221, 0.6243781094527363074, 0.6256218905472636926, 0.6268656716417910779, 0.6281094527363184632, 0.6293532338308457375, 0.6305970149253731227, 0.6318407960199005080, 0.6330845771144278933, 0.6343283582089552786, 0.6355721393034825528, 0.6368159203980099381, 0.6380597014925373234, 0.6393034825870647087, 0.6405472636815920939, 0.6417910447761193682, 0.6430348258706467535, 0.6442786069651741387, 0.6455223880597015240, 0.6467661691542289093, 0.6480099502487561836, 0.6492537313432835688, 0.6504975124378109541, 0.6517412935323383394, 0.6529850746268657247, 0.6542288557213929989, 0.6554726368159203842, 0.6567164179104477695, 0.6579601990049751548, 0.6592039800995025400, 0.6604477611940298143, 0.6616915422885571996, 0.6629353233830845848, 0.6641791044776119701, 0.6654228855721393554, 0.6666666666666666297, 0.6679104477611940149, 0.6691542288557214002, 0.6703980099502487855, 0.6716417910447761708, 0.6728855721393034450, 0.6741293532338308303, 0.6753731343283582156, 0.6766169154228856009, 0.6778606965174129861, 0.6791044776119402604, 0.6803482587064676457, 0.6815920398009950310, 0.6828358208955224162, 0.6840796019900498015, 0.6853233830845770758, 0.6865671641791044610, 0.6878109452736318463, 0.6890547263681592316, 0.6902985074626866169, 0.6915422885572138911, 0.6927860696517412764, 0.6940298507462686617, 0.6952736318407960470, 0.6965174129353234322, 0.6977611940298507065, 0.6990049751243780918, 0.7002487562189054771, 0.7014925373134328623, 0.7027363184079602476, 0.7039800995024875219, 0.7052238805970149071, 0.7064676616915422924, 0.7077114427860696777, 0.7089552238805970630, 0.7101990049751243372, 0.7114427860696517225, 0.7126865671641791078, 0.7139303482587064931, 0.7151741293532338783, 0.7164179104477611526, 0.7176616915422885379, 0.7189054726368159232, 0.7201492537313433084, 0.7213930348258706937, 0.7226368159203979680, 0.7238805970149253532, 0.7251243781094527385, 0.7263681592039801238, 0.7276119402985075091, 0.7288557213930347833, 0.7300995024875621686, 0.7313432835820895539, 0.7325870646766169392, 0.7338308457711443245, 0.7350746268656715987, 0.7363184079601989840, 0.7375621890547263693, 0.7388059701492537545, 0.7400497512437811398, 0.7412935323383084141, 0.7425373134328357994, 0.7437810945273631846, 0.7450248756218905699, 0.7462686567164179552, 0.7475124378109452294, 0.7487562189054726147, 0.7500000000000000000, 0.7512437810945273853, 0.7524875621890547706, 0.7537313432835820448, 0.7549751243781094301, 0.7562189054726368154, 0.7574626865671642006, 0.7587064676616915859, 0.7599502487562188602, 0.7611940298507462455, 0.7624378109452736307, 0.7636815920398010160, 0.7649253731343284013, 0.7661691542288556755, 0.7674129353233830608, 0.7686567164179104461, 0.7699004975124378314, 0.7711442786069652167, 0.7723880597014924909, 0.7736318407960198762, 0.7748756218905472615, 0.7761194029850746468, 0.7773631840796020320, 0.7786069651741293063, 0.7798507462686566916, 0.7810945273631840768, 0.7823383084577114621, 0.7835820895522388474, 0.7848258706467661217, 0.7860696517412935069, 0.7873134328358208922, 0.7885572139303482775, 0.7898009950248756628, 0.7910447761194029370, 0.7922885572139303223, 0.7935323383084577076, 0.7947761194029850929, 0.7960199004975124781, 0.7972636815920397524, 0.7985074626865671377, 0.7997512437810945229, 0.8009950248756219082, 0.8022388059701492935, 0.8034825870646765678, 0.8047263681592039530, 0.8059701492537313383, 0.8072139303482587236, 0.8084577114427861089, 0.8097014925373133831, 0.8109452736318407684, 0.8121890547263681537, 0.8134328358208955390, 0.8146766169154229242, 0.8159203980099501985, 0.8171641791044775838, 0.8184079601990049690, 0.8196517412935323543, 0.8208955223880597396, 0.8221393034825870139, 0.8233830845771143991, 0.8246268656716417844, 0.8258706467661691697, 0.8271144278606965550, 0.8283582089552238292, 0.8296019900497512145, 0.8308457711442785998, 0.8320895522388059851, 0.8333333333333333703, 0.8345771144278606446, 0.8358208955223880299, 0.8370646766169154152, 0.8383084577114428004, 0.8395522388059701857, 0.8407960199004974600, 0.8420398009950248452, 0.8432835820895522305, 0.8445273631840796158, 0.8457711442786070011, 0.8470149253731342753, 0.8482587064676616606, 0.8495024875621890459, 0.8507462686567164312, 0.8519900497512438164, 0.8532338308457710907, 0.8544776119402984760, 0.8557213930348258613, 0.8569651741293532465, 0.8582089552238806318, 0.8594527363184079061, 0.8606965174129352913, 0.8619402985074626766, 0.8631840796019900619, 0.8644278606965174472, 0.8656716417910447214, 0.8669154228855721067, 0.8681592039800994920, 0.8694029850746268773, 0.8706467661691542625, 0.8718905472636815368, 0.8731343283582089221, 0.8743781094527363074, 0.8756218905472636926, 0.8768656716417910779, 0.8781094527363184632, 0.8793532338308457375, 0.8805970149253731227, 0.8818407960199005080, 0.8830845771144278933, 0.8843283582089552786, 0.8855721393034825528, 0.8868159203980099381, 0.8880597014925373234, 0.8893034825870647087, 0.8905472636815920939, 0.8917910447761193682, 0.8930348258706467535, 0.8942786069651741387, 0.8955223880597015240, 0.8967661691542289093, 0.8980099502487561836, 0.8992537313432835688, 0.9004975124378109541, 0.9017412935323383394, 0.9029850746268657247, 0.9042288557213929989, 0.9054726368159203842, 0.9067164179104477695, 0.9079601990049751548, 0.9092039800995025400, 0.9104477611940298143, 0.9116915422885571996, 0.9129353233830845848, 0.9141791044776119701, 0.9154228855721393554, 0.9166666666666666297, 0.9179104477611940149, 0.9191542288557214002, 0.9203980099502487855, 0.9216417910447761708, 0.9228855721393034450, 0.9241293532338308303, 0.9253731343283582156, 0.9266169154228856009, 0.9278606965174129861, 0.9291044776119402604, 0.9303482587064676457, 0.9315920398009950310, 0.9328358208955224162, 0.9340796019900498015, 0.9353233830845770758, 0.9365671641791044610, 0.9378109452736318463, 0.9390547263681592316, 0.9402985074626866169, 0.9415422885572138911, 0.9427860696517412764, 0.9440298507462686617, 0.9452736318407960470, 0.9465174129353234322, 0.9477611940298507065, 0.9490049751243780918, 0.9502487562189054771, 0.9514925373134328623, 0.9527363184079602476, 0.9539800995024875219, 0.9552238805970149071, 0.9564676616915422924, 0.9577114427860696777, 0.9589552238805970630, 0.9601990049751243372, 0.9614427860696517225, 0.9626865671641791078, 0.9639303482587064931, 0.9651741293532338783, 0.9664179104477611526, 0.9676616915422885379, 0.9689054726368159232, 0.9701492537313433084, 0.9713930348258706937, 0.9726368159203979680, 0.9738805970149253532, 0.9751243781094527385, 0.9763681592039801238, 0.9776119402985075091, 0.9788557213930347833, 0.9800995024875621686, 0.9813432835820895539, 0.9825870646766169392, 0.9838308457711443245, 0.9850746268656715987, 0.9863184079601989840, 0.9875621890547263693, 0.9888059701492537545, 0.9900497512437811398, 0.9912935323383084141, 0.9925373134328357994, 0.9937810945273631846, 0.9950248756218905699 ),
 .UNSPECIFIED. ) 
 GEOMETRIC_REPRESENTATION_ITEM ( )  RATIONAL_B_SPLINE_SURFACE ( (
 ( 1.000000000000000000, 0.8660254037844387076, 1.000000000000000000, 0.8660254037844387076, 1.000000000000000000, 0.8660254037844387076, 1.000000000000000000, 0.8660254037844387076, 1.000000000000000000, 0.8660254037844387076, 1.000000000000000000, 0.8660254037844387076, 1.000000000000000000, 0.8660254037844387076, 1.000000000000000000, 0.8660254037844387076, 1.000000000000000000, 0.8660254037844387076, 1.000000000000000000, 0.8660254037844387076, 1.000000000000000000, 0.8660254037844387076, 1.000000000000000000, 0.8660254037844387076, 1.000000000000000000, 0.8660254037844387076, 1.000000000000000000, 0.8660254037844387076, 1.000000000000000000, 0.8660254037844387076, 1.000000000000000000, 0.8660254037844387076, 1.000000000000000000, 0.8660254037844387076, 1.000000000000000000, 0.8660254037844387076, 1.000000000000000000, 0.8660254037844387076, 1.000000000000000000, 0.8660254037844387076, 1.000000000000000000, 0.8660254037844387076, 1.000000000000000000, 0.8660254037844387076, 1.000000000000000000, 0.8660254037844387076, 1.000000000000000000, 0.8660254037844387076, 1.000000000000000000, 0.8660254037844387076, 1.000000000000000000, 0.8660254037844387076, 1.000000000000000000, 0.8660254037844387076, 1.000000000000000000, 0.8660254037844387076, 1.000000000000000000, 0.8660254037844387076, 1.000000000000000000, 0.8660254037844387076, 1.000000000000000000, 0.8660254037844387076, 1.000000000000000000, 0.8660254037844387076, 1.000000000000000000, 0.8660254037844387076, 1.000000000000000000, 0.8660254037844387076, 1.000000000000000000, 0.8660254037844387076, 1.000000000000000000, 0.8660254037844387076, 1.000000000000000000, 0.8660254037844387076, 1.000000000000000000, 0.8660254037844387076, 1.000000000000000000, 0.8660254037844387076, 1.000000000000000000, 0.8660254037844387076, 1.000000000000000000, 0.8660254037844387076, 1.000000000000000000, 0.8660254037844387076, 1.000000000000000000, 0.8660254037844387076, 1.000000000000000000, 0.8660254037844387076, 1.000000000000000000, 0.8660254037844387076, 1.000000000000000000, 0.8660254037844387076, 1.000000000000000000, 0.8660254037844387076, 1.000000000000000000, 0.8660254037844387076, 1.000000000000000000, 0.8660254037844387076, 1.000000000000000000, 0.8660254037844387076, 1.000000000000000000, 0.8660254037844387076, 1.000000000000000000, 0.8660254037844387076, 1.000000000000000000, 0.8660254037844387076, 1.000000000000000000, 0.8660254037844387076, 1.000000000000000000, 0.8660254037844387076, 1.000000000000000000, 0.8660254037844387076, 1.000000000000000000, 0.8660254037844387076, 1.000000000000000000, 0.8660254037844387076, 1.000000000000000000, 0.8660254037844387076, 1.000000000000000000, 0.8660254037844387076, 1.000000000000000000, 0.8660254037844387076, 1.000000000000000000, 0.8660254037844387076, 1.000000000000000000, 0.8660254037844387076, 1.000000000000000000, 0.8660254037844387076, 1.000000000000000000, 0.8660254037844387076, 1.000000000000000000, 0.8660254037844387076, 1.000000000000000000, 0.8660254037844387076, 1.000000000000000000, 0.8660254037844387076, 1.000000000000000000, 0.8660254037844387076, 1.000000000000000000, 0.8660254037844387076, 1.000000000000000000, 0.8660254037844387076, 1.000000000000000000, 0.8660254037844387076, 1.000000000000000000, 0.8660254037844387076, 1.000000000000000000, 0.8660254037844387076, 1.000000000000000000, 0.8660254037844387076, 1.000000000000000000, 0.8660254037844387076, 1.000000000000000000, 0.8660254037844387076, 1.000000000000000000, 0.8660254037844387076, 1.000000000000000000, 0.8660254037844387076, 1.000000000000000000, 0.8660254037844387076, 1.000000000000000000, 0.8660254037844387076, 1.000000000000000000, 0.8660254037844387076, 1.000000000000000000, 0.8660254037844387076, 1.000000000000000000, 0.8660254037844387076, 1.000000000000000000, 0.8660254037844387076, 1.000000000000000000, 0.8660254037844387076, 1.000000000000000000, 0.8660254037844387076, 1.000000000000000000, 0.8660254037844387076, 1.000000000000000000, 0.8660254037844387076, 1.000000000000000000, 0.8660254037844387076, 1.000000000000000000, 0.8660254037844387076, 1.000000000000000000, 0.8660254037844387076, 1.000000000000000000, 0.8660254037844387076, 1.000000000000000000, 0.8660254037844387076, 1.000000000000000000, 0.8660254037844387076, 1.000000000000000000, 0.8660254037844387076, 1.000000000000000000, 0.8660254037844387076, 1.000000000000000000, 0.8660254037844387076, 1.000000000000000000, 0.8660254037844387076, 1.000000000000000000, 0.8660254037844387076, 1.000000000000000000, 0.8660254037844387076, 1.000000000000000000, 0.8660254037844387076, 1.000000000000000000, 0.8660254037844387076, 1.000000000000000000, 0.8660254037844387076, 1.000000000000000000, 0.8660254037844387076, 1.000000000000000000, 0.8660254037844387076, 1.000000000000000000, 0.8660254037844387076, 1.000000000000000000, 0.8660254037844387076, 1.000000000000000000, 0.8660254037844387076, 1.000000000000000000, 0.8660254037844387076, 1.000000000000000000, 0.8660254037844387076, 1.000000000000000000, 0.8660254037844387076, 1.000000000000000000, 0.8660254037844387076, 1.000000000000000000, 0.8660254037844387076, 1.000000000000000000, 0.8660254037844387076, 1.000000000000000000, 0.8660254037844387076, 1.000000000000000000, 0.8660254037844387076, 1.000000000000000000, 0.8660254037844387076, 1.000000000000000000, 0.8660254037844387076, 1.000000000000000000, 0.8660254037844387076, 1.000000000000000000, 0.8660254037844387076, 1.000000000000000000, 0.8660254037844387076, 1.000000000000000000, 0.8660254037844387076, 1.000000000000000000, 0.8660254037844387076, 1.000000000000000000, 0.8660254037844387076, 1.000000000000000000, 0.8660254037844387076, 1.000000000000000000, 0.8660254037844387076, 1.000000000000000000, 0.8660254037844387076, 1.000000000000000000, 0.8660254037844387076, 1.000000000000000000, 0.8660254037844387076, 1.000000000000000000, 0.8660254037844387076, 1.000000000000000000, 0.8660254037844387076, 1.000000000000000000, 0.8660254037844387076, 1.000000000000000000, 0.8660254037844387076, 1.000000000000000000, 0.8660254037844387076, 1.000000000000000000, 0.8660254037844387076, 1.000000000000000000, 0.8660254037844387076, 1.000000000000000000, 0.8660254037844387076, 1.000000000000000000, 0.8660254037844387076, 1.000000000000000000, 0.8660254037844387076, 1.000000000000000000, 0.8660254037844387076, 1.000000000000000000, 0.8660254037844387076, 1.000000000000000000, 0.8660254037844387076, 1.000000000000000000, 0.8660254037844387076, 1.000000000000000000, 0.8660254037844387076, 1.000000000000000000, 0.8660254037844387076, 1.000000000000000000, 0.8660254037844387076, 1.000000000000000000, 0.8660254037844387076, 1.000000000000000000, 0.8660254037844387076, 1.000000000000000000, 0.8660254037844387076, 1.000000000000000000, 0.8660254037844387076, 1.000000000000000000, 0.8660254037844387076, 1.000000000000000000, 0.8660254037844387076, 1.000000000000000000, 0.8660254037844387076, 1.000000000000000000, 0.8660254037844387076, 1.000000000000000000, 0.8660254037844387076, 1.000000000000000000, 0.8660254037844387076, 1.000000000000000000, 0.8660254037844387076, 1.000000000000000000, 0.8660254037844387076, 1.000000000000000000, 0.8660254037844387076, 1.000000000000000000, 0.8660254037844387076, 1.000000000000000000, 0.8660254037844387076, 1.000000000000000000, 0.8660254037844387076, 1.000000000000000000, 0.8660254037844387076, 1.000000000000000000, 0.8660254037844387076, 1.000000000000000000, 0.8660254037844387076, 1.000000000000000000, 0.8660254037844387076, 1.000000000000000000, 0.8660254037844387076, 1.000000000000000000, 0.8660254037844387076, 1.000000000000000000, 0.8660254037844387076, 1.000000000000000000, 0.8660254037844387076, 1.000000000000000000, 0.8660254037844387076, 1.000000000000000000, 0.8660254037844387076, 1.000000000000000000, 0.8660254037844387076, 1.000000000000000000, 0.8660254037844387076, 1.000000000000000000, 0.8660254037844387076, 1.000000000000000000, 0.8660254037844387076, 1.000000000000000000, 0.8660254037844387076, 1.000000000000000000, 0.8660254037844387076, 1.000000000000000000, 0.8660254037844387076, 1.000000000000000000, 0.8660254037844387076, 1.000000000000000000, 0.8660254037844387076, 1.000000000000000000, 0.8660254037844387076, 1.000000000000000000, 0.8660254037844387076, 1.000000000000000000, 0.8660254037844387076, 1.000000000000000000, 0.8660254037844387076, 1.000000000000000000, 0.8660254037844387076, 1.000000000000000000, 0.8660254037844387076, 1.000000000000000000, 0.8660254037844387076, 1.000000000000000000, 0.8660254037844387076, 1.000000000000000000, 0.8660254037844387076, 1.000000000000000000, 0.8660254037844387076, 1.000000000000000000, 0.8660254037844387076, 1.000000000000000000, 0.8660254037844387076, 1.000000000000000000, 0.8660254037844387076, 1.000000000000000000, 0.8660254037844387076, 1.000000000000000000, 0.8660254037844387076, 1.000000000000000000, 0.8660254037844387076, 1.000000000000000000, 0.8660254037844387076, 1.000000000000000000, 0.8660254037844387076, 1.000000000000000000, 0.8660254037844387076, 1.000000000000000000, 0.8660254037844387076, 1.000000000000000000, 0.8660254037844387076, 1.000000000000000000, 0.8660254037844387076, 1.000000000000000000, 0.8660254037844387076, 1.000000000000000000, 0.8660254037844387076, 1.000000000000000000, 0.8660254037844387076, 1.000000000000000000, 0.8660254037844387076, 1.000000000000000000, 0.8660254037844387076, 1.000000000000000000, 0.8660254037844387076, 1.000000000000000000, 0.8660254037844387076, 1.000000000000000000, 0.8660254037844387076, 1.000000000000000000, 0.8660254037844387076, 1.000000000000000000, 0.8660254037844387076, 1.000000000000000000, 0.8660254037844387076, 1.000000000000000000, 0.8660254037844387076, 1.000000000000000000, 0.8660254037844387076, 1.000000000000000000, 0.8660254037844387076, 1.000000000000000000, 0.8660254037844387076, 1.000000000000000000, 0.8660254037844387076, 1.000000000000000000, 0.8660254037844387076, 1.000000000000000000, 0.8660254037844387076, 1.000000000000000000, 0.8660254037844387076, 1.000000000000000000, 0.8660254037844387076, 1.000000000000000000, 0.8660254037844387076, 1.000000000000000000, 0.8660254037844387076, 1.000000000000000000, 0.8660254037844387076, 1.000000000000000000, 0.8660254037844387076, 1.000000000000000000, 0.8660254037844387076, 1.000000000000000000, 0.8660254037844387076, 1.000000000000000000, 0.8660254037844387076, 1.000000000000000000, 0.8660254037844387076, 1.000000000000000000, 0.8660254037844387076, 1.000000000000000000, 0.8660254037844387076, 1.000000000000000000, 0.8660254037844387076, 1.000000000000000000, 0.8660254037844387076, 1.000000000000000000, 0.8660254037844387076, 1.000000000000000000, 0.8660254037844387076, 1.000000000000000000, 0.8660254037844387076, 1.000000000000000000, 0.8660254037844387076, 1.000000000000000000, 0.8660254037844387076, 1.000000000000000000, 0.8660254037844387076, 1.000000000000000000, 0.8660254037844387076, 1.000000000000000000, 0.8660254037844387076, 1.000000000000000000, 0.8660254037844387076, 1.000000000000000000, 0.8660254037844387076, 1.000000000000000000, 0.8660254037844387076, 1.000000000000000000, 0.8660254037844387076, 1.000000000000000000, 0.8660254037844387076, 1.000000000000000000, 0.8660254037844387076, 1.000000000000000000, 0.8660254037844387076, 1.000000000000000000, 0.8660254037844387076, 1.000000000000000000, 0.8660254037844387076, 1.000000000000000000, 0.8660254037844387076, 1.000000000000000000, 0.8660254037844387076, 1.000000000000000000, 0.8660254037844387076, 1.000000000000000000, 0.8660254037844387076, 1.000000000000000000, 0.8660254037844387076, 1.000000000000000000, 0.8660254037844387076, 1.000000000000000000, 0.8660254037844387076, 1.000000000000000000, 0.8660254037844387076, 1.000000000000000000, 0.8660254037844387076, 1.000000000000000000, 0.8660254037844387076, 1.000000000000000000, 0.8660254037844387076, 1.000000000000000000, 0.8660254037844387076, 1.000000000000000000, 0.8660254037844387076, 1.000000000000000000, 0.8660254037844387076, 1.000000000000000000, 0.8660254037844387076, 1.000000000000000000, 0.8660254037844387076, 1.000000000000000000, 0.8660254037844387076, 1.000000000000000000, 0.8660254037844387076, 1.000000000000000000, 0.8660254037844387076, 1.000000000000000000, 0.8660254037844387076, 1.000000000000000000, 0.8660254037844387076, 1.000000000000000000, 0.8660254037844387076, 1.000000000000000000, 0.8660254037844387076, 1.000000000000000000, 0.8660254037844387076, 1.000000000000000000, 0.8660254037844387076, 1.000000000000000000, 0.8660254037844387076, 1.000000000000000000, 0.8660254037844387076, 1.000000000000000000, 0.8660254037844387076, 1.000000000000000000, 0.8660254037844387076, 1.000000000000000000, 0.8660254037844387076, 1.000000000000000000, 0.8660254037844387076, 1.000000000000000000, 0.8660254037844387076, 1.000000000000000000, 0.8660254037844387076, 1.000000000000000000, 0.8660254037844387076, 1.000000000000000000, 0.8660254037844387076, 1.000000000000000000, 0.8660254037844387076, 1.000000000000000000, 0.8660254037844387076, 1.000000000000000000, 0.8660254037844387076, 1.000000000000000000, 0.8660254037844387076, 1.000000000000000000, 0.8660254037844387076, 1.000000000000000000, 0.8660254037844387076, 1.000000000000000000, 0.8660254037844387076, 1.000000000000000000, 0.8660254037844387076, 1.000000000000000000, 0.8660254037844387076, 1.000000000000000000, 0.8660254037844387076, 1.000000000000000000, 0.8660254037844387076, 1.000000000000000000, 0.8660254037844387076, 1.000000000000000000, 0.8660254037844387076, 1.000000000000000000, 0.8660254037844387076, 1.000000000000000000, 0.8660254037844387076, 1.000000000000000000, 0.8660254037844387076, 1.000000000000000000, 0.8660254037844387076, 1.000000000000000000, 0.8660254037844387076, 1.000000000000000000, 0.8660254037844387076, 1.000000000000000000, 0.8660254037844387076, 1.000000000000000000, 0.8660254037844387076, 1.000000000000000000, 0.8660254037844387076, 1.000000000000000000, 0.8660254037844387076, 1.000000000000000000, 0.8660254037844387076, 1.000000000000000000, 0.8660254037844387076, 1.000000000000000000, 0.8660254037844387076, 1.000000000000000000, 0.8660254037844387076, 1.000000000000000000, 0.8660254037844387076, 1.000000000000000000, 0.8660254037844387076, 1.000000000000000000, 0.8660254037844387076, 1.000000000000000000, 0.8660254037844387076, 1.000000000000000000, 0.8660254037844387076, 1.000000000000000000, 0.8660254037844387076, 1.000000000000000000, 0.8660254037844387076, 1.000000000000000000, 0.8660254037844387076, 1.000000000000000000, 0.8660254037844387076, 1.000000000000000000, 0.8660254037844387076, 1.000000000000000000, 0.8660254037844387076, 1.000000000000000000, 0.8660254037844387076, 1.000000000000000000, 0.8660254037844387076, 1.000000000000000000, 0.8660254037844387076, 1.000000000000000000, 0.8660254037844387076, 1.000000000000000000, 0.8660254037844387076, 1.000000000000000000, 0.8660254037844387076, 1.000000000000000000, 0.8660254037844387076, 1.000000000000000000, 0.8660254037844387076, 1.000000000000000000, 0.8660254037844387076, 1.000000000000000000, 0.8660254037844387076, 1.000000000000000000, 0.8660254037844387076, 1.000000000000000000, 0.8660254037844387076, 1.000000000000000000, 0.8660254037844387076, 1.000000000000000000, 0.8660254037844387076, 1.000000000000000000, 0.8660254037844387076, 1.000000000000000000, 0.8660254037844387076, 1.000000000000000000, 0.8660254037844387076, 1.000000000000000000, 0.8660254037844387076, 1.000000000000000000, 0.8660254037844387076, 1.000000000000000000, 0.8660254037844387076, 1.000000000000000000, 0.8660254037844387076, 1.000000000000000000, 0.8660254037844387076, 1.000000000000000000, 0.8660254037844387076, 1.000000000000000000, 0.8660254037844387076, 1.000000000000000000, 0.8660254037844387076, 1.000000000000000000, 0.8660254037844387076, 1.000000000000000000, 0.8660254037844387076, 1.000000000000000000, 0.8660254037844387076, 1.000000000000000000, 0.8660254037844387076, 1.000000000000000000, 0.8660254037844387076, 1.000000000000000000, 0.8660254037844387076, 1.000000000000000000, 0.8660254037844387076, 1.000000000000000000, 0.8660254037844387076, 1.000000000000000000, 0.8660254037844387076, 1.000000000000000000, 0.8660254037844387076, 1.000000000000000000, 0.8660254037844387076, 1.000000000000000000, 0.8660254037844387076, 1.000000000000000000, 0.8660254037844387076, 1.000000000000000000, 0.8660254037844387076, 1.000000000000000000, 0.8660254037844387076, 1.000000000000000000, 0.8660254037844387076, 1.000000000000000000, 0.8660254037844387076, 1.000000000000000000, 0.8660254037844387076, 1.000000000000000000, 0.8660254037844387076, 1.000000000000000000, 0.8660254037844387076, 1.000000000000000000, 0.8660254037844387076, 1.000000000000000000, 0.8660254037844387076, 1.000000000000000000, 0.8660254037844387076, 1.000000000000000000, 0.8660254037844387076, 1.000000000000000000, 0.8660254037844387076, 1.000000000000000000, 0.8660254037844387076, 1.000000000000000000, 0.8660254037844387076, 1.000000000000000000, 0.8660254037844387076, 1.000000000000000000, 0.8660254037844387076, 1.000000000000000000, 0.8660254037844387076, 1.000000000000000000, 0.8660254037844387076, 1.000000000000000000, 0.8660254037844387076, 1.000000000000000000, 0.8660254037844387076, 1.000000000000000000, 0.8660254037844387076, 1.000000000000000000, 0.8660254037844387076, 1.000000000000000000, 0.8660254037844387076, 1.000000000000000000, 0.8660254037844387076, 1.000000000000000000, 0.8660254037844387076, 1.000000000000000000, 0.8660254037844387076, 1.000000000000000000, 0.8660254037844387076, 1.000000000000000000, 0.8660254037844387076, 1.000000000000000000, 0.8660254037844387076, 1.000000000000000000, 0.8660254037844387076, 1.000000000000000000, 0.8660254037844387076, 1.000000000000000000, 0.8660254037844387076, 1.000000000000000000, 0.8660254037844387076, 1.000000000000000000, 0.8660254037844387076, 1.000000000000000000, 0.8660254037844387076, 1.000000000000000000, 0.8660254037844387076, 1.000000000000000000, 0.8660254037844387076, 1.000000000000000000, 0.8660254037844387076, 1.000000000000000000, 0.8660254037844387076, 1.000000000000000000, 0.8660254037844387076, 1.000000000000000000, 0.8660254037844387076, 1.000000000000000000, 0.8660254037844387076, 1.000000000000000000, 0.8660254037844387076, 1.000000000000000000, 0.8660254037844387076, 1.000000000000000000, 0.8660254037844387076, 1.000000000000000000, 0.8660254037844387076, 1.000000000000000000, 0.8660254037844387076, 1.000000000000000000, 0.8660254037844387076, 1.000000000000000000, 0.8660254037844387076, 1.000000000000000000, 0.8660254037844387076, 1.000000000000000000, 0.8660254037844387076, 1.000000000000000000, 0.8660254037844387076, 1.000000000000000000, 0.8660254037844387076, 1.000000000000000000, 0.8660254037844387076, 1.000000000000000000, 0.8660254037844387076, 1.000000000000000000, 0.8660254037844387076, 1.000000000000000000, 0.8660254037844387076, 1.000000000000000000, 0.8660254037844387076, 1.000000000000000000, 0.8660254037844387076, 1.000000000000000000, 0.8660254037844387076, 1.000000000000000000, 0.8660254037844387076, 1.000000000000000000, 0.8660254037844387076, 1.000000000000000000, 0.8660254037844387076, 1.000000000000000000, 0.8660254037844387076, 1.000000000000000000, 0.8660254037844387076, 1.000000000000000000, 0.8660254037844387076, 1.000000000000000000, 0.8660254037844387076, 1.000000000000000000, 0.8660254037844387076, 1.000000000000000000, 0.8660254037844387076, 1.000000000000000000, 0.8660254037844387076, 1.000000000000000000, 0.8660254037844387076, 1.000000000000000000, 0.8660254037844387076, 1.000000000000000000, 0.8660254037844387076, 1.000000000000000000, 0.8660254037844387076, 1.000000000000000000, 0.8660254037844387076, 1.000000000000000000, 0.8660254037844387076, 1.000000000000000000, 0.8660254037844387076, 1.000000000000000000, 0.8660254037844387076, 1.000000000000000000, 0.8660254037844387076, 1.000000000000000000, 0.8660254037844387076, 1.000000000000000000, 0.8660254037844387076, 1.000000000000000000, 0.8660254037844387076, 1.000000000000000000, 0.8660254037844387076, 1.000000000000000000, 0.8660254037844387076, 1.000000000000000000, 0.8660254037844387076, 1.000000000000000000, 0.8660254037844387076, 1.000000000000000000, 0.8660254037844387076, 1.000000000000000000, 0.8660254037844387076, 1.000000000000000000, 0.8660254037844387076, 1.000000000000000000, 0.8660254037844387076, 1.000000000000000000, 0.8660254037844387076, 1.000000000000000000, 0.8660254037844387076, 1.000000000000000000, 0.8660254037844387076, 1.000000000000000000, 0.8660254037844387076, 1.000000000000000000, 0.8660254037844387076, 1.000000000000000000, 0.8660254037844387076, 1.000000000000000000, 0.8660254037844387076, 1.000000000000000000, 0.8660254037844387076, 1.000000000000000000, 0.8660254037844387076, 1.000000000000000000, 0.8660254037844387076, 1.000000000000000000, 0.8660254037844387076, 1.000000000000000000, 0.8660254037844387076, 1.000000000000000000, 0.8660254037844387076, 1.000000000000000000, 0.8660254037844387076, 1.000000000000000000, 0.8660254037844387076, 1.000000000000000000, 0.8660254037844387076, 1.000000000000000000, 0.8660254037844387076, 1.000000000000000000, 0.8660254037844387076, 1.000000000000000000, 0.8660254037844387076, 1.000000000000000000, 0.8660254037844387076, 1.000000000000000000, 0.8660254037844387076, 1.000000000000000000, 0.8660254037844387076, 1.000000000000000000, 0.8660254037844387076, 1.000000000000000000, 0.8660254037844387076, 1.000000000000000000, 0.8660254037844387076, 1.000000000000000000, 0.8660254037844387076, 1.000000000000000000, 0.8660254037844387076, 1.000000000000000000, 0.8660254037844387076, 1.000000000000000000, 0.8660254037844387076, 1.000000000000000000, 0.8660254037844387076, 1.000000000000000000, 0.8660254037844387076, 1.000000000000000000, 0.8660254037844387076, 1.000000000000000000, 0.8660254037844387076, 1.000000000000000000, 0.8660254037844387076, 1.000000000000000000, 0.8660254037844387076, 1.000000000000000000, 0.8660254037844387076, 1.000000000000000000, 0.8660254037844387076, 1.000000000000000000, 0.8660254037844387076, 1.000000000000000000, 0.8660254037844387076, 1.000000000000000000, 0.8660254037844387076, 1.000000000000000000, 0.8660254037844387076, 1.000000000000000000, 0.8660254037844387076, 1.000000000000000000, 0.8660254037844387076, 1.000000000000000000, 0.8660254037844387076, 1.000000000000000000, 0.8660254037844387076, 1.000000000000000000, 0.8660254037844387076, 1.000000000000000000, 0.8660254037844387076, 1.000000000000000000, 0.8660254037844387076, 1.000000000000000000, 0.8660254037844387076, 1.000000000000000000, 0.8660254037844387076, 1.000000000000000000, 0.8660254037844387076, 1.000000000000000000, 0.8660254037844387076, 1.000000000000000000, 0.8660254037844387076, 1.000000000000000000, 0.8660254037844387076, 1.000000000000000000, 0.8660254037844387076, 1.000000000000000000, 0.8660254037844387076, 1.000000000000000000, 0.8660254037844387076, 1.000000000000000000, 0.8660254037844387076, 1.000000000000000000, 0.8660254037844387076, 1.000000000000000000, 0.8660254037844387076, 1.000000000000000000, 0.8660254037844387076, 1.000000000000000000, 0.8660254037844387076, 1.000000000000000000, 0.8660254037844387076, 1.000000000000000000, 0.8660254037844387076, 1.000000000000000000, 0.8660254037844387076, 1.000000000000000000, 0.8660254037844387076, 1.000000000000000000, 0.8660254037844387076, 1.000000000000000000, 0.8660254037844387076, 1.000000000000000000, 0.8660254037844387076, 1.000000000000000000, 0.8660254037844387076, 1.000000000000000000, 0.8660254037844387076, 1.000000000000000000, 0.8660254037844387076, 1.000000000000000000, 0.8660254037844387076, 1.000000000000000000, 0.8660254037844387076, 1.000000000000000000, 0.8660254037844387076, 1.000000000000000000, 0.8660254037844387076, 1.000000000000000000, 0.8660254037844387076, 1.000000000000000000, 0.8660254037844387076, 1.000000000000000000, 0.8660254037844387076, 1.000000000000000000, 0.8660254037844387076, 1.000000000000000000, 0.8660254037844387076, 1.000000000000000000, 0.8660254037844387076, 1.000000000000000000, 0.8660254037844387076, 1.000000000000000000, 0.8660254037844387076, 1.000000000000000000, 0.8660254037844387076, 1.000000000000000000, 0.8660254037844387076, 1.000000000000000000, 0.8660254037844387076, 1.000000000000000000, 0.8660254037844387076, 1.000000000000000000, 0.8660254037844387076, 1.000000000000000000, 0.8660254037844387076, 1.000000000000000000, 0.8660254037844387076, 1.000000000000000000, 0.8660254037844387076, 1.000000000000000000, 0.8660254037844387076, 1.000000000000000000, 0.8660254037844387076, 1.000000000000000000, 0.8660254037844387076, 1.000000000000000000, 0.8660254037844387076, 1.000000000000000000, 0.8660254037844387076, 1.000000000000000000, 0.8660254037844387076, 1.000000000000000000, 0.8660254037844387076, 1.000000000000000000, 0.8660254037844387076, 1.000000000000000000, 0.8660254037844387076, 1.000000000000000000, 0.8660254037844387076, 1.000000000000000000, 0.8660254037844387076, 1.000000000000000000, 0.8660254037844387076, 1.000000000000000000, 0.8660254037844387076, 1.000000000000000000, 0.8660254037844387076, 1.000000000000000000, 0.8660254037844387076, 1.000000000000000000, 0.8660254037844387076, 1.000000000000000000, 0.8660254037844387076, 1.000000000000000000, 0.8660254037844387076, 1.000000000000000000, 0.8660254037844387076, 1.000000000000000000, 0.8660254037844387076, 1.000000000000000000, 0.8660254037844387076, 1.000000000000000000, 0.8660254037844387076, 1.000000000000000000, 0.8660254037844387076, 1.000000000000000000, 0.8660254037844387076, 1.000000000000000000, 0.8660254037844387076, 1.000000000000000000, 0.8660254037844387076, 1.000000000000000000, 0.8660254037844387076, 1.000000000000000000, 0.8660254037844387076, 1.000000000000000000, 0.8660254037844387076, 1.000000000000000000, 0.8660254037844387076, 1.000000000000000000, 0.8660254037844387076, 1.000000000000000000, 0.8660254037844387076, 1.000000000000000000, 0.8660254037844387076, 1.000000000000000000, 0.8660254037844387076, 1.000000000000000000, 0.8660254037844387076, 1.000000000000000000, 0.8660254037844387076, 1.000000000000000000, 0.8660254037844387076, 1.000000000000000000, 0.8660254037844387076, 1.000000000000000000, 0.8660254037844387076, 1.000000000000000000, 0.8660254037844387076, 1.000000000000000000, 0.8660254037844387076, 1.000000000000000000, 0.8660254037844387076, 1.000000000000000000, 0.8660254037844387076, 1.000000000000000000, 0.8660254037844387076, 1.000000000000000000, 0.8660254037844387076, 1.000000000000000000, 0.8660254037844387076, 1.000000000000000000, 0.8660254037844387076, 1.000000000000000000, 0.8660254037844387076, 1.000000000000000000, 0.8660254037844387076, 1.000000000000000000, 0.8660254037844387076, 1.000000000000000000, 0.8660254037844387076, 1.000000000000000000, 0.8660254037844387076, 1.000000000000000000, 0.8660254037844387076, 1.000000000000000000, 0.8660254037844387076, 1.000000000000000000, 0.8660254037844387076, 1.000000000000000000, 0.8660254037844387076, 1.000000000000000000, 0.8660254037844387076, 1.000000000000000000, 0.8660254037844387076, 1.000000000000000000, 0.8660254037844387076, 1.000000000000000000, 0.8660254037844387076, 1.000000000000000000, 0.8660254037844387076, 1.000000000000000000, 0.8660254037844387076, 1.000000000000000000, 0.8660254037844387076, 1.000000000000000000, 0.8660254037844387076, 1.000000000000000000, 0.8660254037844387076, 1.000000000000000000, 0.8660254037844387076, 1.000000000000000000, 0.8660254037844387076, 1.000000000000000000, 0.8660254037844387076, 1.000000000000000000, 0.8660254037844387076, 1.000000000000000000, 0.8660254037844387076, 1.000000000000000000, 0.8660254037844387076, 1.000000000000000000, 0.8660254037844387076, 1.000000000000000000, 0.8660254037844387076, 1.000000000000000000, 0.8660254037844387076, 1.000000000000000000, 0.8660254037844387076, 1.000000000000000000, 0.8660254037844387076, 1.000000000000000000, 0.8660254037844387076, 1.000000000000000000, 0.8660254037844387076, 1.000000000000000000, 0.8660254037844387076, 1.000000000000000000, 0.8660254037844387076, 1.000000000000000000, 0.8660254037844387076, 1.000000000000000000, 0.8660254037844387076, 1.000000000000000000, 0.8660254037844387076, 1.000000000000000000, 0.8660254037844387076, 1.000000000000000000, 0.8660254037844387076, 1.000000000000000000, 0.8660254037844387076, 1.000000000000000000, 0.8660254037844387076, 1.000000000000000000, 0.8660254037844387076, 1.000000000000000000, 0.8660254037844387076, 1.000000000000000000, 0.8660254037844387076, 1.000000000000000000, 0.8660254037844387076, 1.000000000000000000, 0.8660254037844387076, 1.000000000000000000, 0.8660254037844387076, 1.000000000000000000, 0.8660254037844387076, 1.000000000000000000, 0.8660254037844387076, 1.000000000000000000, 0.8660254037844387076, 1.000000000000000000, 0.8660254037844387076, 1.000000000000000000, 0.8660254037844387076, 1.000000000000000000, 0.8660254037844387076, 1.000000000000000000, 0.8660254037844387076, 1.000000000000000000, 0.8660254037844387076, 1.000000000000000000, 0.8660254037844387076, 1.000000000000000000, 0.8660254037844387076, 1.000000000000000000, 0.8660254037844387076, 1.000000000000000000, 0.8660254037844387076, 1.000000000000000000, 0.8660254037844387076, 1.000000000000000000, 0.8660254037844387076, 1.000000000000000000, 0.8660254037844387076, 1.000000000000000000, 0.8660254037844387076, 1.000000000000000000, 0.8660254037844387076, 1.000000000000000000, 0.8660254037844387076, 1.000000000000000000, 0.8660254037844387076, 1.000000000000000000, 0.8660254037844387076, 1.000000000000000000, 0.8660254037844387076, 1.000000000000000000, 0.8660254037844387076, 1.000000000000000000, 0.8660254037844387076, 1.000000000000000000, 0.8660254037844387076, 1.000000000000000000, 0.8660254037844387076, 1.000000000000000000, 0.8660254037844387076, 1.000000000000000000, 0.8660254037844387076, 1.000000000000000000, 0.8660254037844387076, 1.000000000000000000, 0.8660254037844387076, 1.000000000000000000, 0.8660254037844387076, 1.000000000000000000, 0.8660254037844387076, 1.000000000000000000, 0.8660254037844387076, 1.000000000000000000, 0.8660254037844387076, 1.000000000000000000, 0.8660254037844387076, 1.000000000000000000, 0.8660254037844387076, 1.000000000000000000, 0.8660254037844387076, 1.000000000000000000, 0.8660254037844387076, 1.000000000000000000, 0.8660254037844387076, 1.000000000000000000, 0.8660254037844387076, 1.000000000000000000, 0.8660254037844387076, 1.000000000000000000, 0.8660254037844387076, 1.000000000000000000, 0.8660254037844387076, 1.000000000000000000, 0.8660254037844387076, 1.000000000000000000, 0.8660254037844387076, 1.000000000000000000, 0.8660254037844387076, 1.000000000000000000, 0.8660254037844387076, 1.000000000000000000, 0.8660254037844387076, 1.000000000000000000, 0.8660254037844387076, 1.000000000000000000, 0.8660254037844387076, 1.000000000000000000, 0.8660254037844387076, 1.000000000000000000, 0.8660254037844387076, 1.000000000000000000, 0.8660254037844387076, 1.000000000000000000, 0.8660254037844387076, 1.000000000000000000, 0.8660254037844387076, 1.000000000000000000, 0.8660254037844387076, 1.000000000000000000, 0.8660254037844387076, 1.000000000000000000, 0.8660254037844387076, 1.000000000000000000, 0.8660254037844387076, 1.000000000000000000, 0.8660254037844387076, 1.000000000000000000, 0.8660254037844387076, 1.000000000000000000, 0.8660254037844387076, 1.000000000000000000, 0.8660254037844387076, 1.000000000000000000, 0.8660254037844387076, 1.000000000000000000, 0.8660254037844387076, 1.000000000000000000, 0.8660254037844387076, 1.000000000000000000, 0.8660254037844387076, 1.000000000000000000, 0.8660254037844387076, 1.000000000000000000, 0.8660254037844387076, 1.000000000000000000, 0.8660254037844387076, 1.000000000000000000, 0.8660254037844387076, 1.000000000000000000, 0.8660254037844387076, 1.000000000000000000, 0.8660254037844387076, 1.000000000000000000, 0.8660254037844387076, 1.000000000000000000, 0.8660254037844387076, 1.000000000000000000, 0.8660254037844387076, 1.000000000000000000, 0.8660254037844387076, 1.000000000000000000, 0.8660254037844387076, 1.000000000000000000, 0.8660254037844387076, 1.000000000000000000, 0.8660254037844387076, 1.000000000000000000, 0.8660254037844387076, 1.000000000000000000, 0.8660254037844387076, 1.000000000000000000, 0.8660254037844387076, 1.000000000000000000, 0.8660254037844387076, 1.000000000000000000, 0.8660254037844387076, 1.000000000000000000, 0.8660254037844387076, 1.000000000000000000, 0.8660254037844387076, 1.000000000000000000, 0.8660254037844387076, 1.000000000000000000, 0.8660254037844387076, 1.000000000000000000, 0.8660254037844387076, 1.000000000000000000, 0.8660254037844387076, 1.000000000000000000, 0.8660254037844387076, 1.000000000000000000, 0.8660254037844387076, 1.000000000000000000, 0.8660254037844387076, 1.000000000000000000, 0.8660254037844387076, 1.000000000000000000, 0.8660254037844387076, 1.000000000000000000, 0.8660254037844387076, 1.000000000000000000, 0.8660254037844387076, 1.000000000000000000, 0.8660254037844387076, 1.000000000000000000, 0.8660254037844387076, 1.000000000000000000, 0.8660254037844387076, 1.000000000000000000, 0.8660254037844387076, 1.000000000000000000, 0.8660254037844387076, 1.000000000000000000, 0.8660254037844387076, 1.000000000000000000, 0.8660254037844387076, 1.000000000000000000, 0.8660254037844387076, 1.000000000000000000, 0.8660254037844387076, 1.000000000000000000, 0.8660254037844387076, 1.000000000000000000, 0.8660254037844387076, 1.000000000000000000, 0.8660254037844387076, 1.000000000000000000, 0.8660254037844387076, 1.000000000000000000, 0.8660254037844387076, 1.000000000000000000, 0.8660254037844387076, 1.000000000000000000, 0.8660254037844387076, 1.000000000000000000, 0.8660254037844387076, 1.000000000000000000, 0.8660254037844387076, 1.000000000000000000, 0.8660254037844387076, 1.000000000000000000, 0.8660254037844387076, 1.000000000000000000, 0.8660254037844387076, 1.000000000000000000, 0.8660254037844387076, 1.000000000000000000, 0.8660254037844387076, 1.000000000000000000, 0.8660254037844387076, 1.000000000000000000, 0.8660254037844387076, 1.000000000000000000, 0.8660254037844387076, 1.000000000000000000, 0.8660254037844387076, 1.000000000000000000, 0.8660254037844387076, 1.000000000000000000, 0.8660254037844387076, 1.000000000000000000, 0.8660254037844387076, 1.000000000000000000, 0.8660254037844387076, 1.000000000000000000, 0.8660254037844387076, 1.000000000000000000, 0.8660254037844387076, 1.000000000000000000, 0.8660254037844387076, 1.000000000000000000, 0.8660254037844387076, 1.000000000000000000, 0.8660254037844387076, 1.000000000000000000, 0.8660254037844387076, 1.000000000000000000, 0.8660254037844387076, 1.000000000000000000, 0.8660254037844387076, 1.000000000000000000, 0.8660254037844387076, 1.000000000000000000, 0.8660254037844387076, 1.000000000000000000, 0.8660254037844387076, 1.000000000000000000, 0.8660254037844387076, 1.000000000000000000, 0.8660254037844387076, 1.000000000000000000, 0.8660254037844387076, 1.000000000000000000, 0.8660254037844387076, 1.000000000000000000, 0.8660254037844387076, 1.000000000000000000, 0.8660254037844387076, 1.000000000000000000, 0.8660254037844387076, 1.000000000000000000, 0.8660254037844387076, 1.000000000000000000, 0.8660254037844387076, 1.000000000000000000, 0.8660254037844387076, 1.000000000000000000, 0.8660254037844387076, 1.000000000000000000, 0.8660254037844387076, 1.000000000000000000, 0.8660254037844387076, 1.000000000000000000, 0.8660254037844387076, 1.000000000000000000, 0.8660254037844387076, 1.000000000000000000, 0.8660254037844387076, 1.000000000000000000, 0.8660254037844387076, 1.000000000000000000, 0.8660254037844387076, 1.000000000000000000, 0.8660254037844387076, 1.000000000000000000, 0.8660254037844387076, 1.000000000000000000, 0.8660254037844387076, 1.000000000000000000, 0.8660254037844387076, 1.000000000000000000),
 ( 1.000000000000000000, 0.8660254037844387076, 1.000000000000000000, 0.8660254037844387076, 1.000000000000000000, 0.8660254037844387076, 1.000000000000000000, 0.8660254037844387076, 1.000000000000000000, 0.8660254037844387076, 1.000000000000000000, 0.8660254037844387076, 1.000000000000000000, 0.8660254037844387076, 1.000000000000000000, 0.8660254037844387076, 1.000000000000000000, 0.8660254037844387076, 1.000000000000000000, 0.8660254037844387076, 1.000000000000000000, 0.8660254037844387076, 1.000000000000000000, 0.8660254037844387076, 1.000000000000000000, 0.8660254037844387076, 1.000000000000000000, 0.8660254037844387076, 1.000000000000000000, 0.8660254037844387076, 1.000000000000000000, 0.8660254037844387076, 1.000000000000000000, 0.8660254037844387076, 1.000000000000000000, 0.8660254037844387076, 1.000000000000000000, 0.8660254037844387076, 1.000000000000000000, 0.8660254037844387076, 1.000000000000000000, 0.8660254037844387076, 1.000000000000000000, 0.8660254037844387076, 1.000000000000000000, 0.8660254037844387076, 1.000000000000000000, 0.8660254037844387076, 1.000000000000000000, 0.8660254037844387076, 1.000000000000000000, 0.8660254037844387076, 1.000000000000000000, 0.8660254037844387076, 1.000000000000000000, 0.8660254037844387076, 1.000000000000000000, 0.8660254037844387076, 1.000000000000000000, 0.8660254037844387076, 1.000000000000000000, 0.8660254037844387076, 1.000000000000000000, 0.8660254037844387076, 1.000000000000000000, 0.8660254037844387076, 1.000000000000000000, 0.8660254037844387076, 1.000000000000000000, 0.8660254037844387076, 1.000000000000000000, 0.8660254037844387076, 1.000000000000000000, 0.8660254037844387076, 1.000000000000000000, 0.8660254037844387076, 1.000000000000000000, 0.8660254037844387076, 1.000000000000000000, 0.8660254037844387076, 1.000000000000000000, 0.8660254037844387076, 1.000000000000000000, 0.8660254037844387076, 1.000000000000000000, 0.8660254037844387076, 1.000000000000000000, 0.8660254037844387076, 1.000000000000000000, 0.8660254037844387076, 1.000000000000000000, 0.8660254037844387076, 1.000000000000000000, 0.8660254037844387076, 1.000000000000000000, 0.8660254037844387076, 1.000000000000000000, 0.8660254037844387076, 1.000000000000000000, 0.8660254037844387076, 1.000000000000000000, 0.8660254037844387076, 1.000000000000000000, 0.8660254037844387076, 1.000000000000000000, 0.8660254037844387076, 1.000000000000000000, 0.8660254037844387076, 1.000000000000000000, 0.8660254037844387076, 1.000000000000000000, 0.8660254037844387076, 1.000000000000000000, 0.8660254037844387076, 1.000000000000000000, 0.8660254037844387076, 1.000000000000000000, 0.8660254037844387076, 1.000000000000000000, 0.8660254037844387076, 1.000000000000000000, 0.8660254037844387076, 1.000000000000000000, 0.8660254037844387076, 1.000000000000000000, 0.8660254037844387076, 1.000000000000000000, 0.8660254037844387076, 1.000000000000000000, 0.8660254037844387076, 1.000000000000000000, 0.8660254037844387076, 1.000000000000000000, 0.8660254037844387076, 1.000000000000000000, 0.8660254037844387076, 1.000000000000000000, 0.8660254037844387076, 1.000000000000000000, 0.8660254037844387076, 1.000000000000000000, 0.8660254037844387076, 1.000000000000000000, 0.8660254037844387076, 1.000000000000000000, 0.8660254037844387076, 1.000000000000000000, 0.8660254037844387076, 1.000000000000000000, 0.8660254037844387076, 1.000000000000000000, 0.8660254037844387076, 1.000000000000000000, 0.8660254037844387076, 1.000000000000000000, 0.8660254037844387076, 1.000000000000000000, 0.8660254037844387076, 1.000000000000000000, 0.8660254037844387076, 1.000000000000000000, 0.8660254037844387076, 1.000000000000000000, 0.8660254037844387076, 1.000000000000000000, 0.8660254037844387076, 1.000000000000000000, 0.8660254037844387076, 1.000000000000000000, 0.8660254037844387076, 1.000000000000000000, 0.8660254037844387076, 1.000000000000000000, 0.8660254037844387076, 1.000000000000000000, 0.8660254037844387076, 1.000000000000000000, 0.8660254037844387076, 1.000000000000000000, 0.8660254037844387076, 1.000000000000000000, 0.8660254037844387076, 1.000000000000000000, 0.8660254037844387076, 1.000000000000000000, 0.8660254037844387076, 1.000000000000000000, 0.8660254037844387076, 1.000000000000000000, 0.8660254037844387076, 1.000000000000000000, 0.8660254037844387076, 1.000000000000000000, 0.8660254037844387076, 1.000000000000000000, 0.8660254037844387076, 1.000000000000000000, 0.8660254037844387076, 1.000000000000000000, 0.8660254037844387076, 1.000000000000000000, 0.8660254037844387076, 1.000000000000000000, 0.8660254037844387076, 1.000000000000000000, 0.8660254037844387076, 1.000000000000000000, 0.8660254037844387076, 1.000000000000000000, 0.8660254037844387076, 1.000000000000000000, 0.8660254037844387076, 1.000000000000000000, 0.8660254037844387076, 1.000000000000000000, 0.8660254037844387076, 1.000000000000000000, 0.8660254037844387076, 1.000000000000000000, 0.8660254037844387076, 1.000000000000000000, 0.8660254037844387076, 1.000000000000000000, 0.8660254037844387076, 1.000000000000000000, 0.8660254037844387076, 1.000000000000000000, 0.8660254037844387076, 1.000000000000000000, 0.8660254037844387076, 1.000000000000000000, 0.8660254037844387076, 1.000000000000000000, 0.8660254037844387076, 1.000000000000000000, 0.8660254037844387076, 1.000000000000000000, 0.8660254037844387076, 1.000000000000000000, 0.8660254037844387076, 1.000000000000000000, 0.8660254037844387076, 1.000000000000000000, 0.8660254037844387076, 1.000000000000000000, 0.8660254037844387076, 1.000000000000000000, 0.8660254037844387076, 1.000000000000000000, 0.8660254037844387076, 1.000000000000000000, 0.8660254037844387076, 1.000000000000000000, 0.8660254037844387076, 1.000000000000000000, 0.8660254037844387076, 1.000000000000000000, 0.8660254037844387076, 1.000000000000000000, 0.8660254037844387076, 1.000000000000000000, 0.8660254037844387076, 1.000000000000000000, 0.8660254037844387076, 1.000000000000000000, 0.8660254037844387076, 1.000000000000000000, 0.8660254037844387076, 1.000000000000000000, 0.8660254037844387076, 1.000000000000000000, 0.8660254037844387076, 1.000000000000000000, 0.8660254037844387076, 1.000000000000000000, 0.8660254037844387076, 1.000000000000000000, 0.8660254037844387076, 1.000000000000000000, 0.8660254037844387076, 1.000000000000000000, 0.8660254037844387076, 1.000000000000000000, 0.8660254037844387076, 1.000000000000000000, 0.8660254037844387076, 1.000000000000000000, 0.8660254037844387076, 1.000000000000000000, 0.8660254037844387076, 1.000000000000000000, 0.8660254037844387076, 1.000000000000000000, 0.8660254037844387076, 1.000000000000000000, 0.8660254037844387076, 1.000000000000000000, 0.8660254037844387076, 1.000000000000000000, 0.8660254037844387076, 1.000000000000000000, 0.8660254037844387076, 1.000000000000000000, 0.8660254037844387076, 1.000000000000000000, 0.8660254037844387076, 1.000000000000000000, 0.8660254037844387076, 1.000000000000000000, 0.8660254037844387076, 1.000000000000000000, 0.8660254037844387076, 1.000000000000000000, 0.8660254037844387076, 1.000000000000000000, 0.8660254037844387076, 1.000000000000000000, 0.8660254037844387076, 1.000000000000000000, 0.8660254037844387076, 1.000000000000000000, 0.8660254037844387076, 1.000000000000000000, 0.8660254037844387076, 1.000000000000000000, 0.8660254037844387076, 1.000000000000000000, 0.8660254037844387076, 1.000000000000000000, 0.8660254037844387076, 1.000000000000000000, 0.8660254037844387076, 1.000000000000000000, 0.8660254037844387076, 1.000000000000000000, 0.8660254037844387076, 1.000000000000000000, 0.8660254037844387076, 1.000000000000000000, 0.8660254037844387076, 1.000000000000000000, 0.8660254037844387076, 1.000000000000000000, 0.8660254037844387076, 1.000000000000000000, 0.8660254037844387076, 1.000000000000000000, 0.8660254037844387076, 1.000000000000000000, 0.8660254037844387076, 1.000000000000000000, 0.8660254037844387076, 1.000000000000000000, 0.8660254037844387076, 1.000000000000000000, 0.8660254037844387076, 1.000000000000000000, 0.8660254037844387076, 1.000000000000000000, 0.8660254037844387076, 1.000000000000000000, 0.8660254037844387076, 1.000000000000000000, 0.8660254037844387076, 1.000000000000000000, 0.8660254037844387076, 1.000000000000000000, 0.8660254037844387076, 1.000000000000000000, 0.8660254037844387076, 1.000000000000000000, 0.8660254037844387076, 1.000000000000000000, 0.8660254037844387076, 1.000000000000000000, 0.8660254037844387076, 1.000000000000000000, 0.8660254037844387076, 1.000000000000000000, 0.8660254037844387076, 1.000000000000000000, 0.8660254037844387076, 1.000000000000000000, 0.8660254037844387076, 1.000000000000000000, 0.8660254037844387076, 1.000000000000000000, 0.8660254037844387076, 1.000000000000000000, 0.8660254037844387076, 1.000000000000000000, 0.8660254037844387076, 1.000000000000000000, 0.8660254037844387076, 1.000000000000000000, 0.8660254037844387076, 1.000000000000000000, 0.8660254037844387076, 1.000000000000000000, 0.8660254037844387076, 1.000000000000000000, 0.8660254037844387076, 1.000000000000000000, 0.8660254037844387076, 1.000000000000000000, 0.8660254037844387076, 1.000000000000000000, 0.8660254037844387076, 1.000000000000000000, 0.8660254037844387076, 1.000000000000000000, 0.8660254037844387076, 1.000000000000000000, 0.8660254037844387076, 1.000000000000000000, 0.8660254037844387076, 1.000000000000000000, 0.8660254037844387076, 1.000000000000000000, 0.8660254037844387076, 1.000000000000000000, 0.8660254037844387076, 1.000000000000000000, 0.8660254037844387076, 1.000000000000000000, 0.8660254037844387076, 1.000000000000000000, 0.8660254037844387076, 1.000000000000000000, 0.8660254037844387076, 1.000000000000000000, 0.8660254037844387076, 1.000000000000000000, 0.8660254037844387076, 1.000000000000000000, 0.8660254037844387076, 1.000000000000000000, 0.8660254037844387076, 1.000000000000000000, 0.8660254037844387076, 1.000000000000000000, 0.8660254037844387076, 1.000000000000000000, 0.8660254037844387076, 1.000000000000000000, 0.8660254037844387076, 1.000000000000000000, 0.8660254037844387076, 1.000000000000000000, 0.8660254037844387076, 1.000000000000000000, 0.8660254037844387076, 1.000000000000000000, 0.8660254037844387076, 1.000000000000000000, 0.8660254037844387076, 1.000000000000000000, 0.8660254037844387076, 1.000000000000000000, 0.8660254037844387076, 1.000000000000000000, 0.8660254037844387076, 1.000000000000000000, 0.8660254037844387076, 1.000000000000000000, 0.8660254037844387076, 1.000000000000000000, 0.8660254037844387076, 1.000000000000000000, 0.8660254037844387076, 1.000000000000000000, 0.8660254037844387076, 1.000000000000000000, 0.8660254037844387076, 1.000000000000000000, 0.8660254037844387076, 1.000000000000000000, 0.8660254037844387076, 1.000000000000000000, 0.8660254037844387076, 1.000000000000000000, 0.8660254037844387076, 1.000000000000000000, 0.8660254037844387076, 1.000000000000000000, 0.8660254037844387076, 1.000000000000000000, 0.8660254037844387076, 1.000000000000000000, 0.8660254037844387076, 1.000000000000000000, 0.8660254037844387076, 1.000000000000000000, 0.8660254037844387076, 1.000000000000000000, 0.8660254037844387076, 1.000000000000000000, 0.8660254037844387076, 1.000000000000000000, 0.8660254037844387076, 1.000000000000000000, 0.8660254037844387076, 1.000000000000000000, 0.8660254037844387076, 1.000000000000000000, 0.8660254037844387076, 1.000000000000000000, 0.8660254037844387076, 1.000000000000000000, 0.8660254037844387076, 1.000000000000000000, 0.8660254037844387076, 1.000000000000000000, 0.8660254037844387076, 1.000000000000000000, 0.8660254037844387076, 1.000000000000000000, 0.8660254037844387076, 1.000000000000000000, 0.8660254037844387076, 1.000000000000000000, 0.8660254037844387076, 1.000000000000000000, 0.8660254037844387076, 1.000000000000000000, 0.8660254037844387076, 1.000000000000000000, 0.8660254037844387076, 1.000000000000000000, 0.8660254037844387076, 1.000000000000000000, 0.8660254037844387076, 1.000000000000000000, 0.8660254037844387076, 1.000000000000000000, 0.8660254037844387076, 1.000000000000000000, 0.8660254037844387076, 1.000000000000000000, 0.8660254037844387076, 1.000000000000000000, 0.8660254037844387076, 1.000000000000000000, 0.8660254037844387076, 1.000000000000000000, 0.8660254037844387076, 1.000000000000000000, 0.8660254037844387076, 1.000000000000000000, 0.8660254037844387076, 1.000000000000000000, 0.8660254037844387076, 1.000000000000000000, 0.8660254037844387076, 1.000000000000000000, 0.8660254037844387076, 1.000000000000000000, 0.8660254037844387076, 1.000000000000000000, 0.8660254037844387076, 1.000000000000000000, 0.8660254037844387076, 1.000000000000000000, 0.8660254037844387076, 1.000000000000000000, 0.8660254037844387076, 1.000000000000000000, 0.8660254037844387076, 1.000000000000000000, 0.8660254037844387076, 1.000000000000000000, 0.8660254037844387076, 1.000000000000000000, 0.8660254037844387076, 1.000000000000000000, 0.8660254037844387076, 1.000000000000000000, 0.8660254037844387076, 1.000000000000000000, 0.8660254037844387076, 1.000000000000000000, 0.8660254037844387076, 1.000000000000000000, 0.8660254037844387076, 1.000000000000000000, 0.8660254037844387076, 1.000000000000000000, 0.8660254037844387076, 1.000000000000000000, 0.8660254037844387076, 1.000000000000000000, 0.8660254037844387076, 1.000000000000000000, 0.8660254037844387076, 1.000000000000000000, 0.8660254037844387076, 1.000000000000000000, 0.8660254037844387076, 1.000000000000000000, 0.8660254037844387076, 1.000000000000000000, 0.8660254037844387076, 1.000000000000000000, 0.8660254037844387076, 1.000000000000000000, 0.8660254037844387076, 1.000000000000000000, 0.8660254037844387076, 1.000000000000000000, 0.8660254037844387076, 1.000000000000000000, 0.8660254037844387076, 1.000000000000000000, 0.8660254037844387076, 1.000000000000000000, 0.8660254037844387076, 1.000000000000000000, 0.8660254037844387076, 1.000000000000000000, 0.8660254037844387076, 1.000000000000000000, 0.8660254037844387076, 1.000000000000000000, 0.8660254037844387076, 1.000000000000000000, 0.8660254037844387076, 1.000000000000000000, 0.8660254037844387076, 1.000000000000000000, 0.8660254037844387076, 1.000000000000000000, 0.8660254037844387076, 1.000000000000000000, 0.8660254037844387076, 1.000000000000000000, 0.8660254037844387076, 1.000000000000000000, 0.8660254037844387076, 1.000000000000000000, 0.8660254037844387076, 1.000000000000000000, 0.8660254037844387076, 1.000000000000000000, 0.8660254037844387076, 1.000000000000000000, 0.8660254037844387076, 1.000000000000000000, 0.8660254037844387076, 1.000000000000000000, 0.8660254037844387076, 1.000000000000000000, 0.8660254037844387076, 1.000000000000000000, 0.8660254037844387076, 1.000000000000000000, 0.8660254037844387076, 1.000000000000000000, 0.8660254037844387076, 1.000000000000000000, 0.8660254037844387076, 1.000000000000000000, 0.8660254037844387076, 1.000000000000000000, 0.8660254037844387076, 1.000000000000000000, 0.8660254037844387076, 1.000000000000000000, 0.8660254037844387076, 1.000000000000000000, 0.8660254037844387076, 1.000000000000000000, 0.8660254037844387076, 1.000000000000000000, 0.8660254037844387076, 1.000000000000000000, 0.8660254037844387076, 1.000000000000000000, 0.8660254037844387076, 1.000000000000000000, 0.8660254037844387076, 1.000000000000000000, 0.8660254037844387076, 1.000000000000000000, 0.8660254037844387076, 1.000000000000000000, 0.8660254037844387076, 1.000000000000000000, 0.8660254037844387076, 1.000000000000000000, 0.8660254037844387076, 1.000000000000000000, 0.8660254037844387076, 1.000000000000000000, 0.8660254037844387076, 1.000000000000000000, 0.8660254037844387076, 1.000000000000000000, 0.8660254037844387076, 1.000000000000000000, 0.8660254037844387076, 1.000000000000000000, 0.8660254037844387076, 1.000000000000000000, 0.8660254037844387076, 1.000000000000000000, 0.8660254037844387076, 1.000000000000000000, 0.8660254037844387076, 1.000000000000000000, 0.8660254037844387076, 1.000000000000000000, 0.8660254037844387076, 1.000000000000000000, 0.8660254037844387076, 1.000000000000000000, 0.8660254037844387076, 1.000000000000000000, 0.8660254037844387076, 1.000000000000000000, 0.8660254037844387076, 1.000000000000000000, 0.8660254037844387076, 1.000000000000000000, 0.8660254037844387076, 1.000000000000000000, 0.8660254037844387076, 1.000000000000000000, 0.8660254037844387076, 1.000000000000000000, 0.8660254037844387076, 1.000000000000000000, 0.8660254037844387076, 1.000000000000000000, 0.8660254037844387076, 1.000000000000000000, 0.8660254037844387076, 1.000000000000000000, 0.8660254037844387076, 1.000000000000000000, 0.8660254037844387076, 1.000000000000000000, 0.8660254037844387076, 1.000000000000000000, 0.8660254037844387076, 1.000000000000000000, 0.8660254037844387076, 1.000000000000000000, 0.8660254037844387076, 1.000000000000000000, 0.8660254037844387076, 1.000000000000000000, 0.8660254037844387076, 1.000000000000000000, 0.8660254037844387076, 1.000000000000000000, 0.8660254037844387076, 1.000000000000000000, 0.8660254037844387076, 1.000000000000000000, 0.8660254037844387076, 1.000000000000000000, 0.8660254037844387076, 1.000000000000000000, 0.8660254037844387076, 1.000000000000000000, 0.8660254037844387076, 1.000000000000000000, 0.8660254037844387076, 1.000000000000000000, 0.8660254037844387076, 1.000000000000000000, 0.8660254037844387076, 1.000000000000000000, 0.8660254037844387076, 1.000000000000000000, 0.8660254037844387076, 1.000000000000000000, 0.8660254037844387076, 1.000000000000000000, 0.8660254037844387076, 1.000000000000000000, 0.8660254037844387076, 1.000000000000000000, 0.8660254037844387076, 1.000000000000000000, 0.8660254037844387076, 1.000000000000000000, 0.8660254037844387076, 1.000000000000000000, 0.8660254037844387076, 1.000000000000000000, 0.8660254037844387076, 1.000000000000000000, 0.8660254037844387076, 1.000000000000000000, 0.8660254037844387076, 1.000000000000000000, 0.8660254037844387076, 1.000000000000000000, 0.8660254037844387076, 1.000000000000000000, 0.8660254037844387076, 1.000000000000000000, 0.8660254037844387076, 1.000000000000000000, 0.8660254037844387076, 1.000000000000000000, 0.8660254037844387076, 1.000000000000000000, 0.8660254037844387076, 1.000000000000000000, 0.8660254037844387076, 1.000000000000000000, 0.8660254037844387076, 1.000000000000000000, 0.8660254037844387076, 1.000000000000000000, 0.8660254037844387076, 1.000000000000000000, 0.8660254037844387076, 1.000000000000000000, 0.8660254037844387076, 1.000000000000000000, 0.8660254037844387076, 1.000000000000000000, 0.8660254037844387076, 1.000000000000000000, 0.8660254037844387076, 1.000000000000000000, 0.8660254037844387076, 1.000000000000000000, 0.8660254037844387076, 1.000000000000000000, 0.8660254037844387076, 1.000000000000000000, 0.8660254037844387076, 1.000000000000000000, 0.8660254037844387076, 1.000000000000000000, 0.8660254037844387076, 1.000000000000000000, 0.8660254037844387076, 1.000000000000000000, 0.8660254037844387076, 1.000000000000000000, 0.8660254037844387076, 1.000000000000000000, 0.8660254037844387076, 1.000000000000000000, 0.8660254037844387076, 1.000000000000000000, 0.8660254037844387076, 1.000000000000000000, 0.8660254037844387076, 1.000000000000000000, 0.8660254037844387076, 1.000000000000000000, 0.8660254037844387076, 1.000000000000000000, 0.8660254037844387076, 1.000000000000000000, 0.8660254037844387076, 1.000000000000000000, 0.8660254037844387076, 1.000000000000000000, 0.8660254037844387076, 1.000000000000000000, 0.8660254037844387076, 1.000000000000000000, 0.8660254037844387076, 1.000000000000000000, 0.8660254037844387076, 1.000000000000000000, 0.8660254037844387076, 1.000000000000000000, 0.8660254037844387076, 1.000000000000000000, 0.8660254037844387076, 1.000000000000000000, 0.8660254037844387076, 1.000000000000000000, 0.8660254037844387076, 1.000000000000000000, 0.8660254037844387076, 1.000000000000000000, 0.8660254037844387076, 1.000000000000000000, 0.8660254037844387076, 1.000000000000000000, 0.8660254037844387076, 1.000000000000000000, 0.8660254037844387076, 1.000000000000000000, 0.8660254037844387076, 1.000000000000000000, 0.8660254037844387076, 1.000000000000000000, 0.8660254037844387076, 1.000000000000000000, 0.8660254037844387076, 1.000000000000000000, 0.8660254037844387076, 1.000000000000000000, 0.8660254037844387076, 1.000000000000000000, 0.8660254037844387076, 1.000000000000000000, 0.8660254037844387076, 1.000000000000000000, 0.8660254037844387076, 1.000000000000000000, 0.8660254037844387076, 1.000000000000000000, 0.8660254037844387076, 1.000000000000000000, 0.8660254037844387076, 1.000000000000000000, 0.8660254037844387076, 1.000000000000000000, 0.8660254037844387076, 1.000000000000000000, 0.8660254037844387076, 1.000000000000000000, 0.8660254037844387076, 1.000000000000000000, 0.8660254037844387076, 1.000000000000000000, 0.8660254037844387076, 1.000000000000000000, 0.8660254037844387076, 1.000000000000000000, 0.8660254037844387076, 1.000000000000000000, 0.8660254037844387076, 1.000000000000000000, 0.8660254037844387076, 1.000000000000000000, 0.8660254037844387076, 1.000000000000000000, 0.8660254037844387076, 1.000000000000000000, 0.8660254037844387076, 1.000000000000000000, 0.8660254037844387076, 1.000000000000000000, 0.8660254037844387076, 1.000000000000000000, 0.8660254037844387076, 1.000000000000000000, 0.8660254037844387076, 1.000000000000000000, 0.8660254037844387076, 1.000000000000000000, 0.8660254037844387076, 1.000000000000000000, 0.8660254037844387076, 1.000000000000000000, 0.8660254037844387076, 1.000000000000000000, 0.8660254037844387076, 1.000000000000000000, 0.8660254037844387076, 1.000000000000000000, 0.8660254037844387076, 1.000000000000000000, 0.8660254037844387076, 1.000000000000000000, 0.8660254037844387076, 1.000000000000000000, 0.8660254037844387076, 1.000000000000000000, 0.8660254037844387076, 1.000000000000000000, 0.8660254037844387076, 1.000000000000000000, 0.8660254037844387076, 1.000000000000000000, 0.8660254037844387076, 1.000000000000000000, 0.8660254037844387076, 1.000000000000000000, 0.8660254037844387076, 1.000000000000000000, 0.8660254037844387076, 1.000000000000000000, 0.8660254037844387076, 1.000000000000000000, 0.8660254037844387076, 1.000000000000000000, 0.8660254037844387076, 1.000000000000000000, 0.8660254037844387076, 1.000000000000000000, 0.8660254037844387076, 1.000000000000000000, 0.8660254037844387076, 1.000000000000000000, 0.8660254037844387076, 1.000000000000000000, 0.8660254037844387076, 1.000000000000000000, 0.8660254037844387076, 1.000000000000000000, 0.8660254037844387076, 1.000000000000000000, 0.8660254037844387076, 1.000000000000000000, 0.8660254037844387076, 1.000000000000000000, 0.8660254037844387076, 1.000000000000000000, 0.8660254037844387076, 1.000000000000000000, 0.8660254037844387076, 1.000000000000000000, 0.8660254037844387076, 1.000000000000000000, 0.8660254037844387076, 1.000000000000000000, 0.8660254037844387076, 1.000000000000000000, 0.8660254037844387076, 1.000000000000000000, 0.8660254037844387076, 1.000000000000000000, 0.8660254037844387076, 1.000000000000000000, 0.8660254037844387076, 1.000000000000000000, 0.8660254037844387076, 1.000000000000000000, 0.8660254037844387076, 1.000000000000000000, 0.8660254037844387076, 1.000000000000000000, 0.8660254037844387076, 1.000000000000000000, 0.8660254037844387076, 1.000000000000000000, 0.8660254037844387076, 1.000000000000000000, 0.8660254037844387076, 1.000000000000000000, 0.8660254037844387076, 1.000000000000000000, 0.8660254037844387076, 1.000000000000000000, 0.8660254037844387076, 1.000000000000000000, 0.8660254037844387076, 1.000000000000000000, 0.8660254037844387076, 1.000000000000000000, 0.8660254037844387076, 1.000000000000000000, 0.8660254037844387076, 1.000000000000000000, 0.8660254037844387076, 1.000000000000000000, 0.8660254037844387076, 1.000000000000000000, 0.8660254037844387076, 1.000000000000000000, 0.8660254037844387076, 1.000000000000000000, 0.8660254037844387076, 1.000000000000000000, 0.8660254037844387076, 1.000000000000000000, 0.8660254037844387076, 1.000000000000000000, 0.8660254037844387076, 1.000000000000000000, 0.8660254037844387076, 1.000000000000000000, 0.8660254037844387076, 1.000000000000000000, 0.8660254037844387076, 1.000000000000000000, 0.8660254037844387076, 1.000000000000000000, 0.8660254037844387076, 1.000000000000000000, 0.8660254037844387076, 1.000000000000000000, 0.8660254037844387076, 1.000000000000000000, 0.8660254037844387076, 1.000000000000000000, 0.8660254037844387076, 1.000000000000000000, 0.8660254037844387076, 1.000000000000000000, 0.8660254037844387076, 1.000000000000000000, 0.8660254037844387076, 1.000000000000000000, 0.8660254037844387076, 1.000000000000000000, 0.8660254037844387076, 1.000000000000000000, 0.8660254037844387076, 1.000000000000000000, 0.8660254037844387076, 1.000000000000000000, 0.8660254037844387076, 1.000000000000000000, 0.8660254037844387076, 1.000000000000000000, 0.8660254037844387076, 1.000000000000000000, 0.8660254037844387076, 1.000000000000000000, 0.8660254037844387076, 1.000000000000000000, 0.8660254037844387076, 1.000000000000000000, 0.8660254037844387076, 1.000000000000000000, 0.8660254037844387076, 1.000000000000000000, 0.8660254037844387076, 1.000000000000000000, 0.8660254037844387076, 1.000000000000000000, 0.8660254037844387076, 1.000000000000000000, 0.8660254037844387076, 1.000000000000000000, 0.8660254037844387076, 1.000000000000000000, 0.8660254037844387076, 1.000000000000000000, 0.8660254037844387076, 1.000000000000000000, 0.8660254037844387076, 1.000000000000000000, 0.8660254037844387076, 1.000000000000000000, 0.8660254037844387076, 1.000000000000000000, 0.8660254037844387076, 1.000000000000000000, 0.8660254037844387076, 1.000000000000000000, 0.8660254037844387076, 1.000000000000000000, 0.8660254037844387076, 1.000000000000000000, 0.8660254037844387076, 1.000000000000000000, 0.8660254037844387076, 1.000000000000000000, 0.8660254037844387076, 1.000000000000000000, 0.8660254037844387076, 1.000000000000000000, 0.8660254037844387076, 1.000000000000000000, 0.8660254037844387076, 1.000000000000000000, 0.8660254037844387076, 1.000000000000000000, 0.8660254037844387076, 1.000000000000000000, 0.8660254037844387076, 1.000000000000000000, 0.8660254037844387076, 1.000000000000000000, 0.8660254037844387076, 1.000000000000000000, 0.8660254037844387076, 1.000000000000000000, 0.8660254037844387076, 1.000000000000000000, 0.8660254037844387076, 1.000000000000000000, 0.8660254037844387076, 1.000000000000000000, 0.8660254037844387076, 1.000000000000000000, 0.8660254037844387076, 1.000000000000000000, 0.8660254037844387076, 1.000000000000000000, 0.8660254037844387076, 1.000000000000000000, 0.8660254037844387076, 1.000000000000000000, 0.8660254037844387076, 1.000000000000000000, 0.8660254037844387076, 1.000000000000000000, 0.8660254037844387076, 1.000000000000000000, 0.8660254037844387076, 1.000000000000000000, 0.8660254037844387076, 1.000000000000000000, 0.8660254037844387076, 1.000000000000000000, 0.8660254037844387076, 1.000000000000000000, 0.8660254037844387076, 1.000000000000000000, 0.8660254037844387076, 1.000000000000000000, 0.8660254037844387076, 1.000000000000000000, 0.8660254037844387076, 1.000000000000000000, 0.8660254037844387076, 1.000000000000000000, 0.8660254037844387076, 1.000000000000000000, 0.8660254037844387076, 1.000000000000000000, 0.8660254037844387076, 1.000000000000000000, 0.8660254037844387076, 1.000000000000000000, 0.8660254037844387076, 1.000000000000000000, 0.8660254037844387076, 1.000000000000000000, 0.8660254037844387076, 1.000000000000000000, 0.8660254037844387076, 1.000000000000000000, 0.8660254037844387076, 1.000000000000000000, 0.8660254037844387076, 1.000000000000000000, 0.8660254037844387076, 1.000000000000000000, 0.8660254037844387076, 1.000000000000000000, 0.8660254037844387076, 1.000000000000000000, 0.8660254037844387076, 1.000000000000000000, 0.8660254037844387076, 1.000000000000000000, 0.8660254037844387076, 1.000000000000000000, 0.8660254037844387076, 1.000000000000000000, 0.8660254037844387076, 1.000000000000000000, 0.8660254037844387076, 1.000000000000000000, 0.8660254037844387076, 1.000000000000000000, 0.8660254037844387076, 1.000000000000000000, 0.8660254037844387076, 1.000000000000000000, 0.8660254037844387076, 1.000000000000000000, 0.8660254037844387076, 1.000000000000000000, 0.8660254037844387076, 1.000000000000000000, 0.8660254037844387076, 1.000000000000000000, 0.8660254037844387076, 1.000000000000000000, 0.8660254037844387076, 1.000000000000000000, 0.8660254037844387076, 1.000000000000000000, 0.8660254037844387076, 1.000000000000000000, 0.8660254037844387076, 1.000000000000000000, 0.8660254037844387076, 1.000000000000000000, 0.8660254037844387076, 1.000000000000000000, 0.8660254037844387076, 1.000000000000000000, 0.8660254037844387076, 1.000000000000000000, 0.8660254037844387076, 1.000000000000000000, 0.8660254037844387076, 1.000000000000000000, 0.8660254037844387076, 1.000000000000000000, 0.8660254037844387076, 1.000000000000000000, 0.8660254037844387076, 1.000000000000000000, 0.8660254037844387076, 1.000000000000000000, 0.8660254037844387076, 1.000000000000000000, 0.8660254037844387076, 1.000000000000000000, 0.8660254037844387076, 1.000000000000000000, 0.8660254037844387076, 1.000000000000000000, 0.8660254037844387076, 1.000000000000000000, 0.8660254037844387076, 1.000000000000000000, 0.8660254037844387076, 1.000000000000000000, 0.8660254037844387076, 1.000000000000000000, 0.8660254037844387076, 1.000000000000000000, 0.8660254037844387076, 1.000000000000000000, 0.8660254037844387076, 1.000000000000000000, 0.8660254037844387076, 1.000000000000000000, 0.8660254037844387076, 1.000000000000000000, 0.8660254037844387076, 1.000000000000000000, 0.8660254037844387076, 1.000000000000000000, 0.8660254037844387076, 1.000000000000000000, 0.8660254037844387076, 1.000000000000000000, 0.8660254037844387076, 1.000000000000000000, 0.8660254037844387076, 1.000000000000000000, 0.8660254037844387076, 1.000000000000000000, 0.8660254037844387076, 1.000000000000000000, 0.8660254037844387076, 1.000000000000000000, 0.8660254037844387076, 1.000000000000000000, 0.8660254037844387076, 1.000000000000000000, 0.8660254037844387076, 1.000000000000000000, 0.8660254037844387076, 1.000000000000000000, 0.8660254037844387076, 1.000000000000000000, 0.8660254037844387076, 1.000000000000000000, 0.8660254037844387076, 1.000000000000000000, 0.8660254037844387076, 1.000000000000000000, 0.8660254037844387076, 1.000000000000000000, 0.8660254037844387076, 1.000000000000000000, 0.8660254037844387076, 1.000000000000000000, 0.8660254037844387076, 1.000000000000000000, 0.8660254037844387076, 1.000000000000000000, 0.8660254037844387076, 1.000000000000000000, 0.8660254037844387076, 1.000000000000000000, 0.8660254037844387076, 1.000000000000000000, 0.8660254037844387076, 1.000000000000000000, 0.8660254037844387076, 1.000000000000000000, 0.8660254037844387076, 1.000000000000000000, 0.8660254037844387076, 1.000000000000000000, 0.8660254037844387076, 1.000000000000000000, 0.8660254037844387076, 1.000000000000000000, 0.8660254037844387076, 1.000000000000000000, 0.8660254037844387076, 1.000000000000000000, 0.8660254037844387076, 1.000000000000000000, 0.8660254037844387076, 1.000000000000000000, 0.8660254037844387076, 1.000000000000000000, 0.8660254037844387076, 1.000000000000000000, 0.8660254037844387076, 1.000000000000000000, 0.8660254037844387076, 1.000000000000000000, 0.8660254037844387076, 1.000000000000000000, 0.8660254037844387076, 1.000000000000000000, 0.8660254037844387076, 1.000000000000000000, 0.8660254037844387076, 1.000000000000000000, 0.8660254037844387076, 1.000000000000000000, 0.8660254037844387076, 1.000000000000000000, 0.8660254037844387076, 1.000000000000000000, 0.8660254037844387076, 1.000000000000000000, 0.8660254037844387076, 1.000000000000000000, 0.8660254037844387076, 1.000000000000000000, 0.8660254037844387076, 1.000000000000000000, 0.8660254037844387076, 1.000000000000000000, 0.8660254037844387076, 1.000000000000000000, 0.8660254037844387076, 1.000000000000000000, 0.8660254037844387076, 1.000000000000000000, 0.8660254037844387076, 1.000000000000000000, 0.8660254037844387076, 1.000000000000000000, 0.8660254037844387076, 1.000000000000000000, 0.8660254037844387076, 1.000000000000000000, 0.8660254037844387076, 1.000000000000000000, 0.8660254037844387076, 1.000000000000000000, 0.8660254037844387076, 1.000000000000000000, 0.8660254037844387076, 1.000000000000000000, 0.8660254037844387076, 1.000000000000000000, 0.8660254037844387076, 1.000000000000000000, 0.8660254037844387076, 1.000000000000000000, 0.8660254037844387076, 1.000000000000000000, 0.8660254037844387076, 1.000000000000000000, 0.8660254037844387076, 1.000000000000000000, 0.8660254037844387076, 1.000000000000000000, 0.8660254037844387076, 1.000000000000000000, 0.8660254037844387076, 1.000000000000000000, 0.8660254037844387076, 1.000000000000000000, 0.8660254037844387076, 1.000000000000000000, 0.8660254037844387076, 1.000000000000000000, 0.8660254037844387076, 1.000000000000000000, 0.8660254037844387076, 1.000000000000000000, 0.8660254037844387076, 1.000000000000000000, 0.8660254037844387076, 1.000000000000000000, 0.8660254037844387076, 1.000000000000000000, 0.8660254037844387076, 1.000000000000000000, 0.8660254037844387076, 1.000000000000000000, 0.8660254037844387076, 1.000000000000000000, 0.8660254037844387076, 1.000000000000000000, 0.8660254037844387076, 1.000000000000000000, 0.8660254037844387076, 1.000000000000000000, 0.8660254037844387076, 1.000000000000000000, 0.8660254037844387076, 1.000000000000000000, 0.8660254037844387076, 1.000000000000000000, 0.8660254037844387076, 1.000000000000000000, 0.8660254037844387076, 1.000000000000000000, 0.8660254037844387076, 1.000000000000000000, 0.8660254037844387076, 1.000000000000000000, 0.8660254037844387076, 1.000000000000000000, 0.8660254037844387076, 1.000000000000000000, 0.8660254037844387076, 1.000000000000000000, 0.8660254037844387076, 1.000000000000000000, 0.8660254037844387076, 1.000000000000000000, 0.8660254037844387076, 1.000000000000000000, 0.8660254037844387076, 1.000000000000000000, 0.8660254037844387076, 1.000000000000000000, 0.8660254037844387076, 1.000000000000000000, 0.8660254037844387076, 1.000000000000000000, 0.8660254037844387076, 1.000000000000000000, 0.8660254037844387076, 1.000000000000000000, 0.8660254037844387076, 1.000000000000000000, 0.8660254037844387076, 1.000000000000000000, 0.8660254037844387076, 1.000000000000000000, 0.8660254037844387076, 1.000000000000000000, 0.8660254037844387076, 1.000000000000000000, 0.8660254037844387076, 1.000000000000000000, 0.8660254037844387076, 1.000000000000000000, 0.8660254037844387076, 1.000000000000000000, 0.8660254037844387076, 1.000000000000000000, 0.8660254037844387076, 1.000000000000000000, 0.8660254037844387076, 1.000000000000000000, 0.8660254037844387076, 1.000000000000000000, 0.8660254037844387076, 1.000000000000000000, 0.8660254037844387076, 1.000000000000000000, 0.8660254037844387076, 1.000000000000000000, 0.8660254037844387076, 1.000000000000000000, 0.8660254037844387076, 1.000000000000000000, 0.8660254037844387076, 1.000000000000000000, 0.8660254037844387076, 1.000000000000000000, 0.8660254037844387076, 1.000000000000000000, 0.8660254037844387076, 1.000000000000000000, 0.8660254037844387076, 1.000000000000000000, 0.8660254037844387076, 1.000000000000000000, 0.8660254037844387076, 1.000000000000000000, 0.8660254037844387076, 1.000000000000000000, 0.8660254037844387076, 1.000000000000000000, 0.8660254037844387076, 1.000000000000000000, 0.8660254037844387076, 1.000000000000000000, 0.8660254037844387076, 1.000000000000000000, 0.8660254037844387076, 1.000000000000000000, 0.8660254037844387076, 1.000000000000000000, 0.8660254037844387076, 1.000000000000000000, 0.8660254037844387076, 1.000000000000000000, 0.8660254037844387076, 1.000000000000000000, 0.8660254037844387076, 1.000000000000000000, 0.8660254037844387076, 1.000000000000000000) ) ) 
 REPRESENTATION_ITEM ( '' )  SURFACE ( )  );
#4986=CARTESIAN_POINT ( 'NONE',  ( -2.293366432827344421E-15, -12.48450537969573659, -61.90625000204838813 ) ) ;
#4988=ORIENTED_EDGE ( 'NONE', *, *, #16390, .T. ) ;
#4989=ORIENTED_EDGE ( 'NONE', *, *, #41755, .F. ) ;
#4992=CARTESIAN_POINT ( 'NONE',  ( -9.999999999998969713, -5.773502691896847949, -55.50000000409676204 ) ) ;
#4993=CARTESIAN_POINT ( 'NONE',  ( 10.81189881249999729, 0.000000000000000000, -158.8437500020483810 ) ) ;
#4995=( BOUNDED_CURVE ( )  B_SPLINE_CURVE ( 2, ( #40822, #24242, #14268, #7836, #17948, #14922, #31146 ),
 .UNSPECIFIED., .F., .F. ) 
 B_SPLINE_CURVE_WITH_KNOTS ( ( 3, 2, 2, 3 ),
 ( 0.7052238805970151292, 0.7064676616915425145, 0.7077114427860698997, 0.7089552238805972850 ),
 .UNSPECIFIED. ) 
 CURVE ( )  GEOMETRIC_REPRESENTATION_ITEM ( )  RATIONAL_B_SPLINE_CURVE ( ( 0.9999999999999761302, 0.8660254037844625774, 1.000000000000000000, 0.8660254037844387076, 1.000000000000000000, 0.8660254037844148378, 1.000000000000023981 ) ) 
 REPRESENTATION_ITEM ( '' )  );
#4997=CARTESIAN_POINT ( 'NONE',  ( 10.81189881249999551, -6.242252689847874514, -16.46875000204836326 ) ) ;
#4998=CARTESIAN_POINT ( 'NONE',  ( -10.00000000000102496, 5.773502691895664007, -30.25000000409673007 ) ) ;
#4999=CARTESIAN_POINT ( 'NONE',  ( 10.81189881249999729, 0.000000000000000000, -146.8437500020483810 ) ) ;
#5000=CARTESIAN_POINT ( 'NONE',  ( -2.293366432827344421E-15, -12.48450537969573659, -105.4062500020483810 ) ) ;
#5002=CARTESIAN_POINT ( 'NONE',  ( -2.121150477449813534E-15, -11.54700538379251284, -161.3750000000000000 ) ) ;
#5004=CARTESIAN_POINT ( 'NONE',  ( -10.81189881249999729, 1.324075727343319199E-15, -2.093750002048366810 ) ) ;
#5006=CARTESIAN_POINT ( 'NONE',  ( 7.644554776091147741E-16, 12.48450537969573659, -197.6562500020484094 ) ) ;
#5007=CARTESIAN_POINT ( 'NONE',  ( -9.999999999999998224, 1.224646799147353059E-15, -165.1250000040967905 ) ) ;
#5011=CARTESIAN_POINT ( 'NONE',  ( -10.81189881249999729, -6.242252689847864744, -73.96875000204836681 ) ) ;
#5012=CARTESIAN_POINT ( 'NONE',  ( 10.81189881249999729, 0.000000000000000000, -59.84375000204835970 ) ) ;
#5013=CARTESIAN_POINT ( 'NONE',  ( 10.00000000000025402, -5.773502691896113426, -116.5000000040967763 ) ) ;
#5014=CARTESIAN_POINT ( 'NONE',  ( 10.81189881249999729, 0.000000000000000000, -37.53125000204838102 ) ) ;
#5016=CARTESIAN_POINT ( 'NONE',  ( 9.999999999999998224, 0.000000000000000000, -53.37500000409675494 ) ) ;
#5018=CARTESIAN_POINT ( 'NONE',  ( 10.00000000000000000, 5.773502691896255534, -121.8750000000000000 ) ) ;
#5019=ADVANCED_FACE ( 'NONE', ( #29148 ), #2612, .T. ) ;
#5022=CARTESIAN_POINT ( 'NONE',  ( -10.81189881249999729, -6.242252689847864744, -8.156250002048370362 ) ) ;
#5024=CARTESIAN_POINT ( 'NONE',  ( -9.999999999999998224, 1.224646799147353059E-15, -200.0000000000000000 ) ) ;
#5028=CARTESIAN_POINT ( 'NONE',  ( -10.00000000000000000, -5.773502691896251982, -34.50000000409674783 ) ) ;
#5029=EDGE_CURVE ( 'NONE', #23394, #24472, #32300, .T. ) ;
#5032=CARTESIAN_POINT ( 'NONE',  ( 9.999999999999998224, 0.000000000000000000, -99.49999999999998579 ) ) ;
#5033=CARTESIAN_POINT ( 'NONE',  ( -5.405949406249996869, 9.363379034771805109, -146.5312500020483810 ) ) ;
#5034=CARTESIAN_POINT ( 'NONE',  ( 5.405949406249992428, -9.363379034771808662, -124.5937500020483952 ) ) ;
#5036=VERTEX_POINT ( 'NONE', #11281 ) ;
#5037=ORIENTED_EDGE ( 'NONE', *, *, #19605, .F. ) ;
#5038=ORIENTED_EDGE ( 'NONE', *, *, #10150, .F. ) ;
#5040=CARTESIAN_POINT ( 'NONE',  ( -5.405949406249996869, 9.363379034771805109, -185.3437500020483810 ) ) ;
#5041=CARTESIAN_POINT ( 'NONE',  ( 7.644554776091147741E-16, 12.48450537969573659, -41.46875000204835260 ) ) ;
#5043=CARTESIAN_POINT ( 'NONE',  ( 7.644554776091147741E-16, 12.48450537969573659, -173.4687500020483810 ) ) ;
#5044=CARTESIAN_POINT ( 'NONE',  ( -10.81189881249999729, 6.242252689847871849, -150.7187500020483810 ) ) ;
#5045=CARTESIAN_POINT ( 'NONE',  ( -9.999999999999998224, 1.224646799147353059E-15, -76.62500000409677625 ) ) ;
#5049=CARTESIAN_POINT ( 'NONE',  ( -2.121150477449813534E-15, -11.54700538379251284, -155.3750000000000000 ) ) ;
#5050=CARTESIAN_POINT ( 'NONE',  ( 9.999999999999998224, 0.000000000000000000, -170.0000000000000000 ) ) ;
#5052=CARTESIAN_POINT ( 'NONE',  ( -10.81189881249999907, -6.242252689847864744, -78.46875000204838102 ) ) ;
#5053=CARTESIAN_POINT ( 'NONE',  ( -5.405949406250003975, -9.363379034771801557, -60.53125000204836681 ) ) ;
#5056=CARTESIAN_POINT ( 'NONE',  ( 10.81189881249999729, 0.000000000000000000, -111.0312500020483810 ) ) ;
#5057=CARTESIAN_POINT ( 'NONE',  ( -10.81189881249999729, 1.324075727343319199E-15, -158.2812500020484094 ) ) ;
#5058=( BOUNDED_CURVE ( )  B_SPLINE_CURVE ( 2, ( #13780, #36890, #451, #13567, #10341, #27612, #26758 ),
 .UNSPECIFIED., .F., .F. ) 
 B_SPLINE_CURVE_WITH_KNOTS ( ( 3, 2, 2, 3 ),
 ( 0.9776119402985076201, 0.9788557213930348944, 0.9800995024875623907, 0.9813432835820897759 ),
 .UNSPECIFIED. ) 
 CURVE ( )  GEOMETRIC_REPRESENTATION_ITEM ( )  RATIONAL_B_SPLINE_CURVE ( ( 0.9999999999999880096, 0.8660254037844506980, 1.000000000000000000, 0.8660254037844387076, 1.000000000000000000, 0.8660254037844148378, 1.000000000000023981 ) ) 
 REPRESENTATION_ITEM ( '' )  );
#5059=CARTESIAN_POINT ( 'NONE',  ( 9.999999999999998224, 0.000000000000000000, -10.99999999999995381 ) ) ;
#5061=CARTESIAN_POINT ( 'NONE',  ( -9.999999999999998224, 5.773502691896259087, -133.7500000040967905 ) ) ;
#5067=CARTESIAN_POINT ( 'NONE',  ( 10.81189881249999729, 0.000000000000000000, -183.0312500020484094 ) ) ;
#5068=VERTEX_POINT ( 'NONE', #12709 ) ;
#5070=CARTESIAN_POINT ( 'NONE',  ( -9.999999999999998224, 1.224646799147353059E-15, -61.62500000409676204 ) ) ;
#5072=CARTESIAN_POINT ( 'NONE',  ( 9.999999999999998224, 0.000000000000000000, -200.0000000000000000 ) ) ;
#5073=CYLINDRICAL_SURFACE ( 'NONE', #24222, 9.999999999999998224 ) ;
#5074=ADVANCED_FACE ( 'NONE', ( #25496 ), #27918, .T. ) ;
#5078=FACE_OUTER_BOUND ( 'NONE', #6755, .T. ) ;
#5079=CARTESIAN_POINT ( 'NONE',  ( -2.293366432827344421E-15, -12.48450537969573659, -168.4062500020483810 ) ) ;
#5080=CARTESIAN_POINT ( 'NONE',  ( 9.999999999999998224, 0.000000000000000000, -135.8750000040967905 ) ) ;
#5085=FACE_OUTER_BOUND ( 'NONE', #29481, .T. ) ;
#5086=CARTESIAN_POINT ( 'NONE',  ( -2.293366432827344421E-15, -12.48450537969573659, -76.90625000204839523 ) ) ;
#5088=FACE_OUTER_BOUND ( 'NONE', #29859, .T. ) ;
#5089=CARTESIAN_POINT ( 'NONE',  ( -9.999999999999998224, 1.224646799147353059E-15, -200.0000000000000000 ) ) ;
#5090=ORIENTED_EDGE ( 'NONE', *, *, #35509, .T. ) ;
#5092=CARTESIAN_POINT ( 'NONE',  ( -10.81189881249999729, 1.324075727343319199E-15, -41.09375000204837391 ) ) ;
#5093=CARTESIAN_POINT ( 'NONE',  ( -9.999999999999998224, 1.224646799147353059E-15, -53.74999999999996447 ) ) ;
#5094=CARTESIAN_POINT ( 'NONE',  ( 10.81189881249999551, -6.242252689847874514, -10.65625000204838280 ) ) ;
#5095=CARTESIAN_POINT ( 'NONE',  ( 7.644554776091147741E-16, 12.48450537969573659, -62.46875000204839523 ) ) ;
#5097=DIRECTION ( 'NONE',  ( -0.000000000000000000, -0.000000000000000000, 1.000000000000000000 ) ) ;
#5099=CARTESIAN_POINT ( 'NONE',  ( -2.293366432827344421E-15, -12.48450537969573659, -192.2187500020484379 ) ) ;
#5100=CARTESIAN_POINT ( 'NONE',  ( -5.405949406249996869, 9.363379034771805109, -173.3437500020484094 ) ) ;
#5102=( BOUNDED_CURVE ( )  B_SPLINE_CURVE ( 2, ( #28540, #5443, #41672, #21834, #24666, #5656, #38235 ),
 .UNSPECIFIED., .F., .F. ) 
 B_SPLINE_CURVE_WITH_KNOTS ( ( 3, 2, 2, 3 ),
 ( 0.5149253731343285123, 0.5161691542288557866, 0.5174129353233831718, 0.5186567164179105571 ),
 .UNSPECIFIED. ) 
 CURVE ( )  GEOMETRIC_REPRESENTATION_ITEM ( )  RATIONAL_B_SPLINE_CURVE ( ( 0.9999999999999880096, 0.8660254037844506980, 1.000000000000000000, 0.8660254037844387076, 1.000000000000000000, 0.8660254037844267172, 1.000000000000011990 ) ) 
 REPRESENTATION_ITEM ( '' )  );
#5105=CARTESIAN_POINT ( 'NONE',  ( 7.644554776091147741E-16, 12.48450537969573659, -111.9687500020483952 ) ) ;
#5106=DIRECTION ( 'NONE',  ( 1.000000000000000000, 0.000000000000000000, 0.000000000000000000 ) ) ;
#5107=CARTESIAN_POINT ( 'NONE',  ( -2.293366432827344421E-15, -12.48450537969573659, -81.40625000204838102 ) ) ;
#5108=CARTESIAN_POINT ( 'NONE',  ( 5.405949406249992428, -9.363379034771808662, -94.59375000204838102 ) ) ;
#5111=CARTESIAN_POINT ( 'NONE',  ( -5.000000000000003553, -8.660254037844383745, -152.8750000040967905 ) ) ;
#5116=CARTESIAN_POINT ( 'NONE',  ( -9.999999999999941380, -5.773502691896284844, -197.6250000000000000 ) ) ;
#5119=CARTESIAN_POINT ( 'NONE',  ( -10.00000000000000000, -5.773502691896251982, -64.12499999999998579 ) ) ;
#5121=CARTESIAN_POINT ( 'NONE',  ( -9.999999999999998224, 1.224646799147353059E-15, -82.62500000409676204 ) ) ;
#5123=CARTESIAN_POINT ( 'NONE',  ( 9.999999999999998224, 0.000000000000000000, -150.5000000000000000 ) ) ;
#5125=CARTESIAN_POINT ( 'NONE',  ( 5.405949406249999534, 9.363379034771803333, -71.78125000204838102 ) ) ;
#5128=DIRECTION ( 'NONE',  ( 1.000000000000000000, 0.000000000000000000, 0.000000000000000000 ) ) ;
#5131=CARTESIAN_POINT ( 'NONE',  ( 9.999999999999998224, 0.000000000000000000, -0.4999999999999726885 ) ) ;
#5132=ADVANCED_FACE ( 'NONE', ( #9281 ), #35418, .T. ) ;
#5134=CARTESIAN_POINT ( 'NONE',  ( 10.81189881249999729, 6.242252689847867408, -10.21875000204836326 ) ) ;
#5135=CARTESIAN_POINT ( 'NONE',  ( -9.999999999999479527, -5.773502691896549521, -94.50000000409676204 ) ) ;
#5136=CARTESIAN_POINT ( 'NONE',  ( 5.405949406249999534, 9.363379034771803333, -142.0937500020483810 ) ) ;
#5139=CARTESIAN_POINT ( 'NONE',  ( -4.999999999999996447, 8.660254037844387298, -160.8750000040967905 ) ) ;
#5140=CARTESIAN_POINT ( 'NONE',  ( -10.81189881249999907, -6.242252689847864744, -129.6562500020483810 ) ) ;
#5141=CARTESIAN_POINT ( 'NONE',  ( -10.00000000000000000, -5.773502691896251982, -181.1249999999999716 ) ) ;
#5142=DIRECTION ( 'NONE',  ( -0.000000000000000000, -0.000000000000000000, 1.000000000000000000 ) ) ;
#5143=CARTESIAN_POINT ( 'NONE',  ( -5.405949406249996869, 9.363379034771805109, -110.5312500020483810 ) ) ;
#5145=CARTESIAN_POINT ( 'NONE',  ( -9.999999999999998224, 1.224646799147353059E-15, -183.1250000040967905 ) ) ;
#5148=CARTESIAN_POINT ( 'NONE',  ( -5.405949406249996869, 9.363379034771805109, -41.53125000204838102 ) ) ;
#5150=CARTESIAN_POINT ( 'NONE',  ( -10.81189881249999729, 1.324075727343319199E-15, -89.09375000204838102 ) ) ;
#5151=DIRECTION ( 'NONE',  ( -0.000000000000000000, -0.000000000000000000, 1.000000000000000000 ) ) ;
#5156=CARTESIAN_POINT ( 'NONE',  ( 5.405949406249999534, 9.363379034771803333, -116.5937500020483810 ) ) ;
#5158=CYLINDRICAL_SURFACE ( 'NONE', #31624, 9.999999999999998224 ) ;
#5161=CARTESIAN_POINT ( 'NONE',  ( 4.999999999999992006, -8.660254037844389075, -176.6250000040968189 ) ) ;
#5162=CARTESIAN_POINT ( 'NONE',  ( 5.405949406249999534, 9.363379034771803333, -169.2812500020484094 ) ) ;
#5163=CARTESIAN_POINT ( 'NONE',  ( -10.00000000000051337, 5.773502691895962435, -102.2500000040967905 ) ) ;
#5166=CARTESIAN_POINT ( 'NONE',  ( -10.81189881249999729, 6.242252689847871849, -47.21875000204836681 ) ) ;
#5169=CARTESIAN_POINT ( 'NONE',  ( 0.000000000000000000, 0.000000000000000000, -200.0000000000000000 ) ) ;
#5171=CARTESIAN_POINT ( 'NONE',  ( -5.000000000000003553, -8.660254037844383745, -98.49999999999998579 ) ) ;
#5173=CARTESIAN_POINT ( 'NONE',  ( 9.999999999999996447, -5.773502691896262640, -109.0000000040967763 ) ) ;
#5177=CARTESIAN_POINT ( 'NONE',  ( 7.644554776091147741E-16, 12.48450537969573659, -103.1562500020483952 ) ) ;
#5178=VERTEX_POINT ( 'NONE', #22664 ) ;
#5179=VECTOR ( 'NONE', #24692, 1000.000000000000000 ) ;
#5181=CARTESIAN_POINT ( 'NONE',  ( 9.999999999999998224, 0.000000000000000000, -91.99999999999998579 ) ) ;
#5182=CARTESIAN_POINT ( 'NONE',  ( 7.644554776091147741E-16, 12.48450537969573659, -155.6562500020484094 ) ) ;
#5184=ORIENTED_EDGE ( 'NONE', *, *, #31977, .T. ) ;
#5185=CARTESIAN_POINT ( 'NONE',  ( 7.070501591499377789E-16, 11.54700538379251284, -28.62499999999997513 ) ) ;
#5186=CARTESIAN_POINT ( 'NONE',  ( 5.405949406249999534, 9.363379034771803333, -28.28125000204837036 ) ) ;
#5187=CARTESIAN_POINT ( 'NONE',  ( -4.999999999999996447, 8.660254037844387298, -160.5000000000000000 ) ) ;
#5188=CARTESIAN_POINT ( 'NONE',  ( 9.999999999999998224, 0.000000000000000000, -102.5000000000000000 ) ) ;
#5190=EDGE_CURVE ( 'NONE', #2132, #31273, #19207, .T. ) ;
#5191=CARTESIAN_POINT ( 'NONE',  ( -5.405949406249996869, 9.363379034771805109, -137.5312500020484094 ) ) ;
#5192=CARTESIAN_POINT ( 'NONE',  ( -5.000020801129981152, 8.660290040615111096, 0.000000000000000000 ) ) ;
#5193=CARTESIAN_POINT ( 'NONE',  ( -5.000000000000003553, -8.660254037844383745, -68.87500000409677625 ) ) ;
#5194=ORIENTED_EDGE ( 'NONE', *, *, #11704, .F. ) ;
#5195=CARTESIAN_POINT ( 'NONE',  ( 10.81189881249999907, 6.242252689847868297, -58.40625000204838102 ) ) ;
#5197=VERTEX_POINT ( 'NONE', #9497 ) ;
#5198=VERTEX_POINT ( 'NONE', #4611 ) ;
#5200=CARTESIAN_POINT ( 'NONE',  ( 4.999999999999992006, -8.660254037844389075, -183.7500000000000000 ) ) ;
#5201=CARTESIAN_POINT ( 'NONE',  ( -10.81189881249999907, -6.242252689847864744, -154.9687500020484094 ) ) ;
#5202=VECTOR ( 'NONE', #34967, 1000.000000000000000 ) ;
#5204=CARTESIAN_POINT ( 'NONE',  ( 10.81189881249999729, 0.000000000000000000, -10.34375000204834549 ) ) ;
#5205=CARTESIAN_POINT ( 'NONE',  ( 5.405949406249992428, -9.363379034771808662, -136.5937500020483810 ) ) ;
#5206=CARTESIAN_POINT ( 'NONE',  ( 5.405949406249992428, -9.363379034771808662, -96.28125000204838102 ) ) ;
#5208=CARTESIAN_POINT ( 'NONE',  ( 5.000000000000000000, 8.660254037844385522, -55.74999999999996447 ) ) ;
#5210=CARTESIAN_POINT ( 'NONE',  ( 5.405949406249999534, 9.363379034771803333, -4.093750002048368586 ) ) ;
#5212=CARTESIAN_POINT ( 'NONE',  ( -5.405949406249996869, 9.363379034771805109, -197.5312500020484094 ) ) ;
#5213=CARTESIAN_POINT ( 'NONE',  ( -10.00000000000154188, 5.773502691895366468, -11.87499999999992006 ) ) ;
#5216=CARTESIAN_POINT ( 'NONE',  ( -2.293366432827344421E-15, -12.48450537969573659, -73.71875000204836681 ) ) ;
#5217=CARTESIAN_POINT ( 'NONE',  ( -5.405949406250003975, -9.363379034771801557, -55.84375000204835970 ) ) ;
#5219=CARTESIAN_POINT ( 'NONE',  ( 10.81189881249999907, 6.242252689847868297, -35.90625000204835260 ) ) ;
#5223=CARTESIAN_POINT ( 'NONE',  ( 4.999999999999992006, -8.660254037844389075, -123.7500000000000000 ) ) ;
#5228=CARTESIAN_POINT ( 'NONE',  ( 10.81189881249999729, 0.000000000000000000, -7.531250002048350822 ) ) ;
#5229=( BOUNDED_CURVE ( )  B_SPLINE_CURVE ( 2, ( #428, #7100, #40101, #29552, #16573, #26944, #4073 ),
 .UNSPECIFIED., .F., .F. ) 
 B_SPLINE_CURVE_WITH_KNOTS ( ( 3, 2, 2, 3 ),
 ( 0.9253731343283585487, 0.9266169154228859339, 0.9278606965174133192, 0.9291044776119405935 ),
 .UNSPECIFIED. ) 
 CURVE ( )  GEOMETRIC_REPRESENTATION_ITEM ( )  RATIONAL_B_SPLINE_CURVE ( ( 0.9999999999999641398, 0.8660254037844745678, 1.000000000000000000, 0.8660254037844387076, 1.000000000000000000, 0.8660254037844028474, 1.000000000000035971 ) ) 
 REPRESENTATION_ITEM ( '' )  );
#5230=ORIENTED_EDGE ( 'NONE', *, *, #480, .F. ) ;
#5231=VECTOR ( 'NONE', #13385, 1000.000000000000000 ) ;
#5236=CARTESIAN_POINT ( 'NONE',  ( 4.999999999999992006, -8.660254037844389075, -29.62500000409676204 ) ) ;
#5237=CARTESIAN_POINT ( 'NONE',  ( -9.999999999999998224, 1.224646799147353059E-15, -14.74999999999995737 ) ) ;
#5241=CARTESIAN_POINT ( 'NONE',  ( 5.405949406249992428, -9.363379034771808662, -144.2812500020483810 ) ) ;
#5242=CARTESIAN_POINT ( 'NONE',  ( 5.405949406249999534, 9.363379034771803333, -125.5937500020483668 ) ) ;
#5243=CARTESIAN_POINT ( 'NONE',  ( -9.999999999998969713, -5.773502691896847949, -65.62499999999997158 ) ) ;
#5244=DIRECTION ( 'NONE',  ( 1.000000000000000000, 0.000000000000000000, 0.000000000000000000 ) ) ;
#5245=ORIENTED_EDGE ( 'NONE', *, *, #40189, .T. ) ;
#5247=ORIENTED_EDGE ( 'NONE', *, *, #39940, .F. ) ;
#5249=EDGE_CURVE ( 'NONE', #38512, #29237, #13223, .T. ) ;
#5251=CARTESIAN_POINT ( 'NONE',  ( 10.81189881249999729, 0.000000000000000000, -184.3437500020483810 ) ) ;
#5252=CARTESIAN_POINT ( 'NONE',  ( -10.81189881249999729, 1.324075727343319199E-15, -35.09375000204836681 ) ) ;
#5253=CARTESIAN_POINT ( 'NONE',  ( -4.999999999999996447, 8.660254037844387298, -109.8750000040967763 ) ) ;
#5254=CARTESIAN_POINT ( 'NONE',  ( -5.405949406250003975, -9.363379034771801557, -171.3437500020484094 ) ) ;
#5255=CARTESIAN_POINT ( 'NONE',  ( -5.405949406249996869, 9.363379034771805109, -150.8437500020483810 ) ) ;
#5256=CARTESIAN_POINT ( 'NONE',  ( 9.473483644329045106, -5.401111886679669460, 3.466673899897024536E-30 ) ) ;
#5261=CARTESIAN_POINT ( 'NONE',  ( 5.000000000000000000, 8.660254037844385522, -157.7500000000000000 ) ) ;
#5263=CARTESIAN_POINT ( 'NONE',  ( -10.81189881249999729, 1.324075727343319199E-15, -81.59375000204838102 ) ) ;
#5264=CARTESIAN_POINT ( 'NONE',  ( 9.999999999999998224, 0.000000000000000000, -81.87500000409676204 ) ) ;
#5265=CARTESIAN_POINT ( 'NONE',  ( 10.81189881249999729, 0.000000000000000000, -61.53125000204837391 ) ) ;
#5268=CARTESIAN_POINT ( 'NONE',  ( 10.81189881249999907, 6.242252689847868297, -116.9062500020483952 ) ) ;
#5269=CARTESIAN_POINT ( 'NONE',  ( 10.81189881249999551, -6.242252689847874514, -145.6562500020484094 ) ) ;
#5270=CARTESIAN_POINT ( 'NONE',  ( -9.999999999999998224, 1.224646799147353059E-15, -15.12500000409674961 ) ) ;
#5272=CARTESIAN_POINT ( 'NONE',  ( 7.070501591499377789E-16, 11.54700538379251284, -123.5000000040967905 ) ) ;
#5274=ORIENTED_EDGE ( 'NONE', *, *, #538, .T. ) ;
#5277=LINE ( 'NONE', #30975, #31856 ) ;
#5278=CARTESIAN_POINT ( 'NONE',  ( -5.405949406250003975, -9.363379034771801557, -180.5312500020483810 ) ) ;
#5281=CARTESIAN_POINT ( 'NONE',  ( 5.000000000000000000, 8.660254037844385522, -53.12500000409675494 ) ) ;
#5288=CARTESIAN_POINT ( 'NONE',  ( -2.121150477449813534E-15, -11.54700538379251284, -134.7500000040967905 ) ) ;
#5289=CARTESIAN_POINT ( 'NONE',  ( -5.405949406250003975, -9.363379034771801557, -170.0312500020484094 ) ) ;
#5290=CARTESIAN_POINT ( 'NONE',  ( 7.070501591499376803E-16, 11.54700538379251284, -183.5000000040967905 ) ) ;
#5291=CARTESIAN_POINT ( 'NONE',  ( -5.000000000000003553, -8.660254037844383745, -178.0000000000000000 ) ) ;
#5292=ORIENTED_EDGE ( 'NONE', *, *, #356, .T. ) ;
#5293=CARTESIAN_POINT ( 'NONE',  ( -10.00000000000102496, 5.773502691895664007, -84.25000000409676204 ) ) ;
#5294=CARTESIAN_POINT ( 'NONE',  ( -9.999999999999872102, -5.773502691896326589, -194.6250000000000000 ) ) ;
#5295=CARTESIAN_POINT ( 'NONE',  ( -10.00000000000007994, 5.773502691896212013, -195.2500000040968189 ) ) ;
#5296=CARTESIAN_POINT ( 'NONE',  ( -10.81189881249999729, 6.242252689847871849, -78.90625000204838102 ) ) ;
#5297=ORIENTED_EDGE ( 'NONE', *, *, #22828, .F. ) ;
#5299=CARTESIAN_POINT ( 'NONE',  ( -9.999999999999998224, 1.224646799147353059E-15, -29.74999999999997158 ) ) ;
#5302=ORIENTED_EDGE ( 'NONE', *, *, #29746, .T. ) ;
#5303=CARTESIAN_POINT ( 'NONE',  ( -10.81189881249999729, 6.242252689847871849, -35.21875000204835260 ) ) ;
#5304=CARTESIAN_POINT ( 'NONE',  ( -2.121150477449813534E-15, -11.54700538379251284, -170.7500000040968189 ) ) ;
#5305=CARTESIAN_POINT ( 'NONE',  ( 7.644554776091147741E-16, 12.48450537969573659, -5.656250002048358816 ) ) ;
#5306=CARTESIAN_POINT ( 'NONE',  ( -10.81189881249999729, 1.324075727343319199E-15, -56.09375000204835970 ) ) ;
#5309=EDGE_CURVE ( 'NONE', #12174, #41090, #5569, .T. ) ;
#5311=CARTESIAN_POINT ( 'NONE',  ( 10.81189881249999551, -6.242252689847874514, -196.4687500020484094 ) ) ;
#5312=CARTESIAN_POINT ( 'NONE',  ( -10.81189881249999729, 1.324075727343319199E-15, -177.5937500020484094 ) ) ;
#5316=CARTESIAN_POINT ( 'NONE',  ( 9.999999999999998224, 0.000000000000000000, -101.3750000040967905 ) ) ;
#5318=CARTESIAN_POINT ( 'NONE',  ( -2.293366432827344421E-15, -12.48450537969573659, -103.7187500020483668 ) ) ;
#5320=CARTESIAN_POINT ( 'NONE',  ( 10.81189881249999907, 6.242252689847868297, -80.90625000204839523 ) ) ;
#5321=CARTESIAN_POINT ( 'NONE',  ( 7.644554776091147741E-16, 12.48450537969573659, -90.96875000204838102 ) ) ;
#5323=CARTESIAN_POINT ( 'NONE',  ( -10.00000000000000000, -5.773502691896251982, -144.0000000040967905 ) ) ;
#5327=CARTESIAN_POINT ( 'NONE',  ( -9.999999999999998224, 1.224646799147353059E-15, -13.62500000409674961 ) ) ;
#5328=CARTESIAN_POINT ( 'NONE',  ( 10.00000000000012790, 5.773502691896179151, -172.8750000000000000 ) ) ;
#5330=VERTEX_POINT ( 'NONE', #19623 ) ;
#5331=CARTESIAN_POINT ( 'NONE',  ( 5.000000000000000000, 8.660254037844385522, -69.24999999999997158 ) ) ;
#5333=CARTESIAN_POINT ( 'NONE',  ( 5.000000000000000000, 8.660254037844385522, -81.62500000409676204 ) ) ;
#5335=DIRECTION ( 'NONE',  ( -0.000000000000000000, -0.000000000000000000, 1.000000000000000000 ) ) ;
#5337=CARTESIAN_POINT ( 'NONE',  ( -10.81189881249999729, 6.242252689847871849, -74.40625000204836681 ) ) ;
#5339=LINE ( 'NONE', #21949, #22259 ) ;
#5342=CARTESIAN_POINT ( 'NONE',  ( -10.81189881249999729, 6.242252689847871849, -192.9062500020484094 ) ) ;
#5344=CARTESIAN_POINT ( 'NONE',  ( -5.405949406250003975, -9.363379034771801557, -7.843750002048343717 ) ) ;
#5346=CARTESIAN_POINT ( 'NONE',  ( 10.81189881249999551, -6.242252689847874514, -146.9687500020484094 ) ) ;
#5347=CARTESIAN_POINT ( 'NONE',  ( -9.999999999998456346, -5.773502691897145489, -50.62499999999995026 ) ) ;
#5348=PLANE ( 'NONE',  #3164 ) ;
#5349=CARTESIAN_POINT ( 'NONE',  ( 9.999999999999996447, -5.773502691896262640, -171.6250000000000284 ) ) ;
#5350=CARTESIAN_POINT ( 'NONE',  ( 7.070501591499376803E-16, 11.54700538379251284, -176.0000000040967905 ) ) ;
#5351=CARTESIAN_POINT ( 'NONE',  ( -2.293366432827344421E-15, -12.48450537969573659, -102.4062500020483952 ) ) ;
#5352=ORIENTED_EDGE ( 'NONE', *, *, #19995, .F. ) ;
#5353=CARTESIAN_POINT ( 'NONE',  ( 10.00000000000012257, -5.773502691896188921, -161.5000000040968189 ) ) ;
#5354=ORIENTED_EDGE ( 'NONE', *, *, #33499, .F. ) ;
#5355=EDGE_LOOP ( 'NONE', ( #27850, #5544, #28826, #18077 ) ) ;
#5356=( BOUNDED_CURVE ( )  B_SPLINE_CURVE ( 2, ( #9181, #18467, #31875, #11772, #5528, #38961, #41761 ),
 .UNSPECIFIED., .F., .F. ) 
 B_SPLINE_CURVE_WITH_KNOTS ( ( 3, 2, 2, 3 ),
 ( 0.8955223880597017461, 0.8967661691542291313, 0.8980099502487565166, 0.8992537313432839019 ),
 .UNSPECIFIED. ) 
 CURVE ( )  GEOMETRIC_REPRESENTATION_ITEM ( )  RATIONAL_B_SPLINE_CURVE ( ( 0.9999999999999761302, 0.8660254037844625774, 1.000000000000000000, 0.8660254037844387076, 1.000000000000000000, 0.8660254037844028474, 1.000000000000035971 ) ) 
 REPRESENTATION_ITEM ( '' )  );
#5357=CARTESIAN_POINT ( 'NONE',  ( 5.405949406249999534, 9.363379034771803333, -31.28125000204837036 ) ) ;
#5359=CARTESIAN_POINT ( 'NONE',  ( -5.405949406250003975, -9.363379034771801557, -88.84375000204838102 ) ) ;
#5360=CARTESIAN_POINT ( 'NONE',  ( -2.121150477449813534E-15, -11.54700538379251284, -4.250000004096763817 ) ) ;
#5361=EDGE_CURVE ( 'NONE', #24022, #258, #10543, .T. ) ;
#5362=CARTESIAN_POINT ( 'NONE',  ( 5.000000000000000000, 8.660254037844385522, -126.2499999999999716 ) ) ;
#5363=ADVANCED_FACE ( 'NONE', ( #42493 ), #10332, .T. ) ;
#5366=LINE ( 'NONE', #18519, #39817 ) ;
#5368=CARTESIAN_POINT ( 'NONE',  ( 10.00000000000000000, 5.773502691896255534, -8.250000004096751383 ) ) ;
#5369=CYLINDRICAL_SURFACE ( 'NONE', #9484, 9.999999999999998224 ) ;
#5370=CARTESIAN_POINT ( 'NONE',  ( -5.405949406249996869, 9.363379034771805109, -116.3437500020483810 ) ) ;
#5373=CARTESIAN_POINT ( 'NONE',  ( 7.644554776091147741E-16, 12.48450537969573659, -1.156250002048369474 ) ) ;
#5376=CARTESIAN_POINT ( 'NONE',  ( -2.121150477449813534E-15, -11.54700538379251284, -181.2500000040967905 ) ) ;
#5377=CARTESIAN_POINT ( 'NONE',  ( 10.81189881249999729, 6.242252689847867408, -172.4062500020484094 ) ) ;
#5378=CARTESIAN_POINT ( 'NONE',  ( -10.00000000000102496, 5.773502691895664007, -68.87499999999995737 ) ) ;
#5381=CARTESIAN_POINT ( 'NONE',  ( 5.405949406249992428, -9.363379034771808662, -46.59375000204838102 ) ) ;
#5383=CARTESIAN_POINT ( 'NONE',  ( -5.405949406249996869, 9.363379034771805109, -5.531250002048376579 ) ) ;
#5387=CARTESIAN_POINT ( 'NONE',  ( -5.000000000000003553, -8.660254037844383745, -86.49999999999998579 ) ) ;
#5389=CARTESIAN_POINT ( 'NONE',  ( 9.999999999999996447, -5.773502691896262640, -106.0000000040967763 ) ) ;
#5394=CARTESIAN_POINT ( 'NONE',  ( 10.81189881249999729, 0.000000000000000000, -102.0312500020483952 ) ) ;
#5398=CARTESIAN_POINT ( 'NONE',  ( -10.81189881249999907, -6.242252689847864744, -158.1562500020484094 ) ) ;
#5401=EDGE_CURVE ( 'NONE', #23672, #35866, #20422, .T. ) ;
#5402=CARTESIAN_POINT ( 'NONE',  ( -10.00000000000000000, -5.773502691896251982, -19.12499999999997868 ) ) ;
#5404=CARTESIAN_POINT ( 'NONE',  ( 10.81189881249999729, 0.000000000000000000, -28.53125000204837036 ) ) ;
#5405=CARTESIAN_POINT ( 'NONE',  ( -10.00000000000000000, -5.773502691896251982, -151.1250000000000284 ) ) ;
#5406=ADVANCED_FACE ( 'NONE', ( #32808 ), #16584, .T. ) ;
#5407=VECTOR ( 'NONE', #26904, 1000.000000000000000 ) ;
#5410=CARTESIAN_POINT ( 'NONE',  ( 10.81189881249999907, 6.242252689847868297, -125.9062500020483810 ) ) ;
#5411=LINE ( 'NONE', #8222, #7614 ) ;
#5415=VERTEX_POINT ( 'NONE', #3668 ) ;
#5416=CARTESIAN_POINT ( 'NONE',  ( -2.293366432827344421E-15, -12.48450537969573659, -58.90625000204838813 ) ) ;
#5418=CARTESIAN_POINT ( 'NONE',  ( 10.81189881249999551, -6.242252689847874514, -109.4687500020483810 ) ) ;
#5419=ORIENTED_EDGE ( 'NONE', *, *, #29704, .T. ) ;
#5420=VERTEX_POINT ( 'NONE', #22883 ) ;
#5421=CARTESIAN_POINT ( 'NONE',  ( -5.000000000000003553, -8.660254037844383745, -85.37500000409677625 ) ) ;
#5422=CARTESIAN_POINT ( 'NONE',  ( 10.00000000000003020, -5.773502691896243988, -197.5000000040967905 ) ) ;
#5423=CARTESIAN_POINT ( 'NONE',  ( -10.81189881249999729, 1.324075727343319199E-15, -155.0937500020483810 ) ) ;
#5425=CARTESIAN_POINT ( 'NONE',  ( -10.81189881249999729, 6.242252689847871849, -9.718750002048363257 ) ) ;
#5426=CARTESIAN_POINT ( 'NONE',  ( 10.81189881249999729, 6.242252689847867408, -142.2187500020483810 ) ) ;
#5429=CARTESIAN_POINT ( 'NONE',  ( 7.070501591499376803E-16, 11.54700538379251284, -191.0000000040968189 ) ) ;
#5431=CARTESIAN_POINT ( 'NONE',  ( -10.81189881249999729, 1.324075727343319199E-15, -3.593750002048368142 ) ) ;
#5433=CARTESIAN_POINT ( 'NONE',  ( 5.405949406249999534, 9.363379034771803333, -197.7812500020484094 ) ) ;
#5434=CARTESIAN_POINT ( 'NONE',  ( 5.000000000000000000, 8.660254037844385522, -165.6250000040967905 ) ) ;
#5438=CARTESIAN_POINT ( 'NONE',  ( -2.293366432827344421E-15, -12.48450537969573659, -70.71875000204839523 ) ) ;
#5439=CARTESIAN_POINT ( 'NONE',  ( 10.81189881249999907, 6.242252689847868297, -56.71875000204838813 ) ) ;
#5441=CARTESIAN_POINT ( 'NONE',  ( -5.405949406249996869, 9.363379034771805109, -26.53125000204836681 ) ) ;
#5443=CARTESIAN_POINT ( 'NONE',  ( 9.999999999999479527, 5.773502691896553074, -95.25000000409674783 ) ) ;
#5445=CARTESIAN_POINT ( 'NONE',  ( -9.999999999999998224, 5.773502691896259087, -110.8749999999999858 ) ) ;
#5446=CARTESIAN_POINT ( 'NONE',  ( 9.999999999999998224, 0.000000000000000000, -170.0000000000000000 ) ) ;
#5449=CARTESIAN_POINT ( 'NONE',  ( 10.81189881249999551, -6.242252689847874514, -13.65625000204836503 ) ) ;
#5453=LINE ( 'NONE', #3697, #41533 ) ;
#5455=CARTESIAN_POINT ( 'NONE',  ( -5.000000000000003553, -8.660254037844383745, -48.99999999999998579 ) ) ;
#5456=CARTESIAN_POINT ( 'NONE',  ( 5.000000000000000000, 8.660254037844385522, -27.62500000409676204 ) ) ;
#5457=CARTESIAN_POINT ( 'NONE',  ( 4.999999999999992006, -8.660254037844389075, -2.625000004096766926 ) ) ;
#5459=CARTESIAN_POINT ( 'NONE',  ( 4.999999999999992006, -8.660254037844389075, -99.74999999999998579 ) ) ;
#5460=CARTESIAN_POINT ( 'NONE',  ( -5.405949406249996869, 9.363379034771805109, -148.0312500020483810 ) ) ;
#5461=CARTESIAN_POINT ( 'NONE',  ( 10.81189881249999729, 0.000000000000000000, -153.0312500020484094 ) ) ;
#5463=DIRECTION ( 'NONE',  ( -0.000000000000000000, -0.000000000000000000, 1.000000000000000000 ) ) ;
#5464=ORIENTED_EDGE ( 'NONE', *, *, #18255, .F. ) ;
#5466=ORIENTED_EDGE ( 'NONE', *, *, #1000, .T. ) ;
#5467=DIRECTION ( 'NONE',  ( 1.000000000000000000, 0.000000000000000000, 0.000000000000000000 ) ) ;
#5468=CARTESIAN_POINT ( 'NONE',  ( 5.405949406249999534, 9.363379034771803333, -179.5937500020484094 ) ) ;
#5470=CARTESIAN_POINT ( 'NONE',  ( 10.81189881249999729, 0.000000000000000000, -28.34375000204836326 ) ) ;
#5471=CARTESIAN_POINT ( 'NONE',  ( -10.81189881249999729, 6.242252689847871849, -167.2187500020484379 ) ) ;
#5472=CARTESIAN_POINT ( 'NONE',  ( 10.81189881249999907, 6.242252689847868297, -149.7187500020483810 ) ) ;
#5473=DIRECTION ( 'NONE',  ( 1.000000000000000000, 0.000000000000000000, 0.000000000000000000 ) ) ;
#5478=CARTESIAN_POINT ( 'NONE',  ( -10.00000000000076916, 5.773502691895813221, -134.8750000000000000 ) ) ;
#5480=EDGE_CURVE ( 'NONE', #11999, #38843, #6478, .T. ) ;
#5481=CARTESIAN_POINT ( 'NONE',  ( 10.81189881249999551, -6.242252689847874514, -77.96875000204838102 ) ) ;
#5482=CARTESIAN_POINT ( 'NONE',  ( 7.070501591499376803E-16, 11.54700538379251284, -185.0000000040967620 ) ) ;
#5483=CARTESIAN_POINT ( 'NONE',  ( -10.81189881249999729, 6.242252689847871849, -48.90625000204836681 ) ) ;
#5486=CARTESIAN_POINT ( 'NONE',  ( -10.81189881249999729, 1.324075727343319199E-15, -111.7812500020483810 ) ) ;
#5487=CARTESIAN_POINT ( 'NONE',  ( -10.81189881249999729, 6.242252689847871849, -149.4062500020484094 ) ) ;
#5488=CARTESIAN_POINT ( 'NONE',  ( -4.999999999999996447, 8.660254037844387298, -142.8750000040967905 ) ) ;
#5490=CARTESIAN_POINT ( 'NONE',  ( 9.999999999999996447, -5.773502691896262640, -121.0000000040967905 ) ) ;
#5492=ORIENTED_EDGE ( 'NONE', *, *, #7995, .T. ) ;
#5495=CARTESIAN_POINT ( 'NONE',  ( 5.000000000000000000, 8.660254037844385522, -184.7500000000000000 ) ) ;
#5496=CARTESIAN_POINT ( 'NONE',  ( -10.81189881249999729, 6.242252689847871849, -182.4062500020483810 ) ) ;
#5498=CARTESIAN_POINT ( 'NONE',  ( -2.121150477449813534E-15, -11.54700538379251284, -52.25000000409676915 ) ) ;
#5499=DIRECTION ( 'NONE',  ( 1.000000000000000000, 0.000000000000000000, 0.000000000000000000 ) ) ;
#5501=EDGE_CURVE ( 'NONE', #36434, #19099, #24382, .T. ) ;
#5503=CARTESIAN_POINT ( 'NONE',  ( 10.81189881249999551, -6.242252689847874514, -171.1562500020484094 ) ) ;
#5504=CARTESIAN_POINT ( 'NONE',  ( 5.000000000000000000, 8.660254037844385522, -7.749999999999978684 ) ) ;
#5505=CARTESIAN_POINT ( 'NONE',  ( -5.000000000000003553, -8.660254037844383745, -56.49999999999996447 ) ) ;
#5506=ORIENTED_EDGE ( 'NONE', *, *, #14973, .F. ) ;
#5508=DIRECTION ( 'NONE',  ( 1.000000000000000000, 0.000000000000000000, 0.000000000000000000 ) ) ;
#5509=CARTESIAN_POINT ( 'NONE',  ( -10.00000000000076916, 5.773502691895813221, -136.7500000040967620 ) ) ;
#5510=CARTESIAN_POINT ( 'NONE',  ( -10.81189881249999907, -6.242252689847864744, -80.15625000204839523 ) ) ;
#5513=VERTEX_POINT ( 'NONE', #14631 ) ;
#5515=CARTESIAN_POINT ( 'NONE',  ( -10.81189881249999729, 6.242252689847871849, -30.71875000204834905 ) ) ;
#5516=CARTESIAN_POINT ( 'NONE',  ( 9.999999999999998224, 0.000000000000000000, -74.37500000409677625 ) ) ;
#5517=CARTESIAN_POINT ( 'NONE',  ( 10.81189881249999729, 0.000000000000000000, -9.031250002048352599 ) ) ;
#5519=CARTESIAN_POINT ( 'NONE',  ( -5.405949406249996869, 9.363379034771805109, -56.34375000204835970 ) ) ;
#5523=CARTESIAN_POINT ( 'NONE',  ( 10.81189881249999729, 0.000000000000000000, -184.3437500020483810 ) ) ;
#5524=CARTESIAN_POINT ( 'NONE',  ( -10.81189881249999729, 1.324075727343319199E-15, -176.0937500020484094 ) ) ;
#5528=CARTESIAN_POINT ( 'NONE',  ( -4.999999999999996447, 8.660254037844387298, -18.37500000409675494 ) ) ;
#5529=CARTESIAN_POINT ( 'NONE',  ( -2.121150477449813534E-15, -11.54700538379251284, -191.7500000040967905 ) ) ;
#5531=CARTESIAN_POINT ( 'NONE',  ( 10.81189881249999907, 6.242252689847868297, -101.7187500020483810 ) ) ;
#5533=CARTESIAN_POINT ( 'NONE',  ( -10.81189881249999729, 6.242252689847871849, -86.40625000204836681 ) ) ;
#5534=CARTESIAN_POINT ( 'NONE',  ( 7.644554776091147741E-16, 12.48450537969573659, -95.46875000204838102 ) ) ;
#5536=CARTESIAN_POINT ( 'NONE',  ( 4.999999999999992006, -8.660254037844389075, -142.1250000040967905 ) ) ;
#5544=ORIENTED_EDGE ( 'NONE', *, *, #15514, .T. ) ;
#5545=CARTESIAN_POINT ( 'NONE',  ( -9.999999999999998224, 1.224646799147353059E-15, -64.24999999999997158 ) ) ;
#5547=CARTESIAN_POINT ( 'NONE',  ( -9.999999999999998224, 1.224646799147353059E-15, -73.62500000409677625 ) ) ;
#5549=CARTESIAN_POINT ( 'NONE',  ( -2.121150477449813534E-15, -11.54700538379251284, -11.75000000409676737 ) ) ;
#5551=CARTESIAN_POINT ( 'NONE',  ( -5.405949406249996869, 9.363379034771805109, -77.53125000204838102 ) ) ;
#5555=CYLINDRICAL_SURFACE ( 'NONE', #14102, 9.999999999999998224 ) ;
#5556=CARTESIAN_POINT ( 'NONE',  ( -10.81189881249999729, 6.242252689847871849, -191.4062500020484094 ) ) ;
#5557=VECTOR ( 'NONE', #17004, 1000.000000000000000 ) ;
#5560=CARTESIAN_POINT ( 'NONE',  ( -5.405949406249996869, 9.363379034771805109, -2.343750002048366810 ) ) ;
#5561=CARTESIAN_POINT ( 'NONE',  ( 0.000000000000000000, 0.000000000000000000, -200.0000000000000000 ) ) ;
#5562=CARTESIAN_POINT ( 'NONE',  ( -4.999999999999996447, 8.660254037844387298, -192.0000000000000000 ) ) ;
#5563=CARTESIAN_POINT ( 'NONE',  ( 9.999999999999998224, 0.000000000000000000, -35.37500000409676915 ) ) ;
#5564=CARTESIAN_POINT ( 'NONE',  ( -2.121150477449813534E-15, -11.54700538379251284, -177.8750000000000284 ) ) ;
#5565=CARTESIAN_POINT ( 'NONE',  ( 7.644554776091147741E-16, 12.48450537969573659, -103.1562500020483952 ) ) ;
#5566=ORIENTED_EDGE ( 'NONE', *, *, #10403, .F. ) ;
#5568=ORIENTED_EDGE ( 'NONE', *, *, #5896, .F. ) ;
#5569=( BOUNDED_CURVE ( )  B_SPLINE_CURVE ( 2, ( #34401, #17968, #35207, #26749, #30214, #10125, #23090 ),
 .UNSPECIFIED., .F., .F. ) 
 B_SPLINE_CURVE_WITH_KNOTS ( ( 3, 2, 2, 3 ),
 ( 0.9179104477611943480, 0.9191542288557217333, 0.9203980099502490075, 0.9216417910447763928 ),
 .UNSPECIFIED. ) 
 CURVE ( )  GEOMETRIC_REPRESENTATION_ITEM ( )  RATIONAL_B_SPLINE_CURVE ( ( 0.9999999999999641398, 0.8660254037844745678, 1.000000000000000000, 0.8660254037844387076, 1.000000000000000000, 0.8660254037844148378, 1.000000000000023981 ) ) 
 REPRESENTATION_ITEM ( '' )  );
#5571=CARTESIAN_POINT ( 'NONE',  ( -10.81189881249999907, -6.242252689847864744, -30.65625000204835260 ) ) ;
#5573=CARTESIAN_POINT ( 'NONE',  ( 7.644554776091147741E-16, 12.48450537969573659, -77.46875000204838102 ) ) ;
#5575=CARTESIAN_POINT ( 'NONE',  ( -10.81189881249999729, 6.242252689847871849, -198.7187500020484379 ) ) ;
#5579=CARTESIAN_POINT ( 'NONE',  ( -9.999999999999998224, 5.773502691896259087, -13.75000000409676204 ) ) ;
#5581=CARTESIAN_POINT ( 'NONE',  ( -5.405949406249996869, 9.363379034771805109, -128.3437500020484094 ) ) ;
#5583=CARTESIAN_POINT ( 'NONE',  ( 10.81189881249999729, 0.000000000000000000, -116.8437500020483810 ) ) ;
#5587=CARTESIAN_POINT ( 'NONE',  ( -9.999999999999998224, 1.224646799147353059E-15, -172.6250000040968189 ) ) ;
#5588=CARTESIAN_POINT ( 'NONE',  ( 10.81189881249999729, 0.000000000000000000, -172.5312500020484094 ) ) ;
#5589=CARTESIAN_POINT ( 'NONE',  ( 5.000000000000000000, 8.660254037844385522, -69.24999999999997158 ) ) ;
#5592=CARTESIAN_POINT ( 'NONE',  ( 5.405949406249992428, -9.363379034771808662, -48.09375000204838102 ) ) ;
#5594=CARTESIAN_POINT ( 'NONE',  ( 10.81189881249999551, -6.242252689847874514, -6.156250002048360592 ) ) ;
#5596=CARTESIAN_POINT ( 'NONE',  ( 7.070501591499376803E-16, 11.54700538379251284, -6.124999999999964473 ) ) ;
#5598=CARTESIAN_POINT ( 'NONE',  ( 9.999999999999996447, -5.773502691896262640, -86.12499999999998579 ) ) ;
#5600=CARTESIAN_POINT ( 'NONE',  ( -2.121150477449813534E-15, -11.54700538379251284, -101.7500000040967763 ) ) ;
#5603=CARTESIAN_POINT ( 'NONE',  ( -10.81189881249999729, 6.242252689847871849, -96.90625000204839523 ) ) ;
#5606=CARTESIAN_POINT ( 'NONE',  ( -9.999999999999998224, 1.224646799147353059E-15, -4.249999999999976019 ) ) ;
#5607=CARTESIAN_POINT ( 'NONE',  ( -5.405949406249996869, 9.363379034771805109, -154.0312500020484094 ) ) ;
#5610=CARTESIAN_POINT ( 'NONE',  ( 5.000000000000000000, 8.660254037844385522, -16.74999999999996092 ) ) ;
#5611=EDGE_CURVE ( 'NONE', #24501, #24966, #25115, .T. ) ;
#5612=CARTESIAN_POINT ( 'NONE',  ( 10.81189881249999729, 0.000000000000000000, -30.03125000204837036 ) ) ;
#5613=CARTESIAN_POINT ( 'NONE',  ( 9.999999999999996447, -5.773502691896262640, -156.6250000000000000 ) ) ;
#5615=EDGE_CURVE ( 'NONE', #24472, #10661, #15996, .T. ) ;
#5616=AXIS2_PLACEMENT_3D ( 'NONE', #9112, #12744, #9531 ) ;
#5617=( BOUNDED_CURVE ( )  B_SPLINE_CURVE ( 2, ( #23624, #30735, #40624, #11280, #14289, #36769, #7206 ),
 .UNSPECIFIED., .F., .F. ) 
 B_SPLINE_CURVE_WITH_KNOTS ( ( 3, 2, 2, 3 ),
 ( 0.2126865671641791633, 0.2139303482587065208, 0.2151741293532339061, 0.2164179104477612636 ),
 .UNSPECIFIED. ) 
 CURVE ( )  GEOMETRIC_REPRESENTATION_ITEM ( )  RATIONAL_B_SPLINE_CURVE ( ( 0.9999999999999940048, 0.8660254037844447028, 1.000000000000000000, 0.8660254037844387076, 1.000000000000000000, 0.8660254037844297148, 1.000000000000008882 ) ) 
 REPRESENTATION_ITEM ( '' )  );
#5619=CARTESIAN_POINT ( 'NONE',  ( -9.999999999999998224, 5.773502691896259087, -199.3750000000000000 ) ) ;
#5620=CARTESIAN_POINT ( 'NONE',  ( -10.81189881249999907, -6.242252689847864744, -126.6562500020483810 ) ) ;
#5624=( BOUNDED_CURVE ( )  B_SPLINE_CURVE ( 2, ( #36925, #20515, #17057, #33702, #30474, #32278, #903 ),
 .UNSPECIFIED., .F., .F. ) 
 B_SPLINE_CURVE_WITH_KNOTS ( ( 3, 2, 2, 3 ),
 ( 0.4589552238805971740, 0.4601990049751245593, 0.4614427860696518890, 0.4626865671641792743 ),
 .UNSPECIFIED. ) 
 CURVE ( )  GEOMETRIC_REPRESENTATION_ITEM ( )  RATIONAL_B_SPLINE_CURVE ( ( 0.9999999999999820144, 0.8660254037844566932, 1.000000000000000000, 0.8660254037844387076, 1.000000000000000000, 0.8660254037844207220, 1.000000000000017986 ) ) 
 REPRESENTATION_ITEM ( '' )  );
#5625=CARTESIAN_POINT ( 'NONE',  ( 10.81189881249999729, 0.000000000000000000, -55.53125000204836681 ) ) ;
#5627=CIRCLE ( 'NONE', #10431, 9.999999999999998224 ) ;
#5628=CARTESIAN_POINT ( 'NONE',  ( 7.644554776091147741E-16, 12.48450537969573659, -102.9687500020483952 ) ) ;
#5629=ORIENTED_EDGE ( 'NONE', *, *, #32636, .F. ) ;
#5630=ORIENTED_EDGE ( 'NONE', *, *, #23769, .F. ) ;
#5631=EDGE_CURVE ( 'NONE', #22153, #22184, #36443, .T. ) ;
#5633=CARTESIAN_POINT ( 'NONE',  ( 9.999999999999998224, 0.000000000000000000, -197.3750000040967905 ) ) ;
#5634=CARTESIAN_POINT ( 'NONE',  ( -5.405949406250003975, -9.363379034771801557, -160.8437500020484094 ) ) ;
#5636=CARTESIAN_POINT ( 'NONE',  ( 10.81189881249999729, 0.000000000000000000, -7.343750002048343717 ) ) ;
#5638=EDGE_CURVE ( 'NONE', #21857, #21669, #30843, .T. ) ;
#5639=CARTESIAN_POINT ( 'NONE',  ( -5.405949406249996869, 9.363379034771805109, -140.3437500020484094 ) ) ;
#5643=CARTESIAN_POINT ( 'NONE',  ( -5.000000000000003553, -8.660254037844383745, -193.3750000040967905 ) ) ;
#5645=VECTOR ( 'NONE', #18229, 1000.000000000000227 ) ;
#5646=CARTESIAN_POINT ( 'NONE',  ( 5.405949406249992428, -9.363379034771808662, -196.7812500020484094 ) ) ;
#5651=CARTESIAN_POINT ( 'NONE',  ( 10.81189881249999729, 6.242252689847867408, -68.71875000204838102 ) ) ;
#5652=CARTESIAN_POINT ( 'NONE',  ( 5.405949406249992428, -9.363379034771808662, -58.59375000204835970 ) ) ;
#5654=CARTESIAN_POINT ( 'NONE',  ( 10.81189881249999729, 0.000000000000000000, -24.03125000204836681 ) ) ;
#5656=CARTESIAN_POINT ( 'NONE',  ( -10.00000000000051337, 5.773502691895962435, -94.75000000409677625 ) ) ;
#5658=CARTESIAN_POINT ( 'NONE',  ( 10.00000000000000000, 5.773502691896255534, -114.3750000000000000 ) ) ;
#5662=CARTESIAN_POINT ( 'NONE',  ( -10.81189881249999729, -6.242252689847864744, -14.15625000204836503 ) ) ;
#5663=ORIENTED_EDGE ( 'NONE', *, *, #34958, .T. ) ;
#5664=CARTESIAN_POINT ( 'NONE',  ( 4.999999999999992006, -8.660254037844389075, -176.2500000000000284 ) ) ;
#5667=CARTESIAN_POINT ( 'NONE',  ( -10.00000000000000000, -5.773502691896251982, -38.62499999999995737 ) ) ;
#5668=AXIS2_PLACEMENT_3D ( 'NONE', #12172, #21686, #2066 ) ;
#5669=CARTESIAN_POINT ( 'NONE',  ( 7.070501591499377789E-16, 11.54700538379251284, -29.00000000409675494 ) ) ;
#5670=ADVANCED_FACE ( 'NONE', ( #4087 ), #30428, .T. ) ;
#5671=CARTESIAN_POINT ( 'NONE',  ( -10.81189881249999729, 1.324075727343319199E-15, -54.78125000204836681 ) ) ;
#5672=FACE_OUTER_BOUND ( 'NONE', #17159, .T. ) ;
#5674=EDGE_CURVE ( 'NONE', #10661, #15576, #2554, .T. ) ;
#5675=CARTESIAN_POINT ( 'NONE',  ( 5.000000000000000000, 8.660254037844385522, -24.24999999999996447 ) ) ;
#5676=CARTESIAN_POINT ( 'NONE',  ( 10.81189881249999729, 0.000000000000000000, -144.0312500020483810 ) ) ;
#5677=EDGE_CURVE ( 'NONE', #27845, #32468, #26486, .T. ) ;
#5678=CARTESIAN_POINT ( 'NONE',  ( -2.293366432827344421E-15, -12.48450537969573659, -148.9062500020483810 ) ) ;
#5679=CARTESIAN_POINT ( 'NONE',  ( 9.999999999998969713, 5.773502691896851502, -78.75000000409674783 ) ) ;
#5681=CARTESIAN_POINT ( 'NONE',  ( -9.999999999999998224, 1.224646799147353059E-15, -31.24999999999997158 ) ) ;
#5682=EDGE_LOOP ( 'NONE', ( #1759, #20073, #33063, #21543 ) ) ;
#5687=CARTESIAN_POINT ( 'NONE',  ( -5.000000000000003553, -8.660254037844383745, -100.3750000040967905 ) ) ;
#5688=CARTESIAN_POINT ( 'NONE',  ( -10.81189881249999907, -6.242252689847864744, -178.9687500020484094 ) ) ;
#5689=AXIS2_PLACEMENT_3D ( 'NONE', #32372, #15079, #25677 ) ;
#5690=CARTESIAN_POINT ( 'NONE',  ( -10.81189881249999907, -6.242252689847864744, -33.46875000204834549 ) ) ;
#5692=CARTESIAN_POINT ( 'NONE',  ( 10.81189881249999729, 0.000000000000000000, -163.3437500020484094 ) ) ;
#5693=CARTESIAN_POINT ( 'NONE',  ( 5.405949406249992428, -9.363379034771808662, -154.5937500020483810 ) ) ;
#5694=CARTESIAN_POINT ( 'NONE',  ( 9.999999999999998224, 0.000000000000000000, -65.37500000409676204 ) ) ;
#5700=CARTESIAN_POINT ( 'NONE',  ( 5.000000000000000000, 8.660254037844385522, -33.62500000409676915 ) ) ;
#5702=CARTESIAN_POINT ( 'NONE',  ( -10.81189881249999907, -6.242252689847864744, -82.96875000204836681 ) ) ;
#5703=DIRECTION ( 'NONE',  ( 1.000000000000000000, 0.000000000000000000, 0.000000000000000000 ) ) ;
#5704=CARTESIAN_POINT ( 'NONE',  ( -5.405949406250003975, -9.363379034771801557, -53.03125000204836681 ) ) ;
#5705=CYLINDRICAL_SURFACE ( 'NONE', #13000, 9.999999999999998224 ) ;
#5707=CARTESIAN_POINT ( 'NONE',  ( 10.00000000000000000, 5.773502691896255534, -139.8750000000000000 ) ) ;
#5708=CARTESIAN_POINT ( 'NONE',  ( -10.81189881249999729, 1.324075727343319199E-15, -143.2812500020483810 ) ) ;
#5709=CARTESIAN_POINT ( 'NONE',  ( 23.09401076758504345, 1.040834085586084257E-14, 45.00000000000009237 ) ) ;
#5711=CARTESIAN_POINT ( 'NONE',  ( -5.000000000000003553, -8.660254037844383745, -125.8750000040967905 ) ) ;
#5713=ORIENTED_EDGE ( 'NONE', *, *, #36231, .T. ) ;
#5716=CARTESIAN_POINT ( 'NONE',  ( -2.121150477449813534E-15, -11.54700538379251284, -22.25000000409676915 ) ) ;
#5717=CARTESIAN_POINT ( 'NONE',  ( 10.81189881249999551, -6.242252689847874514, -172.6562500020484379 ) ) ;
#5718=CARTESIAN_POINT ( 'NONE',  ( 5.000000000000000000, 8.660254037844385522, -50.12500000409675494 ) ) ;
#5719=CYLINDRICAL_SURFACE ( 'NONE', #14547, 9.999999999999998224 ) ;
#5721=CARTESIAN_POINT ( 'NONE',  ( -9.999999999999998224, 1.224646799147353059E-15, -31.24999999999997158 ) ) ;
#5722=CARTESIAN_POINT ( 'NONE',  ( -2.293366432827344421E-15, -12.48450537969573659, -166.9062500020483810 ) ) ;
#5723=VECTOR ( 'NONE', #28446, 1000.000000000000000 ) ;
#5724=CARTESIAN_POINT ( 'NONE',  ( -9.999999999998969713, -5.773502691896847949, -34.50000000409672651 ) ) ;
#5725=VERTEX_POINT ( 'NONE', #18306 ) ;
#5726=CARTESIAN_POINT ( 'NONE',  ( -9.999999999998969713, -5.773502691896847949, -1.124999999999947597 ) ) ;
#5727=CARTESIAN_POINT ( 'NONE',  ( -10.00000000000154188, 5.773502691895366468, -26.87499999999993960 ) ) ;
#5728=ADVANCED_FACE ( 'NONE', ( #12251 ), #5369, .T. ) ;
#5729=CARTESIAN_POINT ( 'NONE',  ( 7.644554776091147741E-16, 12.48450537969573659, -74.65625000204838102 ) ) ;
#5730=VERTEX_POINT ( 'NONE', #18734 ) ;
#5732=ORIENTED_EDGE ( 'NONE', *, *, #9584, .F. ) ;
#5733=VERTEX_POINT ( 'NONE', #38807 ) ;
#5734=( BOUNDED_CURVE ( )  B_SPLINE_CURVE ( 2, ( #17956, #37401, #4598, #30931, #6098, #28978, #8487 ),
 .UNSPECIFIED., .F., .F. ) 
 B_SPLINE_CURVE_WITH_KNOTS ( ( 3, 2, 2, 3 ),
 ( 0.04477611940298512061, 0.04601990049751248507, 0.04726368159203984259, 0.04850746268656720706 ),
 .UNSPECIFIED. ) 
 CURVE ( )  GEOMETRIC_REPRESENTATION_ITEM ( )  RATIONAL_B_SPLINE_CURVE ( ( 0.9999999999999947820, 0.8660254037844439257, 1.000000000000000000, 0.8660254037844387076, 1.000000000000000000, 0.8660254037844342667, 1.000000000000004441 ) ) 
 REPRESENTATION_ITEM ( '' )  );
#5735=CARTESIAN_POINT ( 'NONE',  ( 7.644554776091147741E-16, 12.48450537969573659, -32.46875000204835970 ) ) ;
#5736=CARTESIAN_POINT ( 'NONE',  ( 10.81189881249999907, 6.242252689847868297, -4.406250002048352599 ) ) ;
#5737=CARTESIAN_POINT ( 'NONE',  ( 5.405949406249992428, -9.363379034771808662, -57.09375000204835970 ) ) ;
#5738=EDGE_LOOP ( 'NONE', ( #4208, #28085, #9434, #17525 ) ) ;
#5741=CARTESIAN_POINT ( 'NONE',  ( 10.81189881249999551, -6.242252689847874514, -190.4687500020484094 ) ) ;
#5742=CARTESIAN_POINT ( 'NONE',  ( 5.405949406249999534, 9.363379034771803333, -176.5937500020484094 ) ) ;
#5745=CARTESIAN_POINT ( 'NONE',  ( -5.000000000000003553, -8.660254037844383745, -75.99999999999998579 ) ) ;
#5748=CARTESIAN_POINT ( 'NONE',  ( 5.405949406249999534, 9.363379034771803333, -104.5937500020483810 ) ) ;
#5749=CYLINDRICAL_SURFACE ( 'NONE', #7963, 9.999999999999998224 ) ;
#5750=CARTESIAN_POINT ( 'NONE',  ( 5.405949406249992428, -9.363379034771808662, -72.28125000204838102 ) ) ;
#5751=CARTESIAN_POINT ( 'NONE',  ( 10.81189881249999551, -6.242252689847874514, -89.96875000204838102 ) ) ;
#5753=CARTESIAN_POINT ( 'NONE',  ( -2.121150477449813534E-15, -11.54700538379251284, -145.2500000040967905 ) ) ;
#5758=CARTESIAN_POINT ( 'NONE',  ( -11.54700538379250396, -20.00000000000000355, 49.99999999999998579 ) ) ;
#5761=ORIENTED_EDGE ( 'NONE', *, *, #4288, .F. ) ;
#5762=CARTESIAN_POINT ( 'NONE',  ( 9.999999999999998224, 0.000000000000000000, -64.99999999999997158 ) ) ;
#5764=CARTESIAN_POINT ( 'NONE',  ( 7.070501591499377789E-16, 11.54700538379251284, -74.00000000409677625 ) ) ;
#5765=CARTESIAN_POINT ( 'NONE',  ( -9.999999999999998224, 1.224646799147353059E-15, -47.74999999999998579 ) ) ;
#5766=LINE ( 'NONE', #31897, #1060 ) ;
#5768=CARTESIAN_POINT ( 'NONE',  ( 5.405949406249992428, -9.363379034771808662, -69.28125000204838102 ) ) ;
#5770=CARTESIAN_POINT ( 'NONE',  ( -9.999999999999998224, 1.224646799147353059E-15, -200.0000000000000000 ) ) ;
#5772=CARTESIAN_POINT ( 'NONE',  ( 9.999999999998969713, 5.773502691896851502, -47.25000000409674072 ) ) ;
#5773=CARTESIAN_POINT ( 'NONE',  ( 5.405949406249999534, 9.363379034771803333, -194.7812500020484094 ) ) ;
#5775=CARTESIAN_POINT ( 'NONE',  ( 10.81189881249999729, 6.242252689847867408, -2.718750002048361480 ) ) ;
#5776=CARTESIAN_POINT ( 'NONE',  ( 10.00000000000076916, -5.773502691895816774, -110.5000000040967763 ) ) ;
#5777=CARTESIAN_POINT ( 'NONE',  ( -2.121150477449813534E-15, -11.54700538379251284, -107.7500000040967763 ) ) ;
#5778=CARTESIAN_POINT ( 'NONE',  ( 9.999999999999998224, 0.000000000000000000, -173.0000000000000284 ) ) ;
#5779=CARTESIAN_POINT ( 'NONE',  ( 9.999999999999996447, -5.773502691896262640, -174.6250000000000000 ) ) ;
#5780=FACE_OUTER_BOUND ( 'NONE', #2693, .T. ) ;
#5781=CARTESIAN_POINT ( 'NONE',  ( -10.81189881249999907, -6.242252689847864744, -105.6562500020483952 ) ) ;
#5782=ORIENTED_EDGE ( 'NONE', *, *, #3528, .F. ) ;
#5783=CARTESIAN_POINT ( 'NONE',  ( 0.000000000000000000, 0.000000000000000000, -200.0000000000000000 ) ) ;
#5784=VERTEX_POINT ( 'NONE', #2565 ) ;
#5786=CARTESIAN_POINT ( 'NONE',  ( 10.81189881249999551, -6.242252689847874514, -27.15625000204838102 ) ) ;
#5788=CARTESIAN_POINT ( 'NONE',  ( 10.81189881249999729, 0.000000000000000000, -82.34375000204836681 ) ) ;
#5791=CARTESIAN_POINT ( 'NONE',  ( 7.644554776091147741E-16, 12.48450537969573659, -197.4687500020484094 ) ) ;
#5792=CARTESIAN_POINT ( 'NONE',  ( 4.999999999999992006, -8.660254037844389075, -130.1250000040967620 ) ) ;
#5793=CARTESIAN_POINT ( 'NONE',  ( -9.999999999999998224, 1.224646799147353059E-15, -16.62500000409675138 ) ) ;
#5795=CARTESIAN_POINT ( 'NONE',  ( 10.00000000000000000, 5.773502691896255534, -12.75000000409675671 ) ) ;
#5797=CARTESIAN_POINT ( 'NONE',  ( 10.81189881249999551, -6.242252689847874514, -127.4687500020483810 ) ) ;
#5798=CARTESIAN_POINT ( 'NONE',  ( -10.81189881249999729, -6.242252689847864744, -117.4687500020483810 ) ) ;
#5801=CARTESIAN_POINT ( 'NONE',  ( -5.000000000000003553, -8.660254037844383745, -167.8750000040967905 ) ) ;
#5805=CARTESIAN_POINT ( 'NONE',  ( -10.81189881249999729, -6.242252689847864744, -43.96875000204835970 ) ) ;
#5807=CARTESIAN_POINT ( 'NONE',  ( 10.81189881249999551, -6.242252689847874514, -4.656250002048353487 ) ) ;
#5811=CARTESIAN_POINT ( 'NONE',  ( -5.000000000000003553, -8.660254037844383745, -90.99999999999998579 ) ) ;
#5813=CARTESIAN_POINT ( 'NONE',  ( -10.00000000000000000, -5.773502691896251982, -102.0000000040967905 ) ) ;
#5814=CYLINDRICAL_SURFACE ( 'NONE', #9289, 9.999999999999998224 ) ;
#5816=CARTESIAN_POINT ( 'NONE',  ( -10.81189881249999729, 6.242252689847871849, -95.40625000204838102 ) ) ;
#5817=ORIENTED_EDGE ( 'NONE', *, *, #28585, .T. ) ;
#5819=CARTESIAN_POINT ( 'NONE',  ( -4.999999999999996447, 8.660254037844387298, -71.99999999999998579 ) ) ;
#5820=CARTESIAN_POINT ( 'NONE',  ( -10.81189881249999729, 1.324075727343319199E-15, -156.7812500020484094 ) ) ;
#5822=ORIENTED_EDGE ( 'NONE', *, *, #26747, .T. ) ;
#5823=CARTESIAN_POINT ( 'NONE',  ( -9.999999999999998224, 5.773502691896259087, -20.87499999999996803 ) ) ;
#5824=CARTESIAN_POINT ( 'NONE',  ( 10.81189881249999551, -6.242252689847874514, -31.65625000204835260 ) ) ;
#5825=CARTESIAN_POINT ( 'NONE',  ( 9.999999999999996447, -5.773502691896262640, -153.6250000000000284 ) ) ;
#5826=( BOUNDED_CURVE ( )  B_SPLINE_CURVE ( 2, ( #24897, #38046, #21855, #35034, #2238, #15362, #38467 ),
 .UNSPECIFIED., .F., .F. ) 
 B_SPLINE_CURVE_WITH_KNOTS ( ( 3, 2, 2, 3 ),
 ( 0.3544776119402986980, 0.3557213930348260278, 0.3569651741293533576, 0.3582089552238806873 ),
 .UNSPECIFIED. ) 
 CURVE ( )  GEOMETRIC_REPRESENTATION_ITEM ( )  RATIONAL_B_SPLINE_CURVE ( ( 0.9999999999999820144, 0.8660254037844566932, 1.000000000000000000, 0.8660254037844387076, 1.000000000000000000, 0.8660254037844267172, 1.000000000000011990 ) ) 
 REPRESENTATION_ITEM ( '' )  );
#5828=CARTESIAN_POINT ( 'NONE',  ( -10.00000000000000000, -5.773502691896251982, -197.6250000000000284 ) ) ;
#5829=CARTESIAN_POINT ( 'NONE',  ( 5.405949406249999534, 9.363379034771803333, -125.7812500020483668 ) ) ;
#5831=CARTESIAN_POINT ( 'NONE',  ( 9.999999999998969713, 5.773502691896851502, -65.25000000409676204 ) ) ;
#5833=CARTESIAN_POINT ( 'NONE',  ( 10.81189881249999729, 0.000000000000000000, -51.03125000204835970 ) ) ;
#5835=CARTESIAN_POINT ( 'NONE',  ( -5.405949406249996869, 9.363379034771805109, -105.8437500020483810 ) ) ;
#5836=VERTEX_POINT ( 'NONE', #29103 ) ;
#5837=ORIENTED_EDGE ( 'NONE', *, *, #36120, .F. ) ;
#5838=CARTESIAN_POINT ( 'NONE',  ( 0.000000000000000000, 0.000000000000000000, -200.0000000000000000 ) ) ;
#5840=CARTESIAN_POINT ( 'NONE',  ( -2.293366432827344421E-15, -12.48450537969573659, -156.2187500020483810 ) ) ;
#5842=CARTESIAN_POINT ( 'NONE',  ( 10.81189881249999729, 0.000000000000000000, -8.843750002048345493 ) ) ;
#5844=EDGE_CURVE ( 'NONE', #38940, #33541, #19043, .T. ) ;
#5845=CARTESIAN_POINT ( 'NONE',  ( -10.81189881249999729, 1.324075727343319199E-15, -143.0937500020483810 ) ) ;
#5848=CARTESIAN_POINT ( 'NONE',  ( 9.999999999999998224, 0.000000000000000000, -200.0000000000000000 ) ) ;
#5850=CARTESIAN_POINT ( 'NONE',  ( 4.999999999999992006, -8.660254037844389075, -196.1250000040967905 ) ) ;
#5852=CARTESIAN_POINT ( 'NONE',  ( 10.81189881249999729, 0.000000000000000000, -192.0312500020484094 ) ) ;
#5857=CARTESIAN_POINT ( 'NONE',  ( 10.81189881249999551, -6.242252689847874514, -67.46875000204838102 ) ) ;
#5858=CARTESIAN_POINT ( 'NONE',  ( 5.405949406249999534, 9.363379034771803333, -55.09375000204835970 ) ) ;
#5860=CARTESIAN_POINT ( 'NONE',  ( -2.293366432827344421E-15, -12.48450537969573659, -30.40625000204834905 ) ) ;
#5862=CARTESIAN_POINT ( 'NONE',  ( -9.999999999999998224, 1.224646799147353059E-15, -21.12500000409675494 ) ) ;
#5864=CARTESIAN_POINT ( 'NONE',  ( 10.00000000000000000, 5.773502691896255534, -109.8750000000000000 ) ) ;
#5868=CARTESIAN_POINT ( 'NONE',  ( -10.81189881249999729, -6.242252689847864744, -114.6562500020483952 ) ) ;
#5869=ORIENTED_EDGE ( 'NONE', *, *, #26514, .T. ) ;
#5870=( BOUNDED_CURVE ( )  B_SPLINE_CURVE ( 2, ( #41313, #24737, #37884, #1856, #34870, #5293, #2069 ),
 .UNSPECIFIED., .F., .F. ) 
 B_SPLINE_CURVE_WITH_KNOTS ( ( 3, 2, 2, 3 ),
 ( 0.5671641791044778058, 0.5684079601990051911, 0.5696517412935325764, 0.5708955223880599616 ),
 .UNSPECIFIED. ) 
 CURVE ( )  GEOMETRIC_REPRESENTATION_ITEM ( )  RATIONAL_B_SPLINE_CURVE ( ( 0.9999999999999761302, 0.8660254037844625774, 1.000000000000000000, 0.8660254037844387076, 1.000000000000000000, 0.8660254037844148378, 1.000000000000023981 ) ) 
 REPRESENTATION_ITEM ( '' )  );
#5871=CARTESIAN_POINT ( 'NONE',  ( -10.00000000000005329, 5.773502691896226224, -196.7500000040968757 ) ) ;
#5875=CARTESIAN_POINT ( 'NONE',  ( -9.999999999999998224, 1.224646799147353059E-15, -43.24999999999998579 ) ) ;
#5876=CARTESIAN_POINT ( 'NONE',  ( -9.999999999999998224, 1.224646799147353059E-15, -27.12500000409676204 ) ) ;
#5877=CARTESIAN_POINT ( 'NONE',  ( 7.644554776091147741E-16, 12.48450537969573659, -52.15625000204838102 ) ) ;
#5880=( BOUNDED_CURVE ( )  B_SPLINE_CURVE ( 2, ( #6266, #21812, #5421, #26326, #33015, #20471, #10120 ),
 .UNSPECIFIED., .F., .F. ) 
 B_SPLINE_CURVE_WITH_KNOTS ( ( 3, 2, 2, 3 ),
 ( 0.5634328358208957610, 0.5646766169154231463, 0.5659203980099504205, 0.5671641791044778058 ),
 .UNSPECIFIED. ) 
 CURVE ( )  GEOMETRIC_REPRESENTATION_ITEM ( )  RATIONAL_B_SPLINE_CURVE ( ( 0.9999999999999761302, 0.8660254037844625774, 1.000000000000000000, 0.8660254037844387076, 1.000000000000000000, 0.8660254037844148378, 1.000000000000023981 ) ) 
 REPRESENTATION_ITEM ( '' )  );
#5881=CARTESIAN_POINT ( 'NONE',  ( -5.000000000000003553, -8.660254037844383745, -105.9999999999999858 ) ) ;
#5882=CARTESIAN_POINT ( 'NONE',  ( -5.405949406249996869, 9.363379034771805109, -145.0312500020483810 ) ) ;
#5883=CARTESIAN_POINT ( 'NONE',  ( -5.405949406249996869, 9.363379034771805109, -149.5312500020483810 ) ) ;
#5885=CARTESIAN_POINT ( 'NONE',  ( -9.999999999999998224, 1.224646799147353059E-15, -200.0000000000000000 ) ) ;
#5886=ORIENTED_EDGE ( 'NONE', *, *, #8126, .T. ) ;
#5888=ORIENTED_EDGE ( 'NONE', *, *, #40899, .F. ) ;
#5889=CARTESIAN_POINT ( 'NONE',  ( 10.00000000000051159, -5.773502691895965988, -100.0000000040968047 ) ) ;
#5890=CARTESIAN_POINT ( 'NONE',  ( 5.405949406249999534, 9.363379034771803333, -185.5937500020483810 ) ) ;
#5891=CARTESIAN_POINT ( 'NONE',  ( 10.81189881249999907, 6.242252689847868297, -31.21875000204835260 ) ) ;
#5892=CARTESIAN_POINT ( 'NONE',  ( -4.999999999999996447, 8.660254037844387298, -118.5000000000000000 ) ) ;
#5894=CARTESIAN_POINT ( 'NONE',  ( -5.405949406249996869, 9.363379034771805109, -161.3437500020484094 ) ) ;
#5895=CARTESIAN_POINT ( 'NONE',  ( 10.81189881249999907, 6.242252689847868297, -151.2187500020483810 ) ) ;
#5896=EDGE_CURVE ( 'NONE', #23620, #3659, #24860, .T. ) ;
#5897=CARTESIAN_POINT ( 'NONE',  ( 10.10436387341741948, -4.101143746035988968, 1.152242674263551285E-14 ) ) ;
#5901=CARTESIAN_POINT ( 'NONE',  ( -10.81189881249999729, 1.324075727343319199E-15, -17.09375000204835260 ) ) ;
#5904=CYLINDRICAL_SURFACE ( 'NONE', #32299, 9.999999999999998224 ) ;
#5905=CARTESIAN_POINT ( 'NONE',  ( 9.999999999999998224, 0.000000000000000000, -70.99999999999998579 ) ) ;
#5907=CARTESIAN_POINT ( 'NONE',  ( -10.81189881249999729, 6.242252689847871849, -81.71875000204838102 ) ) ;
#5909=CARTESIAN_POINT ( 'NONE',  ( -10.81189881249999729, 1.324075727343319199E-15, -50.28125000204835970 ) ) ;
#5913=CARTESIAN_POINT ( 'NONE',  ( -2.121150477449813534E-15, -11.54700538379251284, -135.8750000000000000 ) ) ;
#5914=AXIS2_PLACEMENT_3D ( 'NONE', #41951, #22121, #28399 ) ;
#5915=CARTESIAN_POINT ( 'NONE',  ( 10.81189881249999729, 6.242252689847867408, -148.4062500020484094 ) ) ;
#5917=CARTESIAN_POINT ( 'NONE',  ( 9.999999999999479527, 5.773502691896553074, -143.2500000040967905 ) ) ;
#5918=CARTESIAN_POINT ( 'NONE',  ( 7.070501591499377789E-16, 11.54700538379251284, -120.5000000040967905 ) ) ;
#5920=EDGE_LOOP ( 'NONE', ( #19867, #7524, #23507, #21156 ) ) ;
#5923=CARTESIAN_POINT ( 'NONE',  ( 9.999999999999998224, 0.000000000000000000, -84.87500000409677625 ) ) ;
#5924=CARTESIAN_POINT ( 'NONE',  ( 10.81189881249999729, 0.000000000000000000, -175.5312500020483810 ) ) ;
#5925=CARTESIAN_POINT ( 'NONE',  ( 5.000000000000000000, 8.660254037844385522, -51.62500000409675494 ) ) ;
#5926=CARTESIAN_POINT ( 'NONE',  ( -9.999999999999998224, 1.224646799147353059E-15, -98.74999999999998579 ) ) ;
#5928=CARTESIAN_POINT ( 'NONE',  ( 9.999999999999998224, 0.000000000000000000, -9.875000004096746054 ) ) ;
#5929=CARTESIAN_POINT ( 'NONE',  ( 10.81189881249999907, 6.242252689847868297, -169.4062500020484094 ) ) ;
#5930=EDGE_CURVE ( 'NONE', #34292, #1053, #14353, .T. ) ;
#5931=CARTESIAN_POINT ( 'NONE',  ( 5.000000000000000000, 8.660254037844385522, -183.6250000040967905 ) ) ;
#5932=FACE_OUTER_BOUND ( 'NONE', #16627, .T. ) ;
#5933=ORIENTED_EDGE ( 'NONE', *, *, #3546, .T. ) ;
#5934=CARTESIAN_POINT ( 'NONE',  ( -9.999999999999998224, 1.224646799147353059E-15, -123.1250000040967905 ) ) ;
#5936=VECTOR ( 'NONE', #25218, 1000.000000000000000 ) ;
#5937=CARTESIAN_POINT ( 'NONE',  ( 9.999999999999998224, 0.000000000000000000, -137.3750000040967905 ) ) ;
#5938=CARTESIAN_POINT ( 'NONE',  ( 10.81189881249999907, 6.242252689847868297, -79.40625000204839523 ) ) ;
#5939=VERTEX_POINT ( 'NONE', #41606 ) ;
#5941=DIRECTION ( 'NONE',  ( -0.000000000000000000, -0.000000000000000000, 1.000000000000000000 ) ) ;
#5942=ORIENTED_EDGE ( 'NONE', *, *, #20424, .F. ) ;
#5943=VECTOR ( 'NONE', #21330, 999.9999999999998863 ) ;
#5944=( BOUNDED_CURVE ( )  B_SPLINE_CURVE ( 2, ( #14937, #41269, #34189, #17322, #11707, #21213, #37621 ),
 .UNSPECIFIED., .F., .F. ) 
 B_SPLINE_CURVE_WITH_KNOTS ( ( 3, 2, 2, 3 ),
 ( 0.2649253731343284568, 0.2661691542288558421, 0.2674129353233831718, 0.2686567164179105571 ),
 .UNSPECIFIED. ) 
 CURVE ( )  GEOMETRIC_REPRESENTATION_ITEM ( )  RATIONAL_B_SPLINE_CURVE ( ( 0.9999999999999880096, 0.8660254037844506980, 1.000000000000000000, 0.8660254037844387076, 1.000000000000000000, 0.8660254037844267172, 1.000000000000011990 ) ) 
 REPRESENTATION_ITEM ( '' )  );
#5945=ORIENTED_EDGE ( 'NONE', *, *, #2764, .F. ) ;
#5946=CARTESIAN_POINT ( 'NONE',  ( 10.81189881249999551, -6.242252689847874514, -26.96875000204837747 ) ) ;
#5947=CARTESIAN_POINT ( 'NONE',  ( 9.999999999999998224, 0.000000000000000000, -159.5000000000000000 ) ) ;
#5948=CARTESIAN_POINT ( 'NONE',  ( -5.405949406249996869, 9.363379034771805109, -5.531250002048376579 ) ) ;
#5949=CARTESIAN_POINT ( 'NONE',  ( 5.405949406249992428, -9.363379034771808662, -52.59375000204835260 ) ) ;
#5950=EDGE_LOOP ( 'NONE', ( #25169, #34075, #32926, #26843 ) ) ;
#5951=CARTESIAN_POINT ( 'NONE',  ( 4.999999999999992006, -8.660254037844389075, -3.749999999999975575 ) ) ;
#5953=CARTESIAN_POINT ( 'NONE',  ( 5.405949406249992428, -9.363379034771808662, -190.5937500020484094 ) ) ;
#5954=CARTESIAN_POINT ( 'NONE',  ( 5.405949406249992428, -9.363379034771808662, -177.0937500020484094 ) ) ;
#5957=CARTESIAN_POINT ( 'NONE',  ( 9.999999999999998224, 0.000000000000000000, -125.0000000000000000 ) ) ;
#5958=CARTESIAN_POINT ( 'NONE',  ( 10.00000000000051159, -5.773502691895965988, -101.5000000040967763 ) ) ;
#5960=CARTESIAN_POINT ( 'NONE',  ( 5.405949406249992428, -9.363379034771808662, -108.0937500020483810 ) ) ;
#5961=CARTESIAN_POINT ( 'NONE',  ( 7.644554776091147741E-16, 12.48450537969573659, -77.65625000204838102 ) ) ;
#5962=CARTESIAN_POINT ( 'NONE',  ( 10.81189881249999551, -6.242252689847874514, -85.46875000204836681 ) ) ;
#5965=CARTESIAN_POINT ( 'NONE',  ( -9.999999999999998224, 1.224646799147353059E-15, -147.1250000040967905 ) ) ;
#5970=EDGE_CURVE ( 'NONE', #2425, #39731, #6941, .T. ) ;
#5971=CARTESIAN_POINT ( 'NONE',  ( 10.81189881249999907, 6.242252689847868297, -199.4062500020484094 ) ) ;
#5972=CARTESIAN_POINT ( 'NONE',  ( -5.000000000000003553, -8.660254037844383745, -51.99999999999996447 ) ) ;
#5974=VERTEX_POINT ( 'NONE', #39636 ) ;
#5975=CARTESIAN_POINT ( 'NONE',  ( 5.000000000000000000, 8.660254037844385522, -64.74999999999997158 ) ) ;
#5977=CARTESIAN_POINT ( 'NONE',  ( -5.000000000000003553, -8.660254037844383745, -76.37500000409677625 ) ) ;
#5978=CARTESIAN_POINT ( 'NONE',  ( 0.000000000000000000, 0.000000000000000000, -200.0000000000000000 ) ) ;
#5979=LINE ( 'NONE', #41996, #30034 ) ;
#5981=CARTESIAN_POINT ( 'NONE',  ( 7.644554776091147741E-16, 12.48450537969573659, -68.65625000204840944 ) ) ;
#5984=VERTEX_POINT ( 'NONE', #20000 ) ;
#5985=CARTESIAN_POINT ( 'NONE',  ( 5.405949406249992428, -9.363379034771808662, -189.2812500020484094 ) ) ;
#5987=CARTESIAN_POINT ( 'NONE',  ( -2.293366432827344421E-15, -12.48450537969573659, -3.218750002048363257 ) ) ;
#5989=CARTESIAN_POINT ( 'NONE',  ( -9.999999999999998224, 1.224646799147353059E-15, -181.2500000000000284 ) ) ;
#5990=CARTESIAN_POINT ( 'NONE',  ( 9.999999999999998224, 0.000000000000000000, -155.3750000040967905 ) ) ;
#5991=( BOUNDED_CURVE ( )  B_SPLINE_CURVE ( 2, ( #22073, #5243, #18612, #15991, #21854, #19245, #2437 ),
 .UNSPECIFIED., .F., .F. ) 
 B_SPLINE_CURVE_WITH_KNOTS ( ( 3, 2, 2, 3 ),
 ( 0.6679104477611942370, 0.6691542288557216223, 0.6703980099502490075, 0.6716417910447763928 ),
 .UNSPECIFIED. ) 
 CURVE ( )  GEOMETRIC_REPRESENTATION_ITEM ( )  RATIONAL_B_SPLINE_CURVE ( ( 0.9999999999999761302, 0.8660254037844625774, 1.000000000000000000, 0.8660254037844387076, 1.000000000000000000, 0.8660254037844148378, 1.000000000000023981 ) ) 
 REPRESENTATION_ITEM ( '' )  );
#5992=CARTESIAN_POINT ( 'NONE',  ( 10.00000000000000000, 5.773502691896255534, -174.3750000000000000 ) ) ;
#5993=CARTESIAN_POINT ( 'NONE',  ( 9.999999999999998224, 0.000000000000000000, -116.3750000040967905 ) ) ;
#5994=CARTESIAN_POINT ( 'NONE',  ( 5.405949406249999534, 9.363379034771803333, -104.7812500020483810 ) ) ;
#5995=ORIENTED_EDGE ( 'NONE', *, *, #33288, .T. ) ;
#5996=DIRECTION ( 'NONE',  ( 1.000000000000000000, 0.000000000000000000, 0.000000000000000000 ) ) ;
#5997=ORIENTED_EDGE ( 'NONE', *, *, #6781, .F. ) ;
#5998=VERTEX_POINT ( 'NONE', #22617 ) ;
#5999=CARTESIAN_POINT ( 'NONE',  ( -5.405949406250003975, -9.363379034771801557, -26.03125000204836681 ) ) ;
#6002=CARTESIAN_POINT ( 'NONE',  ( 10.81189881249999551, -6.242252689847874514, -79.46875000204838102 ) ) ;
#6003=FACE_OUTER_BOUND ( 'NONE', #37784, .T. ) ;
#6004=CARTESIAN_POINT ( 'NONE',  ( 0.000000000000000000, 0.000000000000000000, -200.0000000000000000 ) ) ;
#6008=CARTESIAN_POINT ( 'NONE',  ( 9.999999999999998224, 0.000000000000000000, -12.87500000409674783 ) ) ;
#6010=CARTESIAN_POINT ( 'NONE',  ( 10.81189881249999907, 6.242252689847868297, -130.2187500020483810 ) ) ;
#6011=CARTESIAN_POINT ( 'NONE',  ( 5.405949406249992428, -9.363379034771808662, -100.7812500020483952 ) ) ;
#6012=CARTESIAN_POINT ( 'NONE',  ( 7.644554776091147741E-16, 12.48450537969573659, -116.4687500020483668 ) ) ;
#6015=CARTESIAN_POINT ( 'NONE',  ( -9.999999999999998224, 1.224646799147353059E-15, -168.1250000040967905 ) ) ;
#6016=CARTESIAN_POINT ( 'NONE',  ( -9.999999999999227285, -5.773502691896698735, -133.5000000040967620 ) ) ;
#6019=CARTESIAN_POINT ( 'NONE',  ( 10.81189881249999729, 6.242252689847867408, -47.71875000204837391 ) ) ;
#6021=CARTESIAN_POINT ( 'NONE',  ( -2.293366432827344421E-15, -12.48450537969573659, -0.4062500020483658103 ) ) ;
#6023=CARTESIAN_POINT ( 'NONE',  ( 9.999999999999998224, 0.000000000000000000, -87.49999999999998579 ) ) ;
#6025=CARTESIAN_POINT ( 'NONE',  ( -10.00000000000000000, -5.773502691896251982, -91.12499999999998579 ) ) ;
#6027=CARTESIAN_POINT ( 'NONE',  ( 4.999999999999992006, -8.660254037844389075, -94.12500000409677625 ) ) ;
#6028=CARTESIAN_POINT ( 'NONE',  ( 9.999999999999479527, 5.773502691896553074, -150.7500000040967336 ) ) ;
#6030=CARTESIAN_POINT ( 'NONE',  ( 10.81189881249999729, 0.000000000000000000, -94.53125000204838102 ) ) ;
#6031=ORIENTED_EDGE ( 'NONE', *, *, #39381, .F. ) ;
#6036=CARTESIAN_POINT ( 'NONE',  ( 9.999999999999996447, -5.773502691896262640, -18.62499999999997868 ) ) ;
#6037=CARTESIAN_POINT ( 'NONE',  ( 10.81189881249999551, -6.242252689847874514, -22.65625000204837391 ) ) ;
#6038=CARTESIAN_POINT ( 'NONE',  ( -9.999999999999998224, 5.773502691896259087, -157.3749999999999716 ) ) ;
#6040=ADVANCED_FACE ( 'NONE', ( #3831 ), #42239, .T. ) ;
#6041=CARTESIAN_POINT ( 'NONE',  ( 7.070501591499377789E-16, 11.54700538379251284, -195.1250000000000284 ) ) ;
#6042=CARTESIAN_POINT ( 'NONE',  ( 5.405949406249999534, 9.363379034771803333, -122.7812500020483952 ) ) ;
#6043=VERTEX_POINT ( 'NONE', #35791 ) ;
#6044=CARTESIAN_POINT ( 'NONE',  ( -2.121150477449813534E-15, -11.54700538379251284, -12.87499999999996447 ) ) ;
#6045=ORIENTED_EDGE ( 'NONE', *, *, #27910, .F. ) ;
#6046=CARTESIAN_POINT ( 'NONE',  ( 10.81189881249999729, 0.000000000000000000, -54.03125000204836681 ) ) ;
#6048=CARTESIAN_POINT ( 'NONE',  ( -5.405949406250003975, -9.363379034771801557, -100.8437500020483810 ) ) ;
#6049=ORIENTED_EDGE ( 'NONE', *, *, #30937, .T. ) ;
#6051=DIRECTION ( 'NONE',  ( -0.000000000000000000, -0.000000000000000000, 1.000000000000000000 ) ) ;
#6052=CARTESIAN_POINT ( 'NONE',  ( -4.999999999999996447, 8.660254037844387298, -144.3750000040967905 ) ) ;
#6053=CARTESIAN_POINT ( 'NONE',  ( -10.81189881249999729, 1.324075727343319199E-15, -150.5937500020483810 ) ) ;
#6055=CARTESIAN_POINT ( 'NONE',  ( 10.81189881249999729, 0.000000000000000000, 0.1562499979516351889 ) ) ;
#6057=ADVANCED_FACE ( 'NONE', ( #29304 ), #12664, .T. ) ;
#6058=CARTESIAN_POINT ( 'NONE',  ( 7.644554776091147741E-16, 12.48450537969573659, -137.4687500020483810 ) ) ;
#6060=CARTESIAN_POINT ( 'NONE',  ( 4.999999999999992006, -8.660254037844389075, -147.7500000000000000 ) ) ;
#6062=CARTESIAN_POINT ( 'NONE',  ( -9.999999999999998224, 5.773502691896259087, -192.2500000040968189 ) ) ;
#6064=CARTESIAN_POINT ( 'NONE',  ( 7.644554776091147741E-16, 12.48450537969573659, -190.1562500020483810 ) ) ;
#6066=CARTESIAN_POINT ( 'NONE',  ( 9.999999999999479527, 5.773502691896553074, -149.2500000040967905 ) ) ;
#6069=CARTESIAN_POINT ( 'NONE',  ( -10.81189881249999729, -6.242252689847864744, -70.96875000204839523 ) ) ;
#6070=CARTESIAN_POINT ( 'NONE',  ( -5.405949406249996869, 9.363379034771805109, -47.34375000204838102 ) ) ;
#6073=CARTESIAN_POINT ( 'NONE',  ( -5.405949406249996869, 9.363379034771805109, -28.03125000204837036 ) ) ;
#6074=VECTOR ( 'NONE', #10804, 1000.000000000000000 ) ;
#6078=CARTESIAN_POINT ( 'NONE',  ( -10.00000000000000000, -5.773502691896251982, -116.6249999999999858 ) ) ;
#6079=AXIS2_PLACEMENT_3D ( 'NONE', #38693, #11926, #8495 ) ;
#6080=( BOUNDED_CURVE ( )  B_SPLINE_CURVE ( 2, ( #9793, #19925, #33539, #39353, #16674, #12804, #6559 ),
 .UNSPECIFIED., .F., .F. ) 
 B_SPLINE_CURVE_WITH_KNOTS ( ( 3, 2, 2, 3 ),
 ( 0.04477611940298512061, 0.04601990049751248507, 0.04726368159203984259, 0.04850746268656720706 ),
 .UNSPECIFIED. ) 
 CURVE ( )  GEOMETRIC_REPRESENTATION_ITEM ( )  RATIONAL_B_SPLINE_CURVE ( ( 0.9999999999999947820, 0.8660254037844439257, 1.000000000000000000, 0.8660254037844387076, 1.000000000000000000, 0.8660254037844342667, 1.000000000000004441 ) ) 
 REPRESENTATION_ITEM ( '' )  );
#6083=CARTESIAN_POINT ( 'NONE',  ( 5.405949406249999534, 9.363379034771803333, -116.7812500020483952 ) ) ;
#6084=ORIENTED_EDGE ( 'NONE', *, *, #24740, .F. ) ;
#6085=CARTESIAN_POINT ( 'NONE',  ( 7.070501591499376803E-16, 11.54700538379251284, -197.0000000040968189 ) ) ;
#6087=CARTESIAN_POINT ( 'NONE',  ( -2.121150477449813534E-15, -11.54700538379251284, -38.75000000409676204 ) ) ;
#6089=CARTESIAN_POINT ( 'NONE',  ( 9.999999999999998224, 0.000000000000000000, -43.99999999999998579 ) ) ;
#6090=CARTESIAN_POINT ( 'NONE',  ( -9.999999999999998224, 1.224646799147353059E-15, -25.62500000409675849 ) ) ;
#6091=CARTESIAN_POINT ( 'NONE',  ( 5.405949406249992428, -9.363379034771808662, -42.28125000204838102 ) ) ;
#6092=CYLINDRICAL_SURFACE ( 'NONE', #5616, 10.00000000000000178 ) ;
#6096=CARTESIAN_POINT ( 'NONE',  ( -10.81189881249999907, -6.242252689847864744, -140.1562500020484094 ) ) ;
#6097=CARTESIAN_POINT ( 'NONE',  ( -5.405949406250003975, -9.363379034771801557, -149.0312500020483810 ) ) ;
#6098=CARTESIAN_POINT ( 'NONE',  ( -4.999999999999996447, 8.660254037844387298, -190.5000000000000000 ) ) ;
#6099=EDGE_CURVE ( 'NONE', #6043, #15363, #29258, .T. ) ;
#6100=DIRECTION ( 'NONE',  ( 0.000000000000000000, 0.000000000000000000, 1.000000000000000000 ) ) ;
#6102=VERTEX_POINT ( 'NONE', #3194 ) ;
#6104=LINE ( 'NONE', #2654, #20785 ) ;
#6105=CARTESIAN_POINT ( 'NONE',  ( -10.81189881249999907, -6.242252689847864744, -172.9687500020484094 ) ) ;
#6106=CARTESIAN_POINT ( 'NONE',  ( 7.644554776091147741E-16, 12.48450537969573659, -30.96875000204835260 ) ) ;
#6107=CARTESIAN_POINT ( 'NONE',  ( -2.293366432827344421E-15, -12.48450537969573659, -163.7187500020483810 ) ) ;
#6108=CARTESIAN_POINT ( 'NONE',  ( 10.81189881249999729, 0.000000000000000000, -146.8437500020483810 ) ) ;
#6109=FACE_OUTER_BOUND ( 'NONE', #7357, .T. ) ;
#6112=CARTESIAN_POINT ( 'NONE',  ( -2.293366432827344421E-15, -12.48450537969573659, -18.21875000204837036 ) ) ;
#6115=( BOUNDED_CURVE ( )  B_SPLINE_CURVE ( 2, ( #34015, #10898, #40666, #21043, #21261, #40882, #3805 ),
 .UNSPECIFIED., .F., .F. ) 
 B_SPLINE_CURVE_WITH_KNOTS ( ( 3, 2, 2, 3 ),
 ( 0.4104477611940299253, 0.4116915422885572551, 0.4129353233830846959, 0.4141791044776120256 ),
 .UNSPECIFIED. ) 
 CURVE ( )  GEOMETRIC_REPRESENTATION_ITEM ( )  RATIONAL_B_SPLINE_CURVE ( ( 0.9999999999999940048, 0.8660254037844447028, 1.000000000000000000, 0.8660254037844387076, 1.000000000000000000, 0.8660254037844267172, 1.000000000000011990 ) ) 
 REPRESENTATION_ITEM ( '' )  );
#6116=CARTESIAN_POINT ( 'NONE',  ( -9.999999999999998224, 1.224646799147353059E-15, -119.7500000000000000 ) ) ;
#6118=CARTESIAN_POINT ( 'NONE',  ( 5.405949406249992428, -9.363379034771808662, -73.59375000204838102 ) ) ;
#6119=CARTESIAN_POINT ( 'NONE',  ( 10.81189881249999907, 6.242252689847868297, -47.90625000204836681 ) ) ;
#6123=CARTESIAN_POINT ( 'NONE',  ( 9.999999999999998224, 0.000000000000000000, -141.5000000000000000 ) ) ;
#6124=CARTESIAN_POINT ( 'NONE',  ( 10.81189881249999729, 6.242252689847867408, -149.9062500020484094 ) ) ;
#6126=CARTESIAN_POINT ( 'NONE',  ( -4.999999999999996447, 8.660254037844387298, -123.3750000040967905 ) ) ;
#6128=EDGE_LOOP ( 'NONE', ( #7801, #4234, #34167, #15316 ) ) ;
#6129=( BOUNDED_CURVE ( )  B_SPLINE_CURVE ( 2, ( #39477, #17221, #16362 ),
 .UNSPECIFIED., .F., .T. ) 
 B_SPLINE_CURVE_WITH_KNOTS ( ( 3, 3 ),
 ( 0.9894244345683576025, 0.9894279716579621464 ),
 .UNSPECIFIED. ) 
 CURVE ( )  GEOMETRIC_REPRESENTATION_ITEM ( )  RATIONAL_B_SPLINE_CURVE ( ( 0.9330147350531647898, 0.9330126360445730738, 0.9330127040248163972 ) ) 
 REPRESENTATION_ITEM ( '' )  );
#6133=CARTESIAN_POINT ( 'NONE',  ( -10.81189881249999729, 1.324075727343319199E-15, -168.7812500020484094 ) ) ;
#6134=CARTESIAN_POINT ( 'NONE',  ( -9.999999999999998224, 1.224646799147353059E-15, -48.12500000409677625 ) ) ;
#6135=VECTOR ( 'NONE', #26712, 1000.000000000000000 ) ;
#6138=CARTESIAN_POINT ( 'NONE',  ( 11.54700538379250396, 20.00000000000000711, 49.99999999999998579 ) ) ;
#6139=CARTESIAN_POINT ( 'NONE',  ( 10.81189881249999729, 0.000000000000000000, -163.5312500020484094 ) ) ;
#6140=CIRCLE ( 'NONE', #13709, 9.999999999999998224 ) ;
#6141=CARTESIAN_POINT ( 'NONE',  ( 5.405949406249992428, -9.363379034771808662, -144.0937500020483810 ) ) ;
#6142=DIRECTION ( 'NONE',  ( -0.000000000000000000, -0.000000000000000000, 1.000000000000000000 ) ) ;
#6143=CARTESIAN_POINT ( 'NONE',  ( 9.999999999999998224, 0.000000000000000000, -64.99999999999997158 ) ) ;
#6144=EDGE_CURVE ( 'NONE', #19099, #1402, #6223, .T. ) ;
#6145=ORIENTED_EDGE ( 'NONE', *, *, #40683, .F. ) ;
#6146=EDGE_CURVE ( 'NONE', #5178, #13534, #41079, .T. ) ;
#6147=CARTESIAN_POINT ( 'NONE',  ( -5.000000000000003553, -8.660254037844383745, -52.37500000409675494 ) ) ;
#6149=CARTESIAN_POINT ( 'NONE',  ( 7.644554776091147741E-16, 12.48450537969573659, -71.65625000204836681 ) ) ;
#6150=ORIENTED_EDGE ( 'NONE', *, *, #598, .T. ) ;
#6151=CARTESIAN_POINT ( 'NONE',  ( -9.999999999999479527, -5.773502691896549521, -143.6250000000000000 ) ) ;
#6152=ORIENTED_EDGE ( 'NONE', *, *, #32185, .T. ) ;
#6153=ORIENTED_EDGE ( 'NONE', *, *, #21972, .F. ) ;
#6154=CARTESIAN_POINT ( 'NONE',  ( 10.81189881249999729, 0.000000000000000000, -28.34375000204836326 ) ) ;
#6155=CARTESIAN_POINT ( 'NONE',  ( -10.00000000000076916, 5.773502691895813221, -107.8749999999999574 ) ) ;
#6156=CARTESIAN_POINT ( 'NONE',  ( 7.644554776091147741E-16, 12.48450537969573659, -8.656250002048372139 ) ) ;
#6157=CARTESIAN_POINT ( 'NONE',  ( 5.405949406249992428, -9.363379034771808662, -54.09375000204835970 ) ) ;
#6158=CARTESIAN_POINT ( 'NONE',  ( 9.999999999999998224, 0.000000000000000000, -71.37500000409677625 ) ) ;
#6160=EDGE_CURVE ( 'NONE', #40301, #35906, #17383, .T. ) ;
#6161=CARTESIAN_POINT ( 'NONE',  ( 10.81189881249999729, 6.242252689847867408, -188.7187500020484094 ) ) ;
#6162=CARTESIAN_POINT ( 'NONE',  ( 10.81189881249999907, 6.242252689847868297, -169.2187500020483810 ) ) ;
#6168=CARTESIAN_POINT ( 'NONE',  ( -5.405949406249996869, 9.363379034771805109, -108.8437500020483810 ) ) ;
#6169=CARTESIAN_POINT ( 'NONE',  ( -5.000000000000003553, -8.660254037844383745, -72.99999999999998579 ) ) ;
#6170=CARTESIAN_POINT ( 'NONE',  ( -10.81189881249999907, -6.242252689847864744, -72.65625000204836681 ) ) ;
#6171=CARTESIAN_POINT ( 'NONE',  ( 7.070501591499376803E-16, 11.54700538379251284, -96.50000000409677625 ) ) ;
#6172=CARTESIAN_POINT ( 'NONE',  ( -5.405949406250003975, -9.363379034771801557, -87.34375000204836681 ) ) ;
#6175=CARTESIAN_POINT ( 'NONE',  ( -9.999999999999998224, 5.773502691896259087, -144.2500000040967905 ) ) ;
#6177=ORIENTED_EDGE ( 'NONE', *, *, #14835, .T. ) ;
#6181=CARTESIAN_POINT ( 'NONE',  ( 5.405949406249999534, 9.363379034771803333, -193.2812500020484094 ) ) ;
#6182=DIRECTION ( 'NONE',  ( 1.000000000000000000, 0.000000000000000000, 0.000000000000000000 ) ) ;
#6184=ORIENTED_EDGE ( 'NONE', *, *, #40441, .T. ) ;
#6185=CARTESIAN_POINT ( 'NONE',  ( -5.000000000000003553, -8.660254037844383745, -60.99999999999997158 ) ) ;
#6187=CARTESIAN_POINT ( 'NONE',  ( -4.999999999999996447, 8.660254037844387298, -75.37500000409677625 ) ) ;
#6188=CARTESIAN_POINT ( 'NONE',  ( 5.000000000000000000, 8.660254037844385522, -66.24999999999997158 ) ) ;
#6191=CARTESIAN_POINT ( 'NONE',  ( 10.81189881249999729, 0.000000000000000000, -67.53125000204838102 ) ) ;
#6195=CARTESIAN_POINT ( 'NONE',  ( -5.405949406250003975, -9.363379034771801557, -192.5312500020484094 ) ) ;
#6197=CARTESIAN_POINT ( 'NONE',  ( -10.81189881249999729, -6.242252689847864744, -6.468750002048346381 ) ) ;
#6199=( BOUNDED_CURVE ( )  B_SPLINE_CURVE ( 2, ( #4052, #24133, #16984, #27142, #23491, #4477, #37274 ),
 .UNSPECIFIED., .F., .F. ) 
 B_SPLINE_CURVE_WITH_KNOTS ( ( 3, 2, 2, 3 ),
 ( 0.5111940298507463565, 0.5124378109452737418, 0.5136815920398011270, 0.5149253731343285123 ),
 .UNSPECIFIED. ) 
 CURVE ( )  GEOMETRIC_REPRESENTATION_ITEM ( )  RATIONAL_B_SPLINE_CURVE ( ( 0.9999999999999880096, 0.8660254037844506980, 1.000000000000000000, 0.8660254037844387076, 1.000000000000000000, 0.8660254037844267172, 1.000000000000011990 ) ) 
 REPRESENTATION_ITEM ( '' )  );
#6200=FACE_OUTER_BOUND ( 'NONE', #36762, .T. ) ;
#6201=FACE_OUTER_BOUND ( 'NONE', #25952, .T. ) ;
#6202=ADVANCED_FACE ( 'NONE', ( #9868 ), #29735, .T. ) ;
#6203=CARTESIAN_POINT ( 'NONE',  ( -4.999999999999996447, 8.660254037844387298, -171.0000000000000000 ) ) ;
#6204=CARTESIAN_POINT ( 'NONE',  ( 9.999999999998969713, 5.773502691896851502, -1.874999999999918954 ) ) ;
#6205=VECTOR ( 'NONE', #32948, 1000.000000000000000 ) ;
#6206=ADVANCED_FACE ( 'NONE', ( #21065 ), #14358, .T. ) ;
#6207=CARTESIAN_POINT ( 'NONE',  ( 10.81189881249999729, 0.000000000000000000, -97.53125000204839523 ) ) ;
#6212=CARTESIAN_POINT ( 'NONE',  ( -10.81189881249999729, 1.324075727343319199E-15, -32.09375000204836681 ) ) ;
#6213=CARTESIAN_POINT ( 'NONE',  ( -10.81189881249999729, 6.242252689847871849, -33.90625000204836681 ) ) ;
#6215=CARTESIAN_POINT ( 'NONE',  ( 10.81189881249999729, 0.000000000000000000, -79.34375000204838102 ) ) ;
#6216=DIRECTION ( 'NONE',  ( 1.000000000000000000, 0.000000000000000000, 0.000000000000000000 ) ) ;
#6218=EDGE_CURVE ( 'NONE', #29288, #19092, #40690, .T. ) ;
#6219=CYLINDRICAL_SURFACE ( 'NONE', #15688, 9.999999999999998224 ) ;
#6220=CARTESIAN_POINT ( 'NONE',  ( -11.54700538379250396, -20.00000000000000355, 45.00000000000009237 ) ) ;
#6222=CARTESIAN_POINT ( 'NONE',  ( 9.999999999999998224, 0.000000000000000000, -8.375000004096744277 ) ) ;
#6223=LINE ( 'NONE', #13510, #21210 ) ;
#6224=CARTESIAN_POINT ( 'NONE',  ( 5.405949406249992428, -9.363379034771808662, -127.5937500020483668 ) ) ;
#6225=CARTESIAN_POINT ( 'NONE',  ( -2.293366432827344421E-15, -12.48450537969573659, -99.40625000204839523 ) ) ;
#6226=CARTESIAN_POINT ( 'NONE',  ( 10.81189881249999729, 0.000000000000000000, -110.8437500020483810 ) ) ;
#6229=CARTESIAN_POINT ( 'NONE',  ( 9.999999999999998224, 0.000000000000000000, -171.8750000040968189 ) ) ;
#6230=CARTESIAN_POINT ( 'NONE',  ( -5.000000000000003553, -8.660254037844383745, -133.3750000040967905 ) ) ;
#6233=AXIS2_PLACEMENT_3D ( 'NONE', #14338, #8110, #11325 ) ;
#6237=CARTESIAN_POINT ( 'NONE',  ( -10.00000000000102496, 5.773502691895664007, -5.874999999999936939 ) ) ;
#6239=CARTESIAN_POINT ( 'NONE',  ( 5.000000000000000000, 8.660254037844385522, -93.24999999999998579 ) ) ;
#6241=CARTESIAN_POINT ( 'NONE',  ( 4.999999999999992006, -8.660254037844389075, -97.12500000409677625 ) ) ;
#6242=DIRECTION ( 'NONE',  ( -0.000000000000000000, -0.000000000000000000, 1.000000000000000000 ) ) ;
#6244=CARTESIAN_POINT ( 'NONE',  ( -10.81189881249999729, 1.324075727343319199E-15, -92.28125000204838102 ) ) ;
#6246=( BOUNDED_CURVE ( )  B_SPLINE_CURVE ( 2, ( #18104, #41405, #28268, #24399, #41620, #14426, #12054 ),
 .UNSPECIFIED., .F., .F. ) 
 B_SPLINE_CURVE_WITH_KNOTS ( ( 3, 2, 2, 3 ),
 ( 0.1977611940298507898, 0.1990049751243781750, 0.2002487562189055326, 0.2014925373134328901 ),
 .UNSPECIFIED. ) 
 CURVE ( )  GEOMETRIC_REPRESENTATION_ITEM ( )  RATIONAL_B_SPLINE_CURVE ( ( 0.9999999999999940048, 0.8660254037844447028, 1.000000000000000000, 0.8660254037844387076, 1.000000000000000000, 0.8660254037844327124, 1.000000000000005995 ) ) 
 REPRESENTATION_ITEM ( '' )  );
#6248=CARTESIAN_POINT ( 'NONE',  ( 9.999999999999998224, 0.000000000000000000, -72.49999999999998579 ) ) ;
#6250=ORIENTED_EDGE ( 'NONE', *, *, #36218, .T. ) ;
#6251=CARTESIAN_POINT ( 'NONE',  ( -4.999999999999996447, 8.660254037844387298, -20.99999999999996447 ) ) ;
#6252=CARTESIAN_POINT ( 'NONE',  ( -2.121150477449813534E-15, -11.54700538379251284, -153.8750000000000000 ) ) ;
#6254=CARTESIAN_POINT ( 'NONE',  ( 7.644554776091147741E-16, 12.48450537969573659, -128.6562500020483810 ) ) ;
#6256=CARTESIAN_POINT ( 'NONE',  ( 9.999999999999998224, 0.000000000000000000, -92.37500000409677625 ) ) ;
#6257=ORIENTED_EDGE ( 'NONE', *, *, #23342, .T. ) ;
#6258=CARTESIAN_POINT ( 'NONE',  ( -2.293366432827344421E-15, -12.48450537969573659, -54.40625000204838102 ) ) ;
#6260=AXIS2_PLACEMENT_3D ( 'NONE', #21154, #18561, #24423 ) ;
#6261=EDGE_CURVE ( 'NONE', #7227, #17891, #11130, .T. ) ;
#6262=CARTESIAN_POINT ( 'NONE',  ( 5.405949406249999534, 9.363379034771803333, -103.0937500020483810 ) ) ;
#6264=ORIENTED_EDGE ( 'NONE', *, *, #22573, .F. ) ;
#6265=AXIS2_PLACEMENT_3D ( 'NONE', #6138, #6981, #16238 ) ;
#6266=CARTESIAN_POINT ( 'NONE',  ( -9.999999999999998224, 1.224646799147353059E-15, -85.62500000409677625 ) ) ;
#6267=CARTESIAN_POINT ( 'NONE',  ( 0.000000000000000000, 0.000000000000000000, -200.0000000000000000 ) ) ;
#6270=CARTESIAN_POINT ( 'NONE',  ( 5.405949406249999534, 9.363379034771803333, -128.5937500020483810 ) ) ;
#6274=CARTESIAN_POINT ( 'NONE',  ( 9.999999999999998224, 0.000000000000000000, -195.8750000040967905 ) ) ;
#6276=EDGE_CURVE ( 'NONE', #2082, #29986, #24540, .T. ) ;
#6277=CARTESIAN_POINT ( 'NONE',  ( -10.81189881249999729, 1.324075727343319199E-15, -183.7812500020484094 ) ) ;
#6278=PLANE ( 'NONE',  #39219 ) ;
#6281=CARTESIAN_POINT ( 'NONE',  ( 7.644554776091147741E-16, 12.48450537969573659, -65.46875000204836681 ) ) ;
#6282=CARTESIAN_POINT ( 'NONE',  ( 5.405949406249999534, 9.363379034771803333, -52.09375000204835260 ) ) ;
#6285=CARTESIAN_POINT ( 'NONE',  ( -2.293366432827344421E-15, -12.48450537969573659, -22.90625000204837747 ) ) ;
#6289=CARTESIAN_POINT ( 'NONE',  ( -4.999999999999996447, 8.660254037844387298, -117.0000000000000000 ) ) ;
#6293=CARTESIAN_POINT ( 'NONE',  ( 7.644554776091147741E-16, 12.48450537969573659, -118.1562500020483952 ) ) ;
#6294=ORIENTED_EDGE ( 'NONE', *, *, #6971, .F. ) ;
#6300=CARTESIAN_POINT ( 'NONE',  ( -2.121150477449813534E-15, -11.54700538379251284, -39.87499999999996447 ) ) ;
#6301=CARTESIAN_POINT ( 'NONE',  ( -10.00000000000000000, -5.773502691896251982, -21.00000000409677980 ) ) ;
#6302=CARTESIAN_POINT ( 'NONE',  ( 10.81189881249999729, 0.000000000000000000, -40.53125000204838102 ) ) ;
#6306=CARTESIAN_POINT ( 'NONE',  ( 7.644554776091147741E-16, 12.48450537969573659, -137.6562500020483810 ) ) ;
#6307=CARTESIAN_POINT ( 'NONE',  ( 5.405949406249992428, -9.363379034771808662, -150.2812500020483810 ) ) ;
#6308=CARTESIAN_POINT ( 'NONE',  ( -9.999999999999998224, 1.224646799147353059E-15, -110.7499999999999858 ) ) ;
#6309=ORIENTED_EDGE ( 'NONE', *, *, #20273, .T. ) ;
#6310=ADVANCED_FACE ( 'NONE', ( #40473 ), #31015, .T. ) ;
#6311=ORIENTED_EDGE ( 'NONE', *, *, #39923, .T. ) ;
#6312=EDGE_LOOP ( 'NONE', ( #7412, #31573, #14175, #27061, #25280, #34976, #37676 ) ) ;
#6313=VECTOR ( 'NONE', #20614, 1000.000000000000000 ) ;
#6315=CARTESIAN_POINT ( 'NONE',  ( -10.81189881249999907, -6.242252689847864744, -177.4687500020484094 ) ) ;
#6317=CARTESIAN_POINT ( 'NONE',  ( -10.81189881249999729, 1.324075727343319199E-15, -26.09375000204835970 ) ) ;
#6318=CARTESIAN_POINT ( 'NONE',  ( -9.999999999999998224, 1.224646799147353059E-15, -200.0000000000000000 ) ) ;
#6319=CARTESIAN_POINT ( 'NONE',  ( -10.81189881249999729, -6.242252689847864744, -160.9687500020484094 ) ) ;
#6320=CARTESIAN_POINT ( 'NONE',  ( 10.81189881249999729, 0.000000000000000000, -145.3437500020483810 ) ) ;
#6322=( BOUNDED_CURVE ( )  B_SPLINE_CURVE ( 2, ( #12858, #29081, #12437, #39203, #12646, #31692, #32116 ),
 .UNSPECIFIED., .F., .F. ) 
 B_SPLINE_CURVE_WITH_KNOTS ( ( 3, 2, 2, 3 ),
 ( 0.3097014925373136052, 0.3109452736318408794, 0.3121890547263682092, 0.3134328358208955390 ),
 .UNSPECIFIED. ) 
 CURVE ( )  GEOMETRIC_REPRESENTATION_ITEM ( )  RATIONAL_B_SPLINE_CURVE ( ( 0.9999999999999820144, 0.8660254037844566932, 1.000000000000000000, 0.8660254037844387076, 1.000000000000000000, 0.8660254037844387076, 1.000000000000000000 ) ) 
 REPRESENTATION_ITEM ( '' )  );
#6323=CARTESIAN_POINT ( 'NONE',  ( 4.999999999999992006, -8.660254037844389075, -88.12500000409677625 ) ) ;
#6326=CARTESIAN_POINT ( 'NONE',  ( 10.81189881249999551, -6.242252689847874514, -14.96875000204837036 ) ) ;
#6329=DIRECTION ( 'NONE',  ( 1.000000000000000000, 0.000000000000000000, 0.000000000000000000 ) ) ;
#6333=CARTESIAN_POINT ( 'NONE',  ( -10.81189881249999729, 1.324075727343319199E-15, -72.59375000204838102 ) ) ;
#6334=CARTESIAN_POINT ( 'NONE',  ( 10.81189881249999729, 0.000000000000000000, -51.03125000204835970 ) ) ;
#6336=CARTESIAN_POINT ( 'NONE',  ( 10.00000000000154010, -5.773502691895370020, -16.00000000409673362 ) ) ;
#6338=CARTESIAN_POINT ( 'NONE',  ( -9.999999999999998224, 5.773502691896259087, -137.8750000000000000 ) ) ;
#6339=CARTESIAN_POINT ( 'NONE',  ( 5.405949406249992428, -9.363379034771808662, -136.7812500020483810 ) ) ;
#6340=DIRECTION ( 'NONE',  ( 1.000000000000000000, 0.000000000000000000, 0.000000000000000000 ) ) ;
#6341=CARTESIAN_POINT ( 'NONE',  ( 9.999999999999998224, 0.000000000000000000, -113.3750000040967763 ) ) ;
#6346=CARTESIAN_POINT ( 'NONE',  ( -9.999999999999998224, 1.224646799147353059E-15, -141.1250000040967905 ) ) ;
#6347=CARTESIAN_POINT ( 'NONE',  ( -5.405949406249996869, 9.363379034771805109, -176.5312500020483810 ) ) ;
#6348=CARTESIAN_POINT ( 'NONE',  ( 4.999999999999992006, -8.660254037844389075, -38.62500000409676915 ) ) ;
#6351=AXIS2_PLACEMENT_3D ( 'NONE', #15746, #26543, #19837 ) ;
#6352=CARTESIAN_POINT ( 'NONE',  ( 5.405949406249999534, 9.363379034771803333, -158.7812500020484094 ) ) ;
#6353=CARTESIAN_POINT ( 'NONE',  ( 10.81189881249999551, -6.242252689847874514, -143.9687500020483810 ) ) ;
#6354=CARTESIAN_POINT ( 'NONE',  ( 10.00000000000102318, -5.773502691895667560, -50.50000000409673362 ) ) ;
#6355=CARTESIAN_POINT ( 'NONE',  ( 4.999999999999992006, -8.660254037844389075, -195.7500000000000000 ) ) ;
#6356=ORIENTED_EDGE ( 'NONE', *, *, #17169, .F. ) ;
#6357=FACE_OUTER_BOUND ( 'NONE', #17056, .T. ) ;
#6359=CARTESIAN_POINT ( 'NONE',  ( 5.405949406249999534, 9.363379034771803333, -73.28125000204838102 ) ) ;
#6360=EDGE_LOOP ( 'NONE', ( #10845, #42056, #11228, #23275, #19389 ) ) ;
#6362=CARTESIAN_POINT ( 'NONE',  ( -10.81189881249999907, -6.242252689847864744, -121.9687500020483952 ) ) ;
#6363=ORIENTED_EDGE ( 'NONE', *, *, #4762, .T. ) ;
#6364=ORIENTED_EDGE ( 'NONE', *, *, #14285, .F. ) ;
#6365=CARTESIAN_POINT ( 'NONE',  ( -10.81189881249999729, 6.242252689847871849, -26.21875000204837391 ) ) ;
#6366=( BOUNDED_CURVE ( )  B_SPLINE_CURVE ( 2, ( #19737, #32917, #3350, #16483, #34415, #18416, #20797 ),
 .UNSPECIFIED., .F., .F. ) 
 B_SPLINE_CURVE_WITH_KNOTS ( ( 3, 2, 2, 3 ),
 ( 0.000000000000000000, 0.001243781094527364461, 0.002487562189054728923, 0.003731343283582092950 ),
 .UNSPECIFIED. ) 
 CURVE ( )  GEOMETRIC_REPRESENTATION_ITEM ( )  RATIONAL_B_SPLINE_CURVE ( ( 1.000000000000000000, 0.8660254037844387076, 1.000000000000000000, 0.8660254037844387076, 1.000000000000000000, 0.8660254037844383745, 1.000000000000000444 ) ) 
 REPRESENTATION_ITEM ( '' )  );
#6367=CARTESIAN_POINT ( 'NONE',  ( 10.81189881249999551, -6.242252689847874514, -1.656250002048371694 ) ) ;
#6368=CARTESIAN_POINT ( 'NONE',  ( 10.81189881249999907, 6.242252689847868297, -44.71875000204837391 ) ) ;
#6369=DIRECTION ( 'NONE',  ( -0.000000000000000000, -0.000000000000000000, 1.000000000000000000 ) ) ;
#6371=CARTESIAN_POINT ( 'NONE',  ( -2.293366432827344421E-15, -12.48450537969573659, -187.7187500020484094 ) ) ;
#6372=CARTESIAN_POINT ( 'NONE',  ( -2.293366432827344421E-15, -12.48450537969573659, -172.7187500020484094 ) ) ;
#6376=( BOUNDED_CURVE ( )  B_SPLINE_CURVE ( 2, ( #12120, #42104, #19440, #38457, #15979, #12539, #29381 ),
 .UNSPECIFIED., .F., .F. ) 
 B_SPLINE_CURVE_WITH_KNOTS ( ( 3, 2, 2, 3 ),
 ( 0.3544776119402986980, 0.3557213930348260278, 0.3569651741293533576, 0.3582089552238806873 ),
 .UNSPECIFIED. ) 
 CURVE ( )  GEOMETRIC_REPRESENTATION_ITEM ( )  RATIONAL_B_SPLINE_CURVE ( ( 0.9999999999999820144, 0.8660254037844566932, 1.000000000000000000, 0.8660254037844387076, 1.000000000000000000, 0.8660254037844267172, 1.000000000000011990 ) ) 
 REPRESENTATION_ITEM ( '' )  );
#6377=CARTESIAN_POINT ( 'NONE',  ( -10.00000000000154188, 5.773502691895366468, -19.75000000409673362 ) ) ;
#6379=CARTESIAN_POINT ( 'NONE',  ( -10.81189881249999729, 6.242252689847871849, -99.71875000204839523 ) ) ;
#6380=CARTESIAN_POINT ( 'NONE',  ( -10.00000000000051337, 5.773502691895962435, -108.2500000040967763 ) ) ;
#6381=CARTESIAN_POINT ( 'NONE',  ( 10.81189881249999729, 0.000000000000000000, -78.03125000204838102 ) ) ;
#6382=CARTESIAN_POINT ( 'NONE',  ( -9.999999999999998224, 1.224646799147353059E-15, -96.12500000409677625 ) ) ;
#6383=ADVANCED_FACE ( 'NONE', ( #14138 ), #40905, .T. ) ;
#6385=CARTESIAN_POINT ( 'NONE',  ( -5.405949406249996869, 9.363379034771805109, -170.5312500020484094 ) ) ;
#6386=EDGE_CURVE ( 'NONE', #2082, #19929, #1156, .T. ) ;
#6388=CARTESIAN_POINT ( 'NONE',  ( -2.121150477449813534E-15, -11.54700538379251284, -134.7500000040967905 ) ) ;
#6390=ORIENTED_EDGE ( 'NONE', *, *, #35439, .F. ) ;
#6393=CARTESIAN_POINT ( 'NONE',  ( 10.81189881249999729, 0.000000000000000000, -195.0312500020484094 ) ) ;
#6394=CARTESIAN_POINT ( 'NONE',  ( 9.999999999999998224, 0.000000000000000000, -200.0000000000000000 ) ) ;
#6396=VERTEX_POINT ( 'NONE', #14579 ) ;
#6397=CARTESIAN_POINT ( 'NONE',  ( -10.00000000000000000, -5.773502691896251982, -55.12499999999997158 ) ) ;
#6399=CARTESIAN_POINT ( 'NONE',  ( 9.999999999999998224, 0.000000000000000000, -75.87500000409677625 ) ) ;
#6401=CARTESIAN_POINT ( 'NONE',  ( -9.999999999999998224, 1.224646799147353059E-15, -160.6250000040967905 ) ) ;
#6403=CARTESIAN_POINT ( 'NONE',  ( -2.293366432827344421E-15, -12.48450537969573659, -70.90625000204839523 ) ) ;
#6406=CYLINDRICAL_SURFACE ( 'NONE', #24204, 9.999999999999998224 ) ;
#6407=CARTESIAN_POINT ( 'NONE',  ( 5.405949406249999534, 9.363379034771803333, -182.7812500020484094 ) ) ;
#6410=DIRECTION ( 'NONE',  ( 1.000000000000000000, 0.000000000000000000, 0.000000000000000000 ) ) ;
#6413=CARTESIAN_POINT ( 'NONE',  ( -5.000000000000003553, -8.660254037844383745, -169.0000000000000000 ) ) ;
#6414=FACE_OUTER_BOUND ( 'NONE', #18182, .T. ) ;
#6415=CARTESIAN_POINT ( 'NONE',  ( 5.405949406249992428, -9.363379034771808662, -96.28125000204838102 ) ) ;
#6416=ORIENTED_EDGE ( 'NONE', *, *, #37047, .T. ) ;
#6417=CARTESIAN_POINT ( 'NONE',  ( -5.000000000000003553, -8.660254037844383745, -181.3750000040967905 ) ) ;
#6418=DIRECTION ( 'NONE',  ( -0.000000000000000000, -0.000000000000000000, 1.000000000000000000 ) ) ;
#6420=VERTEX_POINT ( 'NONE', #27767 ) ;
#6421=CARTESIAN_POINT ( 'NONE',  ( -10.81189881249999729, 1.324075727343319199E-15, -38.09375000204837391 ) ) ;
#6422=CARTESIAN_POINT ( 'NONE',  ( 10.81189881249999729, 0.000000000000000000, -21.03125000204836326 ) ) ;
#6424=CARTESIAN_POINT ( 'NONE',  ( 10.81189881249999729, 0.000000000000000000, -80.84375000204838102 ) ) ;
#6425=CARTESIAN_POINT ( 'NONE',  ( 5.405949406249999534, 9.363379034771803333, -194.5937500020484094 ) ) ;
#6426=CARTESIAN_POINT ( 'NONE',  ( -11.54700538379251817, 20.00000000000000355, 49.99999999999998579 ) ) ;
#6427=CARTESIAN_POINT ( 'NONE',  ( 9.999999999999998224, 0.000000000000000000, -200.0000000000000000 ) ) ;
#6429=CARTESIAN_POINT ( 'NONE',  ( 5.000000000000000000, 8.660254037844385522, -6.625000004096770923 ) ) ;
#6430=DIRECTION ( 'NONE',  ( -0.000000000000000000, -0.000000000000000000, 1.000000000000000000 ) ) ;
#6431=CARTESIAN_POINT ( 'NONE',  ( 5.405949406249992428, -9.363379034771808662, -118.5937500020483810 ) ) ;
#6432=CARTESIAN_POINT ( 'NONE',  ( -2.293366432827344421E-15, -12.48450537969573659, -97.90625000204839523 ) ) ;
#6433=EDGE_CURVE ( 'NONE', #16098, #30518, #9955, .T. ) ;
#6434=CARTESIAN_POINT ( 'NONE',  ( 5.405949406249999534, 9.363379034771803333, -104.5937500020483810 ) ) ;
#6437=CARTESIAN_POINT ( 'NONE',  ( 9.999999999999996447, -5.773502691896262640, -169.0000000040967905 ) ) ;
#6439=CARTESIAN_POINT ( 'NONE',  ( -9.999999999999998224, 1.224646799147353059E-15, -145.6250000040967905 ) ) ;
#6442=EDGE_CURVE ( 'NONE', #40023, #23935, #40064, .T. ) ;
#6446=CARTESIAN_POINT ( 'NONE',  ( -5.000000000000003553, -8.660254037844383745, -127.0000000000000000 ) ) ;
#6448=CARTESIAN_POINT ( 'NONE',  ( -4.999999999999996447, 8.660254037844387298, -85.49999999999998579 ) ) ;
#6450=CARTESIAN_POINT ( 'NONE',  ( 4.999999999999992006, -8.660254037844389075, -100.1250000040967905 ) ) ;
#6451=( BOUNDED_CURVE ( )  B_SPLINE_CURVE ( 2, ( #19306, #3771, #16905, #13244, #19734, #13032, #39582 ),
 .UNSPECIFIED., .F., .F. ) 
 B_SPLINE_CURVE_WITH_KNOTS ( ( 3, 2, 2, 3 ),
 ( 0.02985074626865674360, 0.03109452736318411153, 0.03233830845771147600, 0.03358208955223884046 ),
 .UNSPECIFIED. ) 
 CURVE ( )  GEOMETRIC_REPRESENTATION_ITEM ( )  RATIONAL_B_SPLINE_CURVE ( ( 0.9999999999999970024, 0.8660254037844417052, 1.000000000000000000, 0.8660254037844387076, 1.000000000000000000, 0.8660254037844349329, 1.000000000000003775 ) ) 
 REPRESENTATION_ITEM ( '' )  );
#6452=CARTESIAN_POINT ( 'NONE',  ( 9.999999999999998224, 0.000000000000000000, -200.0000000000000000 ) ) ;
#6455=CARTESIAN_POINT ( 'NONE',  ( 10.81189881249999551, -6.242252689847874514, -88.65625000204838102 ) ) ;
#6456=ORIENTED_EDGE ( 'NONE', *, *, #8166, .F. ) ;
#6458=CARTESIAN_POINT ( 'NONE',  ( 0.000000000000000000, 0.000000000000000000, -200.0000000000000000 ) ) ;
#6460=EDGE_LOOP ( 'NONE', ( #2524, #40983, #42374, #38132 ) ) ;
#6461=CARTESIAN_POINT ( 'NONE',  ( 9.999999999999996447, -5.773502691896262640, -6.624999999999968026 ) ) ;
#6462=CARTESIAN_POINT ( 'NONE',  ( -4.999999999999996447, 8.660254037844387298, -144.0000000000000000 ) ) ;
#6465=CARTESIAN_POINT ( 'NONE',  ( 5.000000000000000000, 8.660254037844385522, -196.7500000000000000 ) ) ;
#6466=CARTESIAN_POINT ( 'NONE',  ( -5.405949406249996869, 9.363379034771805109, -116.5312500020483952 ) ) ;
#6467=ORIENTED_EDGE ( 'NONE', *, *, #23858, .T. ) ;
#6468=CARTESIAN_POINT ( 'NONE',  ( 4.999999999999992006, -8.660254037844389075, -12.74999999999995559 ) ) ;
#6470=CARTESIAN_POINT ( 'NONE',  ( -10.81189881249999729, 6.242252689847871849, -51.90625000204838813 ) ) ;
#6472=CARTESIAN_POINT ( 'NONE',  ( -2.293366432827344421E-15, -12.48450537969573659, -103.7187500020483668 ) ) ;
#6473=CARTESIAN_POINT ( 'NONE',  ( 10.81189881249999551, -6.242252689847874514, -127.6562500020483810 ) ) ;
#6474=ORIENTED_EDGE ( 'NONE', *, *, #41638, .F. ) ;
#6477=CARTESIAN_POINT ( 'NONE',  ( 5.405949406249999534, 9.363379034771803333, -1.093750002048365921 ) ) ;
#6478=LINE ( 'NONE', #37523, #24560 ) ;
#6479=CARTESIAN_POINT ( 'NONE',  ( -10.81189881249999729, 1.324075727343319199E-15, -135.5937500020483810 ) ) ;
#6481=DIRECTION ( 'NONE',  ( -0.000000000000000000, -0.000000000000000000, 1.000000000000000000 ) ) ;
#6483=CARTESIAN_POINT ( 'NONE',  ( -5.000000000000003553, -8.660254037844383745, -194.8750000040967905 ) ) ;
#6485=CARTESIAN_POINT ( 'NONE',  ( -5.405949406249996869, 9.363379034771805109, -187.0312500020484094 ) ) ;
#6489=CARTESIAN_POINT ( 'NONE',  ( -2.293366432827344421E-15, -12.48450537969573659, -61.71875000204839523 ) ) ;
#6490=CARTESIAN_POINT ( 'NONE',  ( 10.81189881249999907, 6.242252689847868297, -52.21875000204837391 ) ) ;
#6492=CARTESIAN_POINT ( 'NONE',  ( -5.405949406250003975, -9.363379034771801557, -21.53125000204836326 ) ) ;
#6495=CARTESIAN_POINT ( 'NONE',  ( -9.999999999999998224, 1.224646799147353059E-15, -101.7500000000000000 ) ) ;
#6497=CARTESIAN_POINT ( 'NONE',  ( -5.000000000000003553, -8.660254037844383745, -114.9999999999999858 ) ) ;
#6500=CARTESIAN_POINT ( 'NONE',  ( -2.293366432827344421E-15, -12.48450537969573659, -117.4062500020483952 ) ) ;
#6501=ORIENTED_EDGE ( 'NONE', *, *, #11941, .T. ) ;
#6502=CARTESIAN_POINT ( 'NONE',  ( -9.999999999999998224, 1.224646799147353059E-15, -200.0000000000000000 ) ) ;
#6504=CARTESIAN_POINT ( 'NONE',  ( -5.000000000000003553, -8.660254037844383745, -136.3750000040967905 ) ) ;
#6506=ORIENTED_EDGE ( 'NONE', *, *, #3873, .F. ) ;
#6507=CARTESIAN_POINT ( 'NONE',  ( 9.999999999999998224, 0.000000000000000000, -40.99999999999997868 ) ) ;
#6508=EDGE_CURVE ( 'NONE', #5998, #8957, #30898, .T. ) ;
#6509=CARTESIAN_POINT ( 'NONE',  ( 5.000000000000000000, 8.660254037844385522, -15.62500000409675138 ) ) ;
#6510=CARTESIAN_POINT ( 'NONE',  ( -5.405949406249996869, 9.363379034771805109, -41.53125000204838102 ) ) ;
#6513=LINE ( 'NONE', #3068, #37623 ) ;
#6514=CARTESIAN_POINT ( 'NONE',  ( -10.81189881249999907, -6.242252689847864744, -138.6562500020484094 ) ) ;
#6515=CARTESIAN_POINT ( 'NONE',  ( 10.81189881249999551, -6.242252689847874514, -138.1562500020484094 ) ) ;
#6516=CARTESIAN_POINT ( 'NONE',  ( 10.00000000000051159, -5.773502691895965988, -123.6250000000000142 ) ) ;
#6517=EDGE_LOOP ( 'NONE', ( #1159, #8804, #2499, #4989 ) ) ;
#6518=VERTEX_POINT ( 'NONE', #36520 ) ;
#6519=ORIENTED_EDGE ( 'NONE', *, *, #12748, .T. ) ;
#6521=CARTESIAN_POINT ( 'NONE',  ( -10.81189881249999729, 1.324075727343319199E-15, -173.0937500020484094 ) ) ;
#6522=CARTESIAN_POINT ( 'NONE',  ( 7.644554776091147741E-16, 12.48450537969573659, -26.46875000204837747 ) ) ;
#6523=CARTESIAN_POINT ( 'NONE',  ( -9.999999999999998224, 1.224646799147353059E-15, -111.1250000040967763 ) ) ;
#6524=CARTESIAN_POINT ( 'NONE',  ( 5.405949406249999534, 9.363379034771803333, -155.5937500020483810 ) ) ;
#6525=CARTESIAN_POINT ( 'NONE',  ( -2.293366432827344421E-15, -12.48450537969573659, -141.2187500020483810 ) ) ;
#6526=CARTESIAN_POINT ( 'NONE',  ( -9.999999999999998224, 1.224646799147353059E-15, -200.0000000000000000 ) ) ;
#6529=CARTESIAN_POINT ( 'NONE',  ( 7.644554776091147741E-16, 12.48450537969573659, -21.96875000204837391 ) ) ;
#6531=DIRECTION ( 'NONE',  ( -0.000000000000000000, -0.000000000000000000, 1.000000000000000000 ) ) ;
#6532=CARTESIAN_POINT ( 'NONE',  ( -4.999999999999996447, 8.660254037844387298, -25.49999999999996803 ) ) ;
#6535=CARTESIAN_POINT ( 'NONE',  ( 7.644554776091147741E-16, 12.48450537969573659, -71.46875000204838102 ) ) ;
#6536=CARTESIAN_POINT ( 'NONE',  ( 10.81189881249999907, 6.242252689847868297, -41.90625000204836681 ) ) ;
#6540=CARTESIAN_POINT ( 'NONE',  ( -9.999999999999998224, 1.224646799147353059E-15, -136.2499999999999716 ) ) ;
#6541=CARTESIAN_POINT ( 'NONE',  ( 10.81189881249999729, 6.242252689847867408, -134.9062500020483810 ) ) ;
#6542=CARTESIAN_POINT ( 'NONE',  ( 10.00000000000051159, -5.773502691895965988, -98.50000000409677625 ) ) ;
#6543=CARTESIAN_POINT ( 'NONE',  ( 5.000000000000000000, 8.660254037844385522, -117.6250000040967905 ) ) ;
#6545=VERTEX_POINT ( 'NONE', #36100 ) ;
#6548=CARTESIAN_POINT ( 'NONE',  ( -5.000000000000003553, -8.660254037844383745, -48.99999999999998579 ) ) ;
#6549=CARTESIAN_POINT ( 'NONE',  ( -2.293366432827344421E-15, -12.48450537969573659, -172.9062500020484379 ) ) ;
#6550=CARTESIAN_POINT ( 'NONE',  ( 9.999999999999996447, -5.773502691896262640, -38.50000000409676915 ) ) ;
#6551=CARTESIAN_POINT ( 'NONE',  ( -2.121150477449813534E-15, -11.54700538379251284, -91.25000000409677625 ) ) ;
#6553=CARTESIAN_POINT ( 'NONE',  ( 9.999999999999998224, 0.000000000000000000, -45.49999999999998579 ) ) ;
#6554=CARTESIAN_POINT ( 'NONE',  ( -2.293366432827344421E-15, -12.48450537969573659, -159.4062500020483810 ) ) ;
#6555=CARTESIAN_POINT ( 'NONE',  ( 10.81189881249999551, -6.242252689847874514, -145.4687500020483810 ) ) ;
#6556=DIRECTION ( 'NONE',  ( 0.000000000000000000, 0.000000000000000000, 1.000000000000000000 ) ) ;
#6557=LINE ( 'NONE', #32894, #17166 ) ;
#6558=ORIENTED_EDGE ( 'NONE', *, *, #18255, .T. ) ;
#6559=CARTESIAN_POINT ( 'NONE',  ( -9.999999999999998224, 1.224646799147353059E-15, -189.1250000040967905 ) ) ;
#6560=EDGE_CURVE ( 'NONE', #7227, #28673, #29016, .T. ) ;
#6561=CARTESIAN_POINT ( 'NONE',  ( 5.405949406249992428, -9.363379034771808662, -73.78125000204838102 ) ) ;
#6562=ORIENTED_EDGE ( 'NONE', *, *, #32262, .T. ) ;
#6563=CARTESIAN_POINT ( 'NONE',  ( 10.81189881249999729, 0.000000000000000000, -118.3437500020483810 ) ) ;
#6564=VERTEX_POINT ( 'NONE', #16646 ) ;
#6565=VERTEX_POINT ( 'NONE', #33304 ) ;
#6567=CARTESIAN_POINT ( 'NONE',  ( 10.81189881249999729, 6.242252689847867408, -20.71875000204836681 ) ) ;
#6568=CARTESIAN_POINT ( 'NONE',  ( -2.293366432827344421E-15, -12.48450537969573659, -1.906250002048373027 ) ) ;
#6569=CARTESIAN_POINT ( 'NONE',  ( 10.81189881249999551, -6.242252689847874514, -46.46875000204837391 ) ) ;
#6572=CARTESIAN_POINT ( 'NONE',  ( 10.81189881249999729, 6.242252689847867408, -176.7187500020484094 ) ) ;
#6573=CARTESIAN_POINT ( 'NONE',  ( 10.81189881249999907, 6.242252689847868297, -167.7187500020483810 ) ) ;
#6576=CARTESIAN_POINT ( 'NONE',  ( 10.00000000000051159, -5.773502691895965988, -104.5000000040967620 ) ) ;
#6577=CYLINDRICAL_SURFACE ( 'NONE', #9513, 9.999999999999998224 ) ;
#6579=CARTESIAN_POINT ( 'NONE',  ( 10.81189881249999729, 0.000000000000000000, -94.34375000204838102 ) ) ;
#6580=EDGE_CURVE ( 'NONE', #29342, #14673, #39964, .T. ) ;
#6582=CARTESIAN_POINT ( 'NONE',  ( 7.644554776091147741E-16, 12.48450537969573659, -70.15625000204839523 ) ) ;
#6583=CARTESIAN_POINT ( 'NONE',  ( -2.121150477449813534E-15, -11.54700538379251284, -5.374999999999961808 ) ) ;
#6585=CARTESIAN_POINT ( 'NONE',  ( -2.293366432827344421E-15, -12.48450537969573659, -165.4062500020483526 ) ) ;
#6587=CARTESIAN_POINT ( 'NONE',  ( -10.00000000000000000, -5.773502691896251982, -141.0000000040967905 ) ) ;
#6589=ORIENTED_EDGE ( 'NONE', *, *, #5190, .F. ) ;
#6592=CARTESIAN_POINT ( 'NONE',  ( -10.81189881249999729, 1.324075727343319199E-15, -198.7812500020484094 ) ) ;
#6595=VERTEX_POINT ( 'NONE', #22946 ) ;
#6596=CARTESIAN_POINT ( 'NONE',  ( 9.999999999999998224, 0.000000000000000000, -58.99999999999997158 ) ) ;
#6598=CARTESIAN_POINT ( 'NONE',  ( 5.000000000000000000, 8.660254037844385522, -66.62500000409676204 ) ) ;
#6599=DIRECTION ( 'NONE',  ( 1.000000000000000000, 0.000000000000000000, 0.000000000000000000 ) ) ;
#6600=CARTESIAN_POINT ( 'NONE',  ( -2.121150477449813534E-15, -11.54700538379251284, -160.2500000040967620 ) ) ;
#6602=CARTESIAN_POINT ( 'NONE',  ( 5.405949406249999534, 9.363379034771803333, -59.78125000204836681 ) ) ;
#6603=( BOUNDED_CURVE ( )  B_SPLINE_CURVE ( 2, ( #19403, #35191, #2808, #28929, #32593, #35825, #38841 ),
 .UNSPECIFIED., .F., .F. ) 
 B_SPLINE_CURVE_WITH_KNOTS ( ( 3, 2, 2, 3 ),
 ( 0.5447761194029852039, 0.5460199004975125892, 0.5472636815920398634, 0.5485074626865672487 ),
 .UNSPECIFIED. ) 
 CURVE ( )  GEOMETRIC_REPRESENTATION_ITEM ( )  RATIONAL_B_SPLINE_CURVE ( ( 0.9999999999999880096, 0.8660254037844506980, 1.000000000000000000, 0.8660254037844387076, 1.000000000000000000, 0.8660254037844267172, 1.000000000000011990 ) ) 
 REPRESENTATION_ITEM ( '' )  );
#6604=AXIS2_PLACEMENT_3D ( 'NONE', #29393, #9947, #36497 ) ;
#6607=CARTESIAN_POINT ( 'NONE',  ( 9.999999999999998224, 0.000000000000000000, -38.37500000409676915 ) ) ;
#6608=CARTESIAN_POINT ( 'NONE',  ( -5.405949406249996869, 9.363379034771805109, -184.0312500020484094 ) ) ;
#6610=CARTESIAN_POINT ( 'NONE',  ( 9.999999999999998224, 0.000000000000000000, -85.99999999999998579 ) ) ;
#6612=CIRCLE ( 'NONE', #30738, 10.00000000000000178 ) ;
#6615=( BOUNDED_CURVE ( )  B_SPLINE_CURVE ( 2, ( #20275, #17658, #36891, #4307, #4095, #21124, #37534 ),
 .UNSPECIFIED., .F., .F. ) 
 B_SPLINE_CURVE_WITH_KNOTS ( ( 3, 2, 2, 3 ),
 ( 0.3805970149253732338, 0.3818407960199006190, 0.3830845771144278933, 0.3843283582089552786 ),
 .UNSPECIFIED. ) 
 CURVE ( )  GEOMETRIC_REPRESENTATION_ITEM ( )  RATIONAL_B_SPLINE_CURVE ( ( 0.9999999999999880096, 0.8660254037844506980, 1.000000000000000000, 0.8660254037844387076, 1.000000000000000000, 0.8660254037844327124, 1.000000000000005995 ) ) 
 REPRESENTATION_ITEM ( '' )  );
#6616=CARTESIAN_POINT ( 'NONE',  ( -5.000000000000003553, -8.660254037844383745, -170.5000000000000000 ) ) ;
#6617=CARTESIAN_POINT ( 'NONE',  ( 10.81189881249999907, 6.242252689847868297, -97.40625000204839523 ) ) ;
#6618=EDGE_LOOP ( 'NONE', ( #21421, #7789, #41950, #5568 ) ) ;
#6619=CARTESIAN_POINT ( 'NONE',  ( 9.999999999998969713, 5.773502691896851502, -83.25000000409676204 ) ) ;
#6620=EDGE_CURVE ( 'NONE', #27209, #10842, #20676, .T. ) ;
#6621=CARTESIAN_POINT ( 'NONE',  ( 9.999999999999998224, 0.000000000000000000, -24.49999999999996447 ) ) ;
#6622=ORIENTED_EDGE ( 'NONE', *, *, #37625, .F. ) ;
#6623=ORIENTED_EDGE ( 'NONE', *, *, #18083, .T. ) ;
#6624=CARTESIAN_POINT ( 'NONE',  ( -5.405949406250003975, -9.363379034771801557, -33.34375000204836681 ) ) ;
#6625=CARTESIAN_POINT ( 'NONE',  ( 5.405949406249992428, -9.363379034771808662, -25.78125000204836681 ) ) ;
#6628=CARTESIAN_POINT ( 'NONE',  ( 10.81189881249999551, -6.242252689847874514, -74.96875000204838102 ) ) ;
#6629=DIRECTION ( 'NONE',  ( 0.000000000000000000, 0.000000000000000000, -1.000000000000000000 ) ) ;
#6630=CARTESIAN_POINT ( 'NONE',  ( 5.405949406249999534, 9.363379034771803333, -190.0937500020483810 ) ) ;
#6632=CARTESIAN_POINT ( 'NONE',  ( 9.999999999999998224, 0.000000000000000000, -78.87500000409677625 ) ) ;
#6635=CARTESIAN_POINT ( 'NONE',  ( -4.999999999999996447, 8.660254037844387298, -3.375000004096767370 ) ) ;
#6637=CARTESIAN_POINT ( 'NONE',  ( -5.405949406249996869, 9.363379034771805109, -117.8437500020483810 ) ) ;
#6638=CARTESIAN_POINT ( 'NONE',  ( -5.405949406249996869, 9.363379034771805109, -100.0312500020483952 ) ) ;
#6639=CARTESIAN_POINT ( 'NONE',  ( -5.405949406250003975, -9.363379034771801557, -108.3437500020483810 ) ) ;
#6642=CARTESIAN_POINT ( 'NONE',  ( 5.000000000000000000, 8.660254037844385522, -164.1250000040967905 ) ) ;
#6643=FACE_OUTER_BOUND ( 'NONE', #1005, .T. ) ;
#6649=CARTESIAN_POINT ( 'NONE',  ( -9.999999999999998224, 1.224646799147353059E-15, -54.12500000409675494 ) ) ;
#6651=CARTESIAN_POINT ( 'NONE',  ( -9.999999999999998224, 5.773502691896259087, -77.87499999999998579 ) ) ;
#6653=CARTESIAN_POINT ( 'NONE',  ( 9.999999999999996447, -5.773502691896262640, -94.00000000409677625 ) ) ;
#6654=CARTESIAN_POINT ( 'NONE',  ( 0.000000000000000000, 0.000000000000000000, -200.0000000000000000 ) ) ;
#6656=CARTESIAN_POINT ( 'NONE',  ( -5.405949406250003975, -9.363379034771801557, -93.53125000204838102 ) ) ;
#6657=EDGE_LOOP ( 'NONE', ( #21542, #13231, #19181, #40618 ) ) ;
#6659=CARTESIAN_POINT ( 'NONE',  ( -4.999999999999996447, 8.660254037844387298, -47.99999999999998579 ) ) ;
#6661=VERTEX_POINT ( 'NONE', #9555 ) ;
#6662=CARTESIAN_POINT ( 'NONE',  ( 10.00000000000000000, 5.773502691896255534, -12.37499999999996270 ) ) ;
#6663=CARTESIAN_POINT ( 'NONE',  ( -9.999999999999998224, 5.773502691896259087, -142.3750000000000000 ) ) ;
#6664=CARTESIAN_POINT ( 'NONE',  ( -2.121150477449813534E-15, -11.54700538379251284, -32.37499999999995737 ) ) ;
#6666=CARTESIAN_POINT ( 'NONE',  ( -5.000000000000003553, -8.660254037844383745, -190.0000000000000000 ) ) ;
#6667=CARTESIAN_POINT ( 'NONE',  ( 5.405949406249992428, -9.363379034771808662, -117.2812500020483952 ) ) ;
#6669=CARTESIAN_POINT ( 'NONE',  ( 0.000000000000000000, 0.000000000000000000, -200.0000000000000000 ) ) ;
#6671=EDGE_CURVE ( 'NONE', #3950, #37390, #29514, .T. ) ;
#6672=ORIENTED_EDGE ( 'NONE', *, *, #24644, .T. ) ;
#6673=EDGE_CURVE ( 'NONE', #9647, #31274, #39709, .T. ) ;
#6674=CARTESIAN_POINT ( 'NONE',  ( 10.81189881249999551, -6.242252689847874514, -45.15625000204836681 ) ) ;
#6676=CARTESIAN_POINT ( 'NONE',  ( 10.81189881249999551, -6.242252689847874514, -91.46875000204838102 ) ) ;
#6677=CARTESIAN_POINT ( 'NONE',  ( 10.81189881249999551, -6.242252689847874514, -123.1562500020483952 ) ) ;
#6678=ORIENTED_EDGE ( 'NONE', *, *, #8111, .F. ) ;
#6681=CARTESIAN_POINT ( 'NONE',  ( -9.999999999999998224, 1.224646799147353059E-15, -0.1250000040967647053 ) ) ;
#6682=ADVANCED_FACE ( 'NONE', ( #4559 ), #23777, .T. ) ;
#6683=CARTESIAN_POINT ( 'NONE',  ( -5.405949406249996869, 9.363379034771805109, -131.3437500020484094 ) ) ;
#6684=( BOUNDED_CURVE ( )  B_SPLINE_CURVE ( 2, ( #33302, #38914, #42556, #284, #19896, #29416, #6116 ),
 .UNSPECIFIED., .F., .F. ) 
 B_SPLINE_CURVE_WITH_KNOTS ( ( 3, 2, 2, 3 ),
 ( 0.3955223880597015795, 0.3967661691542289648, 0.3980099502487563501, 0.3992537313432836799 ),
 .UNSPECIFIED. ) 
 CURVE ( )  GEOMETRIC_REPRESENTATION_ITEM ( )  RATIONAL_B_SPLINE_CURVE ( ( 0.9999999999999880096, 0.8660254037844506980, 1.000000000000000000, 0.8660254037844387076, 1.000000000000000000, 0.8660254037844267172, 1.000000000000011990 ) ) 
 REPRESENTATION_ITEM ( '' )  );
#6688=CARTESIAN_POINT ( 'NONE',  ( 9.999999999999998224, 0.000000000000000000, -182.3750000040967905 ) ) ;
#6690=CARTESIAN_POINT ( 'NONE',  ( 10.81189881249999729, 0.000000000000000000, -183.0312500020484094 ) ) ;
#6691=LINE ( 'NONE', #23312, #24083 ) ;
#6692=CARTESIAN_POINT ( 'NONE',  ( 5.000000000000000000, 8.660254037844385522, -185.1250000040967905 ) ) ;
#6695=ADVANCED_FACE ( 'NONE', ( #23358 ), #7585, .T. ) ;
#6696=CARTESIAN_POINT ( 'NONE',  ( 10.81189881249999729, 0.000000000000000000, -56.84375000204835970 ) ) ;
#6697=CARTESIAN_POINT ( 'NONE',  ( 10.81189881249999729, 0.000000000000000000, -46.34375000204838102 ) ) ;
#6699=CARTESIAN_POINT ( 'NONE',  ( -5.405949406249996869, 9.363379034771805109, -17.53125000204835970 ) ) ;
#6701=CARTESIAN_POINT ( 'NONE',  ( -10.00000000000154188, 5.773502691895366468, -27.25000000409673007 ) ) ;
#6703=CARTESIAN_POINT ( 'NONE',  ( -10.00000000000000000, -5.773502691896251982, -103.1249999999999858 ) ) ;
#6705=EDGE_CURVE ( 'NONE', #39621, #31210, #33928, .T. ) ;
#6709=CARTESIAN_POINT ( 'NONE',  ( -10.81189881249999729, 1.324075727343319199E-15, -119.2812500020483952 ) ) ;
#6711=CARTESIAN_POINT ( 'NONE',  ( 7.070501591499376803E-16, 11.54700538379251284, -160.6250000000000284 ) ) ;
#6713=CARTESIAN_POINT ( 'NONE',  ( 4.999999999999992006, -8.660254037844389075, -194.6250000040967905 ) ) ;
#6715=VERTEX_POINT ( 'NONE', #16848 ) ;
#6716=CARTESIAN_POINT ( 'NONE',  ( -5.000000000000003553, -8.660254037844383745, -33.99999999999997158 ) ) ;
#6717=CARTESIAN_POINT ( 'NONE',  ( -4.999999999999996447, 8.660254037844387298, -19.87500000409675494 ) ) ;
#6718=CARTESIAN_POINT ( 'NONE',  ( 7.644554776091147741E-16, 12.48450537969573659, -47.65625000204836681 ) ) ;
#6719=ADVANCED_FACE ( 'NONE', ( #33708 ), #36717, .T. ) ;
#6723=CARTESIAN_POINT ( 'NONE',  ( -2.293366432827344421E-15, -12.48450537969573659, -144.4062500020484094 ) ) ;
#6724=CARTESIAN_POINT ( 'NONE',  ( -9.999999999999998224, 1.224646799147353059E-15, -42.12500000409677625 ) ) ;
#6726=ORIENTED_EDGE ( 'NONE', *, *, #11274, .T. ) ;
#6727=VERTEX_POINT ( 'NONE', #27440 ) ;
#6728=CARTESIAN_POINT ( 'NONE',  ( -5.000000000000003553, -8.660254037844383745, -130.0000000000000000 ) ) ;
#6729=( BOUNDED_CURVE ( )  B_SPLINE_CURVE ( 2, ( #33980, #41057, #36989, #4402, #7862, #30743, #40849 ),
 .UNSPECIFIED., .F., .F. ) 
 B_SPLINE_CURVE_WITH_KNOTS ( ( 3, 2, 2, 3 ),
 ( 0.7798507462686569136, 0.7810945273631842989, 0.7823383084577115731, 0.7835820895522389584 ),
 .UNSPECIFIED. ) 
 CURVE ( )  GEOMETRIC_REPRESENTATION_ITEM ( )  RATIONAL_B_SPLINE_CURVE ( ( 0.9999999999999761302, 0.8660254037844625774, 1.000000000000000000, 0.8660254037844387076, 1.000000000000000000, 0.8660254037844267172, 1.000000000000011990 ) ) 
 REPRESENTATION_ITEM ( '' )  );
#6730=CARTESIAN_POINT ( 'NONE',  ( -10.81189881249999729, 1.324075727343319199E-15, -177.5937500020484094 ) ) ;
#6731=CARTESIAN_POINT ( 'NONE',  ( 5.405949406249999534, 9.363379034771803333, -25.09375000204835970 ) ) ;
#6732=AXIS2_PLACEMENT_3D ( 'NONE', #27869, #14682, #34567 ) ;
#6733=CARTESIAN_POINT ( 'NONE',  ( 10.81189881249999729, 0.000000000000000000, -152.8437500020483810 ) ) ;
#6734=VECTOR ( 'NONE', #38055, 1000.000000000000000 ) ;
#6735=CARTESIAN_POINT ( 'NONE',  ( -5.405949406249996869, 9.363379034771805109, -144.8437500020483810 ) ) ;
#6736=LINE ( 'NONE', #6526, #32129 ) ;
#6739=CARTESIAN_POINT ( 'NONE',  ( -10.81189881249999729, 1.324075727343319199E-15, -18.59375000204835260 ) ) ;
#6741=ADVANCED_FACE ( 'NONE', ( #7374 ), #34140, .T. ) ;
#6743=LINE ( 'NONE', #29846, #22016 ) ;
#6745=CARTESIAN_POINT ( 'NONE',  ( -10.00000000000102496, 5.773502691895664007, -55.75000000409674072 ) ) ;
#6746=CARTESIAN_POINT ( 'NONE',  ( -5.405949406249996869, 9.363379034771805109, -75.84375000204838102 ) ) ;
#6747=CARTESIAN_POINT ( 'NONE',  ( -10.81189881249999729, 1.324075727343319199E-15, -44.28125000204838102 ) ) ;
#6750=CARTESIAN_POINT ( 'NONE',  ( -9.999999999999998224, 5.773502691896259087, -131.8749999999999716 ) ) ;
#6751=CARTESIAN_POINT ( 'NONE',  ( 10.81189881249999551, -6.242252689847874514, -135.1562500020483810 ) ) ;
#6753=CARTESIAN_POINT ( 'NONE',  ( 9.999999999999996447, -5.773502691896262640, -113.5000000040967763 ) ) ;
#6755=EDGE_LOOP ( 'NONE', ( #7989, #39422, #27911, #36759 ) ) ;
#6759=CARTESIAN_POINT ( 'NONE',  ( 5.405949406249992428, -9.363379034771808662, -163.7812500020484094 ) ) ;
#6760=CARTESIAN_POINT ( 'NONE',  ( 4.999999999999992006, -8.660254037844389075, -40.12500000409676915 ) ) ;
#6761=CARTESIAN_POINT ( 'NONE',  ( 9.999999999999998224, 0.000000000000000000, -26.37500000409676204 ) ) ;
#6763=DIRECTION ( 'NONE',  ( 1.000000000000000000, 0.000000000000000000, 0.000000000000000000 ) ) ;
#6764=CARTESIAN_POINT ( 'NONE',  ( 10.81189881249999729, 0.000000000000000000, -162.0312500020484094 ) ) ;
#6765=CARTESIAN_POINT ( 'NONE',  ( 7.644554776091147741E-16, 12.48450537969573659, -131.4687500020483810 ) ) ;
#6766=CARTESIAN_POINT ( 'NONE',  ( -9.999999999999998224, 1.224646799147353059E-15, -200.0000000000000000 ) ) ;
#6768=VECTOR ( 'NONE', #16694, 1000.000000000000000 ) ;
#6769=EDGE_LOOP ( 'NONE', ( #11755, #31426, #30833, #8115 ) ) ;
#6770=CARTESIAN_POINT ( 'NONE',  ( 4.999999999999992006, -8.660254037844389075, -30.74999999999997158 ) ) ;
#6771=CARTESIAN_POINT ( 'NONE',  ( -10.81189881249999729, 1.324075727343319199E-15, -71.28125000204838102 ) ) ;
#6774=CARTESIAN_POINT ( 'NONE',  ( 10.81189881249999907, 6.242252689847868297, -119.7187500020483810 ) ) ;
#6777=CARTESIAN_POINT ( 'NONE',  ( -10.81189881249999729, -6.242252689847864744, -21.46875000204837036 ) ) ;
#6778=CARTESIAN_POINT ( 'NONE',  ( -10.81189881249999729, 1.324075727343319199E-15, -197.0937500020484094 ) ) ;
#6780=CARTESIAN_POINT ( 'NONE',  ( -10.81189881249999729, 1.324075727343319199E-15, -48.59375000204838102 ) ) ;
#6781=EDGE_CURVE ( 'NONE', #26104, #20093, #20309, .T. ) ;
#6782=FACE_OUTER_BOUND ( 'NONE', #28411, .T. ) ;
#6784=CARTESIAN_POINT ( 'NONE',  ( -10.81189881249999729, 1.324075727343319199E-15, -183.5937500020483810 ) ) ;
#6785=CARTESIAN_POINT ( 'NONE',  ( 5.405949406249992428, -9.363379034771808662, -169.5937500020484094 ) ) ;
#6788=CARTESIAN_POINT ( 'NONE',  ( 9.999999999999998224, 0.000000000000000000, -117.8750000040967905 ) ) ;
#6789=DIRECTION ( 'NONE',  ( -0.000000000000000000, -0.000000000000000000, 1.000000000000000000 ) ) ;
#6791=CARTESIAN_POINT ( 'NONE',  ( 10.81189881249999907, 6.242252689847868297, -98.71875000204838102 ) ) ;
#6792=CARTESIAN_POINT ( 'NONE',  ( -9.999999999999998224, 1.224646799147353059E-15, -101.7500000000000000 ) ) ;
#6793=CARTESIAN_POINT ( 'NONE',  ( 10.81189881249999729, 0.000000000000000000, -64.53125000204836681 ) ) ;
#6794=CARTESIAN_POINT ( 'NONE',  ( 9.999999999999998224, 0.000000000000000000, -96.87500000409677625 ) ) ;
#6796=CARTESIAN_POINT ( 'NONE',  ( 10.81189881249999729, 0.000000000000000000, -123.0312500020483952 ) ) ;
#6798=CARTESIAN_POINT ( 'NONE',  ( -5.405949406250003975, -9.363379034771801557, -165.5312500020484094 ) ) ;
#6801=CARTESIAN_POINT ( 'NONE',  ( 7.070501591499377789E-16, 11.54700538379251284, -140.0000000040968189 ) ) ;
#6803=ADVANCED_FACE ( 'NONE', ( #40578 ), #33925, .T. ) ;
#6804=ORIENTED_EDGE ( 'NONE', *, *, #15885, .T. ) ;
#6807=CARTESIAN_POINT ( 'NONE',  ( 10.81189881249999551, -6.242252689847874514, -186.1562500020484379 ) ) ;
#6808=CARTESIAN_POINT ( 'NONE',  ( 9.999999999999998224, 0.000000000000000000, -200.0000000000000000 ) ) ;
#6810=VERTEX_POINT ( 'NONE', #7157 ) ;
#6811=CARTESIAN_POINT ( 'NONE',  ( -9.999999999999998224, 5.773502691896259087, -59.87499999999999289 ) ) ;
#6813=CARTESIAN_POINT ( 'NONE',  ( -9.999999999999998224, 1.224646799147353059E-15, -64.62500000409676204 ) ) ;
#6814=CARTESIAN_POINT ( 'NONE',  ( 9.999999999998456346, 5.773502691897149042, -21.75000000409673007 ) ) ;
#6815=CARTESIAN_POINT ( 'NONE',  ( 0.000000000000000000, 0.000000000000000000, -200.0000000000000000 ) ) ;
#6817=CARTESIAN_POINT ( 'NONE',  ( 10.81189881249999551, -6.242252689847874514, -58.65625000204837391 ) ) ;
#6820=CARTESIAN_POINT ( 'NONE',  ( 0.000000000000000000, 0.000000000000000000, -200.0000000000000000 ) ) ;
#6821=CARTESIAN_POINT ( 'NONE',  ( 10.81189881249999729, 0.000000000000000000, -189.0312500020484094 ) ) ;
#6823=DIRECTION ( 'NONE',  ( -0.000000000000000000, -0.000000000000000000, 1.000000000000000000 ) ) ;
#6824=CARTESIAN_POINT ( 'NONE',  ( -9.433396038363706992, 3.431119748995231422, -0.000000000000000000 ) ) ;
#6825=CARTESIAN_POINT ( 'NONE',  ( 5.000000000000000000, 8.660254037844385522, -169.7500000000000000 ) ) ;
#6826=CARTESIAN_POINT ( 'NONE',  ( 9.999999999999994671, -5.773502691896262640, -137.5000000040967905 ) ) ;
#6827=CARTESIAN_POINT ( 'NONE',  ( 7.644554776091147741E-16, 12.48450537969573659, -91.15625000204838102 ) ) ;
#6828=ORIENTED_EDGE ( 'NONE', *, *, #3873, .T. ) ;
#6829=CARTESIAN_POINT ( 'NONE',  ( 9.999999999999998224, 0.000000000000000000, -107.3750000040967763 ) ) ;
#6830=CARTESIAN_POINT ( 'NONE',  ( -9.999999999999998224, 1.224646799147353059E-15, -161.7500000000000000 ) ) ;
#6831=VERTEX_POINT ( 'NONE', #40159 ) ;
#6832=EDGE_LOOP ( 'NONE', ( #14825, #22223, #19986, #23822 ) ) ;
#6834=CARTESIAN_POINT ( 'NONE',  ( -5.405949406249996869, 9.363379034771805109, -32.34375000204836681 ) ) ;
#6835=CARTESIAN_POINT ( 'NONE',  ( 10.81189881249999551, -6.242252689847874514, -24.15625000204838102 ) ) ;
#6838=CARTESIAN_POINT ( 'NONE',  ( -2.293366432827344421E-15, -12.48450537969573659, -69.21875000204839523 ) ) ;
#6840=CARTESIAN_POINT ( 'NONE',  ( -10.81189881249999907, -6.242252689847864744, -189.4687500020484094 ) ) ;
#6841=CARTESIAN_POINT ( 'NONE',  ( 7.644554776091147741E-16, 12.48450537969573659, -149.4687500020484094 ) ) ;
#6844=CARTESIAN_POINT ( 'NONE',  ( -4.999999999999996447, 8.660254037844387298, -112.4999999999999858 ) ) ;
#6846=CARTESIAN_POINT ( 'NONE',  ( 9.999999999999998224, 0.000000000000000000, -5.375000004096769146 ) ) ;
#6847=CARTESIAN_POINT ( 'NONE',  ( 9.999999999999998224, 0.000000000000000000, -125.0000000000000000 ) ) ;
#6848=CARTESIAN_POINT ( 'NONE',  ( -5.405949406250003975, -9.363379034771801557, -117.3437500020483810 ) ) ;
#6849=CARTESIAN_POINT ( 'NONE',  ( 9.999999999999479527, 5.773502691896553074, -109.8749999999999716 ) ) ;
#6850=CARTESIAN_POINT ( 'NONE',  ( 10.81189881249999907, 6.242252689847868297, -89.90625000204839523 ) ) ;
#6851=CARTESIAN_POINT ( 'NONE',  ( -5.405949406250003975, -9.363379034771801557, -106.8437500020483810 ) ) ;
#6854=CARTESIAN_POINT ( 'NONE',  ( -9.999999999999998224, 5.773502691896259087, -165.2500000040967905 ) ) ;
#6855=( BOUNDED_CURVE ( )  B_SPLINE_CURVE ( 2, ( #3606, #6619, #36603, #19985, #29720, #23455, #23669 ),
 .UNSPECIFIED., .F., .F. ) 
 B_SPLINE_CURVE_WITH_KNOTS ( ( 3, 2, 2, 3 ),
 ( 0.5746268656716420065, 0.5758706467661693917, 0.5771144278606968880, 0.5783582089552241623 ),
 .UNSPECIFIED. ) 
 CURVE ( )  GEOMETRIC_REPRESENTATION_ITEM ( )  RATIONAL_B_SPLINE_CURVE ( ( 0.9999999999999761302, 0.8660254037844625774, 1.000000000000000000, 0.8660254037844387076, 1.000000000000000000, 0.8660254037844028474, 1.000000000000035971 ) ) 
 REPRESENTATION_ITEM ( '' )  );
#6861=CARTESIAN_POINT ( 'NONE',  ( 10.00000000000051159, -5.773502691895965988, -149.1249999999999716 ) ) ;
#6864=CARTESIAN_POINT ( 'NONE',  ( -9.999999999999998224, 5.773502691896259087, -79.37500000000000000 ) ) ;
#6866=CARTESIAN_POINT ( 'NONE',  ( 9.999999999999998224, 0.000000000000000000, -90.87500000409677625 ) ) ;
#6867=CARTESIAN_POINT ( 'NONE',  ( -9.999999999999998224, 1.224646799147353059E-15, -150.1250000040967905 ) ) ;
#6869=CARTESIAN_POINT ( 'NONE',  ( 7.644554776091147741E-16, 12.48450537969573659, -85.15625000204838102 ) ) ;
#6870=ORIENTED_EDGE ( 'NONE', *, *, #23177, .T. ) ;
#6872=CARTESIAN_POINT ( 'NONE',  ( -9.999999999999998224, 1.224646799147353059E-15, -154.2500000000000000 ) ) ;
#6874=VERTEX_POINT ( 'NONE', #27652 ) ;
#6875=CARTESIAN_POINT ( 'NONE',  ( -4.999999999999996447, 8.660254037844387298, -11.99999999999995559 ) ) ;
#6877=CARTESIAN_POINT ( 'NONE',  ( 4.999999999999992006, -8.660254037844389075, -144.7500000000000000 ) ) ;
#6878=FACE_OUTER_BOUND ( 'NONE', #22429, .T. ) ;
#6880=CARTESIAN_POINT ( 'NONE',  ( 10.00000000000000000, 5.773502691896255534, -187.8750000000000568 ) ) ;
#6881=LINE ( 'NONE', #39673, #10980 ) ;
#6882=CARTESIAN_POINT ( 'NONE',  ( 10.81189881249999729, 0.000000000000000000, -121.5312500020483952 ) ) ;
#6884=DIRECTION ( 'NONE',  ( -0.000000000000000000, -0.000000000000000000, 1.000000000000000000 ) ) ;
#6885=VERTEX_POINT ( 'NONE', #40793 ) ;
#6886=CARTESIAN_POINT ( 'NONE',  ( -10.81189881249999907, -6.242252689847864744, -48.65625000204836681 ) ) ;
#6888=CARTESIAN_POINT ( 'NONE',  ( 5.405949406249992428, -9.363379034771808662, -97.59375000204838102 ) ) ;
#6889=CARTESIAN_POINT ( 'NONE',  ( 5.405949406249992428, -9.363379034771808662, -123.2812500020483952 ) ) ;
#6891=CARTESIAN_POINT ( 'NONE',  ( 4.999999999999992006, -8.660254037844389075, -111.7499999999999858 ) ) ;
#6892=DIRECTION ( 'NONE',  ( -0.000000000000000000, -0.000000000000000000, 1.000000000000000000 ) ) ;
#6894=DIRECTION ( 'NONE',  ( 1.000000000000000000, 0.000000000000000000, 0.000000000000000000 ) ) ;
#6895=VECTOR ( 'NONE', #24520, 1000.000000000000000 ) ;
#6896=CARTESIAN_POINT ( 'NONE',  ( 10.81189881249999729, 0.000000000000000000, -134.8437500020484094 ) ) ;
#6898=DIRECTION ( 'NONE',  ( 1.000000000000000000, 0.000000000000000000, 0.000000000000000000 ) ) ;
#6900=CARTESIAN_POINT ( 'NONE',  ( -4.999999999999996447, 8.660254037844387298, -186.3750000040967905 ) ) ;
#6902=CARTESIAN_POINT ( 'NONE',  ( -10.81189881249999729, 1.324075727343319199E-15, -188.2812500020484094 ) ) ;
#6906=CARTESIAN_POINT ( 'NONE',  ( 5.405949406249999534, 9.363379034771803333, -62.59375000204836681 ) ) ;
#6907=CARTESIAN_POINT ( 'NONE',  ( -10.81189881249999729, 6.242252689847871849, -47.21875000204836681 ) ) ;
#6909=CARTESIAN_POINT ( 'NONE',  ( -5.405949406249996869, 9.363379034771805109, -20.53125000204836326 ) ) ;
#6914=CARTESIAN_POINT ( 'NONE',  ( -10.00000000000000000, -5.773502691896251982, -104.6249999999999858 ) ) ;
#6917=ADVANCED_FACE ( 'NONE', ( #22192 ), #37790, .T. ) ;
#6920=CARTESIAN_POINT ( 'NONE',  ( -2.293366432827344421E-15, -12.48450537969573659, -103.9062500020483810 ) ) ;
#6924=CARTESIAN_POINT ( 'NONE',  ( 4.999999999999992006, -8.660254037844389075, -136.1250000040967620 ) ) ;
#6926=ORIENTED_EDGE ( 'NONE', *, *, #32437, .T. ) ;
#6927=CARTESIAN_POINT ( 'NONE',  ( 9.999999999999996447, -5.773502691896262640, -32.12499999999995737 ) ) ;
#6928=CARTESIAN_POINT ( 'NONE',  ( 5.000000000000000000, 8.660254037844385522, -17.12500000409675138 ) ) ;
#6929=CARTESIAN_POINT ( 'NONE',  ( 10.81189881249999729, 0.000000000000000000, -46.53125000204838813 ) ) ;
#6933=VECTOR ( 'NONE', #37079, 1000.000000000000000 ) ;
#6934=CARTESIAN_POINT ( 'NONE',  ( -5.405949406249996869, 9.363379034771805109, -143.5312500020483810 ) ) ;
#6935=AXIS2_PLACEMENT_3D ( 'NONE', #7672, #20824, #1418 ) ;
#6937=VERTEX_POINT ( 'NONE', #12454 ) ;
#6938=ORIENTED_EDGE ( 'NONE', *, *, #36139, .F. ) ;
#6941=( BOUNDED_CURVE ( )  B_SPLINE_CURVE ( 2, ( #22403, #19157, #32348, #2772, #16967, #16108, #6847 ),
 .UNSPECIFIED., .F., .F. ) 
 B_SPLINE_CURVE_WITH_KNOTS ( ( 3, 2, 2, 3 ),
 ( 0.3694029850746270438, 0.3706467661691543181, 0.3718905472636817033, 0.3731343283582090331 ),
 .UNSPECIFIED. ) 
 CURVE ( )  GEOMETRIC_REPRESENTATION_ITEM ( )  RATIONAL_B_SPLINE_CURVE ( ( 0.9999999999999820144, 0.8660254037844566932, 1.000000000000000000, 0.8660254037844387076, 1.000000000000000000, 0.8660254037844327124, 1.000000000000005995 ) ) 
 REPRESENTATION_ITEM ( '' )  );
#6943=CYLINDRICAL_SURFACE ( 'NONE', #26998, 9.999999999999998224 ) ;
#6944=CARTESIAN_POINT ( 'NONE',  ( -10.81189881249999907, -6.242252689847864744, -171.4687500020484094 ) ) ;
#6945=CARTESIAN_POINT ( 'NONE',  ( 5.405949406249992428, -9.363379034771808662, -24.09375000204835970 ) ) ;
#6948=CARTESIAN_POINT ( 'NONE',  ( 5.405949406249992428, -9.363379034771808662, -153.0937500020483810 ) ) ;
#6949=CARTESIAN_POINT ( 'NONE',  ( -10.81189881249999729, 1.324075727343319199E-15, -147.5937500020483810 ) ) ;
#6950=CARTESIAN_POINT ( 'NONE',  ( -10.00000000000154188, 5.773502691895366468, -67.37499999999995737 ) ) ;
#6953=CARTESIAN_POINT ( 'NONE',  ( -10.81189881249999729, 6.242252689847871849, -14.21875000204836681 ) ) ;
#6960=CARTESIAN_POINT ( 'NONE',  ( 10.81189881249999729, 0.000000000000000000, -85.34375000204836681 ) ) ;
#6961=CARTESIAN_POINT ( 'NONE',  ( 5.405949406249992428, -9.363379034771808662, -70.59375000204836681 ) ) ;
#6962=CARTESIAN_POINT ( 'NONE',  ( 10.81189881249999729, 0.000000000000000000, -45.03125000204838102 ) ) ;
#6964=CARTESIAN_POINT ( 'NONE',  ( 5.000000000000000000, 8.660254037844385522, -186.2500000000000000 ) ) ;
#6966=EDGE_CURVE ( 'NONE', #9954, #11855, #15894, .T. ) ;
#6967=CARTESIAN_POINT ( 'NONE',  ( -9.999999999999998224, 1.224646799147353059E-15, -125.7499999999999716 ) ) ;
#6968=CARTESIAN_POINT ( 'NONE',  ( -10.81189881249999729, 1.324075727343319199E-15, -140.2812500020483810 ) ) ;
#6969=DIRECTION ( 'NONE',  ( -0.000000000000000000, -0.000000000000000000, 1.000000000000000000 ) ) ;
#6971=EDGE_CURVE ( 'NONE', #42590, #21106, #2802, .T. ) ;
#6977=CARTESIAN_POINT ( 'NONE',  ( 5.405949406249992428, -9.363379034771808662, -165.2812500020484094 ) ) ;
#6978=CARTESIAN_POINT ( 'NONE',  ( -4.999999999999996447, 8.660254037844387298, -42.37500000409677625 ) ) ;
#6979=DIRECTION ( 'NONE',  ( -0.000000000000000000, -0.000000000000000000, 1.000000000000000000 ) ) ;
#6981=DIRECTION ( 'NONE',  ( 1.502314598737160017E-16, -1.000000000000000000, 0.000000000000000000 ) ) ;
#6982=CARTESIAN_POINT ( 'NONE',  ( 10.81189881249999729, 0.000000000000000000, -159.0312500020484094 ) ) ;
#6983=CARTESIAN_POINT ( 'NONE',  ( 7.644554776091147741E-16, 12.48450537969573659, -135.9687500020483810 ) ) ;
#6985=CARTESIAN_POINT ( 'NONE',  ( -2.121150477449813534E-15, -11.54700538379251284, -115.2500000040967905 ) ) ;
#6986=VERTEX_POINT ( 'NONE', #18139 ) ;
#6987=CARTESIAN_POINT ( 'NONE',  ( -9.999999999999998224, 1.224646799147353059E-15, -114.1250000040967763 ) ) ;
#6988=ADVANCED_FACE ( 'NONE', ( #41220 ), #17919, .T. ) ;
#6989=VECTOR ( 'NONE', #16029, 1000.000000000000000 ) ;
#6990=( BOUNDED_CURVE ( )  B_SPLINE_CURVE ( 2, ( #1436, #14349, #18029, #28412, #35522, #18892, #38319 ),
 .UNSPECIFIED., .F., .F. ) 
 B_SPLINE_CURVE_WITH_KNOTS ( ( 3, 2, 2, 3 ),
 ( 0.8507462686567166532, 0.8519900497512440385, 0.8532338308457714238, 0.8544776119402988090 ),
 .UNSPECIFIED. ) 
 CURVE ( )  GEOMETRIC_REPRESENTATION_ITEM ( )  RATIONAL_B_SPLINE_CURVE ( ( 0.9999999999999761302, 0.8660254037844625774, 1.000000000000000000, 0.8660254037844387076, 1.000000000000000000, 0.8660254037844028474, 1.000000000000035971 ) ) 
 REPRESENTATION_ITEM ( '' )  );
#6992=CARTESIAN_POINT ( 'NONE',  ( -10.81189881249999907, -6.242252689847864744, -66.65625000204839523 ) ) ;
#6993=EDGE_LOOP ( 'NONE', ( #4815, #24746, #1485, #8227 ) ) ;
#6995=CARTESIAN_POINT ( 'NONE',  ( 5.405949406249992428, -9.363379034771808662, -118.5937500020483810 ) ) ;
#6996=VERTEX_POINT ( 'NONE', #31335 ) ;
#6997=CARTESIAN_POINT ( 'NONE',  ( -5.405949406250003975, -9.363379034771801557, -22.84375000204835615 ) ) ;
#6999=CARTESIAN_POINT ( 'NONE',  ( -5.405949406249996869, 9.363379034771805109, 0.4687499979516285276 ) ) ;
#7001=CARTESIAN_POINT ( 'NONE',  ( 10.81189881249999729, 0.000000000000000000, -43.34375000204837391 ) ) ;
#7002=DIRECTION ( 'NONE',  ( -0.000000000000000000, -0.000000000000000000, 1.000000000000000000 ) ) ;
#7003=CYLINDRICAL_SURFACE ( 'NONE', #35584, 9.999999999999998224 ) ;
#7004=CARTESIAN_POINT ( 'NONE',  ( -2.293366432827344421E-15, -12.48450537969573659, -178.7187500020484094 ) ) ;
#7005=CARTESIAN_POINT ( 'NONE',  ( -5.405949406249996869, 9.363379034771805109, -165.8437500020484094 ) ) ;
#7009=CARTESIAN_POINT ( 'NONE',  ( -4.999999999999996447, 8.660254037844387298, -19.87500000409675494 ) ) ;
#7011=CARTESIAN_POINT ( 'NONE',  ( 10.81189881249999729, 0.000000000000000000, -98.84375000204838102 ) ) ;
#7013=CARTESIAN_POINT ( 'NONE',  ( -5.405949406250003975, -9.363379034771801557, -65.03125000204838102 ) ) ;
#7014=CARTESIAN_POINT ( 'NONE',  ( 10.00000000000102318, -5.773502691895667560, -5.124999999999934275 ) ) ;
#7016=CARTESIAN_POINT ( 'NONE',  ( 10.81189881249999729, 0.000000000000000000, -124.5312500020483952 ) ) ;
#7017=CARTESIAN_POINT ( 'NONE',  ( 7.644554776091147741E-16, 12.48450537969573659, -160.1562500020484094 ) ) ;
#7019=CARTESIAN_POINT ( 'NONE',  ( 4.999999999999992006, -8.660254037844389075, -134.6250000040967620 ) ) ;
#7022=ORIENTED_EDGE ( 'NONE', *, *, #2979, .F. ) ;
#7025=CARTESIAN_POINT ( 'NONE',  ( 10.81189881249999907, 6.242252689847868297, -185.9062500020484094 ) ) ;
#7026=LINE ( 'NONE', #6808, #24763 ) ;
#7028=VERTEX_POINT ( 'NONE', #5793 ) ;
#7029=CARTESIAN_POINT ( 'NONE',  ( -5.000000000000003553, -8.660254037844383745, -56.49999999999996447 ) ) ;
#7031=CARTESIAN_POINT ( 'NONE',  ( 10.00000000000000000, 5.773502691896255534, -66.75000000409677625 ) ) ;
#7032=CARTESIAN_POINT ( 'NONE',  ( 9.999999999999612754, 5.773502691896477579, -153.3749999999999716 ) ) ;
#7033=CARTESIAN_POINT ( 'NONE',  ( -9.999999999999804601, 5.773502691896371886, -178.7500000040967905 ) ) ;
#7035=CARTESIAN_POINT ( 'NONE',  ( -10.81189881249999729, 1.324075727343319199E-15, -57.78125000204836681 ) ) ;
#7039=CARTESIAN_POINT ( 'NONE',  ( -2.293366432827344421E-15, -12.48450537969573659, -186.4062500020484094 ) ) ;
#7041=EDGE_CURVE ( 'NONE', #40773, #2132, #28093, .T. ) ;
#7043=CARTESIAN_POINT ( 'NONE',  ( 10.81189881249999729, 0.000000000000000000, -1.343750002048366143 ) ) ;
#7044=CARTESIAN_POINT ( 'NONE',  ( 9.999999999999872102, 5.773502691896329253, -165.3750000000000000 ) ) ;
#7046=CARTESIAN_POINT ( 'NONE',  ( 9.999999999999998224, 0.000000000000000000, -200.0000000000000000 ) ) ;
#7047=FACE_OUTER_BOUND ( 'NONE', #8333, .T. ) ;
#7048=CARTESIAN_POINT ( 'NONE',  ( -5.405949406250003975, -9.363379034771801557, -90.53125000204838102 ) ) ;
#7049=ORIENTED_EDGE ( 'NONE', *, *, #1245, .F. ) ;
#7050=CARTESIAN_POINT ( 'NONE',  ( 9.999999999998456346, 5.773502691897149042, -24.75000000409673007 ) ) ;
#7051=CARTESIAN_POINT ( 'NONE',  ( -5.000000000000003553, -8.660254037844383745, -69.99999999999998579 ) ) ;
#7055=CARTESIAN_POINT ( 'NONE',  ( 10.81189881249999729, 0.000000000000000000, -32.84375000204836681 ) ) ;
#7056=CARTESIAN_POINT ( 'NONE',  ( -5.405949406249996869, 9.363379034771805109, -20.53125000204836326 ) ) ;
#7057=CARTESIAN_POINT ( 'NONE',  ( -2.293366432827344421E-15, -12.48450537969573659, -72.21875000204835260 ) ) ;
#7058=CARTESIAN_POINT ( 'NONE',  ( 9.999999999999998224, 0.000000000000000000, -83.37500000409677625 ) ) ;
#7060=CARTESIAN_POINT ( 'NONE',  ( 5.405949406249992428, -9.363379034771808662, -196.5937500020484094 ) ) ;
#7061=CARTESIAN_POINT ( 'NONE',  ( 10.81189881249999907, 6.242252689847868297, -149.7187500020483810 ) ) ;
#7065=CARTESIAN_POINT ( 'NONE',  ( -10.00000000000000000, -5.773502691896251982, -1.500000004096750938 ) ) ;
#7067=CARTESIAN_POINT ( 'NONE',  ( -5.000000000000003553, -8.660254037844383745, -80.49999999999998579 ) ) ;
#7068=CARTESIAN_POINT ( 'NONE',  ( 10.81189881249999551, -6.242252689847874514, -119.9687500020483952 ) ) ;
#7069=CARTESIAN_POINT ( 'NONE',  ( -9.999999999999998224, 1.224646799147353059E-15, -14.74999999999995737 ) ) ;
#7070=CARTESIAN_POINT ( 'NONE',  ( -2.293366432827344421E-15, -12.48450537969573659, -90.40625000204838102 ) ) ;
#7071=CARTESIAN_POINT ( 'NONE',  ( -5.405949406249996869, 9.363379034771805109, -107.3437500020483810 ) ) ;
#7074=CARTESIAN_POINT ( 'NONE',  ( 9.999999999999996447, -5.773502691896262640, -158.5000000040968189 ) ) ;
#7077=DIRECTION ( 'NONE',  ( -0.000000000000000000, -0.000000000000000000, 1.000000000000000000 ) ) ;
#7078=CARTESIAN_POINT ( 'NONE',  ( 0.000000000000000000, 0.000000000000000000, -200.0000000000000000 ) ) ;
#7079=CARTESIAN_POINT ( 'NONE',  ( -9.999999999998969713, -5.773502691896847949, -54.00000000409674072 ) ) ;
#7081=CARTESIAN_POINT ( 'NONE',  ( -10.00000000000000000, -5.773502691896251982, -83.62499999999998579 ) ) ;
#7083=CARTESIAN_POINT ( 'NONE',  ( 5.000000000000000000, 8.660254037844385522, -86.12500000409677625 ) ) ;
#7084=FACE_OUTER_BOUND ( 'NONE', #17858, .T. ) ;
#7086=CARTESIAN_POINT ( 'NONE',  ( -5.405949406250003975, -9.363379034771801557, -87.53125000204838102 ) ) ;
#7087=VERTEX_POINT ( 'NONE', #14895 ) ;
#7089=CARTESIAN_POINT ( 'NONE',  ( 9.999999999999998224, 0.000000000000000000, -188.0000000000000000 ) ) ;
#7091=ORIENTED_EDGE ( 'NONE', *, *, #28102, .T. ) ;
#7092=CARTESIAN_POINT ( 'NONE',  ( -9.999999999999998224, 5.773502691896259087, -13.37499999999996803 ) ) ;
#7094=CARTESIAN_POINT ( 'NONE',  ( -5.000000000000003553, -8.660254037844383745, -146.5000000000000000 ) ) ;
#7096=CARTESIAN_POINT ( 'NONE',  ( 4.999999999999992006, -8.660254037844389075, -188.2500000000000000 ) ) ;
#7098=CARTESIAN_POINT ( 'NONE',  ( 10.81189881249999907, 6.242252689847868297, -121.4062500020483810 ) ) ;
#7100=CARTESIAN_POINT ( 'NONE',  ( 9.999999999998456346, 5.773502691897149042, -13.87499999999993072 ) ) ;
#7101=ORIENTED_EDGE ( 'NONE', *, *, #2237, .F. ) ;
#7102=CARTESIAN_POINT ( 'NONE',  ( 10.81189881249999551, -6.242252689847874514, -43.65625000204838102 ) ) ;
#7104=CARTESIAN_POINT ( 'NONE',  ( -2.293366432827344421E-15, -12.48450537969573659, -96.21875000204839523 ) ) ;
#7105=CARTESIAN_POINT ( 'NONE',  ( -5.405949406250003975, -9.363379034771801557, -120.5312500020483952 ) ) ;
#7106=ORIENTED_EDGE ( 'NONE', *, *, #38786, .F. ) ;
#7108=CARTESIAN_POINT ( 'NONE',  ( 9.999999999998969713, 5.773502691896851502, -33.37499999999994316 ) ) ;
#7112=CARTESIAN_POINT ( 'NONE',  ( 10.81189881249999729, 6.242252689847867408, -134.7187500020483810 ) ) ;
#7114=CARTESIAN_POINT ( 'NONE',  ( 0.000000000000000000, 0.000000000000000000, -200.0000000000000000 ) ) ;
#7116=CARTESIAN_POINT ( 'NONE',  ( 9.999999999999998224, 0.000000000000000000, -185.3750000040967905 ) ) ;
#7118=CARTESIAN_POINT ( 'NONE',  ( 5.405949406249992428, -9.363379034771808662, -178.7812500020484094 ) ) ;
#7122=CARTESIAN_POINT ( 'NONE',  ( 7.644554776091147741E-16, 12.48450537969573659, -60.96875000204838102 ) ) ;
#7123=CARTESIAN_POINT ( 'NONE',  ( -2.293366432827344421E-15, -12.48450537969573659, -42.21875000204835970 ) ) ;
#7125=CARTESIAN_POINT ( 'NONE',  ( 5.405949406249999534, 9.363379034771803333, -20.78125000204836326 ) ) ;
#7129=CARTESIAN_POINT ( 'NONE',  ( 10.00000000000000000, 5.773502691896255534, -108.3749999999999858 ) ) ;
#7131=CARTESIAN_POINT ( 'NONE',  ( -9.999999999999998224, 1.224646799147353059E-15, -49.62500000409675494 ) ) ;
#7134=CARTESIAN_POINT ( 'NONE',  ( -2.293366432827344421E-15, -12.48450537969573659, -109.9062500020483810 ) ) ;
#7135=ORIENTED_EDGE ( 'NONE', *, *, #30471, .T. ) ;
#7141=CARTESIAN_POINT ( 'NONE',  ( 9.999999999999998224, 0.000000000000000000, -31.99999999999997158 ) ) ;
#7142=CARTESIAN_POINT ( 'NONE',  ( -2.293366432827344421E-15, -12.48450537969573659, -33.40625000204835970 ) ) ;
#7143=CARTESIAN_POINT ( 'NONE',  ( 9.999999999999227285, 5.773502691896701400, -111.7500000040967478 ) ) ;
#7145=CARTESIAN_POINT ( 'NONE',  ( -4.999999999999996447, 8.660254037844387298, -133.5000000000000000 ) ) ;
#7146=CARTESIAN_POINT ( 'NONE',  ( 10.81189881249999551, -6.242252689847874514, -142.6562500020484094 ) ) ;
#7147=CARTESIAN_POINT ( 'NONE',  ( 9.999999999999998224, 0.000000000000000000, -200.0000000000000000 ) ) ;
#7149=EDGE_CURVE ( 'NONE', #21158, #20251, #7194, .T. ) ;
#7150=ORIENTED_EDGE ( 'NONE', *, *, #10841, .T. ) ;
#7151=CARTESIAN_POINT ( 'NONE',  ( 0.000000000000000000, 0.000000000000000000, -200.0000000000000000 ) ) ;
#7154=CARTESIAN_POINT ( 'NONE',  ( -10.81189881249999729, 6.242252689847871849, -162.7187500020483810 ) ) ;
#7156=CARTESIAN_POINT ( 'NONE',  ( 10.81189881249999551, -6.242252689847874514, -19.46875000204837391 ) ) ;
#7157=CARTESIAN_POINT ( 'NONE',  ( -9.999999999999998224, 1.224646799147353059E-15, -110.7499999999999858 ) ) ;
#7158=CARTESIAN_POINT ( 'NONE',  ( 5.405949406249992428, -9.363379034771808662, -159.0937500020484094 ) ) ;
#7159=CARTESIAN_POINT ( 'NONE',  ( -5.405949406250003975, -9.363379034771801557, -139.8437500020484094 ) ) ;
#7164=CARTESIAN_POINT ( 'NONE',  ( -10.81189881249999729, 6.242252689847871849, -12.71875000204837747 ) ) ;
#7166=CARTESIAN_POINT ( 'NONE',  ( 9.999999999998969713, 5.773502691896851502, -63.75000000409677625 ) ) ;
#7167=CARTESIAN_POINT ( 'NONE',  ( 7.070501591499376803E-16, 11.54700538379251284, -125.0000000040967763 ) ) ;
#7170=CARTESIAN_POINT ( 'NONE',  ( -10.81189881249999729, -6.242252689847864744, -82.96875000204836681 ) ) ;
#7171=CARTESIAN_POINT ( 'NONE',  ( -10.81189881249999729, 6.242252689847871849, -62.21875000204838813 ) ) ;
#7172=CARTESIAN_POINT ( 'NONE',  ( 10.81189881249999551, -6.242252689847874514, -40.65625000204835970 ) ) ;
#7174=CARTESIAN_POINT ( 'NONE',  ( 7.070501591499376803E-16, 11.54700538379251284, -186.1250000000000000 ) ) ;
#7176=CARTESIAN_POINT ( 'NONE',  ( 7.070501591499377789E-16, 11.54700538379251284, -126.1249999999999858 ) ) ;
#7177=CARTESIAN_POINT ( 'NONE',  ( 7.644554776091147741E-16, 12.48450537969573659, -139.1562500020484094 ) ) ;
#7178=CARTESIAN_POINT ( 'NONE',  ( 4.999999999999992006, -8.660254037844389075, -150.7500000000000000 ) ) ;
#7180=CARTESIAN_POINT ( 'NONE',  ( 5.405949406249992428, -9.363379034771808662, -21.28125000204836326 ) ) ;
#7184=CARTESIAN_POINT ( 'NONE',  ( 5.000000000000000000, 8.660254037844385522, -39.24999999999997868 ) ) ;
#7185=CARTESIAN_POINT ( 'NONE',  ( -4.999999999999996447, 8.660254037844387298, -45.37500000409677625 ) ) ;
#7188=CARTESIAN_POINT ( 'NONE',  ( -9.999999999999998224, 1.224646799147353059E-15, -146.7500000000000000 ) ) ;
#7189=CARTESIAN_POINT ( 'NONE',  ( -10.81189881249999729, 6.242252689847871849, -150.9062500020484094 ) ) ;
#7190=CARTESIAN_POINT ( 'NONE',  ( -2.293366432827344421E-15, -12.48450537969573659, -136.7187500020483810 ) ) ;
#7191=FACE_OUTER_BOUND ( 'NONE', #8752, .T. ) ;
#7192=CARTESIAN_POINT ( 'NONE',  ( -4.999999999999996447, 8.660254037844387298, -151.5000000000000000 ) ) ;
#7193=ORIENTED_EDGE ( 'NONE', *, *, #32563, .T. ) ;
#7194=( BOUNDED_CURVE ( )  B_SPLINE_CURVE ( 2, ( #2562, #9448, #15692, #22614, #12661, #34352, #9231 ),
 .UNSPECIFIED., .F., .F. ) 
 B_SPLINE_CURVE_WITH_KNOTS ( ( 3, 2, 2, 3 ),
 ( 0.7462686567164180662, 0.7475124378109453405, 0.7487562189054727257, 0.7500000000000001110 ),
 .UNSPECIFIED. ) 
 CURVE ( )  GEOMETRIC_REPRESENTATION_ITEM ( )  RATIONAL_B_SPLINE_CURVE ( ( 0.9999999999999880096, 0.8660254037844506980, 1.000000000000000000, 0.8660254037844387076, 1.000000000000000000, 0.8660254037844267172, 1.000000000000011990 ) ) 
 REPRESENTATION_ITEM ( '' )  );
#7195=CARTESIAN_POINT ( 'NONE',  ( 7.644554776091147741E-16, 12.48450537969573659, -61.15625000204838102 ) ) ;
#7196=VERTEX_POINT ( 'NONE', #6220 ) ;
#7198=EDGE_CURVE ( 'NONE', #21756, #36343, #42024, .T. ) ;
#7199=EDGE_CURVE ( 'NONE', #39779, #27592, #38804, .T. ) ;
#7200=CARTESIAN_POINT ( 'NONE',  ( 7.644554776091147741E-16, 12.48450537969573659, -122.4687500020483952 ) ) ;
#7202=EDGE_CURVE ( 'NONE', #14562, #22008, #32345, .T. ) ;
#7203=CARTESIAN_POINT ( 'NONE',  ( 10.81189881249999729, 0.000000000000000000, -20.84375000204835615 ) ) ;
#7204=CARTESIAN_POINT ( 'NONE',  ( 10.81189881249999729, 0.000000000000000000, -199.3437500020484094 ) ) ;
#7205=CARTESIAN_POINT ( 'NONE',  ( 10.81189881249999907, 6.242252689847868297, -49.21875000204835260 ) ) ;
#7206=CARTESIAN_POINT ( 'NONE',  ( 9.999999999999998224, 0.000000000000000000, -155.3750000040967905 ) ) ;
#7207=CARTESIAN_POINT ( 'NONE',  ( 9.999999999999998224, 0.000000000000000000, -9.875000004096746054 ) ) ;
#7208=CARTESIAN_POINT ( 'NONE',  ( 5.405949406249992428, -9.363379034771808662, -183.0937500020483810 ) ) ;
#7209=CARTESIAN_POINT ( 'NONE',  ( 10.81189881249999729, 0.000000000000000000, -164.8437500020484094 ) ) ;
#7214=CARTESIAN_POINT ( 'NONE',  ( 9.999999999999479527, 5.773502691896553074, -36.37499999999995026 ) ) ;
#7216=CARTESIAN_POINT ( 'NONE',  ( -10.81189881249999729, 1.324075727343319199E-15, -101.0937500020483810 ) ) ;
#7217=CARTESIAN_POINT ( 'NONE',  ( 7.070501591499376803E-16, 11.54700538379251284, -34.62499999999995737 ) ) ;
#7218=CARTESIAN_POINT ( 'NONE',  ( -5.405949406249996869, 9.363379034771805109, -68.53125000204838102 ) ) ;
#7219=CARTESIAN_POINT ( 'NONE',  ( -10.00000000000051337, 5.773502691895962435, -145.7500000040967905 ) ) ;
#7221=EDGE_CURVE ( 'NONE', #36222, #31836, #33177, .T. ) ;
#7222=CARTESIAN_POINT ( 'NONE',  ( 10.81189881249999907, 6.242252689847868297, -124.4062500020483810 ) ) ;
#7223=CARTESIAN_POINT ( 'NONE',  ( -10.81189881249999729, 1.324075727343319199E-15, -164.2812500020484094 ) ) ;
#7225=CARTESIAN_POINT ( 'NONE',  ( -10.00000000000000000, -5.773502691896251982, -138.0000000040967905 ) ) ;
#7227=VERTEX_POINT ( 'NONE', #19997 ) ;
#7231=CARTESIAN_POINT ( 'NONE',  ( -10.81189881249999729, 1.324075727343319199E-15, -186.7812500020484094 ) ) ;
#7233=ORIENTED_EDGE ( 'NONE', *, *, #23947, .T. ) ;
#7234=CARTESIAN_POINT ( 'NONE',  ( 4.999999999999992006, -8.660254037844389075, -45.74999999999998579 ) ) ;
#7236=CARTESIAN_POINT ( 'NONE',  ( -10.00000000000000000, -5.773502691896251982, -64.50000000409677625 ) ) ;
#7237=CARTESIAN_POINT ( 'NONE',  ( -2.121150477449813534E-15, -11.54700538379251284, -109.2500000040967763 ) ) ;
#7240=CARTESIAN_POINT ( 'NONE',  ( -5.405949406249996869, 9.363379034771805109, -59.53125000204836681 ) ) ;
#7241=( BOUNDED_CURVE ( )  B_SPLINE_CURVE ( 2, ( #22886, #39692, #36045, #3243, #16587, #28945, #13137 ),
 .UNSPECIFIED., .F., .F. ) 
 B_SPLINE_CURVE_WITH_KNOTS ( ( 3, 2, 2, 3 ),
 ( 0.2052238805970149627, 0.2064676616915423202, 0.2077114427860697055, 0.2089552238805970630 ),
 .UNSPECIFIED. ) 
 CURVE ( )  GEOMETRIC_REPRESENTATION_ITEM ( )  RATIONAL_B_SPLINE_CURVE ( ( 0.9999999999999970024, 0.8660254037844417052, 1.000000000000000000, 0.8660254037844387076, 1.000000000000000000, 0.8660254037844327124, 1.000000000000005995 ) ) 
 REPRESENTATION_ITEM ( '' )  );
#7244=DIRECTION ( 'NONE',  ( -0.000000000000000000, -0.000000000000000000, 1.000000000000000000 ) ) ;
#7245=CARTESIAN_POINT ( 'NONE',  ( -10.81189881249999729, 6.242252689847871849, -182.4062500020483810 ) ) ;
#7247=CARTESIAN_POINT ( 'NONE',  ( -10.00000000000051337, 5.773502691895962435, -79.37499999999998579 ) ) ;
#7248=CARTESIAN_POINT ( 'NONE',  ( 5.000000000000000000, 8.660254037844385522, -165.2500000000000000 ) ) ;
#7251=CARTESIAN_POINT ( 'NONE',  ( -8.223921726897051698, 5.755749732088058401, -0.000000000000000000 ) ) ;
#7252=AXIS2_PLACEMENT_3D ( 'NONE', #40013, #10865, #33558 ) ;
#7253=( BOUNDED_CURVE ( )  B_SPLINE_CURVE ( 2, ( #24411, #37340, #4969, #27418, #34329, #40554, #41191 ),
 .UNSPECIFIED., .F., .F. ) 
 B_SPLINE_CURVE_WITH_KNOTS ( ( 3, 2, 2, 3 ),
 ( 0.2835820895522389029, 0.2848258706467662882, 0.2860696517412936180, 0.2873134328358210032 ),
 .UNSPECIFIED. ) 
 CURVE ( )  GEOMETRIC_REPRESENTATION_ITEM ( )  RATIONAL_B_SPLINE_CURVE ( ( 0.9999999999999880096, 0.8660254037844506980, 1.000000000000000000, 0.8660254037844387076, 1.000000000000000000, 0.8660254037844267172, 1.000000000000011990 ) ) 
 REPRESENTATION_ITEM ( '' )  );
#7255=CARTESIAN_POINT ( 'NONE',  ( -10.81189881249999729, 6.242252689847871849, -84.90625000204838102 ) ) ;
#7257=DIRECTION ( 'NONE',  ( -0.000000000000000000, -0.000000000000000000, 1.000000000000000000 ) ) ;
#7259=ORIENTED_EDGE ( 'NONE', *, *, #11980, .F. ) ;
#7260=ORIENTED_EDGE ( 'NONE', *, *, #38889, .F. ) ;
#7261=CARTESIAN_POINT ( 'NONE',  ( -10.81189881249999907, -6.242252689847864744, -28.96875000204835615 ) ) ;
#7262=CARTESIAN_POINT ( 'NONE',  ( -5.405949406250003975, -9.363379034771801557, -23.03125000204836326 ) ) ;
#7264=CARTESIAN_POINT ( 'NONE',  ( 5.405949406249992428, -9.363379034771808662, -72.09375000204836681 ) ) ;
#7265=CARTESIAN_POINT ( 'NONE',  ( -2.121150477449813534E-15, -11.54700538379251284, -83.75000000409677625 ) ) ;
#7267=CARTESIAN_POINT ( 'NONE',  ( -10.81189881249999729, 6.242252689847871849, -186.7187500020483810 ) ) ;
#7268=CARTESIAN_POINT ( 'NONE',  ( 7.644554776091147741E-16, 12.48450537969573659, -152.4687500020483810 ) ) ;
#7270=FACE_OUTER_BOUND ( 'NONE', #18079, .T. ) ;
#7272=CARTESIAN_POINT ( 'NONE',  ( 10.00000000000000000, 5.773502691896255534, -3.750000004096762041 ) ) ;
#7273=CARTESIAN_POINT ( 'NONE',  ( 0.000000000000000000, 0.000000000000000000, -200.0000000000000000 ) ) ;
#7275=CARTESIAN_POINT ( 'NONE',  ( 10.81189881249999729, 0.000000000000000000, -124.3437500020483952 ) ) ;
#7276=CARTESIAN_POINT ( 'NONE',  ( -9.999999999999998224, 1.224646799147353059E-15, -200.0000000000000000 ) ) ;
#7277=CARTESIAN_POINT ( 'NONE',  ( 5.405949406249992428, -9.363379034771808662, -91.78125000204838102 ) ) ;
#7278=CARTESIAN_POINT ( 'NONE',  ( 10.81189881249999729, 6.242252689847867408, -98.71875000204838102 ) ) ;
#7282=CARTESIAN_POINT ( 'NONE',  ( -5.000000000000003553, -8.660254037844383745, -160.3750000040967905 ) ) ;
#7285=DIRECTION ( 'NONE',  ( -0.000000000000000000, -0.000000000000000000, 1.000000000000000000 ) ) ;
#7287=DIRECTION ( 'NONE',  ( -0.000000000000000000, -0.000000000000000000, 1.000000000000000000 ) ) ;
#7289=CARTESIAN_POINT ( 'NONE',  ( 9.999999999998456346, 5.773502691897149042, -63.37499999999994316 ) ) ;
#7290=CARTESIAN_POINT ( 'NONE',  ( -4.999999999999996447, 8.660254037844387298, -77.99999999999998579 ) ) ;
#7292=CARTESIAN_POINT ( 'NONE',  ( 5.000000000000000000, 8.660254037844385522, -93.62500000409677625 ) ) ;
#7293=AXIS2_PLACEMENT_3D ( 'NONE', #32013, #2018, #5244 ) ;
#7296=CARTESIAN_POINT ( 'NONE',  ( -5.405949406250003975, -9.363379034771801557, -80.03125000204838102 ) ) ;
#7300=ORIENTED_EDGE ( 'NONE', *, *, #109, .F. ) ;
#7301=CARTESIAN_POINT ( 'NONE',  ( -5.000000000000003553, -8.660254037844383745, -8.499999999999952038 ) ) ;
#7303=CARTESIAN_POINT ( 'NONE',  ( 4.999999999999992006, -8.660254037844389075, -146.2500000000000000 ) ) ;
#7304=CARTESIAN_POINT ( 'NONE',  ( -4.999999999999996447, 8.660254037844387298, -45.37500000409677625 ) ) ;
#7306=CARTESIAN_POINT ( 'NONE',  ( 5.405949406249999534, 9.363379034771803333, -139.2812500020483810 ) ) ;
#7307=CARTESIAN_POINT ( 'NONE',  ( 7.070501591499377789E-16, 11.54700538379251284, -192.1250000000000000 ) ) ;
#7308=CARTESIAN_POINT ( 'NONE',  ( 10.81189881249999907, 6.242252689847868297, -118.4062500020484094 ) ) ;
#7309=VERTEX_POINT ( 'NONE', #29516 ) ;
#7310=CARTESIAN_POINT ( 'NONE',  ( 7.070501591499376803E-16, 11.54700538379251284, -23.00000000409677270 ) ) ;
#7314=CARTESIAN_POINT ( 'NONE',  ( -10.81189881249999907, -6.242252689847864744, -42.65625000204837391 ) ) ;
#7316=CARTESIAN_POINT ( 'NONE',  ( 5.405949406249999534, 9.363379034771803333, -92.59375000204838102 ) ) ;
#7317=CARTESIAN_POINT ( 'NONE',  ( -10.81189881249999729, 1.324075727343319199E-15, -126.7812500020483668 ) ) ;
#7318=ORIENTED_EDGE ( 'NONE', *, *, #18835, .T. ) ;
#7320=( BOUNDED_CURVE ( )  B_SPLINE_CURVE ( 2, ( #35060, #5917, #31612, #35276, #5488, #18638, #2268 ),
 .UNSPECIFIED., .F., .F. ) 
 B_SPLINE_CURVE_WITH_KNOTS ( ( 3, 2, 2, 3 ),
 ( 0.2761194029850747578, 0.2773631840796020875, 0.2786069651741294728, 0.2798507462686568026 ),
 .UNSPECIFIED. ) 
 CURVE ( )  GEOMETRIC_REPRESENTATION_ITEM ( )  RATIONAL_B_SPLINE_CURVE ( ( 0.9999999999999880096, 0.8660254037844506980, 1.000000000000000000, 0.8660254037844387076, 1.000000000000000000, 0.8660254037844267172, 1.000000000000011990 ) ) 
 REPRESENTATION_ITEM ( '' )  );
#7322=CARTESIAN_POINT ( 'NONE',  ( -10.81189881249999729, -6.242252689847864744, -195.4687500020484094 ) ) ;
#7324=CARTESIAN_POINT ( 'NONE',  ( -9.999999999999998224, 1.224646799147353059E-15, -200.0000000000000000 ) ) ;
#7326=CARTESIAN_POINT ( 'NONE',  ( -5.405949406250003975, -9.363379034771801557, -120.3437500020483952 ) ) ;
#7331=CARTESIAN_POINT ( 'NONE',  ( 5.000000000000000000, 8.660254037844385522, -186.6250000040967905 ) ) ;
#7333=CARTESIAN_POINT ( 'NONE',  ( 10.81189881249999551, -6.242252689847874514, -180.1562500020484094 ) ) ;
#7334=CARTESIAN_POINT ( 'NONE',  ( -9.999999999999998224, 1.224646799147353059E-15, -107.7499999999999858 ) ) ;
#7335=CARTESIAN_POINT ( 'NONE',  ( 5.000000000000000000, 8.660254037844385522, -181.7500000000000000 ) ) ;
#7337=CARTESIAN_POINT ( 'NONE',  ( -10.81189881249999729, 1.324075727343319199E-15, -57.59375000204835970 ) ) ;
#7338=CARTESIAN_POINT ( 'NONE',  ( -5.405949406250003975, -9.363379034771801557, -39.34375000204837391 ) ) ;
#7340=CARTESIAN_POINT ( 'NONE',  ( -10.81189881249999729, 1.324075727343319199E-15, -9.781250002048352599 ) ) ;
#7342=CARTESIAN_POINT ( 'NONE',  ( 10.00000000000051159, -5.773502691895965988, -92.50000000409676204 ) ) ;
#7344=CARTESIAN_POINT ( 'NONE',  ( -2.121150477449813534E-15, -11.54700538379251284, -104.3749999999999716 ) ) ;
#7347=VECTOR ( 'NONE', #40907, 1000.000000000000000 ) ;
#7350=CARTESIAN_POINT ( 'NONE',  ( 10.81189881249999551, -6.242252689847874514, -106.6562500020484094 ) ) ;
#7352=EDGE_LOOP ( 'NONE', ( #40205, #9413, #39807, #9855 ) ) ;
#7355=CYLINDRICAL_SURFACE ( 'NONE', #36702, 9.999999999999998224 ) ;
#7357=EDGE_LOOP ( 'NONE', ( #40500, #8968, #18834, #24615 ) ) ;
#7358=CARTESIAN_POINT ( 'NONE',  ( -5.000000000000003553, -8.660254037844383745, -35.49999999999997868 ) ) ;
#7359=CARTESIAN_POINT ( 'NONE',  ( 10.81189881249999729, 6.242252689847867408, -37.40625000204836681 ) ) ;
#7362=CARTESIAN_POINT ( 'NONE',  ( 10.81189881249999729, 0.000000000000000000, -142.5312500020483810 ) ) ;
#7363=CARTESIAN_POINT ( 'NONE',  ( -9.999999999999998224, 1.224646799147353059E-15, -162.1250000040967905 ) ) ;
#7365=( BOUNDED_CURVE ( )  B_SPLINE_CURVE ( 2, ( #3536, #736, #3751, #29656, #42585, #30088, #16672 ),
 .UNSPECIFIED., .F., .F. ) 
 B_SPLINE_CURVE_WITH_KNOTS ( ( 3, 2, 2, 3 ),
 ( 0.2462686567164180107, 0.2475124378109453960, 0.2487562189054727535, 0.2500000000000001110 ),
 .UNSPECIFIED. ) 
 CURVE ( )  GEOMETRIC_REPRESENTATION_ITEM ( )  RATIONAL_B_SPLINE_CURVE ( ( 0.9999999999999880096, 0.8660254037844506980, 1.000000000000000000, 0.8660254037844387076, 1.000000000000000000, 0.8660254037844267172, 1.000000000000011990 ) ) 
 REPRESENTATION_ITEM ( '' )  );
#7366=ADVANCED_FACE ( 'NONE', ( #600 ), #19571, .T. ) ;
#7367=ORIENTED_EDGE ( 'NONE', *, *, #39117, .F. ) ;
#7369=DIRECTION ( 'NONE',  ( -0.000000000000000000, -0.000000000000000000, 1.000000000000000000 ) ) ;
#7370=CARTESIAN_POINT ( 'NONE',  ( 5.405949406249999534, 9.363379034771803333, -166.0937500020484094 ) ) ;
#7371=EDGE_CURVE ( 'NONE', #848, #6885, #17177, .T. ) ;
#7373=CARTESIAN_POINT ( 'NONE',  ( 10.81189881249999907, 6.242252689847868297, -14.71875000204837036 ) ) ;
#7374=FACE_OUTER_BOUND ( 'NONE', #28827, .T. ) ;
#7375=CARTESIAN_POINT ( 'NONE',  ( 10.81189881249999551, -6.242252689847874514, -154.4687500020484094 ) ) ;
#7376=CARTESIAN_POINT ( 'NONE',  ( -10.81189881249999729, 1.324075727343319199E-15, -135.5937500020483810 ) ) ;
#7377=CARTESIAN_POINT ( 'NONE',  ( -5.405949406249996869, 9.363379034771805109, -103.0312500020483952 ) ) ;
#7381=CARTESIAN_POINT ( 'NONE',  ( -10.81189881249999907, -6.242252689847864744, -10.96875000204836859 ) ) ;
#7383=DIRECTION ( 'NONE',  ( -0.000000000000000000, -0.000000000000000000, 1.000000000000000000 ) ) ;
#7387=CARTESIAN_POINT ( 'NONE',  ( 5.405949406249999534, 9.363379034771803333, -82.09375000204836681 ) ) ;
#7388=CARTESIAN_POINT ( 'NONE',  ( -10.81189881249999729, 1.324075727343319199E-15, -66.59375000204836681 ) ) ;
#7389=DIRECTION ( 'NONE',  ( -0.000000000000000000, -0.000000000000000000, 1.000000000000000000 ) ) ;
#7390=CARTESIAN_POINT ( 'NONE',  ( -10.81189881249999907, -6.242252689847864744, -45.65625000204837391 ) ) ;
#7394=CARTESIAN_POINT ( 'NONE',  ( -9.999999999999998224, 5.773502691896259087, -130.3750000000000000 ) ) ;
#7395=CARTESIAN_POINT ( 'NONE',  ( 10.81189881249999729, 6.242252689847867408, -133.4062500020483810 ) ) ;
#7396=CARTESIAN_POINT ( 'NONE',  ( -9.999999999999998224, 1.224646799147353059E-15, -94.24999999999998579 ) ) ;
#7398=CARTESIAN_POINT ( 'NONE',  ( 5.405949406249999534, 9.363379034771803333, -20.78125000204836326 ) ) ;
#7399=ORIENTED_EDGE ( 'NONE', *, *, #35671, .F. ) ;
#7402=DIRECTION ( 'NONE',  ( -0.000000000000000000, -0.000000000000000000, 1.000000000000000000 ) ) ;
#7403=CARTESIAN_POINT ( 'NONE',  ( 7.070501591499377789E-16, 11.54700538379251284, -33.50000000409675494 ) ) ;
#7405=LINE ( 'NONE', #30719, #2865 ) ;
#7407=CARTESIAN_POINT ( 'NONE',  ( 7.070501591499376803E-16, 11.54700538379251284, -76.62500000000000000 ) ) ;
#7408=CARTESIAN_POINT ( 'NONE',  ( -10.81189881249999907, -6.242252689847864744, -155.1562500020484094 ) ) ;
#7409=CARTESIAN_POINT ( 'NONE',  ( 5.405949406249999534, 9.363379034771803333, -136.0937500020483810 ) ) ;
#7411=ORIENTED_EDGE ( 'NONE', *, *, #15911, .T. ) ;
#7412=ORIENTED_EDGE ( 'NONE', *, *, #29392, .F. ) ;
#7414=CARTESIAN_POINT ( 'NONE',  ( 10.81189881249999907, 6.242252689847868297, -113.7187500020483810 ) ) ;
#7416=CARTESIAN_POINT ( 'NONE',  ( -9.999999999999998224, 1.224646799147353059E-15, -129.1250000040967620 ) ) ;
#7417=CARTESIAN_POINT ( 'NONE',  ( 10.81189881249999551, -6.242252689847874514, -188.9687500020484094 ) ) ;
#7418=CARTESIAN_POINT ( 'NONE',  ( 5.405949406249992428, -9.363379034771808662, -36.09375000204836681 ) ) ;
#7419=CARTESIAN_POINT ( 'NONE',  ( 4.947751128964601897, -9.422943186768698354, 6.544024882825221806E-15 ) ) ;
#7420=CARTESIAN_POINT ( 'NONE',  ( -5.000020801129981152, 8.660290040615111096, 0.000000000000000000 ) ) ;
#7421=CARTESIAN_POINT ( 'NONE',  ( 10.81189881249999729, 0.000000000000000000, -178.3437500020483810 ) ) ;
#7422=CARTESIAN_POINT ( 'NONE',  ( -5.405949406249996869, 9.363379034771805109, -159.8437500020484094 ) ) ;
#7425=CARTESIAN_POINT ( 'NONE',  ( 9.999999999999479527, 5.773502691896553074, -126.7500000040967478 ) ) ;
#7426=CARTESIAN_POINT ( 'NONE',  ( -9.999999999999998224, 1.224646799147353059E-15, -41.74999999999997868 ) ) ;
#7428=CARTESIAN_POINT ( 'NONE',  ( 10.81189881249999907, 6.242252689847868297, -92.71875000204836681 ) ) ;
#7429=CARTESIAN_POINT ( 'NONE',  ( 9.999999999999998224, 0.000000000000000000, -34.99999999999997868 ) ) ;
#7430=CARTESIAN_POINT ( 'NONE',  ( 5.405949406249999534, 9.363379034771803333, -64.28125000204836681 ) ) ;
#7433=CARTESIAN_POINT ( 'NONE',  ( -2.293366432827344421E-15, -12.48450537969573659, -121.9062500020483952 ) ) ;
#7434=CARTESIAN_POINT ( 'NONE',  ( -2.293366432827344421E-15, -12.48450537969573659, -153.4062500020483810 ) ) ;
#7436=CARTESIAN_POINT ( 'NONE',  ( -2.121150477449813534E-15, -11.54700538379251284, -127.2500000040967905 ) ) ;
#7438=VERTEX_POINT ( 'NONE', #3619 ) ;
#7442=CARTESIAN_POINT ( 'NONE',  ( 10.81189881249999907, 6.242252689847868297, -190.4062500020484094 ) ) ;
#7444=VECTOR ( 'NONE', #7916, 1000.000000000000000 ) ;
#7445=ORIENTED_EDGE ( 'NONE', *, *, #1691, .T. ) ;
#7446=CARTESIAN_POINT ( 'NONE',  ( -2.121150477449813534E-15, -11.54700538379251284, -50.37499999999997868 ) ) ;
#7448=CARTESIAN_POINT ( 'NONE',  ( -9.999999999999998224, 1.224646799147353059E-15, -69.12500000409677625 ) ) ;
#7449=EDGE_CURVE ( 'NONE', #9909, #11999, #36184, .T. ) ;
#7451=CARTESIAN_POINT ( 'NONE',  ( -5.000000000000003553, -8.660254037844383745, -109.3750000040967763 ) ) ;
#7452=( BOUNDED_CURVE ( )  B_SPLINE_CURVE ( 2, ( #17740, #40614, #4171, #4600, #24253, #30934, #27908 ),
 .UNSPECIFIED., .F., .F. ) 
 B_SPLINE_CURVE_WITH_KNOTS ( ( 3, 2, 2, 3 ),
 ( 0.8805970149253734558, 0.8818407960199008411, 0.8830845771144281153, 0.8843283582089555006 ),
 .UNSPECIFIED. ) 
 CURVE ( )  GEOMETRIC_REPRESENTATION_ITEM ( )  RATIONAL_B_SPLINE_CURVE ( ( 0.9999999999999641398, 0.8660254037844745678, 1.000000000000000000, 0.8660254037844387076, 1.000000000000000000, 0.8660254037844148378, 1.000000000000023981 ) ) 
 REPRESENTATION_ITEM ( '' )  );
#7453=DIRECTION ( 'NONE',  ( -0.000000000000000000, -0.000000000000000000, -1.000000000000000000 ) ) ;
#7456=CARTESIAN_POINT ( 'NONE',  ( -10.81189881249999729, 1.324075727343319199E-15, -56.28125000204836681 ) ) ;
#7459=CARTESIAN_POINT ( 'NONE',  ( 9.999999999999742428, 5.773502691896404748, -158.2500000040967905 ) ) ;
#7460=CARTESIAN_POINT ( 'NONE',  ( 10.81189881249999907, 6.242252689847868297, -173.9062500020484094 ) ) ;
#7462=CARTESIAN_POINT ( 'NONE',  ( 5.000000000000000000, 8.660254037844385522, -147.6250000040967905 ) ) ;
#7464=CARTESIAN_POINT ( 'NONE',  ( -9.999999999999998224, 1.224646799147353059E-15, -89.74999999999998579 ) ) ;
#7465=CARTESIAN_POINT ( 'NONE',  ( 0.000000000000000000, 0.000000000000000000, -200.0000000000000000 ) ) ;
#7467=CARTESIAN_POINT ( 'NONE',  ( 10.81189881249999907, 6.242252689847868297, -82.40625000204836681 ) ) ;
#7471=ORIENTED_EDGE ( 'NONE', *, *, #8724, .F. ) ;
#7472=CARTESIAN_POINT ( 'NONE',  ( 5.405949406249999534, 9.363379034771803333, -23.59375000204835970 ) ) ;
#7473=CARTESIAN_POINT ( 'NONE',  ( 10.81189881249999907, 6.242252689847868297, -16.40625000204838102 ) ) ;
#7474=CARTESIAN_POINT ( 'NONE',  ( 10.81189881249999729, 0.000000000000000000, -68.84375000204836681 ) ) ;
#7475=CARTESIAN_POINT ( 'NONE',  ( 7.070501591499376803E-16, 11.54700538379251284, -93.12500000000000000 ) ) ;
#7477=EDGE_CURVE ( 'NONE', #30730, #6810, #8130, .T. ) ;
#7478=VECTOR ( 'NONE', #14412, 1000.000000000000000 ) ;
#7479=CARTESIAN_POINT ( 'NONE',  ( 7.644554776091147741E-16, 12.48450537969573659, -185.4687500020483810 ) ) ;
#7481=CARTESIAN_POINT ( 'NONE',  ( 10.81189881249999551, -6.242252689847874514, 0.03124999795165228286 ) ) ;
#7482=CARTESIAN_POINT ( 'NONE',  ( 5.000000000000000000, 8.660254037844385522, -59.12500000409676204 ) ) ;
#7483=CARTESIAN_POINT ( 'NONE',  ( 9.999999999999998224, 0.000000000000000000, -141.5000000000000000 ) ) ;
#7484=DIRECTION ( 'NONE',  ( 1.000000000000000000, 0.000000000000000000, 0.000000000000000000 ) ) ;
#7485=CARTESIAN_POINT ( 'NONE',  ( -5.405949406249996869, 9.363379034771805109, -113.3437500020483810 ) ) ;
#7486=CARTESIAN_POINT ( 'NONE',  ( 9.999999999999998224, 0.000000000000000000, -54.87500000409675494 ) ) ;
#7487=CARTESIAN_POINT ( 'NONE',  ( -5.405949406249996869, 9.363379034771805109, -91.03125000204838102 ) ) ;
#7488=CARTESIAN_POINT ( 'NONE',  ( -10.81189881249999729, -6.242252689847864744, -102.4687500020483810 ) ) ;
#7491=CARTESIAN_POINT ( 'NONE',  ( 5.000000000000000000, 8.660254037844385522, -165.6250000040967905 ) ) ;
#7492=( BOUNDED_CURVE ( )  B_SPLINE_CURVE ( 2, ( #30670, #37991, #4976, #18122, #31317, #1532, #5188 ),
 .UNSPECIFIED., .F., .F. ) 
 B_SPLINE_CURVE_WITH_KNOTS ( ( 3, 2, 2, 3 ),
 ( 0.4813432835820896649, 0.4825870646766170502, 0.4838308457711443800, 0.4850746268656717652 ),
 .UNSPECIFIED. ) 
 CURVE ( )  GEOMETRIC_REPRESENTATION_ITEM ( )  RATIONAL_B_SPLINE_CURVE ( ( 0.9999999999999880096, 0.8660254037844506980, 1.000000000000000000, 0.8660254037844387076, 1.000000000000000000, 0.8660254037844267172, 1.000000000000011990 ) ) 
 REPRESENTATION_ITEM ( '' )  );
#7496=CARTESIAN_POINT ( 'NONE',  ( -9.999999999999479527, -5.773502691896549521, -109.1249999999999716 ) ) ;
#7498=CARTESIAN_POINT ( 'NONE',  ( -4.999999999999996447, 8.660254037844387298, -62.99999999999997158 ) ) ;
#7499=CARTESIAN_POINT ( 'NONE',  ( -2.121150477449813534E-15, -11.54700538379251284, -72.87499999999995737 ) ) ;
#7501=CARTESIAN_POINT ( 'NONE',  ( 5.000000000000000000, 8.660254037844385522, -89.12500000409677625 ) ) ;
#7502=EDGE_CURVE ( 'NONE', #7578, #22008, #25989, .T. ) ;
#7505=CARTESIAN_POINT ( 'NONE',  ( -10.81189881249999729, -6.242252689847864744, -86.15625000204836681 ) ) ;
#7507=( BOUNDED_CURVE ( )  B_SPLINE_CURVE ( 2, ( #4271, #14163, #33635, #10943, #37714, #37279, #4482 ),
 .UNSPECIFIED., .F., .F. ) 
 B_SPLINE_CURVE_WITH_KNOTS ( ( 3, 2, 2, 3 ),
 ( 0.1567164179104477695, 0.1579601990049751270, 0.1592039800995025123, 0.1604477611940298698 ),
 .UNSPECIFIED. ) 
 CURVE ( )  GEOMETRIC_REPRESENTATION_ITEM ( )  RATIONAL_B_SPLINE_CURVE ( ( 1.000000000000000000, 0.8660254037844387076, 1.000000000000000000, 0.8660254037844387076, 1.000000000000000000, 0.8660254037844357100, 1.000000000000003109 ) ) 
 REPRESENTATION_ITEM ( '' )  );
#7509=CARTESIAN_POINT ( 'NONE',  ( 7.070501591499376803E-16, 11.54700538379251284, -19.62499999999997868 ) ) ;
#7511=ORIENTED_EDGE ( 'NONE', *, *, #38584, .F. ) ;
#7512=CARTESIAN_POINT ( 'NONE',  ( -5.405949406249996869, 9.363379034771805109, -197.5312500020484094 ) ) ;
#7513=EDGE_CURVE ( 'NONE', #36795, #36659, #30795, .T. ) ;
#7515=CARTESIAN_POINT ( 'NONE',  ( -2.293366432827344421E-15, -12.48450537969573659, -16.71875000204836326 ) ) ;
#7516=FACE_OUTER_BOUND ( 'NONE', #8391, .T. ) ;
#7518=CARTESIAN_POINT ( 'NONE',  ( 10.81189881249999907, 6.242252689847868297, -137.9062500020483810 ) ) ;
#7519=CARTESIAN_POINT ( 'NONE',  ( -9.999999999999998224, 1.224646799147353059E-15, -190.2500000000000000 ) ) ;
#7521=CARTESIAN_POINT ( 'NONE',  ( 7.644554776091147741E-16, 12.48450537969573659, -110.6562500020483952 ) ) ;
#7522=ORIENTED_EDGE ( 'NONE', *, *, #26988, .F. ) ;
#7524=ORIENTED_EDGE ( 'NONE', *, *, #38472, .T. ) ;
#7525=ORIENTED_EDGE ( 'NONE', *, *, #7371, .T. ) ;
#7527=CARTESIAN_POINT ( 'NONE',  ( 10.81189881249999907, 6.242252689847868297, -41.90625000204836681 ) ) ;
#7529=CARTESIAN_POINT ( 'NONE',  ( 5.405949406249999534, 9.363379034771803333, -95.59375000204838102 ) ) ;
#7531=DIRECTION ( 'NONE',  ( -0.000000000000000000, -0.000000000000000000, 1.000000000000000000 ) ) ;
#7532=CARTESIAN_POINT ( 'NONE',  ( 5.405949406249992428, -9.363379034771808662, -195.0937500020484094 ) ) ;
#7534=CARTESIAN_POINT ( 'NONE',  ( 7.070501591499376803E-16, 11.54700538379251284, -138.1250000000000000 ) ) ;
#7535=CARTESIAN_POINT ( 'NONE',  ( -10.81189881249999729, -6.242252689847864744, -123.4687500020483952 ) ) ;
#7537=CARTESIAN_POINT ( 'NONE',  ( -9.999999999999998224, 1.224646799147353059E-15, -200.0000000000000000 ) ) ;
#7539=CARTESIAN_POINT ( 'NONE',  ( 5.000000000000000000, 8.660254037844385522, -188.1250000040967905 ) ) ;
#7541=CARTESIAN_POINT ( 'NONE',  ( 10.81189881249999729, 0.000000000000000000, -177.0312500020483810 ) ) ;
#7542=CARTESIAN_POINT ( 'NONE',  ( -4.999999999999996447, 8.660254037844387298, -180.0000000000000000 ) ) ;
#7545=CARTESIAN_POINT ( 'NONE',  ( 7.644554776091147741E-16, 12.48450537969573659, -50.46875000204835970 ) ) ;
#7547=CARTESIAN_POINT ( 'NONE',  ( 10.81189881249999551, -6.242252689847874514, -38.96875000204835970 ) ) ;
#7549=CARTESIAN_POINT ( 'NONE',  ( 10.81189881249999907, 6.242252689847868297, -10.40625000204838102 ) ) ;
#7553=CARTESIAN_POINT ( 'NONE',  ( -5.000000000000003553, -8.660254037844383745, -93.99999999999998579 ) ) ;
#7555=CARTESIAN_POINT ( 'NONE',  ( 9.999999999999996447, -5.773502691896262640, -115.0000000040967763 ) ) ;
#7559=CARTESIAN_POINT ( 'NONE',  ( -10.81189881249999729, 1.324075727343319199E-15, -104.2812500020483810 ) ) ;
#7560=EDGE_LOOP ( 'NONE', ( #29972, #2396, #18984, #18332 ) ) ;
#7561=DIRECTION ( 'NONE',  ( 1.000000000000000000, 0.000000000000000000, 0.000000000000000000 ) ) ;
#7566=CARTESIAN_POINT ( 'NONE',  ( 9.999999999999996447, -5.773502691896262640, -36.62499999999996447 ) ) ;
#7567=CARTESIAN_POINT ( 'NONE',  ( -2.293366432827344421E-15, -12.48450537969573659, -34.90625000204836681 ) ) ;
#7568=CARTESIAN_POINT ( 'NONE',  ( 7.070501591499377789E-16, 11.54700538379251284, -165.1249999999999716 ) ) ;
#7569=CARTESIAN_POINT ( 'NONE',  ( -9.999999999999998224, 1.224646799147353059E-15, -16.24999999999995737 ) ) ;
#7572=CARTESIAN_POINT ( 'NONE',  ( 5.405949406249999534, 9.363379034771803333, -137.7812500020483810 ) ) ;
#7574=CARTESIAN_POINT ( 'NONE',  ( -9.999999999999998224, 1.224646799147353059E-15, -120.1250000040967905 ) ) ;
#7575=ORIENTED_EDGE ( 'NONE', *, *, #17475, .T. ) ;
#7577=EDGE_LOOP ( 'NONE', ( #9073, #29878, #38732, #42687 ) ) ;
#7578=VERTEX_POINT ( 'NONE', #7483 ) ;
#7580=EDGE_CURVE ( 'NONE', #24932, #8912, #38958, .T. ) ;
#7581=CARTESIAN_POINT ( 'NONE',  ( -9.999999999999998224, 1.224646799147353059E-15, -55.62500000409676204 ) ) ;
#7582=CARTESIAN_POINT ( 'NONE',  ( -5.405949406249996869, 9.363379034771805109, -168.8437500020484094 ) ) ;
#7584=CARTESIAN_POINT ( 'NONE',  ( 5.405949406249992428, -9.363379034771808662, -12.09375000204834727 ) ) ;
#7585=CYLINDRICAL_SURFACE ( 'NONE', #37771, 9.999999999999998224 ) ;
#7586=CARTESIAN_POINT ( 'NONE',  ( 10.81189881249999729, 0.000000000000000000, -151.3437500020483810 ) ) ;
#7587=CARTESIAN_POINT ( 'NONE',  ( -10.81189881249999907, -6.242252689847864744, -135.4687500020483810 ) ) ;
#7588=CARTESIAN_POINT ( 'NONE',  ( 10.81189881249999907, 6.242252689847868297, -107.9062500020483668 ) ) ;
#7592=CARTESIAN_POINT ( 'NONE',  ( -2.293366432827344421E-15, -12.48450537969573659, -12.21875000204837391 ) ) ;
#7594=CARTESIAN_POINT ( 'NONE',  ( -9.999999999999998224, 1.224646799147353059E-15, -63.12500000409676204 ) ) ;
#7598=CARTESIAN_POINT ( 'NONE',  ( -5.405949406249996869, 9.363379034771805109, -72.84375000204838102 ) ) ;
#7599=CARTESIAN_POINT ( 'NONE',  ( 5.405949406249999534, 9.363379034771803333, -65.59375000204836681 ) ) ;
#7600=CARTESIAN_POINT ( 'NONE',  ( -2.121150477449813534E-15, -11.54700538379251284, -116.7500000040967905 ) ) ;
#7601=CARTESIAN_POINT ( 'NONE',  ( -10.81189881249999729, 6.242252689847871849, -38.40625000204835260 ) ) ;
#7603=DIRECTION ( 'NONE',  ( -0.000000000000000000, -0.000000000000000000, 1.000000000000000000 ) ) ;
#7605=CARTESIAN_POINT ( 'NONE',  ( 9.999999999999996447, -5.773502691896262640, -132.6249999999999716 ) ) ;
#7606=CARTESIAN_POINT ( 'NONE',  ( -5.405949406249996869, 9.363379034771805109, -130.0312500020484094 ) ) ;
#7609=CARTESIAN_POINT ( 'NONE',  ( -5.405949406249996869, 9.363379034771805109, -16.03125000204835970 ) ) ;
#7613=CARTESIAN_POINT ( 'NONE',  ( 4.999999999999992006, -8.660254037844389075, -185.2500000000000000 ) ) ;
#7614=VECTOR ( 'NONE', #37563, 1000.000000000000000 ) ;
#7615=CARTESIAN_POINT ( 'NONE',  ( 9.999999999999996447, -5.773502691896262640, -31.00000000409674783 ) ) ;
#7616=CARTESIAN_POINT ( 'NONE',  ( -9.999999999999998224, 1.224646799147353059E-15, -11.74999999999995559 ) ) ;
#7618=( BOUNDED_CURVE ( )  B_SPLINE_CURVE ( 2, ( #30692, #27022, #24223, #40168, #23786, #1125, #14248, #11029, #37373, #24868, #38437, #38652, #34792, #15334, #5433, #5006, #5212, #41869, #41663, #28531, #18584, #12306, #5646, #21612, #19007, #35215, #32192, #12099, #18148, #28949, #25293, #31343, #1989, #42086, #18368, #11885, #25503, #9087, #1773, #31556, #8880, #2619, #22255, #41450, #28103, #31772, #35004, #15751, #22043, #18794, #31983, #14903, #41230, #2409, #15540, #24656, #28742, #2201, #35425, #28310, #5852, #37799, #8244, #21392, #34576, #25081, #11667, #38017, #8461, #15115, #38226, #8671, #21824, #19841, #23097, #6064, #36466, #9288, #23311, #42295, #39696, #234, #35637, #19423, #13141, #32404, #20055, #36049, #3038, #9504, #6902, #12928, #15960, #16165, #39488, #12518, #26123, #29156, #3455, #26336, #6485, #32816, #16591, #29361, #22460, #18, #25711, #9711, #2826, #39277, #3247, #19214, #13356, #39066, #33250, #22892, #42500, #16373, #12717, #32613, #26547, #25914, #30003, #22673, #35844, #19632, #6277, #38861, #10132, #29573, #9921, #36260, #6690, #33026, #29794, #3676, #16804, #23954, #17444, #20908, #10340, #10975, #14196, #30640, #26757, #17656, #11193, #36887, #13778, #36678, #7973, #27179, #40532, #40119, #866, #7333, #30851, #23736, #10551, #20482, #1072, #23528, #17022, #4726, #39909, #660, #7118, #33669, #24171, #40322, #34090, #4093, #20272, #17235, #27395, #37318, #4513, #33460, #10763, #13982, #7541, #30436, #33883, #37098, #1288, #20695, #3887, #30221, #26962, #4305, #7764, #14417, #27611, #17875, #40751, #24391, #37532, #21122, #34311, #449, #13566, #18528, #15487, #38386, #31504, #21560, #24597, #28692, #31291, #2148, #2360, #41172, #21774, #11831, #11403, #11611, #5588, #5377, #34952, #25031, #34740, #12046, #28045, #25450, #41612, #38596, #31717, #37746, #35375, #15283, #8190, #8409, #6385, #24819, #18314, #31933, #18741, #21337, #37964, #28481, #34526, #41819, #5162, #4949, #38174, #41396, #9036, #25242, #8827, #21984, #18096, #1720, #35162, #12257, #31071, #22201, #8618, #1505, #1934, #40960, #14639, #27827, #15061, #14849, #28259, #33563, #13039, #16703, #16487, #29900, #40223, #3987, #6798, #6585, #30331, #17129, #39383, #36999, #26233, #129, #39590, #3144, #7223, #32921, #10025, #13252, #3355, #23205, #16913, #9816, #10657, #338, #36571, #40018, #29470, #29686, #42612, #22996, #27080, #761, #13884, #26439, #36364, #36152, #23850, #3569, #30115, #19953, #33141, #19741, #13459, #26653, #39803, #10235, #23422, #7017, #19527, #16271, #20169, #33359, #3779, #552, #13672, #26864, #10448, #32711, #23640, #36786, #20374, #972, #5057, #7651, #21234, #21448, #17550, #40857, #30967, #30544, #30751, #24712, #24491, #37858, #27936, #8302, #31184, #4411, #1829, #17984, #14957, #11297, #14089, #11728, #37644, #27290, #27506, #24926, #1184, #37428, #34631, #18205, #40427, #7871, #31395, #28155, #41289, #24283, #10870, #14527, #17771, #7434, #8083, #34420, #4839, #24062, #37204, #1614, #14743, #20587, #41065, #27721, #11510, #34209, #17341, #14306, #1397, #21019, #33775, #20802, #4197, #33990, #4625, #40640, #11081, #16018, #9353, #25347, #25134, #6124, #22522, #15174, #12786, #5487, #12154, #41716, #38922, #35695, #19269, #8937, #11943, #5915, #32039, #28587, #35487, #32463, #31831, #38071, #2267, #29214, #21881, #19067, #9146, #2888, #42353, #8511, #38712, #18637, #35059, #2675, #21665, #15809, #34846, #5269, #29005, #22101, #42145, #18421, #31611, #12576, #35275, #2043, #28371, #15388, #25561, #2470, #25769, #41510, #38280, #28800, #8727, #38493, #5708, #15598, #18859, #32248, #22314, #41932, #12363, #26396, #16438, #19482, #23593, #39547, #33090, #19905, #25977, #10192, #9773, #36739, #33523, #22736, #30070, #512, #3737, #13627, #6968, #22953, #20329, #36527, #3946, #29855, #32668, #20124, #3097, #7177, #35902, #17084, #12989, #10402, #293, #19695, #30283, #13203, #722, #39128, #39972, #80, #29425, #3517, #36320, #9562, #13414, #23377, #6339, #9978, #42566, #16867, #39757, #16654, #26186, #26608, #33312, #23157, #16226, #36107, #26820, #6751, #39334, #6541, #32878, #3309, #29636, #1572, #4371, #20760, #24235, #4154, #24018, #24452, #37159, #7395, #10825, #27240, #33949, #17510, #37598, #8042, #21187, #30706, #17297, #17722, #27463, #4582, #20542, #31139, #14260, #37386, #27677, #10611, #14045, #23798, #36953, #17940, #34376, #4792, #20976, #40383, #7606, #14482, #14702, #27891, #40180, #7829, #40598, #1137, #13841, #1352, #40815, #30917, #33731, #30502, #11041, #11255, #27035, #34161, #928, #6473, #20469, #39475, #36875, #26742, #3442, #39683, #7317, #4080, #23724, #26534, #13126, #16791, #20042, #30423, #39896, #13555, #10327, #3234, #26324, #3875, #33447, #27167, #17011, #29991, #13763, #36455, #19615, #19828, #3663, #10117, #33657, #32800, #17218, #16359, #6889, #6677, #33237, #854, #13972, #23297, #9908, #9697, #22876, #29558, #36036, #33013, #436, #13343, #10538, #5, #23084, #23515, #36244, #20260, #36664, #222, #7105, #16579, #29782, #30208, #644, #26951, #40107, #9936, #36065, #25727, #6709, #16608, #42311, #19229, #42100, #13373, #32628, #3264, #2841, #6293, #12733, #36278, #29171, #15975, #25933, #6500, #12945, #13158, #23115, #32207, #6083, #2636, #39082, #16393, #3054, #39505, #9521, #15766, #22691, #22909, #29592, #19861, #28963, #16180, #19436, #26140, #42519, #5868, #32835, #12534, #9726, #38876, #22476, #36, #26352, #23331, #33046, #39292, #3473, #35859, #9307, #19649, #19022, #29377, #35652, #29811, #251, #32419, #26565, #39714, #10149, #14434, #7782, #23752, #23546, #4530, #20926, #13582, #11209, #467, #17038, #13796, #36695, #20072, #24188, #7134, #26978, #30238, #20288, #40138, #33900, #37335, #677, #36483, #10566, #27628, #33476, #4323, #39927, #26774, #10355, #34108, #17672, #36905, #3904, #30020, #1303, #20498, #17461, #30867, #14214, #7350, #33685, #4110, #17251, #30452, #881, #3693, #14000, #40767, #33267, #27195, #16821, #40339, #30660, #10781, #27413, #23970, #37115, #1088, #7559, #20712, #40549, #6920, #10993, #38190, #38402, #34540, #15076, #5177, #4744, #4964, #41627, #41413, #28277, #18331, #28062, #2375, #5394, #18757, #34970, #31947, #11847, #17890, #28707, #25048, #31088, #1739, #41834, #18112, #11629, #25257, #12061, #1521, #31307, #8634, #14655, #15502, #31521, #27844, #1950, #34757, #24407, #21790, #18546, #31735, #2165, #15299, #7988, #21577, #37980, #28496, #8844, #37549, #22002, #8207, #35178, #21140, #34326, #5603, #40976, #41188, #11420, #24614, #37763, #21355, #14865, #24835, #8425, #19596, #22854, #5816, #36221, #9050, #23065, #42051, #39455, #29326, #6030, #19180, #12897, #32156, #19806, #35812, #2793, #9255, #6656, #12684, #15715, #15923, #39243, #12271, #25881, #28914, #3214, #26092, #6244, #12479, #9681, #29124, #22216, #42470, #25468, #9471, #2586, #39035, #3005, #35392, #42681, #38826, #32994, #22639, #42259, #16129, #25672, #32369, #13107, #19388, #18969, #22424, #32579, #36016, #26306, #9890, #3422, #6455, #35602, #32778, #16341, #29539, #16559, #29757, #38613, #17622, #7086, #34058, #26719, #10729, #3644, #39871, #829, #24135, #13951, #10305, #23493, #7505, #14161, #20657, #40495, #27360, #33844, #13738, #36433, #6869, #20020, #413, #3852, #10097, #16771, #202, #33632, #10941, #23274, #20236, #20446, #622, #40287, #30398, #37277, #4269, #4055, #17197, #33213, #29971, #37065, #23921, #13323, #17410, #27144, #30608, #26928, #13533, #36640, #36852, #30185, #7725, #33425, #20872, #16986, #40086, #10516, #23703, #4479, #26512, #7296, #1036, #39661, #2114, #7938, #24563, #40924, #4912, #34490, #31680, #15244, #28443, #1682, #4691, #41358, #24782, #21302, #28225, #41579, #37712, #5551, #8154, #21947, #14601, #11795, #18273, #27791, #31462, #12011, #1896, #11367, #18060, #38139, #25207, #8583, #38349, #8789, #21734, #14811, #24353, #37494, #21088, #31036, #31255, #40712, #5337, #30816, #21523, #35127, #11154, #28007, #8373, #41135, #24998, #15025, #1255, #34915, #11576, #37927, #34276, #14379, #1467, #18492, #27576, #34705, #17840, #5125, #16290, #26251, #15456, #22800, #35964, #39194, #6403, #42419, #15662, #13058, #29276, #39401, #22586, #12219, #23015, #9420, #25411, #38779, #29489, #5768, #3163, #35763, #12427, #9836, #5981, #42628, #36169, #32728, #35552, #22166, #25829, #29071, #18703, #6191, #32317, #38557, #8998, #35340, #19333, #38984, #26042, #19544, #31899, #32525, #2327, #28655, #9205, #2954, #19132, #16081, #12850, #41785, #9628, #2742, #22374, #18921, #32105, #2537, #28863, #12635, #41998, #25622, #15869, #42209, #14107, #3371, #10674, #23868, #27096, #37016, #30348, #3588, #989, #17147, #27309, #10465, #149, #10889, #13269, #30560, #16506, #17358, #36384, #33792, #23655, #358, #40445, #36588, #4215, #24081, #20605, #23440, #10043, #13688, #16934, #6602, #36802, #7240, #19758, #20187, #23224, #40238, #20391, #569, #6817, #33583, #4004, #33377, #29703, #16722, #26880, #7035, #32941, #26458, #39608, #19972, #3797, #29917, #30132, #40035, #777, #33158, #13480, #7456, #39821, #26670, #10253, #13903, #11315, #40874, #38677, #9111, #35451, #8100, #11098, #5671, #31202, #27738, #14327, #15774, #18000, #11526, #15566, #4429, #34226, #41895, #24729, #4642, #37874, #19031, #8319, #17789, #30986, #2431, #22280, #28767, #5877, #32215, #1415, #14546, #21464, #1630, #12329, #25528, #12544, #27954, #2643, #17568, #24507, #14759, #37661, #35240, #18822, #28971, #42110, #21251, #34437, #30769, #4858, #41082, #32006, #37221, #7668, #20821, #21036, #34007, #1200, #27523, #40658, #24301, #37445, #7888, #6718, #22700, #20083, #36288, #33277, #29602, #33056, #19871, #19238, #6929, #22484, #36493, #12743, #10159, #45, #19446, #16831, #12954, #23341, #3702, #39724, #42529, #29180, #32844, #36073, #30030, #29387, #9944, #25735, #39300, #42319, #16618, #39515, #19659, #25942, #26363, #23124, #9738, #35660, #35869, #3273, #26149, #476, #6091, #38886, #32426, #9530, #9316, #22919, #6510, #16402, #39091, #32638, #26574, #16189, #2851, #3064, #6302, #13169, #3482, #15985, #29821, #261, #13382, #30247, #24197, #33693, #11003, #33486, #34334, #37123, #30668, #34118, #23555, #10574, #17681, #1096, #23760, #14223, #37557, #27424, #36913, #7359, #20935, #27636, #4539, #20507, #14008, #4120, #1311, #17259, #686, #39935, #14444, #26990, #30463, #890, #40147, #27203, #37346, #3912, #4752, #7567, #40559, #30877, #36703, #7793, #17046, #20295, #13803, #40776, #24417, #40347, #10790, #7142, #21148, #23980, #11217, #20720, #33911, #4331, #7996, #17470, #17899, #31097, #13592, #26783, #10364, #5824, #27852, #1747, #40986, #8433, #41635, #41421, #35185, #37989, #11428, #24842, #18555, #12071, #5612, #24625, #11858, #15087, #8643, #11638, #34978, #25056, #37772, #21586, #18766, #31745, #5404, #38199, #5186, #22226, #25265, #22012, #15308, #21365, #8216, #28284, #8852, #38411, #34548, #34765, #18979, #18340, #31530, #2384, #31955, #4974, #1958, #2173, #18120, #9058, #21798, #28505, #41198, #38622, #15511, #31315, #28716, #41842, #1530, #14874, #12280, #25476, #14663, #35400, #28071, #22431, #42058, #32164, #9263, #2594, #38834, #28922, #35610, #6037, #15723, #12487, #25681, #8045, #932, #1355, #17300, #17087, #40818, #14485, #7180, #4795, #36742, #10614, #7398, #33734, #39975, #17514, #30073, #27244, #20333, #14048, #20763, #10406, #17725, #27039, #40385, #21191, #27680, #30505, #30286, #11258, #24455, #33526, #515, #3949, #23802, #20546, #725, #13630, #30920, #13844, #4156, #36956, #40183, #10828, #27466, #37602, #24021, #26822, #37162, #34379, #7609, #40601, #33952, #4374, #30710, #23597, #1140, #14263, #11044, #24238, #37389, #7832, #20979, #34166, #4585, #5662, #41245, #14917, #28117, #5449, #25096, #25308, #35231, #35442, #8687, #28759, #27894, #38032, #38242, #18383, #15348, #18600, #2424, #35020, #28546, #8894, #1575, #15131, #31572, #21840, #11900, #17943, #2219, #1788, #15557, #25519, #14704, #22058, #18813, #38453, #31998, #41678, #11686, #31787, #37816, #41027, #2004, #41886, #12115, #11470, #12321, #24671, #38667, #5022, #9103, #22271, #24883, #31142, #5228, #8259, #21405, #34591, #34807, #8475, #18163, #28327, #31357, #21629, #41466, #8614, #32296, #28041, #14191, #27390, #37960, #34522, #18310, #21770, #40527, #41168, #10970, #24166, #8405, #14845, #11607, #40956, #37313, #24386, #8186, #1500, #41392, #7759, #28255, #20903, #11399, #11188, #24593, #34948, #11827, #14634, #1283, #25027, #38170, #34086, #7968, #37527, #31066, #17870, #15057, #5373, #19113, #27822, #30846, #24815, #21333, #4721, #21556, #4508, #21117, #17651, #34306 ),
 .UNSPECIFIED., .F., .F. ) 
 B_SPLINE_CURVE_WITH_KNOTS ( ( 3, 2, 2, 2, 2, 2, 2, 2, 2, 2, 2, 2, 2, 2, 2, 2, 2, 2, 2, 2, 2, 2, 2, 2, 2, 2, 2, 2, 2, 2, 2, 2, 2, 2, 2, 2, 2, 2, 2, 2, 2, 2, 2, 2, 2, 2, 2, 2, 2, 2, 2, 2, 2, 2, 2, 2, 2, 2, 2, 2, 2, 2, 2, 2, 2, 2, 2, 2, 2, 2, 2, 2, 2, 2, 2, 2, 2, 2, 2, 2, 2, 2, 2, 2, 2, 2, 2, 2, 2, 2, 2, 2, 2, 2, 2, 2, 2, 2, 2, 2, 2, 2, 2, 2, 2, 2, 2, 2, 2, 2, 2, 2, 2, 2, 2, 2, 2, 2, 2, 2, 2, 2, 2, 2, 2, 2, 2, 2, 2, 2, 2, 2, 2, 2, 2, 2, 2, 2, 2, 2, 2, 2, 2, 2, 2, 2, 2, 2, 2, 2, 2, 2, 2, 2, 2, 2, 2, 2, 2, 2, 2, 2, 2, 2, 2, 2, 2, 2, 2, 2, 2, 2, 2, 2, 2, 2, 2, 2, 2, 2, 2, 2, 2, 2, 2, 2, 2, 2, 2, 2, 2, 2, 2, 2, 2, 2, 2, 2, 2, 2, 2, 2, 2, 2, 2, 2, 2, 2, 2, 2, 2, 2, 2, 2, 2, 2, 2, 2, 2, 2, 2, 2, 2, 2, 2, 2, 2, 2, 2, 2, 2, 2, 2, 2, 2, 2, 2, 2, 2, 2, 2, 2, 2, 2, 2, 2, 2, 2, 2, 2, 2, 2, 2, 2, 2, 2, 2, 2, 2, 2, 2, 2, 2, 2, 2, 2, 2, 2, 2, 2, 2, 2, 2, 2, 2, 2, 2, 2, 2, 2, 2, 2, 2, 2, 2, 2, 2, 2, 2, 2, 2, 2, 2, 2, 2, 2, 2, 2, 2, 2, 2, 2, 2, 2, 2, 2, 2, 2, 2, 2, 2, 2, 2, 2, 2, 2, 2, 2, 2, 2, 2, 2, 2, 2, 2, 2, 2, 2, 2, 2, 2, 2, 2, 2, 2, 2, 2, 2, 2, 2, 2, 2, 2, 2, 2, 2, 2, 2, 2, 2, 2, 2, 2, 2, 2, 2, 2, 2, 2, 2, 2, 2, 2, 2, 2, 2, 2, 2, 2, 2, 2, 2, 2, 2, 2, 2, 2, 2, 2, 2, 2, 2, 2, 2, 2, 2, 2, 2, 2, 2, 2, 2, 2, 2, 2, 2, 2, 2, 2, 2, 2, 2, 2, 2, 2, 2, 2, 2, 2, 2, 2, 2, 2, 2, 2, 2, 2, 2, 2, 2, 2, 2, 2, 2, 2, 2, 2, 2, 2, 2, 2, 2, 2, 2, 2, 2, 2, 2, 2, 2, 2, 2, 2, 2, 2, 2, 2, 2, 2, 2, 2, 2, 2, 2, 2, 2, 2, 2, 2, 2, 2, 2, 2, 2, 2, 2, 2, 2, 2, 2, 2, 2, 2, 2, 2, 2, 2, 2, 2, 2, 2, 2, 2, 2, 2, 2, 2, 2, 2, 2, 2, 2, 2, 2, 2, 2, 2, 2, 2, 2, 2, 2, 2, 2, 2, 2, 2, 2, 2, 2, 2, 2, 2, 2, 2, 2, 2, 2, 2, 2, 2, 2, 2, 2, 2, 2, 2, 2, 2, 2, 2, 2, 2, 2, 2, 2, 2, 2, 2, 2, 2, 2, 2, 2, 2, 2, 2, 2, 2, 2, 2, 2, 2, 2, 2, 2, 2, 2, 2, 2, 2, 2, 2, 2, 2, 2, 2, 2, 2, 2, 2, 2, 2, 2, 2, 2, 2, 2, 2, 2, 2, 2, 2, 2, 2, 2, 2, 2, 2, 2, 2, 2, 2, 2, 2, 2, 2, 2, 2, 2, 2, 2, 2, 2, 2, 2, 2, 2, 2, 2, 2, 2, 2, 2, 2, 2, 2, 2, 2, 2, 2, 2, 2, 2, 2, 2, 2, 2, 2, 2, 2, 2, 2, 2, 2, 2, 2, 2, 2, 2, 2, 2, 2, 2, 2, 2, 2, 2, 2, 2, 2, 2, 2, 2, 2, 2, 2, 2, 2, 2, 2, 2, 2, 2, 2, 2, 2, 2, 2, 2, 2, 2, 2, 2, 2, 2, 2, 2, 2, 2, 2, 2, 2, 2, 2, 2, 2, 2, 2, 2, 2, 2, 2, 2, 2, 2, 2, 2, 2, 2, 2, 2, 2, 2, 2, 2, 2, 2, 2, 2, 2, 2, 2, 2, 2, 2, 2, 2, 2, 2, 2, 2, 2, 2, 2, 2, 2, 2, 2, 2, 2, 2, 2, 2, 2, 2, 2, 2, 2, 2, 2, 2, 2, 2, 2, 2, 2, 2, 2, 2, 2, 2, 2, 2, 2, 2, 2, 2, 2, 2, 2, 2, 2, 2, 2, 2, 2, 2, 2, 2, 2, 2, 2, 2, 2, 2, 2, 2, 2, 2, 2, 2, 2, 2, 2, 2, 2, 2, 2, 2, 2, 2, 2, 2, 2, 2, 2, 2, 2, 3 ),
 ( 0.000000000000000000, 0.001243781094527363160, 0.002487562189054726321, 0.003731343283582089481, 0.004975124378109452641, 0.006218905472636816235, 0.007462686567164178962, 0.008706467661691542556, 0.009950248756218905283, 0.01119402985074626801, 0.01243781094527363247, 0.01368159203980099520, 0.01492537313432835792, 0.01616915422885572065, 0.01741293532338308511, 0.01865671641791044610, 0.01990049751243781057, 0.02114427860696517503, 0.02238805970149253602, 0.02363184079601990048, 0.02487562189054726494, 0.02611940298507462593, 0.02736318407960199039, 0.02860696517412935486, 0.02985074626865671585, 0.03109452736318408031, 0.03233830845771144130, 0.03358208955223880576, 0.03482587064676617022, 0.03606965174129353469, 0.03731343283582089221, 0.03855721393034825667, 0.03980099502487562113, 0.04104477611940298559, 0.04228855721393035005, 0.04353233830845771452, 0.04477611940298507204, 0.04601990049751243650, 0.04726368159203980096, 0.04850746268656716542, 0.04975124378109452988, 0.05099502487562188741, 0.05223880597014925187, 0.05348258706467661633, 0.05472636815920398079, 0.05597014925373134525, 0.05721393034825870971, 0.05845771144278606724, 0.05970149253731343170, 0.06094527363184079616, 0.06218905472636816062, 0.06343283582089552508, 0.06467661691542288260, 0.06592039800995025400, 0.06716417910447761153, 0.06840796019900496905, 0.06965174129353234045, 0.07089552238805969797, 0.07213930348258706937, 0.07338308457711442689, 0.07462686567164178442, 0.07587064676616915582, 0.07711442786069651334, 0.07835820895522388474, 0.07960199004975124226, 0.08084577114427861366, 0.08208955223880597118, 0.08333333333333332871, 0.08457711442786070011, 0.08582089552238805763, 0.08706467661691542903, 0.08830845771144278655, 0.08955223880597014408, 0.09079601990049751548, 0.09203980099502487300, 0.09328358208955224440, 0.09452736318407960192, 0.09577114427860695944, 0.09701492537313433084, 0.09825870646766168837, 0.09950248756218905977, 0.1007462686567164173, 0.1019900497512437748, 0.1032338308457711462, 0.1044776119402985037, 0.1057213930348258751, 0.1069651741293532327, 0.1082089552238805902, 0.1094527363184079616, 0.1106965174129353191, 0.1119402985074626905, 0.1131840796019900480, 0.1144278606965174194, 0.1156716417910447769, 0.1169154228855721345, 0.1181592039800995059, 0.1194029850746268634, 0.1206467661691542348, 0.1218905472636815923, 0.1231343283582089498, 0.1243781094527363212, 0.1256218905472636926, 0.1268656716417910502, 0.1281094527363184077, 0.1293532338308457652, 0.1305970149253731227, 0.1318407960199005080, 0.1330845771144278655, 0.1343283582089552231, 0.1355721393034825806, 0.1368159203980099381, 0.1380597014925373234, 0.1393034825870646809, 0.1405472636815920384, 0.1417910447761193959, 0.1430348258706467535, 0.1442786069651741387, 0.1455223880597014963, 0.1467661691542288538, 0.1480099502487562113, 0.1492537313432835688, 0.1504975124378109541, 0.1517412935323383116, 0.1529850746268656692, 0.1542288557213930267, 0.1554726368159203842, 0.1567164179104477695, 0.1579601990049751270, 0.1592039800995024845, 0.1604477611940298420, 0.1616915422885572273, 0.1629353233830845848, 0.1641791044776119424, 0.1654228855721392999, 0.1666666666666666574, 0.1679104477611940427, 0.1691542288557214002, 0.1703980099502487577, 0.1716417910447761153, 0.1728855721393034728, 0.1741293532338308581, 0.1753731343283582156, 0.1766169154228855731, 0.1778606965174129306, 0.1791044776119402882, 0.1803482587064676734, 0.1815920398009950310, 0.1828358208955223885, 0.1840796019900497460, 0.1853233830845771035, 0.1865671641791044888, 0.1878109452736318463, 0.1890547263681592038, 0.1902985074626865614, 0.1915422885572139189, 0.1927860696517413042, 0.1940298507462686617, 0.1952736318407960192, 0.1965174129353233767, 0.1977611940298507343, 0.1990049751243781195, 0.2002487562189054771, 0.2014925373134328346, 0.2027363184079601921, 0.2039800995024875496, 0.2052238805970149349, 0.2064676616915422924, 0.2077114427860696499, 0.2089552238805970075, 0.2101990049751243650, 0.2114427860696517503, 0.2126865671641791078, 0.2139303482587064653, 0.2151741293532338228, 0.2164179104477611804, 0.2176616915422885656, 0.2189054726368159232, 0.2201492537313432807, 0.2213930348258706382, 0.2226368159203980235, 0.2238805970149253810, 0.2251243781094527385, 0.2263681592039800961, 0.2276119402985074536, 0.2288557213930348389, 0.2300995024875621964, 0.2313432835820895539, 0.2325870646766169114, 0.2338308457711442689, 0.2350746268656716542, 0.2363184079601990117, 0.2375621890547263693, 0.2388059701492537268, 0.2400497512437810843, 0.2412935323383084696, 0.2425373134328358271, 0.2437810945273631846, 0.2450248756218905422, 0.2462686567164178997, 0.2475124378109452850, 0.2487562189054726425, 0.2500000000000000000, 0.2512437810945273853, 0.2524875621890547150, 0.2537313432835821003, 0.2549751243781094301, 0.2562189054726368154, 0.2574626865671642006, 0.2587064676616915304, 0.2599502487562189157, 0.2611940298507462455, 0.2624378109452736307, 0.2636815920398010160, 0.2649253731343283458, 0.2661691542288557311, 0.2674129353233830608, 0.2686567164179104461, 0.2699004975124378314, 0.2711442786069651611, 0.2723880597014925464, 0.2736318407960198762, 0.2748756218905472615, 0.2761194029850746468, 0.2773631840796019765, 0.2786069651741293618, 0.2798507462686566916, 0.2810945273631840768, 0.2823383084577114621, 0.2835820895522387919, 0.2848258706467661772, 0.2860696517412935069, 0.2873134328358208922, 0.2885572139303482775, 0.2898009950248756073, 0.2910447761194029925, 0.2922885572139303223, 0.2935323383084577076, 0.2947761194029850929, 0.2960199004975124226, 0.2972636815920398079, 0.2985074626865671377, 0.2997512437810945229, 0.3009950248756219082, 0.3022388059701492380, 0.3034825870646766233, 0.3047263681592039530, 0.3059701492537313383, 0.3072139303482587236, 0.3084577114427860534, 0.3097014925373134386, 0.3109452736318407684, 0.3121890547263681537, 0.3134328358208955390, 0.3146766169154228687, 0.3159203980099502540, 0.3171641791044776393, 0.3184079601990049690, 0.3196517412935323543, 0.3208955223880596841, 0.3221393034825870694, 0.3233830845771144546, 0.3246268656716417844, 0.3258706467661691697, 0.3271144278606964995, 0.3283582089552238847, 0.3296019900497512700, 0.3308457711442785998, 0.3320895522388059851, 0.3333333333333333148, 0.3345771144278607001, 0.3358208955223880854, 0.3370646766169154152, 0.3383084577114428004, 0.3395522388059701302, 0.3407960199004975155, 0.3420398009950249008, 0.3432835820895522305, 0.3445273631840796158, 0.3457711442786069456, 0.3470149253731343308, 0.3482587064676617161, 0.3495024875621890459, 0.3507462686567164312, 0.3519900497512437609, 0.3532338308457711462, 0.3544776119402985315, 0.3557213930348258613, 0.3569651741293532465, 0.3582089552238805763, 0.3594527363184079616, 0.3606965174129353469, 0.3619402985074626766, 0.3631840796019900619, 0.3644278606965173917, 0.3656716417910447769, 0.3669154228855721622, 0.3681592039800994920, 0.3694029850746268773, 0.3706467661691542070, 0.3718905472636815923, 0.3731343283582089776, 0.3743781094527363074, 0.3756218905472636926, 0.3768656716417910224, 0.3781094527363184077, 0.3793532338308457930, 0.3805970149253731227, 0.3818407960199005080, 0.3830845771144278378, 0.3843283582089552231, 0.3855721393034826083, 0.3868159203980099381, 0.3880597014925373234, 0.3893034825870646531, 0.3905472636815920384, 0.3917910447761194237, 0.3930348258706467535, 0.3942786069651741387, 0.3955223880597014685, 0.3967661691542288538, 0.3980099502487562391, 0.3992537313432835688, 0.4004975124378109541, 0.4017412935323382839, 0.4029850746268656692, 0.4042288557213930544, 0.4054726368159203842, 0.4067164179104477695, 0.4079601990049750992, 0.4092039800995024845, 0.4104477611940298698, 0.4116915422885571996, 0.4129353233830845848, 0.4141791044776119146, 0.4154228855721392999, 0.4166666666666666297, 0.4179104477611940149, 0.4191542288557214002, 0.4203980099502487300, 0.4216417910447761153, 0.4228855721393035005, 0.4241293532338308303, 0.4253731343283582156, 0.4266169154228855454, 0.4278606965174129306, 0.4291044776119403159, 0.4303482587064676457, 0.4315920398009950310, 0.4328358208955223607, 0.4340796019900497460, 0.4353233830845771313, 0.4365671641791044610, 0.4378109452736318463, 0.4390547263681592316, 0.4402985074626865614, 0.4415422885572139466, 0.4427860696517412764, 0.4440298507462686617, 0.4452736318407960470, 0.4465174129353233767, 0.4477611940298507620, 0.4490049751243780918, 0.4502487562189054771, 0.4514925373134328623, 0.4527363184079601921, 0.4539800995024875774, 0.4552238805970149071, 0.4564676616915422924, 0.4577114427860696777, 0.4589552238805970075, 0.4601990049751243927, 0.4614427860696517225, 0.4626865671641791078, 0.4639303482587064931, 0.4651741293532338228, 0.4664179104477612081, 0.4676616915422885379, 0.4689054726368159232, 0.4701492537313433084, 0.4713930348258706382, 0.4726368159203980235, 0.4738805970149253532, 0.4751243781094527385, 0.4763681592039801238, 0.4776119402985074536, 0.4788557213930348389, 0.4800995024875621686, 0.4813432835820895539, 0.4825870646766169392, 0.4838308457711442689, 0.4850746268656716542, 0.4863184079601989840, 0.4875621890547263693, 0.4888059701492537545, 0.4900497512437810843, 0.4912935323383084696, 0.4925373134328357994, 0.4937810945273631846, 0.4950248756218905699, 0.4962686567164178997, 0.4975124378109452850, 0.4987562189054726147, 0.5000000000000000000, 0.5012437810945273853, 0.5024875621890547706, 0.5037313432835820448, 0.5049751243781094301, 0.5062189054726368154, 0.5074626865671642006, 0.5087064676616915859, 0.5099502487562188602, 0.5111940298507462455, 0.5124378109452736307, 0.5136815920398010160, 0.5149253731343284013, 0.5161691542288556755, 0.5174129353233830608, 0.5186567164179104461, 0.5199004975124378314, 0.5211442786069652167, 0.5223880597014924909, 0.5236318407960198762, 0.5248756218905472615, 0.5261194029850746468, 0.5273631840796020320, 0.5286069651741293063, 0.5298507462686566916, 0.5310945273631840768, 0.5323383084577114621, 0.5335820895522388474, 0.5348258706467661217, 0.5360696517412935069, 0.5373134328358208922, 0.5385572139303482775, 0.5398009950248756628, 0.5410447761194029370, 0.5422885572139303223, 0.5435323383084577076, 0.5447761194029850929, 0.5460199004975124781, 0.5472636815920397524, 0.5485074626865671377, 0.5497512437810945229, 0.5509950248756219082, 0.5522388059701492935, 0.5534825870646765678, 0.5547263681592039530, 0.5559701492537313383, 0.5572139303482587236, 0.5584577114427861089, 0.5597014925373133831, 0.5609452736318407684, 0.5621890547263681537, 0.5634328358208955390, 0.5646766169154229242, 0.5659203980099501985, 0.5671641791044775838, 0.5684079601990049690, 0.5696517412935323543, 0.5708955223880597396, 0.5721393034825870139, 0.5733830845771143991, 0.5746268656716417844, 0.5758706467661691697, 0.5771144278606965550, 0.5783582089552238292, 0.5796019900497512145, 0.5808457711442785998, 0.5820895522388059851, 0.5833333333333333703, 0.5845771144278606446, 0.5858208955223880299, 0.5870646766169154152, 0.5883084577114428004, 0.5895522388059701857, 0.5907960199004974600, 0.5920398009950248452, 0.5932835820895522305, 0.5945273631840796158, 0.5957711442786070011, 0.5970149253731342753, 0.5982587064676616606, 0.5995024875621890459, 0.6007462686567164312, 0.6019900497512438164, 0.6032338308457710907, 0.6044776119402984760, 0.6057213930348258613, 0.6069651741293532465, 0.6082089552238806318, 0.6094527363184079061, 0.6106965174129352913, 0.6119402985074626766, 0.6131840796019900619, 0.6144278606965174472, 0.6156716417910447214, 0.6169154228855721067, 0.6181592039800994920, 0.6194029850746268773, 0.6206467661691542625, 0.6218905472636815368, 0.6231343283582089221, 0.6243781094527363074, 0.6256218905472636926, 0.6268656716417910779, 0.6281094527363184632, 0.6293532338308457375, 0.6305970149253731227, 0.6318407960199005080, 0.6330845771144278933, 0.6343283582089552786, 0.6355721393034825528, 0.6368159203980099381, 0.6380597014925373234, 0.6393034825870647087, 0.6405472636815920939, 0.6417910447761193682, 0.6430348258706467535, 0.6442786069651741387, 0.6455223880597015240, 0.6467661691542289093, 0.6480099502487560725, 0.6492537313432835688, 0.6504975124378109541, 0.6517412935323383394, 0.6529850746268657247, 0.6542288557213929989, 0.6554726368159203842, 0.6567164179104477695, 0.6579601990049751548, 0.6592039800995025400, 0.6604477611940298143, 0.6616915422885571996, 0.6629353233830845848, 0.6641791044776119701, 0.6654228855721393554, 0.6666666666666666297, 0.6679104477611940149, 0.6691542288557214002, 0.6703980099502487855, 0.6716417910447761708, 0.6728855721393034450, 0.6741293532338308303, 0.6753731343283582156, 0.6766169154228856009, 0.6778606965174129861, 0.6791044776119402604, 0.6803482587064676457, 0.6815920398009950310, 0.6828358208955224162, 0.6840796019900498015, 0.6853233830845770758, 0.6865671641791044610, 0.6878109452736318463, 0.6890547263681592316, 0.6902985074626866169, 0.6915422885572138911, 0.6927860696517412764, 0.6940298507462686617, 0.6952736318407960470, 0.6965174129353234322, 0.6977611940298507065, 0.6990049751243780918, 0.7002487562189054771, 0.7014925373134328623, 0.7027363184079602476, 0.7039800995024875219, 0.7052238805970149071, 0.7064676616915422924, 0.7077114427860696777, 0.7089552238805970630, 0.7101990049751243372, 0.7114427860696517225, 0.7126865671641791078, 0.7139303482587064931, 0.7151741293532338783, 0.7164179104477611526, 0.7176616915422885379, 0.7189054726368159232, 0.7201492537313433084, 0.7213930348258706937, 0.7226368159203979680, 0.7238805970149253532, 0.7251243781094527385, 0.7263681592039801238, 0.7276119402985075091, 0.7288557213930347833, 0.7300995024875621686, 0.7313432835820895539, 0.7325870646766169392, 0.7338308457711443245, 0.7350746268656715987, 0.7363184079601989840, 0.7375621890547263693, 0.7388059701492537545, 0.7400497512437811398, 0.7412935323383084141, 0.7425373134328357994, 0.7437810945273631846, 0.7450248756218905699, 0.7462686567164179552, 0.7475124378109452294, 0.7487562189054726147, 0.7500000000000000000, 0.7512437810945273853, 0.7524875621890547706, 0.7537313432835820448, 0.7549751243781094301, 0.7562189054726368154, 0.7574626865671642006, 0.7587064676616915859, 0.7599502487562188602, 0.7611940298507462455, 0.7624378109452736307, 0.7636815920398010160, 0.7649253731343284013, 0.7661691542288556755, 0.7674129353233830608, 0.7686567164179104461, 0.7699004975124378314, 0.7711442786069652167, 0.7723880597014924909, 0.7736318407960198762, 0.7748756218905472615, 0.7761194029850746468, 0.7773631840796020320, 0.7786069651741293063, 0.7798507462686566916, 0.7810945273631840768, 0.7823383084577114621, 0.7835820895522388474, 0.7848258706467661217, 0.7860696517412935069, 0.7873134328358208922, 0.7885572139303482775, 0.7898009950248756628, 0.7910447761194029370, 0.7922885572139303223, 0.7935323383084577076, 0.7947761194029850929, 0.7960199004975124781, 0.7972636815920397524, 0.7985074626865671377, 0.7997512437810945229, 0.8009950248756219082, 0.8022388059701492935, 0.8034825870646765678, 0.8047263681592039530, 0.8059701492537313383, 0.8072139303482587236, 0.8084577114427861089, 0.8097014925373133831, 0.8109452736318407684, 0.8121890547263681537, 0.8134328358208955390, 0.8146766169154229242, 0.8159203980099501985, 0.8171641791044775838, 0.8184079601990049690, 0.8196517412935323543, 0.8208955223880597396, 0.8221393034825870139, 0.8233830845771143991, 0.8246268656716417844, 0.8258706467661691697, 0.8271144278606965550, 0.8283582089552238292, 0.8296019900497512145, 0.8308457711442785998, 0.8320895522388059851, 0.8333333333333332593, 0.8345771144278606446, 0.8358208955223880299, 0.8370646766169154152, 0.8383084577114428004, 0.8395522388059701857, 0.8407960199004974600, 0.8420398009950248452, 0.8432835820895522305, 0.8445273631840796158, 0.8457711442786070011, 0.8470149253731342753, 0.8482587064676616606, 0.8495024875621890459, 0.8507462686567164312, 0.8519900497512438164, 0.8532338308457710907, 0.8544776119402984760, 0.8557213930348258613, 0.8569651741293532465, 0.8582089552238806318, 0.8594527363184079061, 0.8606965174129352913, 0.8619402985074626766, 0.8631840796019900619, 0.8644278606965174472, 0.8656716417910447214, 0.8669154228855721067, 0.8681592039800994920, 0.8694029850746268773, 0.8706467661691542625, 0.8718905472636815368, 0.8731343283582089221, 0.8743781094527363074, 0.8756218905472636926, 0.8768656716417910779, 0.8781094527363184632, 0.8793532338308457375, 0.8805970149253731227, 0.8818407960199005080, 0.8830845771144278933, 0.8843283582089552786, 0.8855721393034825528, 0.8868159203980099381, 0.8880597014925373234, 0.8893034825870647087, 0.8905472636815920939, 0.8917910447761193682, 0.8930348258706467535, 0.8942786069651741387, 0.8955223880597015240, 0.8967661691542289093, 0.8980099502487561836, 0.8992537313432835688, 0.9004975124378109541, 0.9017412935323383394, 0.9029850746268657247, 0.9042288557213929989, 0.9054726368159203842, 0.9067164179104477695, 0.9079601990049751548, 0.9092039800995025400, 0.9104477611940298143, 0.9116915422885571996, 0.9129353233830845848, 0.9141791044776119701, 0.9154228855721393554, 0.9166666666666666297, 0.9179104477611940149, 0.9191542288557214002, 0.9203980099502487855, 0.9216417910447761708, 0.9228855721393034450, 0.9241293532338308303, 0.9253731343283582156, 0.9266169154228856009, 0.9278606965174129861, 0.9291044776119402604, 0.9303482587064676457, 0.9315920398009950310, 0.9328358208955224162, 0.9340796019900498015, 0.9353233830845770758, 0.9365671641791044610, 0.9378109452736318463, 0.9390547263681592316, 0.9402985074626866169, 0.9415422885572138911, 0.9427860696517412764, 0.9440298507462686617, 0.9452736318407960470, 0.9465174129353234322, 0.9477611940298507065, 0.9490049751243780918, 0.9502487562189054771, 0.9514925373134328623, 0.9527363184079602476, 0.9539800995024875219, 0.9552238805970149071, 0.9564676616915422924, 0.9577114427860696777, 0.9589552238805970630, 0.9601990049751243372, 0.9614427860696517225, 0.9626865671641791078, 0.9639303482587064931, 0.9651741293532338783, 0.9664179104477611526, 0.9676616915422885379, 0.9689054726368159232, 0.9701492537313433084, 0.9713930348258706937, 0.9726368159203979680, 0.9738805970149253532, 0.9751243781094527385, 0.9763681592039801238, 0.9776119402985075091, 0.9788557213930347833, 0.9800995024875621686, 0.9813432835820895539, 0.9825870646766169392, 0.9838308457711443245, 0.9850746268656715987, 0.9863184079601989840, 0.9875621890547263693, 0.9888059701492537545, 0.9900497512437811398, 0.9912935323383084141, 0.9925373134328357994, 0.9927075504029140296 ),
 .UNSPECIFIED. ) 
 CURVE ( )  GEOMETRIC_REPRESENTATION_ITEM ( )  RATIONAL_B_SPLINE_CURVE ( ( 1.000000000000000000, 0.8660254037844387076, 1.000000000000000000, 0.8660254037844387076, 1.000000000000000000, 0.8660254037844387076, 1.000000000000000000, 0.8660254037844387076, 1.000000000000000000, 0.8660254037844387076, 1.000000000000000000, 0.8660254037844387076, 1.000000000000000000, 0.8660254037844387076, 1.000000000000000000, 0.8660254037844387076, 1.000000000000000000, 0.8660254037844387076, 1.000000000000000000, 0.8660254037844387076, 1.000000000000000000, 0.8660254037844387076, 1.000000000000000000, 0.8660254037844387076, 1.000000000000000000, 0.8660254037844387076, 1.000000000000000000, 0.8660254037844387076, 1.000000000000000000, 0.8660254037844387076, 1.000000000000000000, 0.8660254037844387076, 1.000000000000000000, 0.8660254037844387076, 1.000000000000000000, 0.8660254037844387076, 1.000000000000000000, 0.8660254037844387076, 1.000000000000000000, 0.8660254037844387076, 1.000000000000000000, 0.8660254037844387076, 1.000000000000000000, 0.8660254037844387076, 1.000000000000000000, 0.8660254037844387076, 1.000000000000000000, 0.8660254037844387076, 1.000000000000000000, 0.8660254037844387076, 1.000000000000000000, 0.8660254037844387076, 1.000000000000000000, 0.8660254037844387076, 1.000000000000000000, 0.8660254037844387076, 1.000000000000000000, 0.8660254037844387076, 1.000000000000000000, 0.8660254037844387076, 1.000000000000000000, 0.8660254037844387076, 1.000000000000000000, 0.8660254037844387076, 1.000000000000000000, 0.8660254037844387076, 1.000000000000000000, 0.8660254037844387076, 1.000000000000000000, 0.8660254037844387076, 1.000000000000000000, 0.8660254037844387076, 1.000000000000000000, 0.8660254037844387076, 1.000000000000000000, 0.8660254037844387076, 1.000000000000000000, 0.8660254037844387076, 1.000000000000000000, 0.8660254037844387076, 1.000000000000000000, 0.8660254037844387076, 1.000000000000000000, 0.8660254037844387076, 1.000000000000000000, 0.8660254037844387076, 1.000000000000000000, 0.8660254037844387076, 1.000000000000000000, 0.8660254037844387076, 1.000000000000000000, 0.8660254037844387076, 1.000000000000000000, 0.8660254037844387076, 1.000000000000000000, 0.8660254037844387076, 1.000000000000000000, 0.8660254037844387076, 1.000000000000000000, 0.8660254037844387076, 1.000000000000000000, 0.8660254037844387076, 1.000000000000000000, 0.8660254037844387076, 1.000000000000000000, 0.8660254037844387076, 1.000000000000000000, 0.8660254037844387076, 1.000000000000000000, 0.8660254037844387076, 1.000000000000000000, 0.8660254037844387076, 1.000000000000000000, 0.8660254037844387076, 1.000000000000000000, 0.8660254037844387076, 1.000000000000000000, 0.8660254037844387076, 1.000000000000000000, 0.8660254037844387076, 1.000000000000000000, 0.8660254037844387076, 1.000000000000000000, 0.8660254037844387076, 1.000000000000000000, 0.8660254037844387076, 1.000000000000000000, 0.8660254037844387076, 1.000000000000000000, 0.8660254037844387076, 1.000000000000000000, 0.8660254037844387076, 1.000000000000000000, 0.8660254037844387076, 1.000000000000000000, 0.8660254037844387076, 1.000000000000000000, 0.8660254037844387076, 1.000000000000000000, 0.8660254037844387076, 1.000000000000000000, 0.8660254037844387076, 1.000000000000000000, 0.8660254037844387076, 1.000000000000000000, 0.8660254037844387076, 1.000000000000000000, 0.8660254037844387076, 1.000000000000000000, 0.8660254037844387076, 1.000000000000000000, 0.8660254037844387076, 1.000000000000000000, 0.8660254037844387076, 1.000000000000000000, 0.8660254037844387076, 1.000000000000000000, 0.8660254037844387076, 1.000000000000000000, 0.8660254037844387076, 1.000000000000000000, 0.8660254037844387076, 1.000000000000000000, 0.8660254037844387076, 1.000000000000000000, 0.8660254037844387076, 1.000000000000000000, 0.8660254037844387076, 1.000000000000000000, 0.8660254037844387076, 1.000000000000000000, 0.8660254037844387076, 1.000000000000000000, 0.8660254037844387076, 1.000000000000000000, 0.8660254037844387076, 1.000000000000000000, 0.8660254037844387076, 1.000000000000000000, 0.8660254037844387076, 1.000000000000000000, 0.8660254037844387076, 1.000000000000000000, 0.8660254037844387076, 1.000000000000000000, 0.8660254037844387076, 1.000000000000000000, 0.8660254037844387076, 1.000000000000000000, 0.8660254037844387076, 1.000000000000000000, 0.8660254037844387076, 1.000000000000000000, 0.8660254037844387076, 1.000000000000000000, 0.8660254037844387076, 1.000000000000000000, 0.8660254037844387076, 1.000000000000000000, 0.8660254037844387076, 1.000000000000000000, 0.8660254037844387076, 1.000000000000000000, 0.8660254037844387076, 1.000000000000000000, 0.8660254037844387076, 1.000000000000000000, 0.8660254037844387076, 1.000000000000000000, 0.8660254037844387076, 1.000000000000000000, 0.8660254037844387076, 1.000000000000000000, 0.8660254037844387076, 1.000000000000000000, 0.8660254037844387076, 1.000000000000000000, 0.8660254037844387076, 1.000000000000000000, 0.8660254037844387076, 1.000000000000000000, 0.8660254037844387076, 1.000000000000000000, 0.8660254037844387076, 1.000000000000000000, 0.8660254037844387076, 1.000000000000000000, 0.8660254037844387076, 1.000000000000000000, 0.8660254037844387076, 1.000000000000000000, 0.8660254037844387076, 1.000000000000000000, 0.8660254037844387076, 1.000000000000000000, 0.8660254037844387076, 1.000000000000000000, 0.8660254037844387076, 1.000000000000000000, 0.8660254037844387076, 1.000000000000000000, 0.8660254037844387076, 1.000000000000000000, 0.8660254037844387076, 1.000000000000000000, 0.8660254037844387076, 1.000000000000000000, 0.8660254037844387076, 1.000000000000000000, 0.8660254037844387076, 1.000000000000000000, 0.8660254037844387076, 1.000000000000000000, 0.8660254037844387076, 1.000000000000000000, 0.8660254037844387076, 1.000000000000000000, 0.8660254037844387076, 1.000000000000000000, 0.8660254037844387076, 1.000000000000000000, 0.8660254037844387076, 1.000000000000000000, 0.8660254037844387076, 1.000000000000000000, 0.8660254037844387076, 1.000000000000000000, 0.8660254037844387076, 1.000000000000000000, 0.8660254037844387076, 1.000000000000000000, 0.8660254037844387076, 1.000000000000000000, 0.8660254037844387076, 1.000000000000000000, 0.8660254037844387076, 1.000000000000000000, 0.8660254037844387076, 1.000000000000000000, 0.8660254037844387076, 1.000000000000000000, 0.8660254037844387076, 1.000000000000000000, 0.8660254037844387076, 1.000000000000000000, 0.8660254037844387076, 1.000000000000000000, 0.8660254037844387076, 1.000000000000000000, 0.8660254037844387076, 1.000000000000000000, 0.8660254037844387076, 1.000000000000000000, 0.8660254037844387076, 1.000000000000000000, 0.8660254037844387076, 1.000000000000000000, 0.8660254037844387076, 1.000000000000000000, 0.8660254037844387076, 1.000000000000000000, 0.8660254037844387076, 1.000000000000000000, 0.8660254037844387076, 1.000000000000000000, 0.8660254037844387076, 1.000000000000000000, 0.8660254037844387076, 1.000000000000000000, 0.8660254037844387076, 1.000000000000000000, 0.8660254037844387076, 1.000000000000000000, 0.8660254037844387076, 1.000000000000000000, 0.8660254037844387076, 1.000000000000000000, 0.8660254037844387076, 1.000000000000000000, 0.8660254037844387076, 1.000000000000000000, 0.8660254037844387076, 1.000000000000000000, 0.8660254037844387076, 1.000000000000000000, 0.8660254037844387076, 1.000000000000000000, 0.8660254037844387076, 1.000000000000000000, 0.8660254037844387076, 1.000000000000000000, 0.8660254037844387076, 1.000000000000000000, 0.8660254037844387076, 1.000000000000000000, 0.8660254037844387076, 1.000000000000000000, 0.8660254037844387076, 1.000000000000000000, 0.8660254037844387076, 1.000000000000000000, 0.8660254037844387076, 1.000000000000000000, 0.8660254037844387076, 1.000000000000000000, 0.8660254037844387076, 1.000000000000000000, 0.8660254037844387076, 1.000000000000000000, 0.8660254037844387076, 1.000000000000000000, 0.8660254037844387076, 1.000000000000000000, 0.8660254037844387076, 1.000000000000000000, 0.8660254037844387076, 1.000000000000000000, 0.8660254037844387076, 1.000000000000000000, 0.8660254037844387076, 1.000000000000000000, 0.8660254037844387076, 1.000000000000000000, 0.8660254037844387076, 1.000000000000000000, 0.8660254037844387076, 1.000000000000000000, 0.8660254037844387076, 1.000000000000000000, 0.8660254037844387076, 1.000000000000000000, 0.8660254037844387076, 1.000000000000000000, 0.8660254037844387076, 1.000000000000000000, 0.8660254037844387076, 1.000000000000000000, 0.8660254037844387076, 1.000000000000000000, 0.8660254037844387076, 1.000000000000000000, 0.8660254037844387076, 1.000000000000000000, 0.8660254037844387076, 1.000000000000000000, 0.8660254037844387076, 1.000000000000000000, 0.8660254037844387076, 1.000000000000000000, 0.8660254037844387076, 1.000000000000000000, 0.8660254037844387076, 1.000000000000000000, 0.8660254037844387076, 1.000000000000000000, 0.8660254037844387076, 1.000000000000000000, 0.8660254037844387076, 1.000000000000000000, 0.8660254037844387076, 1.000000000000000000, 0.8660254037844387076, 1.000000000000000000, 0.8660254037844387076, 1.000000000000000000, 0.8660254037844387076, 1.000000000000000000, 0.8660254037844387076, 1.000000000000000000, 0.8660254037844387076, 1.000000000000000000, 0.8660254037844387076, 1.000000000000000000, 0.8660254037844387076, 1.000000000000000000, 0.8660254037844387076, 1.000000000000000000, 0.8660254037844387076, 1.000000000000000000, 0.8660254037844387076, 1.000000000000000000, 0.8660254037844387076, 1.000000000000000000, 0.8660254037844387076, 1.000000000000000000, 0.8660254037844387076, 1.000000000000000000, 0.8660254037844387076, 1.000000000000000000, 0.8660254037844387076, 1.000000000000000000, 0.8660254037844387076, 1.000000000000000000, 0.8660254037844387076, 1.000000000000000000, 0.8660254037844387076, 1.000000000000000000, 0.8660254037844387076, 1.000000000000000000, 0.8660254037844387076, 1.000000000000000000, 0.8660254037844387076, 1.000000000000000000, 0.8660254037844387076, 1.000000000000000000, 0.8660254037844387076, 1.000000000000000000, 0.8660254037844387076, 1.000000000000000000, 0.8660254037844387076, 1.000000000000000000, 0.8660254037844387076, 1.000000000000000000, 0.8660254037844387076, 1.000000000000000000, 0.8660254037844387076, 1.000000000000000000, 0.8660254037844387076, 1.000000000000000000, 0.8660254037844387076, 1.000000000000000000, 0.8660254037844387076, 1.000000000000000000, 0.8660254037844387076, 1.000000000000000000, 0.8660254037844387076, 1.000000000000000000, 0.8660254037844387076, 1.000000000000000000, 0.8660254037844387076, 1.000000000000000000, 0.8660254037844387076, 1.000000000000000000, 0.8660254037844387076, 1.000000000000000000, 0.8660254037844387076, 1.000000000000000000, 0.8660254037844387076, 1.000000000000000000, 0.8660254037844387076, 1.000000000000000000, 0.8660254037844387076, 1.000000000000000000, 0.8660254037844387076, 1.000000000000000000, 0.8660254037844387076, 1.000000000000000000, 0.8660254037844387076, 1.000000000000000000, 0.8660254037844387076, 1.000000000000000000, 0.8660254037844387076, 1.000000000000000000, 0.8660254037844387076, 1.000000000000000000, 0.8660254037844387076, 1.000000000000000000, 0.8660254037844387076, 1.000000000000000000, 0.8660254037844387076, 1.000000000000000000, 0.8660254037844387076, 1.000000000000000000, 0.8660254037844387076, 1.000000000000000000, 0.8660254037844387076, 1.000000000000000000, 0.8660254037844387076, 1.000000000000000000, 0.8660254037844387076, 1.000000000000000000, 0.8660254037844387076, 1.000000000000000000, 0.8660254037844387076, 1.000000000000000000, 0.8660254037844387076, 1.000000000000000000, 0.8660254037844387076, 1.000000000000000000, 0.8660254037844387076, 1.000000000000000000, 0.8660254037844387076, 1.000000000000000000, 0.8660254037844387076, 1.000000000000000000, 0.8660254037844387076, 1.000000000000000000, 0.8660254037844387076, 1.000000000000000000, 0.8660254037844387076, 1.000000000000000000, 0.8660254037844387076, 1.000000000000000000, 0.8660254037844387076, 1.000000000000000000, 0.8660254037844387076, 1.000000000000000000, 0.8660254037844387076, 1.000000000000000000, 0.8660254037844387076, 1.000000000000000000, 0.8660254037844387076, 1.000000000000000000, 0.8660254037844387076, 1.000000000000000000, 0.8660254037844387076, 1.000000000000000000, 0.8660254037844387076, 1.000000000000000000, 0.8660254037844387076, 1.000000000000000000, 0.8660254037844387076, 1.000000000000000000, 0.8660254037844387076, 1.000000000000000000, 0.8660254037844387076, 1.000000000000000000, 0.8660254037844387076, 1.000000000000000000, 0.8660254037844387076, 1.000000000000000000, 0.8660254037844387076, 1.000000000000000000, 0.8660254037844387076, 1.000000000000000000, 0.8660254037844387076, 1.000000000000000000, 0.8660254037844387076, 1.000000000000000000, 0.8660254037844387076, 1.000000000000000000, 0.8660254037844387076, 1.000000000000000000, 0.8660254037844387076, 1.000000000000000000, 0.8660254037844387076, 1.000000000000000000, 0.8660254037844387076, 1.000000000000000000, 0.8660254037844387076, 1.000000000000000000, 0.8660254037844387076, 1.000000000000000000, 0.8660254037844387076, 1.000000000000000000, 0.8660254037844387076, 1.000000000000000000, 0.8660254037844387076, 1.000000000000000000, 0.8660254037844387076, 1.000000000000000000, 0.8660254037844387076, 1.000000000000000000, 0.8660254037844387076, 1.000000000000000000, 0.8660254037844387076, 1.000000000000000000, 0.8660254037844387076, 1.000000000000000000, 0.8660254037844387076, 1.000000000000000000, 0.8660254037844387076, 1.000000000000000000, 0.8660254037844387076, 1.000000000000000000, 0.8660254037844387076, 1.000000000000000000, 0.8660254037844387076, 1.000000000000000000, 0.8660254037844387076, 1.000000000000000000, 0.8660254037844387076, 1.000000000000000000, 0.8660254037844387076, 1.000000000000000000, 0.8660254037844387076, 1.000000000000000000, 0.8660254037844387076, 1.000000000000000000, 0.8660254037844387076, 1.000000000000000000, 0.8660254037844387076, 1.000000000000000000, 0.8660254037844387076, 1.000000000000000000, 0.8660254037844387076, 1.000000000000000000, 0.8660254037844387076, 1.000000000000000000, 0.8660254037844387076, 1.000000000000000000, 0.8660254037844387076, 1.000000000000000000, 0.8660254037844387076, 1.000000000000000000, 0.8660254037844387076, 1.000000000000000000, 0.8660254037844387076, 1.000000000000000000, 0.8660254037844387076, 1.000000000000000000, 0.8660254037844387076, 1.000000000000000000, 0.8660254037844387076, 1.000000000000000000, 0.8660254037844387076, 1.000000000000000000, 0.8660254037844387076, 1.000000000000000000, 0.8660254037844387076, 1.000000000000000000, 0.8660254037844387076, 1.000000000000000000, 0.8660254037844387076, 1.000000000000000000, 0.8660254037844387076, 1.000000000000000000, 0.8660254037844387076, 1.000000000000000000, 0.8660254037844387076, 1.000000000000000000, 0.8660254037844387076, 1.000000000000000000, 0.8660254037844387076, 1.000000000000000000, 0.8660254037844387076, 1.000000000000000000, 0.8660254037844387076, 1.000000000000000000, 0.8660254037844387076, 1.000000000000000000, 0.8660254037844387076, 1.000000000000000000, 0.8660254037844387076, 1.000000000000000000, 0.8660254037844387076, 1.000000000000000000, 0.8660254037844387076, 1.000000000000000000, 0.8660254037844387076, 1.000000000000000000, 0.8660254037844387076, 1.000000000000000000, 0.8660254037844387076, 1.000000000000000000, 0.8660254037844387076, 1.000000000000000000, 0.8660254037844387076, 1.000000000000000000, 0.8660254037844387076, 1.000000000000000000, 0.8660254037844387076, 1.000000000000000000, 0.8660254037844387076, 1.000000000000000000, 0.8660254037844387076, 1.000000000000000000, 0.8660254037844387076, 1.000000000000000000, 0.8660254037844387076, 1.000000000000000000, 0.8660254037844387076, 1.000000000000000000, 0.8660254037844387076, 1.000000000000000000, 0.8660254037844387076, 1.000000000000000000, 0.8660254037844387076, 1.000000000000000000, 0.8660254037844387076, 1.000000000000000000, 0.8660254037844387076, 1.000000000000000000, 0.8660254037844387076, 1.000000000000000000, 0.8660254037844387076, 1.000000000000000000, 0.8660254037844387076, 1.000000000000000000, 0.8660254037844387076, 1.000000000000000000, 0.8660254037844387076, 1.000000000000000000, 0.8660254037844387076, 1.000000000000000000, 0.8660254037844387076, 1.000000000000000000, 0.8660254037844387076, 1.000000000000000000, 0.8660254037844387076, 1.000000000000000000, 0.8660254037844387076, 1.000000000000000000, 0.8660254037844387076, 1.000000000000000000, 0.8660254037844387076, 1.000000000000000000, 0.8660254037844387076, 1.000000000000000000, 0.8660254037844387076, 1.000000000000000000, 0.8660254037844387076, 1.000000000000000000, 0.8660254037844387076, 1.000000000000000000, 0.8660254037844387076, 1.000000000000000000, 0.8660254037844387076, 1.000000000000000000, 0.8660254037844387076, 1.000000000000000000, 0.8660254037844387076, 1.000000000000000000, 0.8660254037844387076, 1.000000000000000000, 0.8660254037844387076, 1.000000000000000000, 0.8660254037844387076, 1.000000000000000000, 0.8660254037844387076, 1.000000000000000000, 0.8660254037844387076, 1.000000000000000000, 0.8660254037844387076, 1.000000000000000000, 0.8660254037844387076, 1.000000000000000000, 0.8660254037844387076, 1.000000000000000000, 0.8660254037844387076, 1.000000000000000000, 0.8660254037844387076, 1.000000000000000000, 0.8660254037844387076, 1.000000000000000000, 0.8660254037844387076, 1.000000000000000000, 0.8660254037844387076, 1.000000000000000000, 0.8660254037844387076, 1.000000000000000000, 0.8660254037844387076, 1.000000000000000000, 0.8660254037844387076, 1.000000000000000000, 0.8660254037844387076, 1.000000000000000000, 0.8660254037844387076, 1.000000000000000000, 0.8660254037844387076, 1.000000000000000000, 0.8660254037844387076, 1.000000000000000000, 0.8660254037844387076, 1.000000000000000000, 0.8660254037844387076, 1.000000000000000000, 0.8660254037844387076, 1.000000000000000000, 0.8660254037844387076, 1.000000000000000000, 0.8660254037844387076, 1.000000000000000000, 0.8660254037844387076, 1.000000000000000000, 0.8660254037844387076, 1.000000000000000000, 0.8660254037844387076, 1.000000000000000000, 0.8660254037844387076, 1.000000000000000000, 0.8660254037844387076, 1.000000000000000000, 0.8660254037844387076, 1.000000000000000000, 0.8660254037844387076, 1.000000000000000000, 0.8660254037844387076, 1.000000000000000000, 0.8660254037844387076, 1.000000000000000000, 0.8660254037844387076, 1.000000000000000000, 0.8660254037844387076, 1.000000000000000000, 0.8660254037844387076, 1.000000000000000000, 0.8660254037844387076, 1.000000000000000000, 0.8660254037844387076, 1.000000000000000000, 0.8660254037844387076, 1.000000000000000000, 0.8660254037844387076, 1.000000000000000000, 0.8660254037844387076, 1.000000000000000000, 0.8660254037844387076, 1.000000000000000000, 0.8660254037844387076, 1.000000000000000000, 0.8660254037844387076, 1.000000000000000000, 0.8660254037844387076, 1.000000000000000000, 0.8660254037844387076, 1.000000000000000000, 0.8660254037844387076, 1.000000000000000000, 0.8660254037844387076, 1.000000000000000000, 0.8660254037844387076, 1.000000000000000000, 0.8660254037844387076, 1.000000000000000000, 0.8660254037844387076, 1.000000000000000000, 0.8660254037844387076, 1.000000000000000000, 0.8660254037844387076, 1.000000000000000000, 0.8660254037844387076, 1.000000000000000000, 0.8660254037844387076, 1.000000000000000000, 0.8660254037844387076, 1.000000000000000000, 0.8660254037844387076, 1.000000000000000000, 0.8660254037844387076, 1.000000000000000000, 0.8660254037844387076, 1.000000000000000000, 0.8660254037844387076, 1.000000000000000000, 0.8660254037844387076, 1.000000000000000000, 0.8660254037844387076, 1.000000000000000000, 0.8660254037844387076, 1.000000000000000000, 0.8660254037844387076, 1.000000000000000000, 0.8660254037844387076, 1.000000000000000000, 0.8660254037844387076, 1.000000000000000000, 0.8660254037844387076, 1.000000000000000000, 0.8660254037844387076, 1.000000000000000000, 0.8660254037844387076, 1.000000000000000000, 0.8660254037844387076, 1.000000000000000000, 0.8660254037844387076, 1.000000000000000000, 0.8660254037844387076, 1.000000000000000000, 0.8660254037844387076, 1.000000000000000000, 0.8660254037844387076, 1.000000000000000000, 0.8660254037844387076, 1.000000000000000000, 0.8660254037844387076, 1.000000000000000000, 0.8660254037844387076, 1.000000000000000000, 0.8660254037844387076, 1.000000000000000000, 0.8660254037844387076, 1.000000000000000000, 0.8660254037844387076, 1.000000000000000000, 0.8660254037844387076, 1.000000000000000000, 0.8660254037844387076, 1.000000000000000000, 0.8660254037844387076, 1.000000000000000000, 0.8660254037844387076, 1.000000000000000000, 0.8660254037844387076, 1.000000000000000000, 0.8660254037844387076, 1.000000000000000000, 0.8660254037844387076, 1.000000000000000000, 0.8660254037844387076, 1.000000000000000000, 0.8660254037844387076, 1.000000000000000000, 0.8660254037844387076, 1.000000000000000000, 0.8660254037844387076, 1.000000000000000000, 0.8660254037844387076, 1.000000000000000000, 0.8660254037844387076, 1.000000000000000000, 0.8660254037844387076, 1.000000000000000000, 0.8660254037844387076, 1.000000000000000000, 0.8660254037844387076, 1.000000000000000000, 0.8660254037844387076, 1.000000000000000000, 0.8660254037844387076, 1.000000000000000000, 0.8660254037844387076, 1.000000000000000000, 0.8660254037844387076, 1.000000000000000000, 0.8660254037844387076, 1.000000000000000000, 0.8660254037844387076, 1.000000000000000000, 0.8660254037844387076, 1.000000000000000000, 0.8660254037844387076, 1.000000000000000000, 0.8660254037844387076, 1.000000000000000000, 0.8660254037844387076, 1.000000000000000000, 0.8660254037844387076, 1.000000000000000000, 0.8660254037844387076, 1.000000000000000000, 0.8660254037844387076, 1.000000000000000000, 0.8660254037844387076, 1.000000000000000000, 0.8660254037844387076, 1.000000000000000000, 0.8660254037844387076, 1.000000000000000000, 0.8660254037844387076, 1.000000000000000000, 0.8660254037844387076, 1.000000000000000000, 0.8660254037844387076, 1.000000000000000000, 0.8660254037844387076, 1.000000000000000000, 0.8660254037844387076, 1.000000000000000000, 0.8660254037844387076, 1.000000000000000000, 0.8660254037844387076, 1.000000000000000000, 0.8660254037844387076, 1.000000000000000000, 0.8660254037844387076, 1.000000000000000000, 0.8660254037844387076, 1.000000000000000000, 0.8660254037844387076, 1.000000000000000000, 0.8660254037844387076, 1.000000000000000000, 0.8660254037844387076, 1.000000000000000000, 0.8660254037844387076, 1.000000000000000000, 0.8660254037844387076, 1.000000000000000000, 0.8660254037844387076, 1.000000000000000000, 0.8660254037844387076, 1.000000000000000000, 0.8660254037844387076, 1.000000000000000000, 0.8660254037844387076, 1.000000000000000000, 0.8660254037844387076, 1.000000000000000000, 0.8660254037844387076, 1.000000000000000000, 0.8660254037844387076, 1.000000000000000000, 0.8660254037844387076, 1.000000000000000000, 0.8660254037844387076, 1.000000000000000000, 0.8660254037844387076, 1.000000000000000000, 0.8660254037844387076, 1.000000000000000000, 0.8660254037844387076, 1.000000000000000000, 0.8660254037844387076, 1.000000000000000000, 0.8660254037844387076, 1.000000000000000000, 0.8660254037844387076, 1.000000000000000000, 0.8660254037844387076, 1.000000000000000000, 0.8660254037844387076, 1.000000000000000000, 0.8660254037844387076, 1.000000000000000000, 0.8660254037844387076, 1.000000000000000000, 0.8660254037844387076, 1.000000000000000000, 0.8660254037844387076, 1.000000000000000000, 0.8660254037844387076, 1.000000000000000000, 0.8660254037844387076, 1.000000000000000000, 0.8660254037844387076, 1.000000000000000000, 0.8660254037844387076, 1.000000000000000000, 0.8660254037844387076, 1.000000000000000000, 0.8660254037844387076, 1.000000000000000000, 0.8660254037844387076, 1.000000000000000000, 0.8660254037844387076, 1.000000000000000000, 0.8660254037844387076, 1.000000000000000000, 0.8660254037844387076, 1.000000000000000000, 0.8660254037844387076, 1.000000000000000000, 0.8660254037844387076, 1.000000000000000000, 0.8660254037844387076, 1.000000000000000000, 0.8660254037844387076, 1.000000000000000000, 0.8660254037844387076, 1.000000000000000000, 0.8660254037844387076, 1.000000000000000000, 0.8660254037844387076, 1.000000000000000000, 0.8660254037844387076, 1.000000000000000000, 0.8660254037844387076, 1.000000000000000000, 0.8660254037844387076, 1.000000000000000000, 0.8660254037844387076, 1.000000000000000000, 0.8660254037844387076, 1.000000000000000000, 0.8660254037844387076, 1.000000000000000000, 0.8660254037844387076, 1.000000000000000000, 0.8660254037844387076, 1.000000000000000000, 0.8660254037844387076, 1.000000000000000000, 0.8660254037844387076, 1.000000000000000000, 0.8660254037844387076, 1.000000000000000000, 0.8660254037844387076, 1.000000000000000000, 0.8660254037844387076, 1.000000000000000000, 0.8660254037844387076, 1.000000000000000000, 0.8660254037844387076, 1.000000000000000000, 0.8660254037844387076, 1.000000000000000000, 0.8660254037844387076, 1.000000000000000000, 0.8660254037844387076, 1.000000000000000000, 0.8660254037844387076, 1.000000000000000000, 0.8660254037844387076, 1.000000000000000000, 0.8660254037844387076, 1.000000000000000000, 0.8660254037844387076, 1.000000000000000000, 0.8660254037844387076, 1.000000000000000000, 0.8660254037844387076, 1.000000000000000000, 0.8660254037844387076, 1.000000000000000000, 0.8660254037844387076, 1.000000000000000000, 0.8660254037844387076, 1.000000000000000000, 0.8660254037844387076, 1.000000000000000000, 0.8660254037844387076, 1.000000000000000000, 0.8660254037844387076, 1.000000000000000000, 0.8660254037844387076, 1.000000000000000000, 0.8660254037844387076, 1.000000000000000000, 0.8660254037844387076, 1.000000000000000000, 0.8660254037844387076, 1.000000000000000000, 0.8660254037844387076, 1.000000000000000000, 0.8660254037844387076, 1.000000000000000000, 0.8660254037844387076, 1.000000000000000000, 0.8660254037844387076, 1.000000000000000000, 0.8660254037844387076, 1.000000000000000000, 0.8660254037844387076, 1.000000000000000000, 0.8660254037844387076, 1.000000000000000000, 0.8660254037844387076, 1.000000000000000000, 0.8660254037844387076, 1.000000000000000000, 0.8660254037844387076, 1.000000000000000000, 0.8660254037844387076, 1.000000000000000000, 0.8660254037844387076, 1.000000000000000000, 0.8660254037844387076, 1.000000000000000000, 0.8660254037844387076, 1.000000000000000000, 0.8660254037844387076, 1.000000000000000000, 0.8660254037844387076, 1.000000000000000000, 0.8660254037844387076, 1.000000000000000000, 0.8660254037844387076, 1.000000000000000000, 0.8660254037844387076, 1.000000000000000000, 0.8660254037844387076, 1.000000000000000000, 0.8660254037844387076, 1.000000000000000000, 0.8660254037844387076, 1.000000000000000000, 0.8660254037844387076, 1.000000000000000000, 0.8660254037844387076, 1.000000000000000000, 0.8660254037844387076, 1.000000000000000000, 0.8660254037844387076, 1.000000000000000000, 0.8660254037844387076, 1.000000000000000000, 0.8660254037844387076, 1.000000000000000000, 0.8660254037844387076, 1.000000000000000000, 0.8660254037844387076, 1.000000000000000000, 0.8660254037844387076, 1.000000000000000000, 0.8660254037844387076, 1.000000000000000000, 0.8660254037844387076, 1.000000000000000000, 0.8660254037844387076, 1.000000000000000000, 0.8660254037844387076, 1.000000000000000000, 0.8660254037844387076, 1.000000000000000000, 0.8660254037844387076, 1.000000000000000000, 0.8660254037844387076, 1.000000000000000000, 0.8660254037844387076, 1.000000000000000000, 0.8660254037844387076, 1.000000000000000000, 0.8660254037844387076, 1.000000000000000000, 0.8660254037844387076, 1.000000000000000000, 0.8660254037844387076, 1.000000000000000000, 0.8660254037844387076, 1.000000000000000000, 0.8660254037844387076, 1.000000000000000000, 0.8660254037844387076, 1.000000000000000000, 0.8660254037844387076, 1.000000000000000000, 0.8660254037844387076, 1.000000000000000000, 0.8660254037844387076, 1.000000000000000000, 0.8660254037844387076, 1.000000000000000000, 0.8660254037844387076, 1.000000000000000000, 0.8660254037844387076, 1.000000000000000000, 0.8660254037844387076, 1.000000000000000000, 0.8660254037844387076, 1.000000000000000000, 0.8660254037844387076, 1.000000000000000000, 0.8660254037844387076, 1.000000000000000000, 0.8660254037844387076, 1.000000000000000000, 0.8660254037844387076, 1.000000000000000000, 0.8660254037844387076, 1.000000000000000000, 0.8660254037844387076, 1.000000000000000000, 0.8660254037844387076, 1.000000000000000000, 0.8660254037844387076, 1.000000000000000000, 0.8660254037844387076, 1.000000000000000000, 0.8660254037844387076, 1.000000000000000000, 0.8660254037844387076, 1.000000000000000000, 0.8660254037844387076, 1.000000000000000000, 0.8660254037844387076, 1.000000000000000000, 0.8660254037844387076, 1.000000000000000000, 0.8660254037844387076, 1.000000000000000000, 0.8660254037844387076, 1.000000000000000000, 0.8660254037844387076, 1.000000000000000000, 0.8660254037844387076, 1.000000000000000000, 0.8660254037844387076, 1.000000000000000000, 0.8660254037844387076, 1.000000000000000000, 0.8660254037844387076, 1.000000000000000000, 0.8660254037844387076, 1.000000000000000000, 0.8660254037844387076, 1.000000000000000000, 0.8660254037844387076, 1.000000000000000000, 0.8660254037844387076, 1.000000000000000000, 0.8660254037844387076, 1.000000000000000000, 0.8660254037844387076, 1.000000000000000000, 0.8660254037844387076, 1.000000000000000000, 0.8660254037844387076, 1.000000000000000000, 0.8660254037844387076, 1.000000000000000000, 0.8660254037844387076, 1.000000000000000000, 0.8660254037844387076, 1.000000000000000000, 0.8660254037844387076, 1.000000000000000000, 0.8660254037844387076, 1.000000000000000000, 0.8660254037844387076, 1.000000000000000000, 0.8660254037844387076, 1.000000000000000000, 0.8660254037844387076, 1.000000000000000000, 0.8660254037844387076, 1.000000000000000000, 0.8660254037844387076, 1.000000000000000000, 0.8660254037844387076, 1.000000000000000000, 0.8660254037844387076, 1.000000000000000000, 0.8660254037844387076, 1.000000000000000000, 0.8660254037844387076, 1.000000000000000000, 0.8660254037844387076, 1.000000000000000000, 0.8660254037844387076, 1.000000000000000000, 0.8660254037844387076, 1.000000000000000000, 0.8660254037844387076, 1.000000000000000000, 0.8660254037844387076, 1.000000000000000000, 0.8660254037844387076, 1.000000000000000000, 0.8660254037844387076, 1.000000000000000000, 0.8660254037844387076, 1.000000000000000000, 0.8660254037844387076, 1.000000000000000000, 0.8660254037844387076, 1.000000000000000000, 0.8660254037844387076, 1.000000000000000000, 0.8660254037844387076, 1.000000000000000000, 0.8660254037844387076, 1.000000000000000000, 0.8660254037844387076, 1.000000000000000000, 0.8660254037844387076, 1.000000000000000000, 0.8660254037844387076, 1.000000000000000000, 0.8660254037844387076, 1.000000000000000000, 0.8660254037844387076, 1.000000000000000000, 0.8660254037844387076, 1.000000000000000000, 0.8660254037844387076, 1.000000000000000000, 0.8660254037844387076, 1.000000000000000000, 0.8660254037844387076, 1.000000000000000000, 0.8660254037844387076, 1.000000000000000000, 0.8660254037844387076, 1.000000000000000000, 0.8660254037844387076, 1.000000000000000000, 0.8660254037844387076, 1.000000000000000000, 0.8660254037844387076, 1.000000000000000000, 0.8660254037844387076, 1.000000000000000000, 0.8660254037844387076, 1.000000000000000000, 0.8660254037844387076, 1.000000000000000000, 0.8660254037844387076, 1.000000000000000000, 0.8660254037844387076, 1.000000000000000000, 0.8660254037844387076, 1.000000000000000000, 0.8660254037844387076, 1.000000000000000000, 0.8660254037844387076, 1.000000000000000000, 0.8660254037844387076, 1.000000000000000000, 0.8660254037844387076, 1.000000000000000000, 0.8660254037844387076, 1.000000000000000000, 0.8660254037844387076, 1.000000000000000000, 0.8660254037844387076, 1.000000000000000000, 0.8660254037844387076, 1.000000000000000000, 0.8660254037844387076, 1.000000000000000000, 0.8660254037844387076, 1.000000000000000000, 0.8660254037844387076, 1.000000000000000000, 0.8660254037844387076, 1.000000000000000000, 0.8660254037844387076, 1.000000000000000000, 0.8660254037844387076, 1.000000000000000000, 0.8660254037844387076, 1.000000000000000000, 0.8660254037844387076, 1.000000000000000000, 0.8660254037844387076, 1.000000000000000000, 0.8660254037844387076, 1.000000000000000000, 0.8660254037844387076, 1.000000000000000000, 0.8660254037844387076, 1.000000000000000000, 0.8660254037844387076, 1.000000000000000000, 0.8660254037844387076, 1.000000000000000000, 0.8660254037844387076, 1.000000000000000000, 0.8660254037844387076, 1.000000000000000000, 0.8660254037844387076, 1.000000000000000000, 0.8660254037844387076, 1.000000000000000000, 0.8660254037844387076, 1.000000000000000000, 0.8660254037844387076, 1.000000000000000000, 0.8660254037844387076, 1.000000000000000000, 0.8660254037844387076, 1.000000000000000000, 0.8660254037844387076, 1.000000000000000000, 0.8660254037844387076, 1.000000000000000000, 0.8660254037844387076, 1.000000000000000000, 0.8660254037844387076, 1.000000000000000000, 0.8660254037844387076, 1.000000000000000000, 0.8660254037844387076, 1.000000000000000000, 0.8660254037844387076, 1.000000000000000000, 0.8660254037844387076, 1.000000000000000000, 0.8660254037844387076, 1.000000000000000000, 0.8660254037844387076, 1.000000000000000000, 0.8660254037844387076, 1.000000000000000000, 0.8660254037844387076, 1.000000000000000000, 0.8660254037844387076, 1.000000000000000000, 0.8660254037844387076, 1.000000000000000000, 0.8660254037844387076, 1.000000000000000000, 0.8660254037844387076, 1.000000000000000000, 0.8660254037844387076, 1.000000000000000000, 0.8660254037844387076, 1.000000000000000000, 0.8660254037844387076, 1.000000000000000000, 0.8660254037844387076, 1.000000000000000000, 0.8660254037844387076, 1.000000000000000000, 0.8660254037844387076, 1.000000000000000000, 0.8660254037844387076, 1.000000000000000000, 0.8660254037844387076, 1.000000000000000000, 0.8660254037844387076, 1.000000000000000000, 0.8660254037844387076, 1.000000000000000000, 0.8660254037844387076, 1.000000000000000000, 0.8660254037844387076, 1.000000000000000000, 0.8660254037844387076, 1.000000000000000000, 0.8660254037844387076, 1.000000000000000000, 0.8660254037844387076, 1.000000000000000000, 0.8660254037844387076, 1.000000000000000000, 0.8660254037844387076, 1.000000000000000000, 0.8660254037844387076, 1.000000000000000000, 0.8660254037844387076, 1.000000000000000000, 0.8660254037844387076, 1.000000000000000000, 0.8660254037844387076, 1.000000000000000000, 0.8660254037844387076, 1.000000000000000000, 0.8660254037844387076, 1.000000000000000000, 0.8660254037844387076, 1.000000000000000000, 0.8660254037844387076, 1.000000000000000000, 0.8660254037844387076, 1.000000000000000000, 0.8660254037844387076, 1.000000000000000000, 0.8660254037844387076, 1.000000000000000000, 0.8660254037844387076, 1.000000000000000000, 0.8660254037844387076, 1.000000000000000000, 0.8660254037844387076, 1.000000000000000000, 0.8660254037844387076, 1.000000000000000000, 0.8660254037844387076, 1.000000000000000000, 0.8660254037844387076, 1.000000000000000000, 0.8660254037844387076, 1.000000000000000000, 0.8660254037844387076, 1.000000000000000000, 0.8660254037844387076, 1.000000000000000000, 0.8660254037844387076, 1.000000000000000000, 0.8660254037844387076, 1.000000000000000000, 0.8660254037844387076, 1.000000000000000000, 0.8660254037844387076, 1.000000000000000000, 0.8660254037844387076, 1.000000000000000000, 0.8660254037844387076, 1.000000000000000000, 0.8660254037844387076, 1.000000000000000000, 0.8660254037844387076, 1.000000000000000000, 0.8660254037844387076, 1.000000000000000000, 0.9816628268209384167, 0.9683452906431763152 ) ) 
 REPRESENTATION_ITEM ( '' )  );
#7619=ADVANCED_FACE ( 'NONE', ( #11128 ), #27553, .T. ) ;
#7620=CARTESIAN_POINT ( 'NONE',  ( -10.81189881249999729, 6.242252689847871849, -149.4062500020484094 ) ) ;
#7621=CARTESIAN_POINT ( 'NONE',  ( -5.405949406249996869, 9.363379034771805109, -135.8437500020484094 ) ) ;
#7622=CARTESIAN_POINT ( 'NONE',  ( 9.999999999999998224, 0.000000000000000000, -104.3750000040967763 ) ) ;
#7623=VERTEX_POINT ( 'NONE', #806 ) ;
#7625=EDGE_LOOP ( 'NONE', ( #39994, #19293, #21103, #27263 ) ) ;
#7626=ORIENTED_EDGE ( 'NONE', *, *, #4173, .F. ) ;
#7627=CARTESIAN_POINT ( 'NONE',  ( -10.81189881249999729, 1.324075727343319199E-15, -111.5937500020483810 ) ) ;
#7630=CARTESIAN_POINT ( 'NONE',  ( 7.070501591499376803E-16, 11.54700538379251284, -129.5000000040967905 ) ) ;
#7631=CARTESIAN_POINT ( 'NONE',  ( 10.81189881249999907, 6.242252689847868297, -188.7187500020484094 ) ) ;
#7633=CARTESIAN_POINT ( 'NONE',  ( -10.81189881249999729, 6.242252689847871849, -39.71875000204835970 ) ) ;
#7634=CARTESIAN_POINT ( 'NONE',  ( -5.941590193206447879, -8.275517156161180665, 5.985441654281309245E-15 ) ) ;
#7636=AXIS2_PLACEMENT_3D ( 'NONE', #30722, #27252, #37398 ) ;
#7637=CARTESIAN_POINT ( 'NONE',  ( -10.81189881249999729, -6.242252689847864744, -174.4687500020483526 ) ) ;
#7638=CARTESIAN_POINT ( 'NONE',  ( -10.81189881249999729, 6.242252689847871849, -164.2187500020483810 ) ) ;
#7639=CARTESIAN_POINT ( 'NONE',  ( 10.00000000000051159, -5.773502691895965988, -76.00000000409676204 ) ) ;
#7642=CARTESIAN_POINT ( 'NONE',  ( -5.000000000000003553, -8.660254037844383745, -93.99999999999998579 ) ) ;
#7643=CARTESIAN_POINT ( 'NONE',  ( 7.070501591499376803E-16, 11.54700538379251284, -66.50000000409676204 ) ) ;
#7645=CARTESIAN_POINT ( 'NONE',  ( -10.81189881249999729, 6.242252689847871849, -90.71875000204838102 ) ) ;
#7647=CARTESIAN_POINT ( 'NONE',  ( -10.81189881249999729, 1.324075727343319199E-15, -56.28125000204836681 ) ) ;
#7650=CARTESIAN_POINT ( 'NONE',  ( -10.81189881249999729, 6.242252689847871849, -123.9062500020483952 ) ) ;
#7651=CARTESIAN_POINT ( 'NONE',  ( -10.81189881249999729, -6.242252689847864744, -158.1562500020484094 ) ) ;
#7654=CARTESIAN_POINT ( 'NONE',  ( -2.121150477449813534E-15, -11.54700538379251284, -128.7500000040967620 ) ) ;
#7656=VERTEX_POINT ( 'NONE', #4455 ) ;
#7660=CARTESIAN_POINT ( 'NONE',  ( -5.405949406250003975, -9.363379034771801557, -192.5312500020484094 ) ) ;
#7662=CARTESIAN_POINT ( 'NONE',  ( -4.999999999999996447, 8.660254037844387298, -50.99999999999996447 ) ) ;
#7664=CARTESIAN_POINT ( 'NONE',  ( 7.070501591499377789E-16, 11.54700538379251284, -60.50000000409677625 ) ) ;
#7665=CARTESIAN_POINT ( 'NONE',  ( -10.00000000000025580, 5.773502691896109873, -152.8750000000000000 ) ) ;
#7668=CARTESIAN_POINT ( 'NONE',  ( -10.81189881249999729, 6.242252689847871849, -48.90625000204837391 ) ) ;
#7672=CARTESIAN_POINT ( 'NONE',  ( 0.000000000000000000, 0.000000000000000000, -200.0000000000000000 ) ) ;
#7673=CARTESIAN_POINT ( 'NONE',  ( 7.644554776091147741E-16, 12.48450537969573659, -178.1562500020484094 ) ) ;
#7680=CARTESIAN_POINT ( 'NONE',  ( 10.00000000000025402, -5.773502691896113426, -163.0000000040967905 ) ) ;
#7681=CARTESIAN_POINT ( 'NONE',  ( -10.81189881249999729, 6.242252689847871849, -87.90625000204838102 ) ) ;
#7682=VERTEX_POINT ( 'NONE', #14356 ) ;
#7683=CARTESIAN_POINT ( 'NONE',  ( 7.070501591499376803E-16, 11.54700538379251284, -92.00000000409677625 ) ) ;
#7684=EDGE_LOOP ( 'NONE', ( #33652, #17316, #37883, #3215 ) ) ;
#7685=ORIENTED_EDGE ( 'NONE', *, *, #30937, .F. ) ;
#7686=CARTESIAN_POINT ( 'NONE',  ( 5.405949406249999534, 9.363379034771803333, -38.59375000204837391 ) ) ;
#7687=CARTESIAN_POINT ( 'NONE',  ( -2.293366432827344421E-15, -12.48450537969573659, -28.71875000204835615 ) ) ;
#7688=CARTESIAN_POINT ( 'NONE',  ( 10.81189881249999551, -6.242252689847874514, -15.15625000204837036 ) ) ;
#7689=CARTESIAN_POINT ( 'NONE',  ( 5.405949406249999534, 9.363379034771803333, -62.59375000204836681 ) ) ;
#7690=CARTESIAN_POINT ( 'NONE',  ( -4.999999999999996447, 8.660254037844387298, -163.8750000040967905 ) ) ;
#7693=CARTESIAN_POINT ( 'NONE',  ( -5.405949406250003975, -9.363379034771801557, -183.3437500020483810 ) ) ;
#7694=ADVANCED_FACE ( 'NONE', ( #31013 ), #4667, .T. ) ;
#7696=VECTOR ( 'NONE', #37669, 1000.000000000000000 ) ;
#7698=CARTESIAN_POINT ( 'NONE',  ( 0.000000000000000000, 0.000000000000000000, -200.0000000000000000 ) ) ;
#7699=DIRECTION ( 'NONE',  ( 1.000000000000000000, 0.000000000000000000, 0.000000000000000000 ) ) ;
#7701=DIRECTION ( 'NONE',  ( 1.000000000000000000, 0.000000000000000000, 0.000000000000000000 ) ) ;
#7704=CARTESIAN_POINT ( 'NONE',  ( 10.81189881249999907, 6.242252689847868297, -110.7187500020483810 ) ) ;
#7706=CARTESIAN_POINT ( 'NONE',  ( -10.81189881249999729, 6.242252689847871849, -93.90625000204839523 ) ) ;
#7707=CARTESIAN_POINT ( 'NONE',  ( -10.81189881249999729, 6.242252689847871849, -98.21875000204838102 ) ) ;
#7711=CARTESIAN_POINT ( 'NONE',  ( -5.000000000000003553, -8.660254037844383745, -157.3750000040967905 ) ) ;
#7715=VECTOR ( 'NONE', #28163, 1000.000000000000000 ) ;
#7719=CARTESIAN_POINT ( 'NONE',  ( -9.999999999999998224, 1.224646799147353059E-15, -18.12500000409675138 ) ) ;
#7720=CARTESIAN_POINT ( 'NONE',  ( -5.000000000000003553, -8.660254037844383745, -69.99999999999998579 ) ) ;
#7722=CARTESIAN_POINT ( 'NONE',  ( -2.121150477449813534E-15, -11.54700538379251284, -79.25000000409677625 ) ) ;
#7725=CARTESIAN_POINT ( 'NONE',  ( 10.81189881249999551, -6.242252689847874514, -81.15625000204842365 ) ) ;
#7729=CARTESIAN_POINT ( 'NONE',  ( 4.999999999999992006, -8.660254037844389075, -2.249999999999974243 ) ) ;
#7731=CARTESIAN_POINT ( 'NONE',  ( 10.81189881249999729, 0.000000000000000000, -11.84375000204834727 ) ) ;
#7732=CARTESIAN_POINT ( 'NONE',  ( 9.999999999999998224, 0.000000000000000000, -143.0000000000000000 ) ) ;
#7734=CARTESIAN_POINT ( 'NONE',  ( -10.81189881249999729, 1.324075727343319199E-15, -132.7812500020483810 ) ) ;
#7736=CARTESIAN_POINT ( 'NONE',  ( -10.00000000000000000, -5.773502691896251982, -179.6250000000000284 ) ) ;
#7737=DIRECTION ( 'NONE',  ( -0.000000000000000000, -0.000000000000000000, 1.000000000000000000 ) ) ;
#7738=CARTESIAN_POINT ( 'NONE',  ( -10.81189881249999907, -6.242252689847864744, -110.1562500020483952 ) ) ;
#7740=LINE ( 'NONE', #14395, #22093 ) ;
#7743=CARTESIAN_POINT ( 'NONE',  ( -5.405949406249996869, 9.363379034771805109, -34.03125000204837391 ) ) ;
#7745=VECTOR ( 'NONE', #37993, 1000.000000000000000 ) ;
#7746=CARTESIAN_POINT ( 'NONE',  ( 10.81189881249999907, 6.242252689847868297, -89.71875000204836681 ) ) ;
#7747=CARTESIAN_POINT ( 'NONE',  ( -9.999999999999998224, 1.224646799147353059E-15, -196.6250000040967905 ) ) ;
#7749=LINE ( 'NONE', #37305, #13506 ) ;
#7750=EDGE_CURVE ( 'NONE', #18023, #36127, #24362, .T. ) ;
#7751=( BOUNDED_CURVE ( )  B_SPLINE_CURVE ( 2, ( #20603, #17145, #20819, #10672, #27094, #34005, #30346 ),
 .UNSPECIFIED., .F., .F. ) 
 B_SPLINE_CURVE_WITH_KNOTS ( ( 3, 2, 2, 3 ),
 ( 0.1679104477611940427, 0.1691542288557214002, 0.1703980099502487855, 0.1716417910447761430 ),
 .UNSPECIFIED. ) 
 CURVE ( )  GEOMETRIC_REPRESENTATION_ITEM ( )  RATIONAL_B_SPLINE_CURVE ( ( 1.000000000000000000, 0.8660254037844387076, 1.000000000000000000, 0.8660254037844387076, 1.000000000000000000, 0.8660254037844357100, 1.000000000000003109 ) ) 
 REPRESENTATION_ITEM ( '' )  );
#7752=DIRECTION ( 'NONE',  ( -0.000000000000000000, -0.000000000000000000, 1.000000000000000000 ) ) ;
#7754=CARTESIAN_POINT ( 'NONE',  ( -9.999999999999998224, 1.224646799147353059E-15, -68.74999999999997158 ) ) ;
#7756=CARTESIAN_POINT ( 'NONE',  ( -5.405949406249996869, 9.363379034771805109, -126.8437500020483952 ) ) ;
#7759=CARTESIAN_POINT ( 'NONE',  ( -2.293366432827344421E-15, -12.48450537969573659, -3.406250002048348158 ) ) ;
#7762=CARTESIAN_POINT ( 'NONE',  ( -9.999999999999998224, 1.224646799147353059E-15, -174.1250000040968189 ) ) ;
#7764=CARTESIAN_POINT ( 'NONE',  ( 5.405949406249992428, -9.363379034771808662, -175.7812500020484094 ) ) ;
#7765=( BOUNDED_CURVE ( )  B_SPLINE_CURVE ( 2, ( #17153, #4863, #7462, #20612, #27744, #17795, #30354 ),
 .UNSPECIFIED., .F., .F. ) 
 B_SPLINE_CURVE_WITH_KNOTS ( ( 3, 2, 2, 3 ),
 ( 0.2537313432835822113, 0.2549751243781095411, 0.2562189054726369264, 0.2574626865671643117 ),
 .UNSPECIFIED. ) 
 CURVE ( )  GEOMETRIC_REPRESENTATION_ITEM ( )  RATIONAL_B_SPLINE_CURVE ( ( 0.9999999999999880096, 0.8660254037844506980, 1.000000000000000000, 0.8660254037844387076, 1.000000000000000000, 0.8660254037844267172, 1.000000000000011990 ) ) 
 REPRESENTATION_ITEM ( '' )  );
#7766=CARTESIAN_POINT ( 'NONE',  ( 0.000000000000000000, 0.000000000000000000, -200.0000000000000000 ) ) ;
#7769=CARTESIAN_POINT ( 'NONE',  ( 5.405949406249992428, -9.363379034771808662, -49.59375000204838102 ) ) ;
#7770=CARTESIAN_POINT ( 'NONE',  ( 5.405949406249992428, -9.363379034771808662, -42.09375000204837391 ) ) ;
#7772=CARTESIAN_POINT ( 'NONE',  ( 10.81189881249999729, 0.000000000000000000, -13.53125000204835615 ) ) ;
#7774=CARTESIAN_POINT ( 'NONE',  ( 9.999999999999479527, 5.773502691896553074, -145.8750000000000000 ) ) ;
#7776=CARTESIAN_POINT ( 'NONE',  ( -5.000000000000003553, -8.660254037844383745, -99.99999999999998579 ) ) ;
#7778=CARTESIAN_POINT ( 'NONE',  ( 9.999999999999998224, 0.000000000000000000, -114.8750000040967905 ) ) ;
#7779=CARTESIAN_POINT ( 'NONE',  ( -9.999999999999998224, 1.224646799147353059E-15, -200.0000000000000000 ) ) ;
#7782=CARTESIAN_POINT ( 'NONE',  ( -5.405949406250003975, -9.363379034771801557, -111.5312500020483810 ) ) ;
#7783=ORIENTED_EDGE ( 'NONE', *, *, #20719, .F. ) ;
#7784=CARTESIAN_POINT ( 'NONE',  ( -4.999999999999996447, 8.660254037844387298, -7.875000004096744277 ) ) ;
#7787=CARTESIAN_POINT ( 'NONE',  ( 10.81189881249999551, -6.242252689847874514, -163.6562500020484094 ) ) ;
#7789=ORIENTED_EDGE ( 'NONE', *, *, #18009, .T. ) ;
#7791=CARTESIAN_POINT ( 'NONE',  ( 10.00000000000000000, 5.773502691896255534, -25.87499999999997868 ) ) ;
#7792=VECTOR ( 'NONE', #10618, 1000.000000000000000 ) ;
#7793=CARTESIAN_POINT ( 'NONE',  ( 10.81189881249999729, 6.242252689847867408, -34.40625000204836681 ) ) ;
#7794=CARTESIAN_POINT ( 'NONE',  ( 9.999999999999998224, 0.000000000000000000, -162.5000000000000000 ) ) ;
#7795=CARTESIAN_POINT ( 'NONE',  ( 9.999999999999998224, 0.000000000000000000, -15.49999999999995737 ) ) ;
#7797=CARTESIAN_POINT ( 'NONE',  ( -10.81189881249999907, -6.242252689847864744, -132.6562500020484094 ) ) ;
#7798=CYLINDRICAL_SURFACE ( 'NONE', #6260, 9.999999999999998224 ) ;
#7799=EDGE_LOOP ( 'NONE', ( #37780, #20677, #30661, #7300, #35776, #18181, #41937, #19352, #1106, #29399, #32439, #4763, #37515, #3965, #13074, #2439, #32178, #36375, #31000, #3010, #32162, #163, #19144, #34293, #37175, #14888, #42162, #17994, #20998, #23861, #6678, #6153, #35070, #12238, #12337, #34612, #23298, #5037, #13222, #3359, #33995, #41267, #16394, #19508, #6294, #42646, #40139, #39293, #16889, #13127, #11810, #36399, #27479, #31700, #41294, #17776, #41043, #13178, #33283, #31224, #4169, #14815, #16345, #32634, #5888, #1105, #2606, #19147, #13914, #36451, #20889, #34109, #35146, #10906, #39338, #24239, #41648, #22929, #41351, #16186, #27364, #11848, #12338, #31867, #34851, #12759, #35983, #21908, #20838, #22233, #21047, #24370, #15603, #28448, #39933, #24635, #12396, #21527, #42195, #30460, #1589, #36298, #30147, #20513, #40671, #37121, #12495, #42119, #7367, #314, #28295, #1951, #14773, #2970, #22957, #19668, #3017, #2391, #38144, #20561, #30039, #1642, #22658, #2166, #11971, #24736, #24840, #11171, #24853, #10945, #16823, #3285, #794, #15399, #42378, #14123, #29501, #30253, #35251, #19880, #27054, #16792, #38285, #23240, #12235, #12951, #15826, #42357, #11652, #30144, #38471, #30978, #833, #12946, #21377, #11545, #40515, #19455, #22712, #9483, #17039, #38002, #21023, #7626, #33686, #24408, #22820, #167, #12755, #34494, #34343, #16022, #39418, #6506, #36456, #31588, #11308, #18296, #23814, #38158, #26535, #5038, #11919, #7877, #13599, #3427, #16673, #42643, #2505, #35672, #13437, #4233, #25223, #35089, #30520, #32097, #15730, #14221, #38637, #28915, #16144, #29696, #8012, #4019, #42406, #11327, #41042, #39887, #11214, #21260, #42488, #41028, #1323, #31862, #26733, #38368, #17739, #3853, #24990, #41744, #11381, #21092, #24672, #6390, #17530, #7993, #5761, #22339, #22544, #36700, #25728, #12964, #29758, #22362, #34131, #14124, #14265, #22024, #15263, #15621, #9168, #38526, #20675, #4656, #31417, #4587, #32594, #15649, #34446, #19507, #26206, #24621, #203, #4927, #6456, #42170, #34608, #11688, #3182, #28879, #22910, #33752, #20713, #5464, #26738, #9587, #21858, #26868, #34219, #12704 ) ) ;
#7800=ORIENTED_EDGE ( 'NONE', *, *, #22997, .T. ) ;
#7801=ORIENTED_EDGE ( 'NONE', *, *, #6146, .T. ) ;
#7803=CARTESIAN_POINT ( 'NONE',  ( 4.999999999999992006, -8.660254037844389075, -55.12500000409675494 ) ) ;
#7804=CARTESIAN_POINT ( 'NONE',  ( 10.81189881249999551, -6.242252689847874514, -163.4687500020483810 ) ) ;
#7806=CARTESIAN_POINT ( 'NONE',  ( -5.405949406250003975, -9.363379034771801557, -16.84375000204835260 ) ) ;
#7807=CARTESIAN_POINT ( 'NONE',  ( 0.000000000000000000, 0.000000000000000000, -200.0000000000000000 ) ) ;
#7808=CARTESIAN_POINT ( 'NONE',  ( 5.405949406249992428, -9.363379034771808662, -147.0937500020483810 ) ) ;
#7809=CARTESIAN_POINT ( 'NONE',  ( -10.81189881249999907, -6.242252689847864744, -139.9687500020483810 ) ) ;
#7810=CARTESIAN_POINT ( 'NONE',  ( -5.405949406250003975, -9.363379034771801557, -104.0312500020483810 ) ) ;
#7814=CARTESIAN_POINT ( 'NONE',  ( -5.405949406250003975, -9.363379034771801557, -10.84375000204834727 ) ) ;
#7820=EDGE_CURVE ( 'NONE', #437, #22340, #39210, .T. ) ;
#7821=CARTESIAN_POINT ( 'NONE',  ( -5.405949406249996869, 9.363379034771805109, -75.84375000204838102 ) ) ;
#7822=CARTESIAN_POINT ( 'NONE',  ( 10.81189881249999907, 6.242252689847868297, -65.71875000204836681 ) ) ;
#7823=LINE ( 'NONE', #24663, #40788 ) ;
#7824=CARTESIAN_POINT ( 'NONE',  ( 7.644554776091147741E-16, 12.48450537969573659, -34.15625000204836681 ) ) ;
#7828=CARTESIAN_POINT ( 'NONE',  ( -9.999999999999998224, 1.224646799147353059E-15, -119.7500000000000000 ) ) ;
#7829=CARTESIAN_POINT ( 'NONE',  ( -2.293366432827344421E-15, -12.48450537969573659, -129.4062500020483810 ) ) ;
#7830=CYLINDRICAL_SURFACE ( 'NONE', #31401, 9.999999999999998224 ) ;
#7832=CARTESIAN_POINT ( 'NONE',  ( 7.644554776091147741E-16, 12.48450537969573659, -14.65625000204836859 ) ) ;
#7833=ORIENTED_EDGE ( 'NONE', *, *, #2216, .T. ) ;
#7836=CARTESIAN_POINT ( 'NONE',  ( -2.121150477449813534E-15, -11.54700538379251284, -56.75000000409677625 ) ) ;
#7837=CARTESIAN_POINT ( 'NONE',  ( 10.00000000000000000, 5.773502691896255534, -32.25000000409675494 ) ) ;
#7838=( BOUNDED_CURVE ( )  B_SPLINE_CURVE ( 2, ( #7334, #17445, #33462, #14418, #14197, #30222, #40533 ),
 .UNSPECIFIED., .F., .F. ) 
 B_SPLINE_CURVE_WITH_KNOTS ( ( 3, 2, 2, 3 ),
 ( 0.4589552238805971740, 0.4601990049751245593, 0.4614427860696518890, 0.4626865671641792743 ),
 .UNSPECIFIED. ) 
 CURVE ( )  GEOMETRIC_REPRESENTATION_ITEM ( )  RATIONAL_B_SPLINE_CURVE ( ( 0.9999999999999820144, 0.8660254037844566932, 1.000000000000000000, 0.8660254037844387076, 1.000000000000000000, 0.8660254037844207220, 1.000000000000017986 ) ) 
 REPRESENTATION_ITEM ( '' )  );
#7839=CARTESIAN_POINT ( 'NONE',  ( 5.000000000000000000, 8.660254037844385522, -148.7500000000000000 ) ) ;
#7841=CARTESIAN_POINT ( 'NONE',  ( -5.000000000000003553, -8.660254037844383745, -40.37500000409677625 ) ) ;
#7842=CARTESIAN_POINT ( 'NONE',  ( 10.81189881249999907, 6.242252689847868297, -151.4062500020484094 ) ) ;
#7843=CARTESIAN_POINT ( 'NONE',  ( -10.81189881249999729, 6.242252689847871849, -126.7187500020483952 ) ) ;
#7845=ORIENTED_EDGE ( 'NONE', *, *, #35988, .F. ) ;
#7846=CARTESIAN_POINT ( 'NONE',  ( 7.070501591499376803E-16, 11.54700538379251284, -31.62499999999995737 ) ) ;
#7847=ORIENTED_EDGE ( 'NONE', *, *, #40405, .T. ) ;
#7849=CARTESIAN_POINT ( 'NONE',  ( 7.644554776091147741E-16, 12.48450537969573659, -111.9687500020483952 ) ) ;
#7850=ORIENTED_EDGE ( 'NONE', *, *, #11814, .T. ) ;
#7851=CARTESIAN_POINT ( 'NONE',  ( 9.999999999999998224, 0.000000000000000000, -41.37500000409677625 ) ) ;
#7852=CARTESIAN_POINT ( 'NONE',  ( 7.644554776091147741E-16, 12.48450537969573659, -186.9687500020483810 ) ) ;
#7853=CARTESIAN_POINT ( 'NONE',  ( -2.293366432827344421E-15, -12.48450537969573659, -40.71875000204835260 ) ) ;
#7855=CARTESIAN_POINT ( 'NONE',  ( 0.000000000000000000, 0.000000000000000000, -200.0000000000000000 ) ) ;
#7856=CARTESIAN_POINT ( 'NONE',  ( -10.81189881249999729, -6.242252689847864744, -175.9687500020483526 ) ) ;
#7857=CARTESIAN_POINT ( 'NONE',  ( 10.81189881249999551, -6.242252689847874514, -164.9687500020484094 ) ) ;
#7858=CARTESIAN_POINT ( 'NONE',  ( -5.000000000000003553, -8.660254037844383745, -25.37500000409675849 ) ) ;
#7862=CARTESIAN_POINT ( 'NONE',  ( 4.999999999999992006, -8.660254037844389075, -42.74999999999998579 ) ) ;
#7865=CARTESIAN_POINT ( 'NONE',  ( -5.405949406250003975, -9.363379034771801557, -85.84375000204836681 ) ) ;
#7867=CARTESIAN_POINT ( 'NONE',  ( -10.81189881249999729, 6.242252689847871849, -57.90625000204838813 ) ) ;
#7868=CARTESIAN_POINT ( 'NONE',  ( 9.999999999999998224, 0.000000000000000000, -87.87500000409677625 ) ) ;
#7870=CARTESIAN_POINT ( 'NONE',  ( -5.405949406249996869, 9.363379034771805109, -116.5312500020483952 ) ) ;
#7871=CARTESIAN_POINT ( 'NONE',  ( 10.81189881249999729, 6.242252689847867408, -154.4062500020483810 ) ) ;
#7874=CARTESIAN_POINT ( 'NONE',  ( 9.999999999999998224, 0.000000000000000000, -126.8750000040967905 ) ) ;
#7877=ORIENTED_EDGE ( 'NONE', *, *, #631, .F. ) ;
#7880=CARTESIAN_POINT ( 'NONE',  ( 10.81189881249999907, 6.242252689847868297, -178.4062500020484094 ) ) ;
#7881=VERTEX_POINT ( 'NONE', #28202 ) ;
#7882=CARTESIAN_POINT ( 'NONE',  ( -10.00000000000000000, -5.773502691896251982, -52.12499999999997158 ) ) ;
#7884=CARTESIAN_POINT ( 'NONE',  ( 10.00000000000000000, 5.773502691896255534, -56.25000000409676915 ) ) ;
#7885=DIRECTION ( 'NONE',  ( -0.000000000000000000, -0.000000000000000000, 1.000000000000000000 ) ) ;
#7886=CARTESIAN_POINT ( 'NONE',  ( 9.999999999999998224, 0.000000000000000000, -67.99999999999997158 ) ) ;
#7888=CARTESIAN_POINT ( 'NONE',  ( 5.405949406249999534, 9.363379034771803333, -47.78125000204838813 ) ) ;
#7892=CARTESIAN_POINT ( 'NONE',  ( 5.000000000000000000, 8.660254037844385522, -158.1250000040967905 ) ) ;
#7893=CARTESIAN_POINT ( 'NONE',  ( 10.81189881249999907, 6.242252689847868297, -178.4062500020484094 ) ) ;
#7895=CARTESIAN_POINT ( 'NONE',  ( -9.999999999998969713, -5.773502691896847949, -88.12499999999995737 ) ) ;
#7899=CARTESIAN_POINT ( 'NONE',  ( 7.644554776091147741E-16, 12.48450537969573659, -82.15625000204838102 ) ) ;
#7900=ORIENTED_EDGE ( 'NONE', *, *, #23193, .F. ) ;
#7905=CARTESIAN_POINT ( 'NONE',  ( 10.81189881249999729, 0.000000000000000000, -40.34375000204837391 ) ) ;
#7906=CARTESIAN_POINT ( 'NONE',  ( 7.644554776091147741E-16, 12.48450537969573659, -29.46875000204835970 ) ) ;
#7907=CARTESIAN_POINT ( 'NONE',  ( 10.81189881249999551, -6.242252689847874514, -12.15625000204835793 ) ) ;
#7908=CARTESIAN_POINT ( 'NONE',  ( 10.81189881249999729, 0.000000000000000000, -61.34375000204836681 ) ) ;
#7909=CARTESIAN_POINT ( 'NONE',  ( 9.999999999999479527, 5.773502691896553074, -93.37499999999997158 ) ) ;
#7910=EDGE_CURVE ( 'NONE', #8336, #28565, #2307, .T. ) ;
#7912=CARTESIAN_POINT ( 'NONE',  ( -5.405949406249996869, 9.363379034771805109, -185.3437500020483810 ) ) ;
#7915=CARTESIAN_POINT ( 'NONE',  ( 9.999999999999998224, 0.000000000000000000, -132.5000000000000000 ) ) ;
#7916=DIRECTION ( 'NONE',  ( -0.000000000000000000, -0.000000000000000000, 1.000000000000000000 ) ) ;
#7917=CARTESIAN_POINT ( 'NONE',  ( -5.000000000000003553, -8.660254037844383745, -104.4999999999999858 ) ) ;
#7918=CARTESIAN_POINT ( 'NONE',  ( -5.000000000000003553, -8.660254037844383745, -89.87500000409677625 ) ) ;
#7919=CARTESIAN_POINT ( 'NONE',  ( -5.405949406249996869, 9.363379034771805109, -111.8437500020483810 ) ) ;
#7920=CYLINDRICAL_SURFACE ( 'NONE', #30768, 9.999999999999998224 ) ;
#7921=CARTESIAN_POINT ( 'NONE',  ( -10.81189881249999907, -6.242252689847864744, -81.65625000204839523 ) ) ;
#7922=CARTESIAN_POINT ( 'NONE',  ( -5.405949406250003975, -9.363379034771801557, -100.8437500020483810 ) ) ;
#7925=CARTESIAN_POINT ( 'NONE',  ( -9.999999999999998224, 5.773502691896259087, -150.2500000040968189 ) ) ;
#7930=CARTESIAN_POINT ( 'NONE',  ( 9.999999999999998224, 0.000000000000000000, -182.0000000000000000 ) ) ;
#7933=CARTESIAN_POINT ( 'NONE',  ( -9.999999999999998224, 5.773502691896259087, -73.37499999999997158 ) ) ;
#7935=CARTESIAN_POINT ( 'NONE',  ( 10.00000000000000000, 5.773502691896255534, -84.75000000409677625 ) ) ;
#7936=CARTESIAN_POINT ( 'NONE',  ( -10.00000000000076916, 5.773502691895813221, -115.3749999999999716 ) ) ;
#7938=CARTESIAN_POINT ( 'NONE',  ( 10.81189881249999729, 0.000000000000000000, -79.53125000204838102 ) ) ;
#7941=ORIENTED_EDGE ( 'NONE', *, *, #24908, .T. ) ;
#7942=CARTESIAN_POINT ( 'NONE',  ( 7.070501591499377789E-16, 11.54700538379251284, -4.624999999999958256 ) ) ;
#7944=EDGE_CURVE ( 'NONE', #4606, #37408, #40570, .T. ) ;
#7945=CARTESIAN_POINT ( 'NONE',  ( -10.81189881249999729, 1.324075727343319199E-15, -12.59375000204834905 ) ) ;
#7946=CARTESIAN_POINT ( 'NONE',  ( 4.999999999999992006, -8.660254037844389075, -94.12500000409677625 ) ) ;
#7948=CARTESIAN_POINT ( 'NONE',  ( -10.81189881249999729, 1.324075727343319199E-15, -126.7812500020483668 ) ) ;
#7949=AXIS2_PLACEMENT_3D ( 'NONE', #5978, #28860, #19129 ) ;
#7950=CARTESIAN_POINT ( 'NONE',  ( 10.00000000000000000, 5.773502691896255534, -178.8750000000000000 ) ) ;
#7952=CARTESIAN_POINT ( 'NONE',  ( -10.81189881249999729, 1.324075727343319199E-15, -107.2812500020483810 ) ) ;
#7953=ORIENTED_EDGE ( 'NONE', *, *, #40732, .F. ) ;
#7954=CARTESIAN_POINT ( 'NONE',  ( 9.999999999999998224, 0.000000000000000000, -153.8750000040967905 ) ) ;
#7956=ORIENTED_EDGE ( 'NONE', *, *, #32021, .T. ) ;
#7957=CARTESIAN_POINT ( 'NONE',  ( -2.293366432827344421E-15, -12.48450537969573659, -37.90625000204836681 ) ) ;
#7959=CARTESIAN_POINT ( 'NONE',  ( 5.405949406249992428, -9.363379034771808662, -85.59375000204836681 ) ) ;
#7960=DIRECTION ( 'NONE',  ( 1.000000000000000000, 0.000000000000000000, 0.000000000000000000 ) ) ;
#7961=DIRECTION ( 'NONE',  ( -0.000000000000000000, -0.000000000000000000, 1.000000000000000000 ) ) ;
#7962=( BOUNDED_CURVE ( )  B_SPLINE_CURVE ( 2, ( #11101, #24304, #37448, #5288, #22327, #2483, #41308 ),
 .UNSPECIFIED., .F., .F. ) 
 B_SPLINE_CURVE_WITH_KNOTS ( ( 3, 2, 2, 3 ),
 ( 0.3171641791044778058, 0.3184079601990050801, 0.3196517412935324653, 0.3208955223880597396 ),
 .UNSPECIFIED. ) 
 CURVE ( )  GEOMETRIC_REPRESENTATION_ITEM ( )  RATIONAL_B_SPLINE_CURVE ( ( 0.9999999999999820144, 0.8660254037844566932, 1.000000000000000000, 0.8660254037844387076, 1.000000000000000000, 0.8660254037844327124, 1.000000000000005995 ) ) 
 REPRESENTATION_ITEM ( '' )  );
#7963=AXIS2_PLACEMENT_3D ( 'NONE', #12408, #35741, #42608 ) ;
#7966=CARTESIAN_POINT ( 'NONE',  ( -10.81189881249999729, -6.242252689847864744, -127.9687500020483810 ) ) ;
#7968=CARTESIAN_POINT ( 'NONE',  ( 5.405949406249992428, -9.363379034771808662, -1.781250002048373471 ) ) ;
#7971=CARTESIAN_POINT ( 'NONE',  ( -9.999999999999998224, 1.224646799147353059E-15, -181.6250000040967905 ) ) ;
#7973=CARTESIAN_POINT ( 'NONE',  ( -10.81189881249999729, 1.324075727343319199E-15, -180.7812500020484094 ) ) ;
#7976=CARTESIAN_POINT ( 'NONE',  ( -10.81189881249999729, -6.242252689847864744, -48.46875000204837391 ) ) ;
#7978=CARTESIAN_POINT ( 'NONE',  ( -5.405949406250003975, -9.363379034771801557, -6.531250002048377468 ) ) ;
#7980=CARTESIAN_POINT ( 'NONE',  ( -10.00000000000102496, 5.773502691895664007, -53.87499999999993605 ) ) ;
#7982=CARTESIAN_POINT ( 'NONE',  ( 9.999999999999998224, 0.000000000000000000, -94.99999999999998579 ) ) ;
#7984=CARTESIAN_POINT ( 'NONE',  ( 7.070501591499377789E-16, 11.54700538379251284, -105.5000000040967763 ) ) ;
#7985=CARTESIAN_POINT ( 'NONE',  ( 9.999999999999998224, 0.000000000000000000, -26.37500000409676204 ) ) ;
#7988=CARTESIAN_POINT ( 'NONE',  ( -10.81189881249999729, 1.324075727343319199E-15, -98.28125000204839523 ) ) ;
#7989=ORIENTED_EDGE ( 'NONE', *, *, #6218, .F. ) ;
#7991=CARTESIAN_POINT ( 'NONE',  ( -10.81189881249999729, 1.324075727343319199E-15, -161.2812500020484094 ) ) ;
#7993=ORIENTED_EDGE ( 'NONE', *, *, #18445, .F. ) ;
#7994=CARTESIAN_POINT ( 'NONE',  ( -4.999999999999996447, 8.660254037844387298, -26.99999999999996803 ) ) ;
#7995=EDGE_CURVE ( 'NONE', #8341, #32539, #25184, .T. ) ;
#7996=CARTESIAN_POINT ( 'NONE',  ( -5.405949406249996869, 9.363379034771805109, -32.53125000204837391 ) ) ;
#7997=CARTESIAN_POINT ( 'NONE',  ( 4.999999999999992006, -8.660254037844389075, -158.2500000000000000 ) ) ;
#7998=CARTESIAN_POINT ( 'NONE',  ( -9.999999999999998224, 1.224646799147353059E-15, -177.1250000040968189 ) ) ;
#8001=AXIS2_PLACEMENT_3D ( 'NONE', #42000, #2539, #35342 ) ;
#8002=( BOUNDED_CURVE ( )  B_SPLINE_CURVE ( 2, ( #28240, #25014, #4705, #30832, #4495, #17638, #37728 ),
 .UNSPECIFIED., .F., .F. ) 
 B_SPLINE_CURVE_WITH_KNOTS ( ( 3, 2, 2, 3 ),
 ( 0.2985074626865671932, 0.2997512437810946340, 0.3009950248756220192, 0.3022388059701494045 ),
 .UNSPECIFIED. ) 
 CURVE ( )  GEOMETRIC_REPRESENTATION_ITEM ( )  RATIONAL_B_SPLINE_CURVE ( ( 0.9999999999999940048, 0.8660254037844447028, 1.000000000000000000, 0.8660254037844387076, 1.000000000000000000, 0.8660254037844207220, 1.000000000000017986 ) ) 
 REPRESENTATION_ITEM ( '' )  );
#8003=EDGE_CURVE ( 'NONE', #14981, #15576, #2514, .T. ) ;
#8004=CARTESIAN_POINT ( 'NONE',  ( 5.405949406249999534, 9.363379034771803333, -133.2812500020483810 ) ) ;
#8005=CARTESIAN_POINT ( 'NONE',  ( -4.999999999999996447, 8.660254037844387298, -139.8750000040968189 ) ) ;
#8007=CARTESIAN_POINT ( 'NONE',  ( 5.000000000000000000, 8.660254037844385522, -162.6250000040967905 ) ) ;
#8009=( BOUNDED_CURVE ( )  B_SPLINE_CURVE ( 2, ( #6401, #16288, #2952, #6600, #32726, #15660, #32523 ),
 .UNSPECIFIED., .F., .F. ) 
 B_SPLINE_CURVE_WITH_KNOTS ( ( 3, 2, 2, 3 ),
 ( 0.1902985074626866169, 0.1915422885572139744, 0.1927860696517413319, 0.1940298507462686894 ),
 .UNSPECIFIED. ) 
 CURVE ( )  GEOMETRIC_REPRESENTATION_ITEM ( )  RATIONAL_B_SPLINE_CURVE ( ( 0.9999999999999940048, 0.8660254037844447028, 1.000000000000000000, 0.8660254037844387076, 1.000000000000000000, 0.8660254037844357100, 1.000000000000003109 ) ) 
 REPRESENTATION_ITEM ( '' )  );
#8010=CARTESIAN_POINT ( 'NONE',  ( -5.405949406249996869, 9.363379034771805109, -59.53125000204836681 ) ) ;
#8011=EDGE_LOOP ( 'NONE', ( #41801, #17586, #10572, #2294 ) ) ;
#8012=ORIENTED_EDGE ( 'NONE', *, *, #9538, .F. ) ;
#8013=ADVANCED_FACE ( 'NONE', ( #123 ), #6577, .T. ) ;
#8016=CARTESIAN_POINT ( 'NONE',  ( -2.293366432827344421E-15, -12.48450537969573659, -165.2187500020484094 ) ) ;
#8017=( BOUNDED_CURVE ( )  B_SPLINE_CURVE ( 2, ( #18346, #1962, #2178, #26834, #38202, #8647, #21802 ),
 .UNSPECIFIED., .F., .F. ) 
 B_SPLINE_CURVE_WITH_KNOTS ( ( 3, 2, 2, 3 ),
 ( 0.5858208955223881409, 0.5870646766169155262, 0.5883084577114429115, 0.5895522388059702967 ),
 .UNSPECIFIED. ) 
 CURVE ( )  GEOMETRIC_REPRESENTATION_ITEM ( )  RATIONAL_B_SPLINE_CURVE ( ( 0.9999999999999880096, 0.8660254037844506980, 1.000000000000000000, 0.8660254037844387076, 1.000000000000000000, 0.8660254037844267172, 1.000000000000011990 ) ) 
 REPRESENTATION_ITEM ( '' )  );
#8020=CARTESIAN_POINT ( 'NONE',  ( 10.81189881249999729, 0.000000000000000000, -11.84375000204834727 ) ) ;
#8022=CARTESIAN_POINT ( 'NONE',  ( -5.405949406249996869, 9.363379034771805109, -144.8437500020483810 ) ) ;
#8023=CARTESIAN_POINT ( 'NONE',  ( 7.644554776091147741E-16, 12.48450537969573659, -132.9687500020483810 ) ) ;
#8024=CARTESIAN_POINT ( 'NONE',  ( -10.81189881249999729, 1.324075727343319199E-15, -108.7812500020483810 ) ) ;
#8028=CARTESIAN_POINT ( 'NONE',  ( 10.81189881249999729, 0.000000000000000000, 0.1562499979516351889 ) ) ;
#8034=CARTESIAN_POINT ( 'NONE',  ( 5.405949406249999534, 9.363379034771803333, -73.09375000204838102 ) ) ;
#8035=CARTESIAN_POINT ( 'NONE',  ( -5.405949406249996869, 9.363379034771805109, -68.34375000204836681 ) ) ;
#8036=CARTESIAN_POINT ( 'NONE',  ( -9.999999999999998224, 1.224646799147353059E-15, -76.24999999999998579 ) ) ;
#8037=CARTESIAN_POINT ( 'NONE',  ( -10.81189881249999729, 6.242252689847871849, -33.90625000204836681 ) ) ;
#8041=CARTESIAN_POINT ( 'NONE',  ( -5.000000000000003553, -8.660254037844383745, -125.5000000000000000 ) ) ;
#8042=CARTESIAN_POINT ( 'NONE',  ( -10.81189881249999729, -6.242252689847864744, -132.6562500020483810 ) ) ;
#8045=CARTESIAN_POINT ( 'NONE',  ( 7.644554776091147741E-16, 12.48450537969573659, -22.15625000204837391 ) ) ;
#8046=ORIENTED_EDGE ( 'NONE', *, *, #22874, .T. ) ;
#8049=CARTESIAN_POINT ( 'NONE',  ( 7.070501591499377789E-16, 11.54700538379251284, -36.50000000409675494 ) ) ;
#8054=CARTESIAN_POINT ( 'NONE',  ( -9.999999999999834799, -5.773502691896343464, -191.6250000000000000 ) ) ;
#8055=CARTESIAN_POINT ( 'NONE',  ( -5.405949406250003975, -9.363379034771801557, -152.0312500020484094 ) ) ;
#8056=CARTESIAN_POINT ( 'NONE',  ( 10.81189881249999907, 6.242252689847868297, -130.2187500020483810 ) ) ;
#8059=DIRECTION ( 'NONE',  ( 1.000000000000000000, 0.000000000000000000, 0.000000000000000000 ) ) ;
#8060=ORIENTED_EDGE ( 'NONE', *, *, #25451, .T. ) ;
#8062=EDGE_LOOP ( 'NONE', ( #26932, #21159, #427, #37434 ) ) ;
#8063=EDGE_CURVE ( 'NONE', #34185, #17371, #21311, .T. ) ;
#8064=CARTESIAN_POINT ( 'NONE',  ( -9.999999999999998224, 1.224646799147353059E-15, -42.12500000409677625 ) ) ;
#8065=CARTESIAN_POINT ( 'NONE',  ( -10.81189881249999907, -6.242252689847864744, -187.9687500020484094 ) ) ;
#8066=CARTESIAN_POINT ( 'NONE',  ( 10.81189881249999907, 6.242252689847868297, -37.21875000204835970 ) ) ;
#8068=CARTESIAN_POINT ( 'NONE',  ( -5.405949406250003975, -9.363379034771801557, -175.8437500020483810 ) ) ;
#8069=CARTESIAN_POINT ( 'NONE',  ( 10.81189881249999907, 6.242252689847868297, -160.2187500020483810 ) ) ;
#8070=DIRECTION ( 'NONE',  ( 1.000000000000000000, 0.000000000000000000, 0.000000000000000000 ) ) ;
#8074=CARTESIAN_POINT ( 'NONE',  ( 7.070501591499376803E-16, 11.54700538379251284, -134.0000000040967905 ) ) ;
#8075=CARTESIAN_POINT ( 'NONE',  ( -9.999999999999998224, 1.224646799147353059E-15, -66.12500000409676204 ) ) ;
#8077=CARTESIAN_POINT ( 'NONE',  ( -2.293366432827344421E-15, -12.48450537969573659, -90.21875000204838102 ) ) ;
#8079=CARTESIAN_POINT ( 'NONE',  ( 5.405949406249999534, 9.363379034771803333, -58.28125000204836681 ) ) ;
#8082=CARTESIAN_POINT ( 'NONE',  ( -10.81189881249999907, -6.242252689847864744, -116.1562500020483952 ) ) ;
#8083=CARTESIAN_POINT ( 'NONE',  ( 5.405949406249992428, -9.363379034771808662, -153.2812500020484094 ) ) ;
#8084=( BOUNDED_CURVE ( )  B_SPLINE_CURVE ( 2, ( #19008, #29157, #22675, #9290, #25712, #29574, #19 ),
 .UNSPECIFIED., .F., .F. ) 
 B_SPLINE_CURVE_WITH_KNOTS ( ( 3, 2, 2, 3 ),
 ( 0.7574626865671643117, 0.7587064676616916969, 0.7599502487562190822, 0.7611940298507464675 ),
 .UNSPECIFIED. ) 
 CURVE ( )  GEOMETRIC_REPRESENTATION_ITEM ( )  RATIONAL_B_SPLINE_CURVE ( ( 0.9999999999999880096, 0.8660254037844506980, 1.000000000000000000, 0.8660254037844387076, 1.000000000000000000, 0.8660254037844148378, 1.000000000000023981 ) ) 
 REPRESENTATION_ITEM ( '' )  );
#8087=CARTESIAN_POINT ( 'NONE',  ( -4.999999999999996447, 8.660254037844387298, -127.8750000040967905 ) ) ;
#8089=ORIENTED_EDGE ( 'NONE', *, *, #34117, .T. ) ;
#8092=CARTESIAN_POINT ( 'NONE',  ( 9.999999999998969713, 5.773502691896851502, -68.25000000409676204 ) ) ;
#8093=CARTESIAN_POINT ( 'NONE',  ( -5.405949406250003975, -9.363379034771801557, -177.5312500020483810 ) ) ;
#8096=CARTESIAN_POINT ( 'NONE',  ( 9.999999999999996447, -5.773502691896262640, -58.00000000409676915 ) ) ;
#8097=CARTESIAN_POINT ( 'NONE',  ( -9.999999999999998224, 1.224646799147353059E-15, -97.24999999999998579 ) ) ;
#8098=CARTESIAN_POINT ( 'NONE',  ( 5.000000000000000000, 8.660254037844385522, -135.6250000040967620 ) ) ;
#8100=CARTESIAN_POINT ( 'NONE',  ( -5.405949406249996869, 9.363379034771805109, -55.03125000204836681 ) ) ;
#8103=LINE ( 'NONE', #34011, #26925 ) ;
#8104=CARTESIAN_POINT ( 'NONE',  ( -2.293366432827344421E-15, -12.48450537969573659, -180.4062500020484379 ) ) ;
#8106=DIRECTION ( 'NONE',  ( 0.000000000000000000, 0.9961946980917455452, -0.08715574274765837404 ) ) ;
#8108=CARTESIAN_POINT ( 'NONE',  ( -9.999999999999998224, 1.224646799147353059E-15, -154.2500000000000000 ) ) ;
#8110=DIRECTION ( 'NONE',  ( -0.000000000000000000, -0.000000000000000000, 1.000000000000000000 ) ) ;
#8111=EDGE_CURVE ( 'NONE', #16149, #21857, #24098, .T. ) ;
#8112=CARTESIAN_POINT ( 'NONE',  ( -10.81189881249999729, 6.242252689847871849, -86.40625000204836681 ) ) ;
#8113=VERTEX_POINT ( 'NONE', #20161 ) ;
#8114=LINE ( 'NONE', #31425, #41298 ) ;
#8115=ORIENTED_EDGE ( 'NONE', *, *, #23366, .F. ) ;
#8117=CARTESIAN_POINT ( 'NONE',  ( -10.81189881249999729, 6.242252689847871849, -36.71875000204835970 ) ) ;
#8118=CARTESIAN_POINT ( 'NONE',  ( -2.293366432827344421E-15, -12.48450537969573659, -30.21875000204834905 ) ) ;
#8119=CARTESIAN_POINT ( 'NONE',  ( -5.405949406250003975, -9.363379034771801557, -11.03125000204835438 ) ) ;
#8120=CARTESIAN_POINT ( 'NONE',  ( 10.81189881249999551, -6.242252689847874514, -62.96875000204838813 ) ) ;
#8124=CARTESIAN_POINT ( 'NONE',  ( 10.81189881249999907, 6.242252689847868297, -188.7187500020484094 ) ) ;
#8126=EDGE_CURVE ( 'NONE', #22125, #15042, #6451, .T. ) ;
#8127=( BOUNDED_CURVE ( )  B_SPLINE_CURVE ( 2, ( #8292, #11288, #37635, #8074, #33765, #30536, #1174 ),
 .UNSPECIFIED., .F., .F. ) 
 B_SPLINE_CURVE_WITH_KNOTS ( ( 3, 2, 2, 3 ),
 ( 0.3208955223880597396, 0.3221393034825871804, 0.3233830845771145657, 0.3246268656716419510 ),
 .UNSPECIFIED. ) 
 CURVE ( )  GEOMETRIC_REPRESENTATION_ITEM ( )  RATIONAL_B_SPLINE_CURVE ( ( 0.9999999999999940048, 0.8660254037844447028, 1.000000000000000000, 0.8660254037844387076, 1.000000000000000000, 0.8660254037844207220, 1.000000000000017986 ) ) 
 REPRESENTATION_ITEM ( '' )  );
#8128=CARTESIAN_POINT ( 'NONE',  ( -4.999999999999996447, 8.660254037844387298, -43.49999999999998579 ) ) ;
#8129=CARTESIAN_POINT ( 'NONE',  ( -5.000000000000003553, -8.660254037844383745, -193.0000000000000000 ) ) ;
#8130=LINE ( 'NONE', #34254, #40512 ) ;
#8131=CYLINDRICAL_SURFACE ( 'NONE', #27308, 9.999999999999998224 ) ;
#8132=CARTESIAN_POINT ( 'NONE',  ( 4.999999999999992006, -8.660254037844389075, -89.62500000409677625 ) ) ;
#8133=CARTESIAN_POINT ( 'NONE',  ( -10.81189881249999907, -6.242252689847864744, -114.4687500020483810 ) ) ;
#8135=VECTOR ( 'NONE', #34037, 1000.000000000000000 ) ;
#8136=CARTESIAN_POINT ( 'NONE',  ( -10.81189881249999907, -6.242252689847864744, -83.15625000204836681 ) ) ;
#8137=CARTESIAN_POINT ( 'NONE',  ( 10.81189881249999729, 6.242252689847867408, -97.21875000204838102 ) ) ;
#8138=VECTOR ( 'NONE', #3618, 1000.000000000000000 ) ;
#8141=CARTESIAN_POINT ( 'NONE',  ( -10.00000000000000000, -5.773502691896251982, -154.5000000040967905 ) ) ;
#8145=CARTESIAN_POINT ( 'NONE',  ( -5.000000000000003553, -8.660254037844383745, -175.0000000000000284 ) ) ;
#8146=CARTESIAN_POINT ( 'NONE',  ( 5.000000000000000000, 8.660254037844385522, -172.7500000000000284 ) ) ;
#8148=CARTESIAN_POINT ( 'NONE',  ( 9.999999999999998224, 0.000000000000000000, -120.8750000040967905 ) ) ;
#8149=CARTESIAN_POINT ( 'NONE',  ( 4.999999999999992006, -8.660254037844389075, -74.24999999999998579 ) ) ;
#8151=CARTESIAN_POINT ( 'NONE',  ( -9.999999999999998224, 5.773502691896259087, -82.75000000409676204 ) ) ;
#8152=CARTESIAN_POINT ( 'NONE',  ( 4.999999999999992006, -8.660254037844389075, -142.1250000040967905 ) ) ;
#8154=CARTESIAN_POINT ( 'NONE',  ( -10.81189881249999729, 6.242252689847871849, -77.40625000204838102 ) ) ;
#8156=CARTESIAN_POINT ( 'NONE',  ( -9.999999999998456346, -5.773502691897145489, -59.62499999999995737 ) ) ;
#8158=ORIENTED_EDGE ( 'NONE', *, *, #13702, .T. ) ;
#8159=CARTESIAN_POINT ( 'NONE',  ( -4.999999999999996447, 8.660254037844387298, -4.499999999999976019 ) ) ;
#8161=CARTESIAN_POINT ( 'NONE',  ( 5.405949406249992428, -9.363379034771808662, -16.59375000204835260 ) ) ;
#8165=CARTESIAN_POINT ( 'NONE',  ( 7.644554776091147741E-16, 12.48450537969573659, -130.1562500020483810 ) ) ;
#8166=EDGE_CURVE ( 'NONE', #38628, #8276, #13850, .T. ) ;
#8167=CARTESIAN_POINT ( 'NONE',  ( 7.070501591499377789E-16, 11.54700538379251284, -186.1250000000000000 ) ) ;
#8168=DIRECTION ( 'NONE',  ( 1.000000000000000000, 0.000000000000000000, 0.000000000000000000 ) ) ;
#8169=CARTESIAN_POINT ( 'NONE',  ( 5.405949406249999534, 9.363379034771803333, -113.7812500020483952 ) ) ;
#8170=VERTEX_POINT ( 'NONE', #16058 ) ;
#8172=AXIS2_PLACEMENT_3D ( 'NONE', #29462, #26015, #30105 ) ;
#8173=EDGE_LOOP ( 'NONE', ( #899, #21050, #39461, #9268 ) ) ;
#8174=EDGE_LOOP ( 'NONE', ( #31194, #9121, #10151, #31189 ) ) ;
#8175=CARTESIAN_POINT ( 'NONE',  ( 10.81189881249999729, 0.000000000000000000, -40.53125000204838102 ) ) ;
#8177=CARTESIAN_POINT ( 'NONE',  ( 5.405949406249992428, -9.363379034771808662, -87.09375000204836681 ) ) ;
#8178=LINE ( 'NONE', #33867, #2240 ) ;
#8179=FACE_OUTER_BOUND ( 'NONE', #23562, .T. ) ;
#8180=CARTESIAN_POINT ( 'NONE',  ( -2.121150477449813534E-15, -11.54700538379251284, -32.75000000409675494 ) ) ;
#8182=CARTESIAN_POINT ( 'NONE',  ( 5.000000000000000000, 8.660254037844385522, -54.62500000409675494 ) ) ;
#8184=CARTESIAN_POINT ( 'NONE',  ( -2.293366432827344421E-15, -12.48450537969573659, -124.7187500020483952 ) ) ;
#8186=CARTESIAN_POINT ( 'NONE',  ( -10.81189881249999729, 1.324075727343319199E-15, -3.781250002048375247 ) ) ;
#8189=CARTESIAN_POINT ( 'NONE',  ( -10.00000000000000000, -5.773502691896251982, -181.5000000040967905 ) ) ;
#8190=CARTESIAN_POINT ( 'NONE',  ( 5.405949406249999534, 9.363379034771803333, -170.7812500020484094 ) ) ;
#8191=CARTESIAN_POINT ( 'NONE',  ( -5.000000000000003553, -8.660254037844383745, -28.37500000409676204 ) ) ;
#8194=CARTESIAN_POINT ( 'NONE',  ( -5.405949406250003975, -9.363379034771801557, -52.84375000204835970 ) ) ;
#8196=CARTESIAN_POINT ( 'NONE',  ( -2.293366432827344421E-15, -12.48450537969573659, -10.90625000204838457 ) ) ;
#8200=CARTESIAN_POINT ( 'NONE',  ( -5.000000000000003553, -8.660254037844383745, -96.99999999999998579 ) ) ;
#8202=CARTESIAN_POINT ( 'NONE',  ( 4.999999999999992006, -8.660254037844389075, -104.6250000040967763 ) ) ;
#8203=VECTOR ( 'NONE', #4957, 1000.000000000000000 ) ;
#8204=CARTESIAN_POINT ( 'NONE',  ( -9.999999999999479527, -5.773502691896549521, -150.0000000040967905 ) ) ;
#8207=CARTESIAN_POINT ( 'NONE',  ( 10.81189881249999729, 6.242252689847867408, -97.40625000204839523 ) ) ;
#8212=CARTESIAN_POINT ( 'NONE',  ( 10.81189881249999729, 0.000000000000000000, -166.5312500020484094 ) ) ;
#8215=CARTESIAN_POINT ( 'NONE',  ( -5.000000000000003553, -8.660254037844383745, -21.99999999999996447 ) ) ;
#8216=CARTESIAN_POINT ( 'NONE',  ( -5.405949406250003975, -9.363379034771801557, -27.53125000204836681 ) ) ;
#8217=CARTESIAN_POINT ( 'NONE',  ( 5.000000000000000000, 8.660254037844385522, -157.7500000000000000 ) ) ;
#8218=FACE_OUTER_BOUND ( 'NONE', #30549, .T. ) ;
#8220=DIRECTION ( 'NONE',  ( -0.000000000000000000, 1.000000000000000000, -0.000000000000000000 ) ) ;
#8221=CARTESIAN_POINT ( 'NONE',  ( -10.81189881249999729, 1.324075727343319199E-15, -132.7812500020483810 ) ) ;
#8222=CARTESIAN_POINT ( 'NONE',  ( -9.999999999999998224, 1.224646799147353059E-15, -200.0000000000000000 ) ) ;
#8223=CARTESIAN_POINT ( 'NONE',  ( -5.000000000000003553, -8.660254037844383745, -44.87500000409677625 ) ) ;
#8224=ORIENTED_EDGE ( 'NONE', *, *, #9990, .F. ) ;
#8225=CARTESIAN_POINT ( 'NONE',  ( 5.405949406249992428, -9.363379034771808662, -63.28125000204837391 ) ) ;
#8227=ORIENTED_EDGE ( 'NONE', *, *, #22293, .F. ) ;
#8228=VERTEX_POINT ( 'NONE', #3979 ) ;
#8229=CARTESIAN_POINT ( 'NONE',  ( -2.121150477449813534E-15, -11.54700538379251284, -120.8749999999999858 ) ) ;
#8230=CARTESIAN_POINT ( 'NONE',  ( -9.999999999999998224, 1.224646799147353059E-15, -141.1250000040967905 ) ) ;
#8231=CARTESIAN_POINT ( 'NONE',  ( 5.405949406249992428, -9.363379034771808662, -160.5937500020484094 ) ) ;
#8233=CARTESIAN_POINT ( 'NONE',  ( 5.405949406249992428, -9.363379034771808662, -16.59375000204835260 ) ) ;
#8234=VECTOR ( 'NONE', #18693, 1000.000000000000000 ) ;
#8236=CARTESIAN_POINT ( 'NONE',  ( 10.81189881249999729, 0.000000000000000000, -148.3437500020483810 ) ) ;
#8238=CARTESIAN_POINT ( 'NONE',  ( -10.81189881249999729, 6.242252689847871849, -107.4062500020483810 ) ) ;
#8240=CARTESIAN_POINT ( 'NONE',  ( -9.999999999999998224, 1.224646799147353059E-15, -161.7500000000000000 ) ) ;
#8242=CARTESIAN_POINT ( 'NONE',  ( -10.81189881249999907, -6.242252689847864744, -3.468750002048364145 ) ) ;
#8244=CARTESIAN_POINT ( 'NONE',  ( 5.405949406249999534, 9.363379034771803333, -191.7812500020484094 ) ) ;
#8245=AXIS2_PLACEMENT_3D ( 'NONE', #35799, #39442, #3201 ) ;
#8249=CARTESIAN_POINT ( 'NONE',  ( 10.81189881249999729, 6.242252689847867408, -79.21875000204839523 ) ) ;
#8250=CARTESIAN_POINT ( 'NONE',  ( -10.81189881249999729, 6.242252689847871849, -53.21875000204837391 ) ) ;
#8251=DIRECTION ( 'NONE',  ( -0.000000000000000000, -0.000000000000000000, 1.000000000000000000 ) ) ;
#8252=CARTESIAN_POINT ( 'NONE',  ( -5.405949406250003975, -9.363379034771801557, -35.03125000204837391 ) ) ;
#8254=CARTESIAN_POINT ( 'NONE',  ( 9.999999999999998224, 0.000000000000000000, -137.0000000000000000 ) ) ;
#8256=CARTESIAN_POINT ( 'NONE',  ( 9.999999999999996447, -5.773502691896262640, -123.6250000000000000 ) ) ;
#8257=CARTESIAN_POINT ( 'NONE',  ( 9.999999999999479527, 5.773502691896553074, -42.37499999999997158 ) ) ;
#8259=CARTESIAN_POINT ( 'NONE',  ( 10.81189881249999729, 6.242252689847867408, -7.406250002048366810 ) ) ;
#8261=EDGE_LOOP ( 'NONE', ( #6257, #30204, #39601, #32374 ) ) ;
#8265=CARTESIAN_POINT ( 'NONE',  ( 10.00000000000000000, 5.773502691896255534, -33.75000000409674783 ) ) ;
#8266=CARTESIAN_POINT ( 'NONE',  ( 7.070501591499376803E-16, 11.54700538379251284, -61.62499999999998579 ) ) ;
#8268=( BOUNDED_CURVE ( )  B_SPLINE_CURVE ( 2, ( #27736, #1845, #2280, #28599, #14971, #34435, #11313 ),
 .UNSPECIFIED., .F., .F. ) 
 B_SPLINE_CURVE_WITH_KNOTS ( ( 3, 2, 2, 3 ),
 ( 0.3432835820895522860, 0.3445273631840797268, 0.3457711442786070566, 0.3470149253731344974 ),
 .UNSPECIFIED. ) 
 CURVE ( )  GEOMETRIC_REPRESENTATION_ITEM ( )  RATIONAL_B_SPLINE_CURVE ( ( 0.9999999999999940048, 0.8660254037844447028, 1.000000000000000000, 0.8660254037844387076, 1.000000000000000000, 0.8660254037844207220, 1.000000000000017986 ) ) 
 REPRESENTATION_ITEM ( '' )  );
#8269=FACE_OUTER_BOUND ( 'NONE', #24687, .T. ) ;
#8270=CARTESIAN_POINT ( 'NONE',  ( 10.81189881249999907, 6.242252689847868297, -142.4062500020484094 ) ) ;
#8271=AXIS2_PLACEMENT_3D ( 'NONE', #4492, #40509, #23285 ) ;
#8272=CARTESIAN_POINT ( 'NONE',  ( -5.405949406249996869, 9.363379034771805109, -123.8437500020483952 ) ) ;
#8273=CARTESIAN_POINT ( 'NONE',  ( 9.999999999998969713, 5.773502691896851502, -3.750000004096736284 ) ) ;
#8274=ADVANCED_FACE ( 'NONE', ( #17120 ), #10648, .T. ) ;
#8275=CARTESIAN_POINT ( 'NONE',  ( 9.999999999999998224, 0.000000000000000000, -200.0000000000000000 ) ) ;
#8276=VERTEX_POINT ( 'NONE', #36991 ) ;
#8277=VERTEX_POINT ( 'NONE', #7426 ) ;
#8278=EDGE_LOOP ( 'NONE', ( #15863, #10747, #42471, #36696 ) ) ;
#8280=CARTESIAN_POINT ( 'NONE',  ( -5.405949406249996869, 9.363379034771805109, -180.8437500020483810 ) ) ;
#8281=CARTESIAN_POINT ( 'NONE',  ( -10.81189881249999907, -6.242252689847864744, -36.46875000204835970 ) ) ;
#8283=DIRECTION ( 'NONE',  ( 1.000000000000000000, 0.000000000000000000, 0.000000000000000000 ) ) ;
#8284=EDGE_CURVE ( 'NONE', #23120, #28565, #12229, .T. ) ;
#8285=CARTESIAN_POINT ( 'NONE',  ( -10.81189881249999729, 6.242252689847871849, -171.7187500020483810 ) ) ;
#8286=CARTESIAN_POINT ( 'NONE',  ( -10.81189881249999729, 1.324075727343319199E-15, -150.5937500020483810 ) ) ;
#8291=EDGE_CURVE ( 'NONE', #26792, #32801, #11289, .T. ) ;
#8292=CARTESIAN_POINT ( 'NONE',  ( 9.999999999999998224, 0.000000000000000000, -134.3750000040967905 ) ) ;
#8293=CARTESIAN_POINT ( 'NONE',  ( -10.00000000000051337, 5.773502691895962435, -70.37499999999997158 ) ) ;
#8296=EDGE_CURVE ( 'NONE', #26141, #42072, #21226, .T. ) ;
#8297=CARTESIAN_POINT ( 'NONE',  ( 7.644554776091147741E-16, 12.48450537969573659, -92.46875000204838102 ) ) ;
#8298=CARTESIAN_POINT ( 'NONE',  ( 9.999999999999998224, 0.000000000000000000, -180.8750000040967905 ) ) ;
#8299=CARTESIAN_POINT ( 'NONE',  ( -10.81189881249999729, 1.324075727343319199E-15, -60.78125000204836681 ) ) ;
#8301=CARTESIAN_POINT ( 'NONE',  ( -2.293366432827344421E-15, -12.48450537969573659, -115.9062500020483810 ) ) ;
#8302=CARTESIAN_POINT ( 'NONE',  ( -10.81189881249999729, -6.242252689847864744, -156.6562500020484094 ) ) ;
#8304=CARTESIAN_POINT ( 'NONE',  ( -9.999999999999998224, 1.224646799147353059E-15, -200.0000000000000000 ) ) ;
#8306=CARTESIAN_POINT ( 'NONE',  ( -9.999999999999998224, 5.773502691896259087, -129.2500000040967905 ) ) ;
#8308=ORIENTED_EDGE ( 'NONE', *, *, #38527, .F. ) ;
#8312=CARTESIAN_POINT ( 'NONE',  ( -5.405949406249996869, 9.363379034771805109, -184.0312500020484094 ) ) ;
#8313=ORIENTED_EDGE ( 'NONE', *, *, #37146, .F. ) ;
#8315=CARTESIAN_POINT ( 'NONE',  ( -2.121150477449813534E-15, -11.54700538379251284, -59.75000000409676915 ) ) ;
#8317=DIRECTION ( 'NONE',  ( 1.000000000000000000, 0.000000000000000000, 0.000000000000000000 ) ) ;
#8319=CARTESIAN_POINT ( 'NONE',  ( -2.293366432827344421E-15, -12.48450537969573659, -52.90625000204837391 ) ) ;
#8320=EDGE_CURVE ( 'NONE', #36297, #27433, #34821, .T. ) ;
#8323=CYLINDRICAL_SURFACE ( 'NONE', #25559, 9.999999999999998224 ) ;
#8324=CARTESIAN_POINT ( 'NONE',  ( 5.405949406249999534, 9.363379034771803333, -179.7812500020484094 ) ) ;
#8325=CARTESIAN_POINT ( 'NONE',  ( 9.999999999999479527, 5.773502691896553074, -2.250000004096741613 ) ) ;
#8328=CARTESIAN_POINT ( 'NONE',  ( 9.999999999998969713, 5.773502691896851502, -17.25000000409673717 ) ) ;
#8329=LINE ( 'NONE', #18013, #15559 ) ;
#8330=DIRECTION ( 'NONE',  ( 1.000000000000000000, 0.000000000000000000, 0.000000000000000000 ) ) ;
#8331=VECTOR ( 'NONE', #18293, 1000.000000000000000 ) ;
#8332=CARTESIAN_POINT ( 'NONE',  ( 10.81189881249999907, 6.242252689847868297, -76.40625000204839523 ) ) ;
#8333=EDGE_LOOP ( 'NONE', ( #2278, #12553, #14454, #7783 ) ) ;
#8334=CARTESIAN_POINT ( 'NONE',  ( 9.999999999999998224, 0.000000000000000000, -81.49999999999998579 ) ) ;
#8336=VERTEX_POINT ( 'NONE', #30744 ) ;
#8337=CARTESIAN_POINT ( 'NONE',  ( 10.81189881249999729, 6.242252689847867408, -37.21875000204835970 ) ) ;
#8338=CARTESIAN_POINT ( 'NONE',  ( -10.00000000000051337, 5.773502691895962435, -76.75000000409677625 ) ) ;
#8339=CARTESIAN_POINT ( 'NONE',  ( -10.81189881249999907, -6.242252689847864744, -14.15625000204836859 ) ) ;
#8340=CARTESIAN_POINT ( 'NONE',  ( 10.81189881249999907, 6.242252689847868297, -59.71875000204838102 ) ) ;
#8341=VERTEX_POINT ( 'NONE', #14297 ) ;
#8342=FACE_OUTER_BOUND ( 'NONE', #4289, .T. ) ;
#8344=CARTESIAN_POINT ( 'NONE',  ( -10.81189881249999729, 6.242252689847871849, -198.7187500020484379 ) ) ;
#8345=CARTESIAN_POINT ( 'NONE',  ( 5.405949406249999534, 9.363379034771803333, -173.5937500020484094 ) ) ;
#8346=( BOUNDED_CURVE ( )  B_SPLINE_CURVE ( 2, ( #22944, #9553, #30060, #2879, #6532, #42344, #25968 ),
 .UNSPECIFIED., .F., .F. ) 
 B_SPLINE_CURVE_WITH_KNOTS ( ( 3, 2, 2, 3 ),
 ( 0.8656716417910450545, 0.8669154228855724398, 0.8681592039800998251, 0.8694029850746272103 ),
 .UNSPECIFIED. ) 
 CURVE ( )  GEOMETRIC_REPRESENTATION_ITEM ( )  RATIONAL_B_SPLINE_CURVE ( ( 0.9999999999999641398, 0.8660254037844745678, 1.000000000000000000, 0.8660254037844387076, 1.000000000000000000, 0.8660254037844028474, 1.000000000000035971 ) ) 
 REPRESENTATION_ITEM ( '' )  );
#8349=CARTESIAN_POINT ( 'NONE',  ( 4.999999999999992006, -8.660254037844389075, -192.7500000000000000 ) ) ;
#8350=CARTESIAN_POINT ( 'NONE',  ( 7.070501591499376803E-16, 11.54700538379251284, -71.00000000409676204 ) ) ;
#8352=CARTESIAN_POINT ( 'NONE',  ( -2.293366432827344421E-15, -12.48450537969573659, -109.7187500020483668 ) ) ;
#8354=CARTESIAN_POINT ( 'NONE',  ( 7.644554776091147741E-16, 12.48450537969573659, -85.15625000204838102 ) ) ;
#8355=CARTESIAN_POINT ( 'NONE',  ( 7.644554776091147741E-16, 12.48450537969573659, -93.96875000204838102 ) ) ;
#8358=CARTESIAN_POINT ( 'NONE',  ( -10.00000000000000000, -5.773502691896251982, -153.0000000040967905 ) ) ;
#8364=CARTESIAN_POINT ( 'NONE',  ( 9.999999999999998224, 0.000000000000000000, -174.5000000000000284 ) ) ;
#8365=DIRECTION ( 'NONE',  ( -0.000000000000000000, -0.000000000000000000, 1.000000000000000000 ) ) ;
#8368=CARTESIAN_POINT ( 'NONE',  ( -10.00000000000000000, -5.773502691896251982, -74.62499999999997158 ) ) ;
#8370=CARTESIAN_POINT ( 'NONE',  ( 7.070501591499377789E-16, 11.54700538379251284, -84.50000000409677625 ) ) ;
#8371=CARTESIAN_POINT ( 'NONE',  ( 7.070501591499376803E-16, 11.54700538379251284, -26.00000000409676915 ) ) ;
#8373=CARTESIAN_POINT ( 'NONE',  ( 10.81189881249999551, -6.242252689847874514, -73.65625000204835260 ) ) ;
#8375=CARTESIAN_POINT ( 'NONE',  ( -9.999999999999998224, 1.224646799147353059E-15, -112.6250000040967763 ) ) ;
#8378=CARTESIAN_POINT ( 'NONE',  ( 7.070501591499377789E-16, 11.54700538379251284, -0.1249999999999685252 ) ) ;
#8380=CARTESIAN_POINT ( 'NONE',  ( -5.405949406250003975, -9.363379034771801557, -16.84375000204835260 ) ) ;
#8382=CARTESIAN_POINT ( 'NONE',  ( -10.81189881249999729, 1.324075727343319199E-15, -146.0937500020483810 ) ) ;
#8383=CARTESIAN_POINT ( 'NONE',  ( -9.999999999999998224, 1.224646799147353059E-15, -50.74999999999996447 ) ) ;
#8385=CARTESIAN_POINT ( 'NONE',  ( -2.293366432827344421E-15, -12.48450537969573659, -130.9062500020483810 ) ) ;
#8386=CARTESIAN_POINT ( 'NONE',  ( -9.999999999999998224, 1.224646799147353059E-15, -181.2500000000000284 ) ) ;
#8387=CARTESIAN_POINT ( 'NONE',  ( 7.070501591499376803E-16, 11.54700538379251284, -106.6249999999999858 ) ) ;
#8388=CARTESIAN_POINT ( 'NONE',  ( -2.293366432827344421E-15, -12.48450537969573659, -111.4062500020483952 ) ) ;
#8390=VERTEX_POINT ( 'NONE', #34201 ) ;
#8391=EDGE_LOOP ( 'NONE', ( #8490, #8089, #40202, #31753 ) ) ;
#8392=VECTOR ( 'NONE', #25943, 1000.000000000000000 ) ;
#8393=( BOUNDED_CURVE ( )  B_SPLINE_CURVE ( 2, ( #2250, #15369, #28782, #1813, #5892, #34616, #19049 ),
 .UNSPECIFIED., .F., .F. ) 
 B_SPLINE_CURVE_WITH_KNOTS ( ( 3, 2, 2, 3 ),
 ( 0.4029850746268657802, 0.4042288557213931655, 0.4054726368159204397, 0.4067164179104478250 ),
 .UNSPECIFIED. ) 
 CURVE ( )  GEOMETRIC_REPRESENTATION_ITEM ( )  RATIONAL_B_SPLINE_CURVE ( ( 0.9999999999999880096, 0.8660254037844506980, 1.000000000000000000, 0.8660254037844387076, 1.000000000000000000, 0.8660254037844327124, 1.000000000000005995 ) ) 
 REPRESENTATION_ITEM ( '' )  );
#8394=CARTESIAN_POINT ( 'NONE',  ( -10.81189881249999729, 1.324075727343319199E-15, -36.78125000204837391 ) ) ;
#8397=CARTESIAN_POINT ( 'NONE',  ( -10.81189881249999729, 6.242252689847871849, -89.21875000204836681 ) ) ;
#8399=DIRECTION ( 'NONE',  ( -0.000000000000000000, -0.000000000000000000, 1.000000000000000000 ) ) ;
#8400=DIRECTION ( 'NONE',  ( -0.000000000000000000, -0.000000000000000000, 1.000000000000000000 ) ) ;
#8402=VECTOR ( 'NONE', #57, 1000.000000000000000 ) ;
#8403=CARTESIAN_POINT ( 'NONE',  ( -10.81189881249999729, 1.324075727343319199E-15, -116.0937500020483810 ) ) ;
#8405=CARTESIAN_POINT ( 'NONE',  ( 10.81189881249999729, 0.000000000000000000, -4.531250002048375691 ) ) ;
#8408=CARTESIAN_POINT ( 'NONE',  ( 9.999999999999998224, 0.000000000000000000, -177.8750000040967905 ) ) ;
#8409=CARTESIAN_POINT ( 'NONE',  ( 7.644554776091147741E-16, 12.48450537969573659, -170.6562500020484094 ) ) ;
#8410=CARTESIAN_POINT ( 'NONE',  ( -9.999999999999998224, 1.224646799147353059E-15, -103.2500000000000000 ) ) ;
#8413=CARTESIAN_POINT ( 'NONE',  ( 10.81189881249999551, -6.242252689847874514, -53.96875000204838102 ) ) ;
#8415=CARTESIAN_POINT ( 'NONE',  ( -10.81189881249999907, -6.242252689847864744, -3.656250002048349046 ) ) ;
#8417=CARTESIAN_POINT ( 'NONE',  ( 10.00000000000012257, -5.773502691896187144, -164.5000000040967905 ) ) ;
#8419=CARTESIAN_POINT ( 'NONE',  ( -9.999999999999998224, 5.773502691896259087, -98.87499999999998579 ) ) ;
#8421=CARTESIAN_POINT ( 'NONE',  ( -4.999999999999996447, 8.660254037844387298, -106.8750000040967763 ) ) ;
#8422=CARTESIAN_POINT ( 'NONE',  ( 9.999999999998969713, 5.773502691896851502, -82.87499999999995737 ) ) ;
#8425=CARTESIAN_POINT ( 'NONE',  ( 5.405949406249999534, 9.363379034771803333, -95.78125000204838102 ) ) ;
#8426=ORIENTED_EDGE ( 'NONE', *, *, #26529, .T. ) ;
#8429=CARTESIAN_POINT ( 'NONE',  ( 5.405949406249992428, -9.363379034771808662, -157.7812500020484094 ) ) ;
#8431=VERTEX_POINT ( 'NONE', #4617 ) ;
#8432=CARTESIAN_POINT ( 'NONE',  ( -2.121150477449813534E-15, -11.54700538379251284, -26.37499999999997868 ) ) ;
#8433=CARTESIAN_POINT ( 'NONE',  ( 7.644554776091147741E-16, 12.48450537969573659, -31.15625000204835260 ) ) ;
#8434=CARTESIAN_POINT ( 'NONE',  ( 7.070501591499377789E-16, 11.54700538379251284, -162.1250000000000284 ) ) ;
#8435=CYLINDRICAL_SURFACE ( 'NONE', #40733, 9.999999999999998224 ) ;
#8440=CARTESIAN_POINT ( 'NONE',  ( -2.293366432827344421E-15, -12.48450537969573659, -136.9062500020484094 ) ) ;
#8441=CARTESIAN_POINT ( 'NONE',  ( 8.143302022011770447, 6.762395603866230509, -7.434655202704447971E-15 ) ) ;
#8442=CARTESIAN_POINT ( 'NONE',  ( -9.999999999999998224, 1.224646799147353059E-15, -188.7500000000000000 ) ) ;
#8443=ORIENTED_EDGE ( 'NONE', *, *, #30940, .T. ) ;
#8444=CARTESIAN_POINT ( 'NONE',  ( -10.81189881249999729, 6.242252689847871849, -65.40625000204838102 ) ) ;
#8446=ORIENTED_EDGE ( 'NONE', *, *, #11221, .T. ) ;
#8447=ORIENTED_EDGE ( 'NONE', *, *, #11980, .T. ) ;
#8449=AXIS2_PLACEMENT_3D ( 'NONE', #173, #6629, #26275 ) ;
#8451=CARTESIAN_POINT ( 'NONE',  ( 10.81189881249999907, 6.242252689847868297, -155.7187500020483810 ) ) ;
#8453=CARTESIAN_POINT ( 'NONE',  ( -10.81189881249999729, 6.242252689847871849, -5.218750002048340164 ) ) ;
#8454=CARTESIAN_POINT ( 'NONE',  ( -5.405949406250003975, -9.363379034771801557, -148.8437500020483810 ) ) ;
#8455=CARTESIAN_POINT ( 'NONE',  ( 5.405949406249992428, -9.363379034771808662, -94.78125000204838102 ) ) ;
#8457=CARTESIAN_POINT ( 'NONE',  ( 4.999999999999992006, -8.660254037844389075, -161.2500000000000000 ) ) ;
#8459=CARTESIAN_POINT ( 'NONE',  ( -10.81189881249999729, 1.324075727343319199E-15, -0.5937500020483654772 ) ) ;
#8461=CARTESIAN_POINT ( 'NONE',  ( -5.405949406250003975, -9.363379034771801557, -191.0312500020484094 ) ) ;
#8466=CARTESIAN_POINT ( 'NONE',  ( -2.293366432827344421E-15, -12.48450537969573659, -78.21875000204838102 ) ) ;
#8467=CARTESIAN_POINT ( 'NONE',  ( 5.405949406249999534, 9.363379034771803333, -58.09375000204835970 ) ) ;
#8469=CARTESIAN_POINT ( 'NONE',  ( 5.405949406249992428, -9.363379034771808662, -36.28125000204837391 ) ) ;
#8472=CARTESIAN_POINT ( 'NONE',  ( -9.999999999999998224, 5.773502691896259087, -122.8750000000000142 ) ) ;
#8475=CARTESIAN_POINT ( 'NONE',  ( -10.81189881249999729, 6.242252689847871849, -6.906250002048365033 ) ) ;
#8479=CARTESIAN_POINT ( 'NONE',  ( 9.999999999999998224, 0.000000000000000000, -179.3750000040967905 ) ) ;
#8481=CARTESIAN_POINT ( 'NONE',  ( 7.070501591499377789E-16, 11.54700538379251284, -24.50000000409676204 ) ) ;
#8482=CARTESIAN_POINT ( 'NONE',  ( -9.999999999999998224, 1.224646799147353059E-15, -61.24999999999997158 ) ) ;
#8485=CARTESIAN_POINT ( 'NONE',  ( -10.81189881249999729, 1.324075727343319199E-15, -146.2812500020483810 ) ) ;
#8486=CARTESIAN_POINT ( 'NONE',  ( -2.293366432827344421E-15, -12.48450537969573659, -127.7187500020483668 ) ) ;
#8487=CARTESIAN_POINT ( 'NONE',  ( -9.999999999999998224, 1.224646799147353059E-15, -190.2500000000000000 ) ) ;
#8488=ADVANCED_FACE ( 'NONE', ( #31176 ), #14735, .T. ) ;
#8489=CARTESIAN_POINT ( 'NONE',  ( -9.999999999999998224, 1.224646799147353059E-15, -6.125000004096770034 ) ) ;
#8490=ORIENTED_EDGE ( 'NONE', *, *, #21256, .F. ) ;
#8491=EDGE_LOOP ( 'NONE', ( #18877, #38420, #27482, #13753 ) ) ;
#8493=CARTESIAN_POINT ( 'NONE',  ( -10.81189881249999907, -6.242252689847864744, -181.9687500020484094 ) ) ;
#8494=CARTESIAN_POINT ( 'NONE',  ( -5.405949406250003975, -9.363379034771801557, -31.84375000204836681 ) ) ;
#8495=DIRECTION ( 'NONE',  ( 1.000000000000000000, 0.000000000000000000, 0.000000000000000000 ) ) ;
#8496=CARTESIAN_POINT ( 'NONE',  ( 10.81189881249999729, 0.000000000000000000, -175.3437500020483810 ) ) ;
#8497=CARTESIAN_POINT ( 'NONE',  ( -5.405949406250003975, -9.363379034771801557, -151.8437500020483810 ) ) ;
#8498=CARTESIAN_POINT ( 'NONE',  ( 5.000000000000000000, 8.660254037844385522, -178.7500000000000284 ) ) ;
#8501=( BOUNDED_CURVE ( )  B_SPLINE_CURVE ( 2, ( #42286, #30584, #40264, #1015, #25906, #39057, #9496 ),
 .UNSPECIFIED., .F., .F. ) 
 B_SPLINE_CURVE_WITH_KNOTS ( ( 3, 2, 2, 3 ),
 ( 0.1194029850746269744, 0.1206467661691543042, 0.1218905472636816062, 0.1231343283582089221 ),
 .UNSPECIFIED. ) 
 CURVE ( )  GEOMETRIC_REPRESENTATION_ITEM ( )  RATIONAL_B_SPLINE_CURVE ( ( 0.9999999999999880096, 0.8660254037844506980, 1.000000000000000000, 0.8660254037844387076, 1.000000000000000000, 0.8660254037844417052, 0.9999999999999970024 ) ) 
 REPRESENTATION_ITEM ( '' )  );
#8505=CARTESIAN_POINT ( 'NONE',  ( -5.405949406249996869, 9.363379034771805109, -83.34375000204836681 ) ) ;
#8506=CARTESIAN_POINT ( 'NONE',  ( -9.999999999999998224, 1.224646799147353059E-15, -82.62500000409676204 ) ) ;
#8507=CARTESIAN_POINT ( 'NONE',  ( 7.644554776091147741E-16, 12.48450537969573659, -56.65625000204838102 ) ) ;
#8510=CARTESIAN_POINT ( 'NONE',  ( 5.405949406249992428, -9.363379034771808662, -117.2812500020483952 ) ) ;
#8511=CARTESIAN_POINT ( 'NONE',  ( 7.644554776091147741E-16, 12.48450537969573659, -146.6562500020484094 ) ) ;
#8512=DIRECTION ( 'NONE',  ( -0.000000000000000000, -0.000000000000000000, 1.000000000000000000 ) ) ;
#8514=CARTESIAN_POINT ( 'NONE',  ( -2.121150477449813534E-15, -11.54700538379251284, -118.2500000040968047 ) ) ;
#8519=CARTESIAN_POINT ( 'NONE',  ( 5.000000000000000000, 8.660254037844385522, -192.6250000040967905 ) ) ;
#8520=CARTESIAN_POINT ( 'NONE',  ( 10.81189881249999551, -6.242252689847874514, -184.6562500020484094 ) ) ;
#8523=CARTESIAN_POINT ( 'NONE',  ( -5.000000000000003553, -8.660254037844383745, -56.87500000409676204 ) ) ;
#8529=FACE_OUTER_BOUND ( 'NONE', #27731, .T. ) ;
#8530=CARTESIAN_POINT ( 'NONE',  ( 7.644554776091147741E-16, 12.48450537969573659, -169.1562500020484094 ) ) ;
#8531=DIRECTION ( 'NONE',  ( 0.6123724356957962467, -0.3535533905932744525, 0.7071067811865456854 ) ) ;
#8532=DIRECTION ( 'NONE',  ( 0.000000000000000000, 0.000000000000000000, -1.000000000000000000 ) ) ;
#8533=EDGE_CURVE ( 'NONE', #107, #19501, #12476, .T. ) ;
#8536=EDGE_CURVE ( 'NONE', #16036, #4388, #25743, .T. ) ;
#8539=CARTESIAN_POINT ( 'NONE',  ( -4.999999999999996447, 8.660254037844387298, -195.3750000040967905 ) ) ;
#8540=CARTESIAN_POINT ( 'NONE',  ( 10.81189881249999907, 6.242252689847868297, -77.90625000204836681 ) ) ;
#8543=CARTESIAN_POINT ( 'NONE',  ( -2.121150477449813534E-15, -11.54700538379251284, -119.3749999999999858 ) ) ;
#8546=EDGE_LOOP ( 'NONE', ( #16230, #29599, #8443, #24742 ) ) ;
#8547=CARTESIAN_POINT ( 'NONE',  ( 7.644554776091147741E-16, 12.48450537969573659, -36.96875000204835970 ) ) ;
#8548=CARTESIAN_POINT ( 'NONE',  ( -9.999999999999998224, 1.224646799147353059E-15, -49.24999999999998579 ) ) ;
#8549=CARTESIAN_POINT ( 'NONE',  ( -2.293366432827344421E-15, -12.48450537969573659, -9.406250002048375691 ) ) ;
#8550=CARTESIAN_POINT ( 'NONE',  ( -10.81189881249999729, 6.242252689847871849, -62.21875000204838813 ) ) ;
#8551=ORIENTED_EDGE ( 'NONE', *, *, #24095, .T. ) ;
#8554=EDGE_CURVE ( 'NONE', #41628, #11855, #14090, .T. ) ;
#8555=CARTESIAN_POINT ( 'NONE',  ( -10.81189881249999729, -6.242252689847864744, -196.9687500020484094 ) ) ;
#8556=CARTESIAN_POINT ( 'NONE',  ( 10.81189881249999907, 6.242252689847868297, -176.7187500020483810 ) ) ;
#8561=EDGE_CURVE ( 'NONE', #32336, #26629, #2303, .T. ) ;
#8563=CARTESIAN_POINT ( 'NONE',  ( 7.644554776091147741E-16, 12.48450537969573659, -108.9687500020483952 ) ) ;
#8565=CARTESIAN_POINT ( 'NONE',  ( 10.81189881249999551, -6.242252689847874514, -84.15625000204838102 ) ) ;
#8566=CARTESIAN_POINT ( 'NONE',  ( -5.405949406250003975, -9.363379034771801557, -90.34375000204838102 ) ) ;
#8568=CARTESIAN_POINT ( 'NONE',  ( 9.999999999999998224, 0.000000000000000000, -152.3750000040967905 ) ) ;
#8572=CARTESIAN_POINT ( 'NONE',  ( -2.121150477449813534E-15, -11.54700538379251284, -39.87499999999996447 ) ) ;
#8575=VERTEX_POINT ( 'NONE', #41708 ) ;
#8576=CARTESIAN_POINT ( 'NONE',  ( -4.999999999999996447, 8.660254037844387298, -65.99999999999997158 ) ) ;
#8578=CARTESIAN_POINT ( 'NONE',  ( -9.999999999999998224, 1.224646799147353059E-15, -79.62500000409677625 ) ) ;
#8579=EDGE_CURVE ( 'NONE', #9067, #38736, #15254, .T. ) ;
#8581=CYLINDRICAL_SURFACE ( 'NONE', #24518, 9.999999999999998224 ) ;
#8583=CARTESIAN_POINT ( 'NONE',  ( -10.81189881249999729, 1.324075727343319199E-15, -75.78125000204838102 ) ) ;
#8585=CARTESIAN_POINT ( 'NONE',  ( -9.999999999999479527, -5.773502691896549521, -78.00000000409676204 ) ) ;
#8588=CARTESIAN_POINT ( 'NONE',  ( -2.293366432827344421E-15, -12.48450537969573659, -196.9062500020484094 ) ) ;
#8590=CARTESIAN_POINT ( 'NONE',  ( 10.81189881249999551, -6.242252689847874514, -5.968750002048344605 ) ) ;
#8592=CARTESIAN_POINT ( 'NONE',  ( -10.81189881249999907, -6.242252689847864744, -144.4687500020484094 ) ) ;
#8593=CARTESIAN_POINT ( 'NONE',  ( 9.999999999999998224, 0.000000000000000000, -192.5000000000000000 ) ) ;
#8595=CARTESIAN_POINT ( 'NONE',  ( -5.000000000000003553, -8.660254037844383745, -179.5000000000000000 ) ) ;
#8596=CARTESIAN_POINT ( 'NONE',  ( -9.999999999999998224, 1.224646799147353059E-15, -3.125000004096767370 ) ) ;
#8597=CARTESIAN_POINT ( 'NONE',  ( -5.405949406249996869, 9.363379034771805109, -100.0312500020483952 ) ) ;
#8598=EDGE_LOOP ( 'NONE', ( #39309, #11953, #27811, #40894 ) ) ;
#8599=CARTESIAN_POINT ( 'NONE',  ( -5.000000000000003553, -8.660254037844383745, -164.5000000000000000 ) ) ;
#8602=ORIENTED_EDGE ( 'NONE', *, *, #16822, .F. ) ;
#8603=CARTESIAN_POINT ( 'NONE',  ( 5.405949406249992428, -9.363379034771808662, -27.28125000204836681 ) ) ;
#8605=EDGE_CURVE ( 'NONE', #42167, #10458, #9137, .T. ) ;
#8606=CARTESIAN_POINT ( 'NONE',  ( -5.405949406249996869, 9.363379034771805109, -83.34375000204836681 ) ) ;
#8611=CARTESIAN_POINT ( 'NONE',  ( -4.999999999999996447, 8.660254037844387298, -10.87500000409674605 ) ) ;
#8612=CARTESIAN_POINT ( 'NONE',  ( -2.293366432827344421E-15, -12.48450537969573659, -117.2187500020483668 ) ) ;
#8614=CARTESIAN_POINT ( 'NONE',  ( 10.81189881249999551, -6.242252689847874514, -6.156250002048360592 ) ) ;
#8617=CARTESIAN_POINT ( 'NONE',  ( 9.999999999999996447, -5.773502691896262640, -178.0000000040967905 ) ) ;
#8618=CARTESIAN_POINT ( 'NONE',  ( -5.405949406249996869, 9.363379034771805109, -167.5312500020484094 ) ) ;
#8619=CARTESIAN_POINT ( 'NONE',  ( 7.070501591499376803E-16, 11.54700538379251284, -102.5000000040967905 ) ) ;
#8622=CARTESIAN_POINT ( 'NONE',  ( 7.644554776091147741E-16, 12.48450537969573659, -45.96875000204837391 ) ) ;
#8624=CARTESIAN_POINT ( 'NONE',  ( 10.81189881249999907, 6.242252689847868297, -4.406250002048352599 ) ) ;
#8626=CARTESIAN_POINT ( 'NONE',  ( 9.999999999999998224, 0.000000000000000000, -164.3750000040967905 ) ) ;
#8628=CARTESIAN_POINT ( 'NONE',  ( 4.999999999999992006, -8.660254037844389075, -90.74999999999998579 ) ) ;
#8630=CARTESIAN_POINT ( 'NONE',  ( -5.000000000000003553, -8.660254037844383745, -106.3750000040967763 ) ) ;
#8634=CARTESIAN_POINT ( 'NONE',  ( -10.81189881249999729, 6.242252689847871849, -99.90625000204839523 ) ) ;
#8635=ORIENTED_EDGE ( 'NONE', *, *, #17172, .T. ) ;
#8636=AXIS2_PLACEMENT_3D ( 'NONE', #38260, #38689, #15578 ) ;
#8638=CARTESIAN_POINT ( 'NONE',  ( -4.999999999999996447, 8.660254037844387298, -28.87500000409676204 ) ) ;
#8639=CARTESIAN_POINT ( 'NONE',  ( -10.81189881249999729, 6.242252689847871849, -155.4062500020483810 ) ) ;
#8642=CARTESIAN_POINT ( 'NONE',  ( 10.00000000000000000, 5.773502691896255534, -27.37499999999998579 ) ) ;
#8643=CARTESIAN_POINT ( 'NONE',  ( -5.405949406249996869, 9.363379034771805109, -29.53125000204837036 ) ) ;
#8644=CARTESIAN_POINT ( 'NONE',  ( -5.000000000000003553, -8.660254037844383745, -157.0000000000000000 ) ) ;
#8646=( BOUNDED_CURVE ( )  B_SPLINE_CURVE ( 2, ( #15464, #22177, #35349, #29714, #16299, #32736, #32949 ),
 .UNSPECIFIED., .F., .F. ) 
 B_SPLINE_CURVE_WITH_KNOTS ( ( 3, 2, 2, 3 ),
 ( 0.6753731343283584376, 0.6766169154228858229, 0.6778606965174133192, 0.6791044776119405935 ),
 .UNSPECIFIED. ) 
 CURVE ( )  GEOMETRIC_REPRESENTATION_ITEM ( )  RATIONAL_B_SPLINE_CURVE ( ( 0.9999999999999761302, 0.8660254037844625774, 1.000000000000000000, 0.8660254037844387076, 1.000000000000000000, 0.8660254037844028474, 1.000000000000035971 ) ) 
 REPRESENTATION_ITEM ( '' )  );
#8647=CARTESIAN_POINT ( 'NONE',  ( 10.00000000000051159, -5.773502691895965988, -80.50000000409674783 ) ) ;
#8648=CARTESIAN_POINT ( 'NONE',  ( -10.81189881249999907, -6.242252689847864744, -122.1562500020484094 ) ) ;
#8649=CARTESIAN_POINT ( 'NONE',  ( -10.00000000000076916, 5.773502691895813221, -110.8749999999999574 ) ) ;
#8651=AXIS2_PLACEMENT_3D ( 'NONE', #22061, #28761, #29379 ) ;
#8654=CARTESIAN_POINT ( 'NONE',  ( 10.81189881249999729, 0.000000000000000000, -63.03125000204837391 ) ) ;
#8656=EDGE_CURVE ( 'NONE', #27948, #6661, #16624, .T. ) ;
#8657=CARTESIAN_POINT ( 'NONE',  ( -5.405949406250003975, -9.363379034771801557, -108.3437500020483810 ) ) ;
#8658=VERTEX_POINT ( 'NONE', #8718 ) ;
#8661=CARTESIAN_POINT ( 'NONE',  ( 10.81189881249999551, -6.242252689847874514, -157.4687500020484094 ) ) ;
#8663=CARTESIAN_POINT ( 'NONE',  ( 5.405949406249999534, 9.363379034771803333, -5.593750002048370362 ) ) ;
#8664=CARTESIAN_POINT ( 'NONE',  ( 10.81189881249999729, 6.242252689847867408, -136.2187500020483810 ) ) ;
#8666=CARTESIAN_POINT ( 'NONE',  ( -4.999999999999996447, 8.660254037844387298, -55.49999999999996447 ) ) ;
#8668=CARTESIAN_POINT ( 'NONE',  ( 5.405949406249992428, -9.363379034771808662, -0.09375000204836503315 ) ) ;
#8670=EDGE_CURVE ( 'NONE', #23066, #10458, #3420, .T. ) ;
#8671=CARTESIAN_POINT ( 'NONE',  ( 10.81189881249999551, -6.242252689847874514, -190.6562500020484094 ) ) ;
#8675=CARTESIAN_POINT ( 'NONE',  ( 10.81189881249999551, -6.242252689847874514, -64.46875000204838102 ) ) ;
#8676=CARTESIAN_POINT ( 'NONE',  ( 10.81189881249999729, 0.000000000000000000, -55.34375000204835970 ) ) ;
#8678=CARTESIAN_POINT ( 'NONE',  ( -2.293366432827344421E-15, -12.48450537969573659, -27.40625000204838102 ) ) ;
#8682=CARTESIAN_POINT ( 'NONE',  ( -9.999999999999998224, 1.224646799147353059E-15, -115.2499999999999858 ) ) ;
#8683=CARTESIAN_POINT ( 'NONE',  ( 9.999999999999998224, 0.000000000000000000, -82.99999999999997158 ) ) ;
#8687=CARTESIAN_POINT ( 'NONE',  ( -5.405949406249996869, 9.363379034771805109, -13.03125000204835615 ) ) ;
#8689=CIRCLE ( 'NONE', #432, 10.00000000000000178 ) ;
#8691=CARTESIAN_POINT ( 'NONE',  ( -2.121150477449813534E-15, -11.54700538379251284, -86.75000000409677625 ) ) ;
#8693=CARTESIAN_POINT ( 'NONE',  ( -9.999999999999998224, 5.773502691896259087, -47.87499999999996447 ) ) ;
#8694=CARTESIAN_POINT ( 'NONE',  ( 9.999999999999998224, 0.000000000000000000, -29.37500000409676204 ) ) ;
#8696=CARTESIAN_POINT ( 'NONE',  ( 9.999999999999998224, 0.000000000000000000, -75.49999999999998579 ) ) ;
#8698=DIRECTION ( 'NONE',  ( -0.000000000000000000, -0.000000000000000000, 1.000000000000000000 ) ) ;
#8699=CARTESIAN_POINT ( 'NONE',  ( -10.81189881249999729, 6.242252689847871849, -146.4062500020484094 ) ) ;
#8700=CARTESIAN_POINT ( 'NONE',  ( 10.81189881249999729, 0.000000000000000000, -124.3437500020483952 ) ) ;
#8701=DIRECTION ( 'NONE',  ( -0.000000000000000000, -0.000000000000000000, 1.000000000000000000 ) ) ;
#8703=ORIENTED_EDGE ( 'NONE', *, *, #4732, .T. ) ;
#8704=EDGE_CURVE ( 'NONE', #14015, #36368, #6684, .T. ) ;
#8705=ORIENTED_EDGE ( 'NONE', *, *, #26212, .T. ) ;
#8707=CARTESIAN_POINT ( 'NONE',  ( -9.999999999999998224, 1.224646799147353059E-15, -40.24999999999997868 ) ) ;
#8708=CARTESIAN_POINT ( 'NONE',  ( -2.293366432827344421E-15, -12.48450537969573659, -178.7187500020484094 ) ) ;
#8709=CARTESIAN_POINT ( 'NONE',  ( 5.405949406249999534, 9.363379034771803333, -29.59375000204836326 ) ) ;
#8710=LINE ( 'NONE', #37841, #12941 ) ;
#8711=CARTESIAN_POINT ( 'NONE',  ( 10.81189881249999729, 6.242252689847867408, -167.7187500020483526 ) ) ;
#8712=CARTESIAN_POINT ( 'NONE',  ( -10.81189881249999729, 6.242252689847871849, -155.2187500020483810 ) ) ;
#8713=CARTESIAN_POINT ( 'NONE',  ( 0.000000000000000000, 0.000000000000000000, -200.0000000000000000 ) ) ;
#8717=CYLINDRICAL_SURFACE ( 'NONE', #17785, 9.999999999999998224 ) ;
#8718=CARTESIAN_POINT ( 'NONE',  ( 9.999999999999998224, 0.000000000000000000, -81.49999999999998579 ) ) ;
#8720=CARTESIAN_POINT ( 'NONE',  ( -10.81189881249999729, 1.324075727343319199E-15, -78.59375000204838102 ) ) ;
#8721=CYLINDRICAL_SURFACE ( 'NONE', #38268, 9.999999999999998224 ) ;
#8722=CARTESIAN_POINT ( 'NONE',  ( 10.81189881249999729, 0.000000000000000000, -48.03125000204838813 ) ) ;
#8724=EDGE_CURVE ( 'NONE', #22389, #12029, #26177, .T. ) ;
#8726=CARTESIAN_POINT ( 'NONE',  ( -5.405949406249996869, 9.363379034771805109, -112.0312500020483810 ) ) ;
#8727=CARTESIAN_POINT ( 'NONE',  ( -5.405949406249996869, 9.363379034771805109, -143.5312500020483810 ) ) ;
#8728=CARTESIAN_POINT ( 'NONE',  ( -9.999999999999998224, 1.224646799147353059E-15, -195.1250000040967905 ) ) ;
#8730=CARTESIAN_POINT ( 'NONE',  ( 9.999999999999996447, -5.773502691896262640, -125.5000000040967763 ) ) ;
#8732=ORIENTED_EDGE ( 'NONE', *, *, #6620, .T. ) ;
#8735=LINE ( 'NONE', #24720, #28468 ) ;
#8736=CARTESIAN_POINT ( 'NONE',  ( -5.405949406250003975, -9.363379034771801557, -183.5312500020484094 ) ) ;
#8739=CARTESIAN_POINT ( 'NONE',  ( -10.00000000000000000, -5.773502691896251982, -46.50000000409676915 ) ) ;
#8740=CARTESIAN_POINT ( 'NONE',  ( 0.000000000000000000, 0.000000000000000000, -200.0000000000000000 ) ) ;
#8744=CARTESIAN_POINT ( 'NONE',  ( -10.81189881249999729, 1.324075727343319199E-15, -167.2812500020484094 ) ) ;
#8745=CARTESIAN_POINT ( 'NONE',  ( -9.999999999999998224, 1.224646799147353059E-15, -1.625000004096766038 ) ) ;
#8747=FACE_OUTER_BOUND ( 'NONE', #12503, .T. ) ;
#8748=CARTESIAN_POINT ( 'NONE',  ( -11.54700538379251817, 20.00000000000000355, 49.99999999999998579 ) ) ;
#8749=CARTESIAN_POINT ( 'NONE',  ( -4.999999999999996447, 8.660254037844387298, -136.8750000040967905 ) ) ;
#8750=CARTESIAN_POINT ( 'NONE',  ( -5.405949406250003975, -9.363379034771801557, -81.53125000204839523 ) ) ;
#8752=EDGE_LOOP ( 'NONE', ( #18216, #6519, #15813, #40254 ) ) ;
#8753=ORIENTED_EDGE ( 'NONE', *, *, #34357, .T. ) ;
#8754=( BOUNDED_CURVE ( )  B_SPLINE_CURVE ( 2, ( #37291, #30620, #33646, #26524, #4069, #13963, #29771 ),
 .UNSPECIFIED., .F., .F. ) 
 B_SPLINE_CURVE_WITH_KNOTS ( ( 3, 2, 2, 3 ),
 ( 0.07089552238805976736, 0.07213930348258713876, 0.07338308457711449628, 0.07462686567164185381 ),
 .UNSPECIFIED. ) 
 CURVE ( )  GEOMETRIC_REPRESENTATION_ITEM ( )  RATIONAL_B_SPLINE_CURVE ( ( 0.9999999999999925615, 0.8660254037844461461, 1.000000000000000000, 0.8660254037844387076, 1.000000000000000000, 0.8660254037844312691, 1.000000000000007550 ) ) 
 REPRESENTATION_ITEM ( '' )  );
#8755=CARTESIAN_POINT ( 'NONE',  ( 10.81189881249999729, 0.000000000000000000, -31.34375000204836681 ) ) ;
#8757=CARTESIAN_POINT ( 'NONE',  ( -5.405949406250003975, -9.363379034771801557, -3.531250002048374803 ) ) ;
#8758=CARTESIAN_POINT ( 'NONE',  ( -5.405949406250003975, -9.363379034771801557, -52.84375000204835970 ) ) ;
#8759=ORIENTED_EDGE ( 'NONE', *, *, #37817, .F. ) ;
#8760=CARTESIAN_POINT ( 'NONE',  ( 9.999999999999998224, 0.000000000000000000, -3.499999999999975131 ) ) ;
#8762=CARTESIAN_POINT ( 'NONE',  ( -2.293366432827344421E-15, -12.48450537969573659, -184.7187500020484094 ) ) ;
#8763=CARTESIAN_POINT ( 'NONE',  ( -10.81189881249999729, 6.242252689847871849, -177.7187500020483810 ) ) ;
#8769=CARTESIAN_POINT ( 'NONE',  ( 5.405949406249992428, -9.363379034771808662, -102.0937500020483810 ) ) ;
#8770=CARTESIAN_POINT ( 'NONE',  ( 0.000000000000000000, 0.000000000000000000, -200.0000000000000000 ) ) ;
#8771=CARTESIAN_POINT ( 'NONE',  ( 10.81189881249999729, 0.000000000000000000, -79.53125000204838102 ) ) ;
#8773=CARTESIAN_POINT ( 'NONE',  ( -5.405949406249996869, 9.363379034771805109, -95.34375000204838102 ) ) ;
#8774=ADVANCED_FACE ( 'NONE', ( #19684 ), #3727, .T. ) ;
#8776=CARTESIAN_POINT ( 'NONE',  ( 7.070501591499377789E-16, 11.54700538379251284, -149.0000000040968189 ) ) ;
#8780=CARTESIAN_POINT ( 'NONE',  ( 9.999999999999479527, 5.773502691896553074, -98.25000000409676204 ) ) ;
#8781=CARTESIAN_POINT ( 'NONE',  ( 0.000000000000000000, 0.000000000000000000, -200.0000000000000000 ) ) ;
#8784=CARTESIAN_POINT ( 'NONE',  ( 7.070501591499377789E-16, 11.54700538379251284, -63.12499999999997158 ) ) ;
#8786=CARTESIAN_POINT ( 'NONE',  ( 9.999999999999996447, -5.773502691896262640, -73.00000000409676204 ) ) ;
#8787=CARTESIAN_POINT ( 'NONE',  ( -9.999999999999998224, 1.224646799147353059E-15, -175.6250000040968189 ) ) ;
#8789=CARTESIAN_POINT ( 'NONE',  ( -5.405949406250003975, -9.363379034771801557, -75.53125000204838102 ) ) ;
#8793=ORIENTED_EDGE ( 'NONE', *, *, #40131, .T. ) ;
#8794=CARTESIAN_POINT ( 'NONE',  ( 10.81189881249999907, 6.242252689847868297, -193.4062500020484094 ) ) ;
#8796=CARTESIAN_POINT ( 'NONE',  ( -5.405949406250003975, -9.363379034771801557, -3.343750002048367698 ) ) ;
#8797=CARTESIAN_POINT ( 'NONE',  ( 0.000000000000000000, 0.000000000000000000, -200.0000000000000000 ) ) ;
#8798=EDGE_CURVE ( 'NONE', #15872, #4341, #6743, .T. ) ;
#8799=CARTESIAN_POINT ( 'NONE',  ( 4.999999999999992006, -8.660254037844389075, -107.6250000040967763 ) ) ;
#8800=LINE ( 'NONE', #38790, #30059 ) ;
#8801=CARTESIAN_POINT ( 'NONE',  ( 9.999999999999998224, 0.000000000000000000, -173.0000000000000284 ) ) ;
#8802=CARTESIAN_POINT ( 'NONE',  ( 9.999999999999998224, 0.000000000000000000, -176.3750000040967905 ) ) ;
#8803=CARTESIAN_POINT ( 'NONE',  ( 10.81189881249999551, -6.242252689847874514, -103.6562500020483668 ) ) ;
#8804=ORIENTED_EDGE ( 'NONE', *, *, #36914, .T. ) ;
#8806=EDGE_CURVE ( 'NONE', #38258, #25635, #22963, .T. ) ;
#8808=EDGE_LOOP ( 'NONE', ( #13232, #15418, #36641, #23217 ) ) ;
#8809=CARTESIAN_POINT ( 'NONE',  ( 10.81189881249999907, 6.242252689847868297, -28.40625000204838813 ) ) ;
#8811=CARTESIAN_POINT ( 'NONE',  ( -10.81189881249999907, -6.242252689847864744, -81.46875000204838102 ) ) ;
#8812=FACE_OUTER_BOUND ( 'NONE', #15212, .T. ) ;
#8814=VECTOR ( 'NONE', #4454, 1000.000000000000000 ) ;
#8815=CARTESIAN_POINT ( 'NONE',  ( 10.81189881249999729, 0.000000000000000000, -199.3437500020484094 ) ) ;
#8818=CARTESIAN_POINT ( 'NONE',  ( 5.000000000000000000, 8.660254037844385522, -12.62500000409674783 ) ) ;
#8819=DIRECTION ( 'NONE',  ( -0.000000000000000000, -0.000000000000000000, 1.000000000000000000 ) ) ;
#8820=CARTESIAN_POINT ( 'NONE',  ( 10.81189881249999729, 0.000000000000000000, -127.3437500020483952 ) ) ;
#8822=CARTESIAN_POINT ( 'NONE',  ( -5.405949406249996869, 9.363379034771805109, -119.3437500020483810 ) ) ;
#8826=CARTESIAN_POINT ( 'NONE',  ( 5.000000000000000000, 8.660254037844385522, -173.1250000040968189 ) ) ;
#8827=CARTESIAN_POINT ( 'NONE',  ( -5.405949406250003975, -9.363379034771801557, -168.5312500020484094 ) ) ;
#8828=EDGE_CURVE ( 'NONE', #14871, #4606, #8346, .T. ) ;
#8829=CARTESIAN_POINT ( 'NONE',  ( 9.999999999999998224, 0.000000000000000000, -102.8750000040967763 ) ) ;
#8832=CARTESIAN_POINT ( 'NONE',  ( 10.81189881249999729, 6.242252689847867408, -41.71875000204835260 ) ) ;
#8833=ADVANCED_FACE ( 'NONE', ( #3300 ), #26387, .T. ) ;
#8835=CARTESIAN_POINT ( 'NONE',  ( 10.81189881249999907, 6.242252689847868297, -1.406250002048370584 ) ) ;
#8839=CARTESIAN_POINT ( 'NONE',  ( 10.00000000000000000, 5.773502691896255534, -90.37499999999998579 ) ) ;
#8841=CARTESIAN_POINT ( 'NONE',  ( 9.999999999999996447, -5.773502691896262640, -103.0000000040967620 ) ) ;
#8842=CARTESIAN_POINT ( 'NONE',  ( -5.000000000000003553, -8.660254037844383745, -149.8750000040967905 ) ) ;
#8844=CARTESIAN_POINT ( 'NONE',  ( 5.405949406249992428, -9.363379034771808662, -97.78125000204839523 ) ) ;
#8845=ORIENTED_EDGE ( 'NONE', *, *, #35327, .F. ) ;
#8847=CARTESIAN_POINT ( 'NONE',  ( -9.999999999999998224, 1.224646799147353059E-15, -134.7499999999999716 ) ) ;
#8848=CARTESIAN_POINT ( 'NONE',  ( 5.405949406249992428, -9.363379034771808662, -159.2812500020484094 ) ) ;
#8850=VERTEX_POINT ( 'NONE', #36098 ) ;
#8851=CARTESIAN_POINT ( 'NONE',  ( -5.000000000000003553, -8.660254037844383745, -15.99999999999995914 ) ) ;
#8852=CARTESIAN_POINT ( 'NONE',  ( 5.405949406249992428, -9.363379034771808662, -27.28125000204836681 ) ) ;
#8853=CARTESIAN_POINT ( 'NONE',  ( 10.00000000000000000, 5.773502691896255534, -151.8750000000000000 ) ) ;
#8855=( BOUNDED_CURVE ( )  B_SPLINE_CURVE ( 2, ( #14804, #17404, #17834, #40489, #34484, #24128, #4906 ),
 .UNSPECIFIED., .F., .F. ) 
 B_SPLINE_CURVE_WITH_KNOTS ( ( 3, 2, 2, 3 ),
 ( 0.9402985074626868389, 0.9415422885572141132, 0.9427860696517416095, 0.9440298507462689948 ),
 .UNSPECIFIED. ) 
 CURVE ( )  GEOMETRIC_REPRESENTATION_ITEM ( )  RATIONAL_B_SPLINE_CURVE ( ( 0.9999999999999761302, 0.8660254037844625774, 1.000000000000000000, 0.8660254037844387076, 1.000000000000000000, 0.8660254037844028474, 1.000000000000035971 ) ) 
 REPRESENTATION_ITEM ( '' )  );
#8858=CARTESIAN_POINT ( 'NONE',  ( 9.999999999999996447, -5.773502691896262640, -195.6250000000000284 ) ) ;
#8859=CARTESIAN_POINT ( 'NONE',  ( 5.405949406249999534, 9.363379034771803333, -128.7812500020483810 ) ) ;
#8861=CARTESIAN_POINT ( 'NONE',  ( 4.999999999999992006, -8.660254037844389075, -188.2500000000000000 ) ) ;
#8862=ORIENTED_EDGE ( 'NONE', *, *, #31488, .T. ) ;
#8863=CARTESIAN_POINT ( 'NONE',  ( -5.405949406250003975, -9.363379034771801557, -56.03125000204836681 ) ) ;
#8865=CARTESIAN_POINT ( 'NONE',  ( -5.405949406249996869, 9.363379034771805109, -107.3437500020483810 ) ) ;
#8868=CYLINDRICAL_SURFACE ( 'NONE', #16246, 9.999999999999998224 ) ;
#8869=CARTESIAN_POINT ( 'NONE',  ( -9.999999999999998224, 1.224646799147353059E-15, -164.7500000000000000 ) ) ;
#8870=CARTESIAN_POINT ( 'NONE',  ( 5.405949406249992428, -9.363379034771808662, -159.0937500020484094 ) ) ;
#8872=CARTESIAN_POINT ( 'NONE',  ( 10.81189881249999729, 0.000000000000000000, -5.843750002048370362 ) ) ;
#8873=CARTESIAN_POINT ( 'NONE',  ( -2.293366432827344421E-15, -12.48450537969573659, -142.7187500020483810 ) ) ;
#8874=VECTOR ( 'NONE', #39498, 1000.000000000000000 ) ;
#8878=CARTESIAN_POINT ( 'NONE',  ( -2.121150477449813534E-15, -11.54700538379251284, -193.2500000040968473 ) ) ;
#8880=CARTESIAN_POINT ( 'NONE',  ( -5.405949406249996869, 9.363379034771805109, -194.5312500020484094 ) ) ;
#8881=CARTESIAN_POINT ( 'NONE',  ( 9.999999999999998224, 0.000000000000000000, -5.375000004096769146 ) ) ;
#8884=CARTESIAN_POINT ( 'NONE',  ( 5.405949406249992428, -9.363379034771808662, -67.59375000204836681 ) ) ;
#8885=CARTESIAN_POINT ( 'NONE',  ( -5.405949406250003975, -9.363379034771801557, -57.34375000204835970 ) ) ;
#8887=CARTESIAN_POINT ( 'NONE',  ( -10.81189881249999729, 6.242252689847871849, -24.90625000204838813 ) ) ;
#8891=CARTESIAN_POINT ( 'NONE',  ( 7.070501591499377789E-16, 11.54700538379251284, -117.1249999999999858 ) ) ;
#8894=CARTESIAN_POINT ( 'NONE',  ( 7.644554776091147741E-16, 12.48450537969573659, -11.65625000204835438 ) ) ;
#8895=ORIENTED_EDGE ( 'NONE', *, *, #4965, .F. ) ;
#8898=CARTESIAN_POINT ( 'NONE',  ( -9.999999999999998224, 1.224646799147353059E-15, -39.12500000409676915 ) ) ;
#8900=CARTESIAN_POINT ( 'NONE',  ( 7.070501591499377789E-16, 11.54700538379251284, -39.12499999999996447 ) ) ;
#8902=CARTESIAN_POINT ( 'NONE',  ( 9.999999999999996447, -5.773502691896262640, -29.50000000409675494 ) ) ;
#8906=CARTESIAN_POINT ( 'NONE',  ( -9.999999999999998224, 1.224646799147353059E-15, -43.24999999999998579 ) ) ;
#8907=CARTESIAN_POINT ( 'NONE',  ( -2.293366432827344421E-15, -12.48450537969573659, -142.9062500020483810 ) ) ;
#8908=CARTESIAN_POINT ( 'NONE',  ( -5.405949406249996869, 9.363379034771805109, -146.5312500020483810 ) ) ;
#8910=VECTOR ( 'NONE', #12818, 1000.000000000000000 ) ;
#8911=CARTESIAN_POINT ( 'NONE',  ( -9.999999999999998224, 1.224646799147353059E-15, -178.2500000000000284 ) ) ;
#8912=VERTEX_POINT ( 'NONE', #17285 ) ;
#8914=ORIENTED_EDGE ( 'NONE', *, *, #23902, .T. ) ;
#8915=VERTEX_POINT ( 'NONE', #21175 ) ;
#8917=CARTESIAN_POINT ( 'NONE',  ( 5.405949406249992428, -9.363379034771808662, -184.5937500020483810 ) ) ;
#8919=CARTESIAN_POINT ( 'NONE',  ( -2.293366432827344421E-15, -12.48450537969573659, -28.71875000204835615 ) ) ;
#8921=CARTESIAN_POINT ( 'NONE',  ( -10.81189881249999729, 1.324075727343319199E-15, -164.0937500020484094 ) ) ;
#8922=CARTESIAN_POINT ( 'NONE',  ( 5.405949406249999534, 9.363379034771803333, -152.5937500020483810 ) ) ;
#8923=CARTESIAN_POINT ( 'NONE',  ( 10.90460581041948984, 0.09205482696659748887, -1.027162637006526080E-30 ) ) ;
#8928=CARTESIAN_POINT ( 'NONE',  ( -4.999999999999996447, 8.660254037844387298, -129.0000000000000000 ) ) ;
#8929=CARTESIAN_POINT ( 'NONE',  ( -4.999999999999996447, 8.660254037844387298, -183.0000000000000000 ) ) ;
#8931=CARTESIAN_POINT ( 'NONE',  ( 7.644554776091147741E-16, 12.48450537969573659, -77.46875000204838102 ) ) ;
#8933=CARTESIAN_POINT ( 'NONE',  ( 10.81189881249999729, 0.000000000000000000, -52.53125000204835970 ) ) ;
#8936=CARTESIAN_POINT ( 'NONE',  ( 4.999999999999992006, -8.660254037844389075, -138.7499999999999716 ) ) ;
#8937=CARTESIAN_POINT ( 'NONE',  ( 10.81189881249999551, -6.242252689847874514, -148.6562500020484094 ) ) ;
#8940=CARTESIAN_POINT ( 'NONE',  ( -9.999999999999998224, 5.773502691896259087, -123.2500000040967763 ) ) ;
#8942=ORIENTED_EDGE ( 'NONE', *, *, #41083, .T. ) ;
#8945=DIRECTION ( 'NONE',  ( -0.000000000000000000, -0.000000000000000000, 1.000000000000000000 ) ) ;
#8946=VECTOR ( 'NONE', #786, 1000.000000000000000 ) ;
#8947=CARTESIAN_POINT ( 'NONE',  ( 7.644554776091147741E-16, 12.48450537969573659, -176.6562500020484094 ) ) ;
#8948=CARTESIAN_POINT ( 'NONE',  ( 9.999999999999998224, 0.000000000000000000, -53.37500000409675494 ) ) ;
#8952=CARTESIAN_POINT ( 'NONE',  ( 0.000000000000000000, 0.000000000000000000, -200.0000000000000000 ) ) ;
#8953=CARTESIAN_POINT ( 'NONE',  ( 5.405949406249999534, 9.363379034771803333, -172.2812500020484094 ) ) ;
#8954=CYLINDRICAL_SURFACE ( 'NONE', #29780, 9.999999999999998224 ) ;
#8955=CARTESIAN_POINT ( 'NONE',  ( 0.000000000000000000, 0.000000000000000000, -200.0000000000000000 ) ) ;
#8957=VERTEX_POINT ( 'NONE', #36942 ) ;
#8958=FACE_OUTER_BOUND ( 'NONE', #21755, .T. ) ;
#8959=CARTESIAN_POINT ( 'NONE',  ( 4.999999999999992006, -8.660254037844389075, -52.12500000409675494 ) ) ;
#8960=CARTESIAN_POINT ( 'NONE',  ( -5.405949406249996869, 9.363379034771805109, -76.03125000204838102 ) ) ;
#8963=( BOUNDED_CURVE ( )  B_SPLINE_CURVE ( 2, ( #31034, #18271, #28005, #8371, #14599, #40922, #11365 ),
 .UNSPECIFIED., .F., .F. ) 
 B_SPLINE_CURVE_WITH_KNOTS ( ( 3, 2, 2, 3 ),
 ( 0.8582089552238808539, 0.8594527363184081281, 0.8606965174129356244, 0.8619402985074630097 ),
 .UNSPECIFIED. ) 
 CURVE ( )  GEOMETRIC_REPRESENTATION_ITEM ( )  RATIONAL_B_SPLINE_CURVE ( ( 0.9999999999999761302, 0.8660254037844625774, 1.000000000000000000, 0.8660254037844387076, 1.000000000000000000, 0.8660254037844028474, 1.000000000000035971 ) ) 
 REPRESENTATION_ITEM ( '' )  );
#8965=CARTESIAN_POINT ( 'NONE',  ( -10.81189881249999729, -6.242252689847864744, -28.96875000204835615 ) ) ;
#8966=CARTESIAN_POINT ( 'NONE',  ( -5.405949406250003975, -9.363379034771801557, -6.531250002048377468 ) ) ;
#8967=CARTESIAN_POINT ( 'NONE',  ( 10.81189881249999907, 6.242252689847868297, -55.21875000204836681 ) ) ;
#8968=ORIENTED_EDGE ( 'NONE', *, *, #40000, .T. ) ;
#8971=CARTESIAN_POINT ( 'NONE',  ( -5.405949406249996869, 9.363379034771805109, -188.3437500020483810 ) ) ;
#8972=CARTESIAN_POINT ( 'NONE',  ( 10.81189881249999551, -6.242252689847874514, -179.9687500020484094 ) ) ;
#8975=CARTESIAN_POINT ( 'NONE',  ( -4.999999999999996447, 8.660254037844387298, -124.5000000000000000 ) ) ;
#8978=CARTESIAN_POINT ( 'NONE',  ( -5.405949406250003975, -9.363379034771801557, -108.3437500020483810 ) ) ;
#8979=CARTESIAN_POINT ( 'NONE',  ( -5.000000000000003553, -8.660254037844383745, -47.87500000409677625 ) ) ;
#8980=CARTESIAN_POINT ( 'NONE',  ( 7.644554776091147741E-16, 12.48450537969573659, -76.15625000204839523 ) ) ;
#8981=CARTESIAN_POINT ( 'NONE',  ( -10.81189881249999729, 6.242252689847871849, -90.71875000204838102 ) ) ;
#8983=CARTESIAN_POINT ( 'NONE',  ( 4.999999999999992006, -8.660254037844389075, -148.1250000040967905 ) ) ;
#8988=DIRECTION ( 'NONE',  ( -0.000000000000000000, -0.000000000000000000, 1.000000000000000000 ) ) ;
#8989=CARTESIAN_POINT ( 'NONE',  ( 9.999999999999998224, 0.000000000000000000, -200.0000000000000000 ) ) ;
#8991=VERTEX_POINT ( 'NONE', #37149 ) ;
#8992=CARTESIAN_POINT ( 'NONE',  ( -4.999999999999996447, 8.660254037844387298, -64.49999999999997158 ) ) ;
#8994=CARTESIAN_POINT ( 'NONE',  ( -4.999999999999996447, 8.660254037844387298, -73.87500000409677625 ) ) ;
#8995=CARTESIAN_POINT ( 'NONE',  ( -4.999999999999996447, 8.660254037844387298, -102.0000000000000000 ) ) ;
#8996=DIRECTION ( 'NONE',  ( -0.000000000000000000, -0.000000000000000000, 1.000000000000000000 ) ) ;
#8998=CARTESIAN_POINT ( 'NONE',  ( 7.644554776091147741E-16, 12.48450537969573659, -67.15625000204839523 ) ) ;
#9002=ORIENTED_EDGE ( 'NONE', *, *, #25949, .F. ) ;
#9003=CARTESIAN_POINT ( 'NONE',  ( 10.81189881249999907, 6.242252689847868297, -191.9062500020484094 ) ) ;
#9004=AXIS2_PLACEMENT_3D ( 'NONE', #5783, #2759, #32121 ) ;
#9006=CARTESIAN_POINT ( 'NONE',  ( 10.81189881249999729, 0.000000000000000000, -8.843750002048345493 ) ) ;
#9007=CARTESIAN_POINT ( 'NONE',  ( -10.00000000000025580, 5.773502691896109873, -186.2500000040967905 ) ) ;
#9009=CARTESIAN_POINT ( 'NONE',  ( 9.999999999999998224, 0.000000000000000000, -159.8750000040967905 ) ) ;
#9010=( BOUNDED_CURVE ( )  B_SPLINE_CURVE ( 2, ( #3207, #9044, #6446, #39028, #42044, #13100, #16333 ),
 .UNSPECIFIED., .F., .F. ) 
 B_SPLINE_CURVE_WITH_KNOTS ( ( 3, 2, 2, 3 ),
 ( 0.3619402985074628432, 0.3631840796019901729, 0.3644278606965175027, 0.3656716417910448325 ),
 .UNSPECIFIED. ) 
 CURVE ( )  GEOMETRIC_REPRESENTATION_ITEM ( )  RATIONAL_B_SPLINE_CURVE ( ( 0.9999999999999820144, 0.8660254037844566932, 1.000000000000000000, 0.8660254037844387076, 1.000000000000000000, 0.8660254037844327124, 1.000000000000005995 ) ) 
 REPRESENTATION_ITEM ( '' )  );
#9011=CARTESIAN_POINT ( 'NONE',  ( 7.070501591499377789E-16, 11.54700538379251284, -172.6249999999999716 ) ) ;
#9012=DIRECTION ( 'NONE',  ( 1.000000000000000000, 0.000000000000000000, 0.000000000000000000 ) ) ;
#9013=CARTESIAN_POINT ( 'NONE',  ( -10.81189881249999907, -6.242252689847864744, -104.1562500020483668 ) ) ;
#9015=FACE_OUTER_BOUND ( 'NONE', #19294, .T. ) ;
#9016=EDGE_CURVE ( 'NONE', #32390, #14564, #27369, .T. ) ;
#9017=EDGE_LOOP ( 'NONE', ( #32592, #14618, #20037, #8895, #33117 ) ) ;
#9018=EDGE_CURVE ( 'NONE', #28714, #4880, #41968, .T. ) ;
#9020=CARTESIAN_POINT ( 'NONE',  ( -10.81189881249999729, 1.324075727343319199E-15, -29.28125000204837036 ) ) ;
#9022=CARTESIAN_POINT ( 'NONE',  ( -5.405949406250003975, -9.363379034771801557, -79.84375000204838102 ) ) ;
#9023=CARTESIAN_POINT ( 'NONE',  ( -9.999999999999998224, 1.224646799147353059E-15, -4.625000004096769146 ) ) ;
#9025=CARTESIAN_POINT ( 'NONE',  ( 5.000000000000000000, 8.660254037844385522, -69.62500000409677625 ) ) ;
#9028=CARTESIAN_POINT ( 'NONE',  ( 7.070501591499377789E-16, 11.54700538379251284, -11.00000000409676382 ) ) ;
#9030=CARTESIAN_POINT ( 'NONE',  ( -5.000000000000003553, -8.660254037844383745, -74.87500000409677625 ) ) ;
#9031=CARTESIAN_POINT ( 'NONE',  ( -10.81189881249999729, 1.324075727343319199E-15, -128.0937500020483810 ) ) ;
#9032=CARTESIAN_POINT ( 'NONE',  ( 5.405949406249999534, 9.363379034771803333, -119.5937500020483810 ) ) ;
#9035=CARTESIAN_POINT ( 'NONE',  ( -9.999999999999998224, 1.224646799147353059E-15, -171.1250000040968189 ) ) ;
#9036=CARTESIAN_POINT ( 'NONE',  ( -10.81189881249999729, 1.324075727343319199E-15, -168.7812500020484094 ) ) ;
#9037=CYLINDRICAL_SURFACE ( 'NONE', #8245, 9.999999999999998224 ) ;
#9040=CARTESIAN_POINT ( 'NONE',  ( -2.293366432827344421E-15, -12.48450537969573659, -46.71875000204835970 ) ) ;
#9042=CARTESIAN_POINT ( 'NONE',  ( -9.999999999999998224, 1.224646799147353059E-15, -85.62500000409677625 ) ) ;
#9044=CARTESIAN_POINT ( 'NONE',  ( -9.999999999999227285, -5.773502691896698735, -127.1249999999999574 ) ) ;
#9046=CARTESIAN_POINT ( 'NONE',  ( 7.070501591499377789E-16, 11.54700538379251284, -90.12499999999997158 ) ) ;
#9048=CARTESIAN_POINT ( 'NONE',  ( 9.999999999999996447, -5.773502691896262640, -101.5000000040967905 ) ) ;
#9050=CARTESIAN_POINT ( 'NONE',  ( -10.81189881249999729, -6.242252689847864744, -95.15625000204839523 ) ) ;
#9051=ORIENTED_EDGE ( 'NONE', *, *, #8704, .T. ) ;
#9053=CARTESIAN_POINT ( 'NONE',  ( -10.00000000000102496, 5.773502691895664007, -4.374999999999930722 ) ) ;
#9054=CARTESIAN_POINT ( 'NONE',  ( -5.405949406249996869, 9.363379034771805109, -158.5312500020484094 ) ) ;
#9057=CARTESIAN_POINT ( 'NONE',  ( 9.999999999999998224, 0.000000000000000000, -21.49999999999996447 ) ) ;
#9058=CARTESIAN_POINT ( 'NONE',  ( 10.81189881249999551, -6.242252689847874514, -25.65625000204838813 ) ) ;
#9059=CARTESIAN_POINT ( 'NONE',  ( 5.000000000000000000, 8.660254037844385522, -150.2500000000000000 ) ) ;
#9063=CARTESIAN_POINT ( 'NONE',  ( -10.81189881249999729, 6.242252689847871849, -126.9062500020483810 ) ) ;
#9064=ORIENTED_EDGE ( 'NONE', *, *, #41763, .T. ) ;
#9065=DIRECTION ( 'NONE',  ( 0.000000000000000000, -0.000000000000000000, 1.000000000000000000 ) ) ;
#9067=VERTEX_POINT ( 'NONE', #27229 ) ;
#9068=EDGE_CURVE ( 'NONE', #37209, #32336, #3670, .T. ) ;
#9069=CARTESIAN_POINT ( 'NONE',  ( -2.293366432827344421E-15, -12.48450537969573659, -51.40625000204838102 ) ) ;
#9071=CARTESIAN_POINT ( 'NONE',  ( -10.81189881249999729, 6.242252689847871849, -104.2187500020483810 ) ) ;
#9073=ORIENTED_EDGE ( 'NONE', *, *, #12694, .T. ) ;
#9074=DIRECTION ( 'NONE',  ( -0.000000000000000000, -0.000000000000000000, 1.000000000000000000 ) ) ;
#9077=CARTESIAN_POINT ( 'NONE',  ( -10.81189881249999907, -6.242252689847864744, -156.4687500020484379 ) ) ;
#9079=CARTESIAN_POINT ( 'NONE',  ( -10.81189881249999729, 6.242252689847871849, -3.718750002048365477 ) ) ;
#9081=CARTESIAN_POINT ( 'NONE',  ( 10.81189881249999551, -6.242252689847874514, -137.9687500020483810 ) ) ;
#9083=CYLINDRICAL_SURFACE ( 'NONE', #19422, 9.999999999999998224 ) ;
#9085=CARTESIAN_POINT ( 'NONE',  ( -5.000000000000003553, -8.660254037844383745, -196.3750000040967905 ) ) ;
#9087=CARTESIAN_POINT ( 'NONE',  ( 10.81189881249999729, 6.242252689847867408, -194.9062500020484094 ) ) ;
#9088=CARTESIAN_POINT ( 'NONE',  ( -9.999999999999998224, 1.224646799147353059E-15, -6.125000004096770034 ) ) ;
#9091=EDGE_CURVE ( 'NONE', #20035, #2553, #21573, .T. ) ;
#9093=CARTESIAN_POINT ( 'NONE',  ( 10.81189881249999729, 6.242252689847867408, -65.71875000204836681 ) ) ;
#9094=CARTESIAN_POINT ( 'NONE',  ( 7.644554776091147741E-16, 12.48450537969573659, -53.46875000204837391 ) ) ;
#9096=CARTESIAN_POINT ( 'NONE',  ( -10.81189881249999729, 6.242252689847871849, -26.40625000204837747 ) ) ;
#9099=CARTESIAN_POINT ( 'NONE',  ( 10.00000000000000000, 5.773502691896255534, -115.8749999999999858 ) ) ;
#9103=CARTESIAN_POINT ( 'NONE',  ( -5.405949406250003975, -9.363379034771801557, -8.031250002048350822 ) ) ;
#9107=CARTESIAN_POINT ( 'NONE',  ( -9.999999999999998224, 1.224646799147353059E-15, -8.749999999999952038 ) ) ;
#9109=CARTESIAN_POINT ( 'NONE',  ( 7.070501591499377789E-16, 11.54700538379251284, -43.62499999999996447 ) ) ;
#9110=CARTESIAN_POINT ( 'NONE',  ( 10.00000000000000000, 5.773502691896255534, -23.25000000409677270 ) ) ;
#9111=CARTESIAN_POINT ( 'NONE',  ( 5.405949406249999534, 9.363379034771803333, -55.28125000204836681 ) ) ;
#9112=CARTESIAN_POINT ( 'NONE',  ( -1.040834085586084257E-14, -20.00000000000000355, 22.49999999999999289 ) ) ;
#9114=CARTESIAN_POINT ( 'NONE',  ( -8.660254037844447694, 15.00000000000010836, 49.99999999999998579 ) ) ;
#9115=CARTESIAN_POINT ( 'NONE',  ( 10.81189881249999551, -6.242252689847874514, -148.6562500020484094 ) ) ;
#9116=CARTESIAN_POINT ( 'NONE',  ( -10.81189881249999729, 6.242252689847871849, -152.4062500020483810 ) ) ;
#9117=CARTESIAN_POINT ( 'NONE',  ( 7.070501591499376803E-16, 11.54700538379251284, -78.50000000409677625 ) ) ;
#9118=CARTESIAN_POINT ( 'NONE',  ( 4.999999999999992006, -8.660254037844389075, -57.74999999999997158 ) ) ;
#9119=ORIENTED_EDGE ( 'NONE', *, *, #19327, .F. ) ;
#9120=ORIENTED_EDGE ( 'NONE', *, *, #25986, .T. ) ;
#9121=ORIENTED_EDGE ( 'NONE', *, *, #3109, .T. ) ;
#9122=DIRECTION ( 'NONE',  ( 0.000000000000000000, 0.000000000000000000, 1.000000000000000000 ) ) ;
#9123=CARTESIAN_POINT ( 'NONE',  ( 10.81189881249999551, -6.242252689847874514, -182.9687500020484094 ) ) ;
#9124=AXIS2_PLACEMENT_3D ( 'NONE', #41725, #38502, #39137 ) ;
#9125=CARTESIAN_POINT ( 'NONE',  ( 10.81189881249999729, 0.000000000000000000, -31.34375000204836681 ) ) ;
#9126=EDGE_CURVE ( 'NONE', #13498, #36973, #11082, .T. ) ;
#9127=CARTESIAN_POINT ( 'NONE',  ( 9.999999999999998224, 0.000000000000000000, -114.4999999999999858 ) ) ;
#9128=CARTESIAN_POINT ( 'NONE',  ( -10.81189881249999729, 1.324075727343319199E-15, -167.0937500020484094 ) ) ;
#9129=CARTESIAN_POINT ( 'NONE',  ( 5.405949406249992428, -9.363379034771808662, -151.5937500020483810 ) ) ;
#9133=CARTESIAN_POINT ( 'NONE',  ( 10.81189881249999551, -6.242252689847874514, -17.96875000204837036 ) ) ;
#9136=( BOUNDED_CURVE ( )  B_SPLINE_CURVE ( 2, ( #14254, #17716, #37592, #33943, #30911, #27671, #31133 ),
 .UNSPECIFIED., .F., .F. ) 
 B_SPLINE_CURVE_WITH_KNOTS ( ( 3, 2, 2, 3 ),
 ( 0.8917910447761197013, 0.8930348258706470865, 0.8942786069651743608, 0.8955223880597017461 ),
 .UNSPECIFIED. ) 
 CURVE ( )  GEOMETRIC_REPRESENTATION_ITEM ( )  RATIONAL_B_SPLINE_CURVE ( ( 0.9999999999999641398, 0.8660254037844745678, 1.000000000000000000, 0.8660254037844387076, 1.000000000000000000, 0.8660254037844148378, 1.000000000000023981 ) ) 
 REPRESENTATION_ITEM ( '' )  );
#9137=LINE ( 'NONE', #2259, #30271 ) ;
#9139=CARTESIAN_POINT ( 'NONE',  ( 5.405949406249999534, 9.363379034771803333, -83.59375000204836681 ) ) ;
#9141=CARTESIAN_POINT ( 'NONE',  ( -5.405949406249996869, 9.363379034771805109, -47.53125000204838813 ) ) ;
#9143=CARTESIAN_POINT ( 'NONE',  ( -4.999999999999996447, 8.660254037844387298, -90.37500000409677625 ) ) ;
#9145=CARTESIAN_POINT ( 'NONE',  ( 7.070501591499377789E-16, 11.54700538379251284, -135.1250000000000000 ) ) ;
#9146=CARTESIAN_POINT ( 'NONE',  ( 10.81189881249999729, 0.000000000000000000, -147.0312500020483810 ) ) ;
#9149=CARTESIAN_POINT ( 'NONE',  ( -5.000000000000003553, -8.660254037844383745, -121.3750000040967905 ) ) ;
#9152=( BOUNDED_CURVE ( )  B_SPLINE_CURVE ( 2, ( #42152, #42360, #6548, #2276, #19074, #2682, #35283 ),
 .UNSPECIFIED., .F., .F. ) 
 B_SPLINE_CURVE_WITH_KNOTS ( ( 3, 2, 2, 3 ),
 ( 0.7500000000000001110, 0.7512437810945274963, 0.7524875621890549926, 0.7537313432835822669 ),
 .UNSPECIFIED. ) 
 CURVE ( )  GEOMETRIC_REPRESENTATION_ITEM ( )  RATIONAL_B_SPLINE_CURVE ( ( 0.9999999999999880096, 0.8660254037844506980, 1.000000000000000000, 0.8660254037844387076, 1.000000000000000000, 0.8660254037844148378, 1.000000000000023981 ) ) 
 REPRESENTATION_ITEM ( '' )  );
#9155=CARTESIAN_POINT ( 'NONE',  ( 10.81189881249999551, -6.242252689847874514, -174.1562500020484094 ) ) ;
#9156=CARTESIAN_POINT ( 'NONE',  ( 4.999999999999992006, -8.660254037844389075, -46.12500000409677625 ) ) ;
#9158=CARTESIAN_POINT ( 'NONE',  ( 5.000000000000000000, 8.660254037844385522, -84.24999999999997158 ) ) ;
#9159=CARTESIAN_POINT ( 'NONE',  ( -10.81189881249999729, 6.242252689847871849, -170.4062500020484094 ) ) ;
#9161=CARTESIAN_POINT ( 'NONE',  ( -4.999999999999996447, 8.660254037844387298, -64.49999999999997158 ) ) ;
#9162=ORIENTED_EDGE ( 'NONE', *, *, #42504, .F. ) ;
#9163=CARTESIAN_POINT ( 'NONE',  ( -10.00000000000051337, 5.773502691895962435, -123.2500000040967763 ) ) ;
#9165=CARTESIAN_POINT ( 'NONE',  ( 10.81189881249999907, 6.242252689847868297, -80.90625000204839523 ) ) ;
#9166=ORIENTED_EDGE ( 'NONE', *, *, #10072, .T. ) ;
#9167=CARTESIAN_POINT ( 'NONE',  ( -5.000000000000003553, -8.660254037844383745, -119.5000000000000000 ) ) ;
#9168=ORIENTED_EDGE ( 'NONE', *, *, #8561, .F. ) ;
#9170=CARTESIAN_POINT ( 'NONE',  ( -2.293366432827344421E-15, -12.48450537969573659, -33.21875000204834549 ) ) ;
#9171=CARTESIAN_POINT ( 'NONE',  ( -10.00000000000000000, -5.773502691896252870, -171.0000000040967905 ) ) ;
#9172=CARTESIAN_POINT ( 'NONE',  ( -10.81189881249999729, 1.324075727343319199E-15, -8.281250002048350822 ) ) ;
#9173=CARTESIAN_POINT ( 'NONE',  ( 5.405949406249992428, -9.363379034771808662, -55.59375000204835970 ) ) ;
#9174=EDGE_LOOP ( 'NONE', ( #39456, #3783, #36548, #35412 ) ) ;
#9175=FACE_OUTER_BOUND ( 'NONE', #41140, .T. ) ;
#9177=CARTESIAN_POINT ( 'NONE',  ( -10.81189881249999729, -6.242252689847864744, -186.4687500020484094 ) ) ;
#9178=CARTESIAN_POINT ( 'NONE',  ( 10.81189881249999551, -6.242252689847874514, -175.4687500020484094 ) ) ;
#9181=CARTESIAN_POINT ( 'NONE',  ( 9.999999999999998224, 0.000000000000000000, -18.87500000409675494 ) ) ;
#9184=CARTESIAN_POINT ( 'NONE',  ( 5.405949406249999534, 9.363379034771803333, -109.0937500020483810 ) ) ;
#9185=CARTESIAN_POINT ( 'NONE',  ( -9.999999999999998224, 1.224646799147353059E-15, -64.62500000409676204 ) ) ;
#9186=CARTESIAN_POINT ( 'NONE',  ( -2.293366432827344421E-15, -12.48450537969573659, -78.40625000204838102 ) ) ;
#9187=CARTESIAN_POINT ( 'NONE',  ( -10.81189881249999729, -6.242252689847864744, -94.96875000204838102 ) ) ;
#9189=CARTESIAN_POINT ( 'NONE',  ( 9.999999999999998224, 0.000000000000000000, -147.8750000040967905 ) ) ;
#9192=ORIENTED_EDGE ( 'NONE', *, *, #5615, .T. ) ;
#9195=CARTESIAN_POINT ( 'NONE',  ( -5.405949406249996869, 9.363379034771805109, -194.5312500020484094 ) ) ;
#9198=ORIENTED_EDGE ( 'NONE', *, *, #26935, .T. ) ;
#9199=CARTESIAN_POINT ( 'NONE',  ( 10.00000000000000000, 5.773502691896255534, -64.87499999999998579 ) ) ;
#9201=CARTESIAN_POINT ( 'NONE',  ( -2.121150477449813534E-15, -11.54700538379251284, -76.25000000409677625 ) ) ;
#9203=FACE_OUTER_BOUND ( 'NONE', #14753, .T. ) ;
#9205=CARTESIAN_POINT ( 'NONE',  ( 10.81189881249999729, 6.242252689847867408, -65.90625000204839523 ) ) ;
#9207=CARTESIAN_POINT ( 'NONE',  ( -10.00000000000051337, 5.773502691895962435, -93.25000000409676204 ) ) ;
#9209=CARTESIAN_POINT ( 'NONE',  ( -5.405949406249996869, 9.363379034771805109, -191.5312500020484094 ) ) ;
#9211=CARTESIAN_POINT ( 'NONE',  ( 5.405949406249999534, 9.363379034771803333, -2.593750002048367254 ) ) ;
#9212=CARTESIAN_POINT ( 'NONE',  ( 9.999999999999479527, 5.773502691896553074, -140.2500000040967620 ) ) ;
#9214=CARTESIAN_POINT ( 'NONE',  ( -9.999999999999998224, 1.224646799147353059E-15, -108.1250000040967763 ) ) ;
#9215=DIRECTION ( 'NONE',  ( 1.000000000000000000, 0.000000000000000000, 0.000000000000000000 ) ) ;
#9216=EDGE_CURVE ( 'NONE', #1967, #25696, #653, .T. ) ;
#9217=CARTESIAN_POINT ( 'NONE',  ( 7.070501591499377789E-16, 11.54700538379251284, -174.1250000000000000 ) ) ;
#9218=CARTESIAN_POINT ( 'NONE',  ( 9.999999999999998224, 0.000000000000000000, -1.999999999999974021 ) ) ;
#9219=CARTESIAN_POINT ( 'NONE',  ( 7.644554776091147741E-16, 12.48450537969573659, -98.65625000204838102 ) ) ;
#9220=ORIENTED_EDGE ( 'NONE', *, *, #39923, .F. ) ;
#9221=ADVANCED_FACE ( 'NONE', ( #31127 ), #25505, .T. ) ;
#9222=CARTESIAN_POINT ( 'NONE',  ( 5.000000000000000000, 8.660254037844385522, -37.74999999999997868 ) ) ;
#9224=ORIENTED_EDGE ( 'NONE', *, *, #9538, .T. ) ;
#9225=CARTESIAN_POINT ( 'NONE',  ( -10.81189881249999729, 1.324075727343319199E-15, -26.28125000204836681 ) ) ;
#9227=CARTESIAN_POINT ( 'NONE',  ( 10.81189881249999907, 6.242252689847868297, -77.71875000204838102 ) ) ;
#9229=FACE_OUTER_BOUND ( 'NONE', #38797, .T. ) ;
#9231=CARTESIAN_POINT ( 'NONE',  ( -9.999999999999998224, 1.224646799147353059E-15, -49.24999999999998579 ) ) ;
#9233=CARTESIAN_POINT ( 'NONE',  ( -4.999999999999996447, 8.660254037844387298, -9.375000004096744277 ) ) ;
#9235=CARTESIAN_POINT ( 'NONE',  ( -5.405949406249996869, 9.363379034771805109, -131.3437500020484094 ) ) ;
#9236=CARTESIAN_POINT ( 'NONE',  ( 10.81189881249999551, -6.242252689847874514, -99.15625000204838102 ) ) ;
#9237=CARTESIAN_POINT ( 'NONE',  ( 5.405949406249999534, 9.363379034771803333, -113.5937500020483810 ) ) ;
#9240=CARTESIAN_POINT ( 'NONE',  ( -10.00000000000000000, -5.773502691896251982, -172.5000000040967905 ) ) ;
#9243=CARTESIAN_POINT ( 'NONE',  ( 7.644554776091147741E-16, 12.48450537969573659, -44.46875000204836681 ) ) ;
#9245=CARTESIAN_POINT ( 'NONE',  ( -10.81189881249999729, 6.242252689847871849, -0.9062500020483681418 ) ) ;
#9247=CARTESIAN_POINT ( 'NONE',  ( 9.999999999999998224, 0.000000000000000000, -6.499999999999977796 ) ) ;
#9250=CARTESIAN_POINT ( 'NONE',  ( 10.00000000000000000, 5.773502691896255534, -93.37499999999997158 ) ) ;
#9252=CARTESIAN_POINT ( 'NONE',  ( 9.999999999999996447, -5.773502691896262640, -100.0000000040967763 ) ) ;
#9255=CARTESIAN_POINT ( 'NONE',  ( -10.81189881249999729, -6.242252689847864744, -93.65625000204840944 ) ) ;
#9259=CARTESIAN_POINT ( 'NONE',  ( 9.999999999999998224, 0.000000000000000000, -29.37500000409676204 ) ) ;
#9261=ORIENTED_EDGE ( 'NONE', *, *, #26728, .F. ) ;
#9262=CARTESIAN_POINT ( 'NONE',  ( -4.999999999999996447, 8.660254037844387298, -16.49999999999995737 ) ) ;
#9263=CARTESIAN_POINT ( 'NONE',  ( -10.81189881249999729, 1.324075727343319199E-15, -23.28125000204836326 ) ) ;
#9264=CARTESIAN_POINT ( 'NONE',  ( 9.999999999999998224, 0.000000000000000000, -156.5000000000000000 ) ) ;
#9267=CARTESIAN_POINT ( 'NONE',  ( -5.405949406249996869, 9.363379034771805109, -127.0312500020483952 ) ) ;
#9268=ORIENTED_EDGE ( 'NONE', *, *, #31909, .F. ) ;
#9269=CARTESIAN_POINT ( 'NONE',  ( 5.000000000000000000, 8.660254037844385522, -117.6250000040967905 ) ) ;
#9271=CARTESIAN_POINT ( 'NONE',  ( -10.81189881249999729, 1.324075727343319199E-15, -50.28125000204835970 ) ) ;
#9273=CARTESIAN_POINT ( 'NONE',  ( -5.405949406249996869, 9.363379034771805109, -104.3437500020483810 ) ) ;
#9275=ORIENTED_EDGE ( 'NONE', *, *, #24028, .T. ) ;
#9276=CARTESIAN_POINT ( 'NONE',  ( -10.00000000000012790, -5.773502691896177375, -175.5000000040967905 ) ) ;
#9277=CARTESIAN_POINT ( 'NONE',  ( 9.999999999999998224, 0.000000000000000000, -144.8750000040967905 ) ) ;
#9278=CARTESIAN_POINT ( 'NONE',  ( -10.81189881249999729, 1.324075727343319199E-15, -147.5937500020483810 ) ) ;
#9280=CARTESIAN_POINT ( 'NONE',  ( -10.81189881249999907, -6.242252689847864744, -10.96875000204836859 ) ) ;
#9281=FACE_OUTER_BOUND ( 'NONE', #28596, .T. ) ;
#9282=CARTESIAN_POINT ( 'NONE',  ( 10.81189881249999729, 6.242252689847867408, -139.2187500020483810 ) ) ;
#9284=CARTESIAN_POINT ( 'NONE',  ( -2.121150477449813534E-15, -11.54700538379251284, -147.8750000000000000 ) ) ;
#9286=CARTESIAN_POINT ( 'NONE',  ( -9.999999999999998224, 5.773502691896259087, -190.7500000040968189 ) ) ;
#9288=CARTESIAN_POINT ( 'NONE',  ( -10.81189881249999729, 6.242252689847871849, -189.9062500020484379 ) ) ;
#9289=AXIS2_PLACEMENT_3D ( 'NONE', #41625, #18328, #18543 ) ;
#9290=CARTESIAN_POINT ( 'NONE',  ( -2.121150477449813534E-15, -11.54700538379251284, -47.37499999999996447 ) ) ;
#9293=EDGE_CURVE ( 'NONE', #8991, #38740, #24869, .T. ) ;
#9294=CARTESIAN_POINT ( 'NONE',  ( -2.293366432827344421E-15, -12.48450537969573659, -69.21875000204838102 ) ) ;
#9295=CARTESIAN_POINT ( 'NONE',  ( -10.81189881249999907, -6.242252689847864744, -46.96875000204835970 ) ) ;
#9297=CARTESIAN_POINT ( 'NONE',  ( 7.644554776091147741E-16, 12.48450537969573659, -26.65625000204837747 ) ) ;
#9302=CARTESIAN_POINT ( 'NONE',  ( -9.999999999999998224, 1.224646799147353059E-15, -113.7499999999999858 ) ) ;
#9303=CARTESIAN_POINT ( 'NONE',  ( -9.999999999999998224, 1.224646799147353059E-15, -118.6250000040967905 ) ) ;
#9304=EDGE_CURVE ( 'NONE', #33047, #29342, #15499, .T. ) ;
#9307=CARTESIAN_POINT ( 'NONE',  ( -5.405949406250003975, -9.363379034771801557, -113.0312500020483952 ) ) ;
#9309=ORIENTED_EDGE ( 'NONE', *, *, #5844, .T. ) ;
#9310=CARTESIAN_POINT ( 'NONE',  ( 7.070501591499376803E-16, 11.54700538379251284, -121.6249999999999858 ) ) ;
#9312=DIRECTION ( 'NONE',  ( -0.000000000000000000, -0.000000000000000000, 1.000000000000000000 ) ) ;
#9314=CARTESIAN_POINT ( 'NONE',  ( -9.999999999999998224, 5.773502691896259087, -41.87499999999997868 ) ) ;
#9315=CARTESIAN_POINT ( 'NONE',  ( -5.000000000000003553, -8.660254037844383745, -26.87500000409676204 ) ) ;
#9316=CARTESIAN_POINT ( 'NONE',  ( 5.405949406249999534, 9.363379034771803333, -41.78125000204838102 ) ) ;
#9317=CARTESIAN_POINT ( 'NONE',  ( -9.999999999999479527, -5.773502691896549521, -142.1249999999999716 ) ) ;
#9319=VECTOR ( 'NONE', #21876, 1000.000000000000000 ) ;
#9321=CARTESIAN_POINT ( 'NONE',  ( 5.405949406249992428, -9.363379034771808662, -135.2812500020483810 ) ) ;
#9322=CARTESIAN_POINT ( 'NONE',  ( 5.405949406249999534, 9.363379034771803333, -152.7812500020484094 ) ) ;
#9323=CARTESIAN_POINT ( 'NONE',  ( 7.070501591499376803E-16, 11.54700538379251284, -60.12499999999998579 ) ) ;
#9324=EDGE_CURVE ( 'NONE', #3757, #32390, #35932, .T. ) ;
#9327=AXIS2_PLACEMENT_3D ( 'NONE', #1300, #27625, #27192 ) ;
#9329=ORIENTED_EDGE ( 'NONE', *, *, #40131, .F. ) ;
#9330=ORIENTED_EDGE ( 'NONE', *, *, #27150, .T. ) ;
#9332=CARTESIAN_POINT ( 'NONE',  ( 5.405949406249992428, -9.363379034771808662, -174.0937500020484094 ) ) ;
#9333=CARTESIAN_POINT ( 'NONE',  ( -10.81189881249999907, -6.242252689847864744, -34.96875000204835260 ) ) ;
#9334=CARTESIAN_POINT ( 'NONE',  ( 4.999999999999992006, -8.660254037844389075, -128.6250000040967620 ) ) ;
#9335=CARTESIAN_POINT ( 'NONE',  ( -2.293366432827344421E-15, -12.48450537969573659, -165.2187500020483810 ) ) ;
#9336=CARTESIAN_POINT ( 'NONE',  ( -5.405949406250003975, -9.363379034771801557, -148.8437500020483810 ) ) ;
#9337=( BOUNDED_CURVE ( )  B_SPLINE_CURVE ( 2, ( #36964, #24032, #30514, #7407, #37170, #20554, #40194 ),
 .UNSPECIFIED., .F., .F. ) 
 B_SPLINE_CURVE_WITH_KNOTS ( ( 3, 2, 2, 3 ),
 ( 0.6119402985074627876, 0.6131840796019901729, 0.6144278606965176692, 0.6156716417910449435 ),
 .UNSPECIFIED. ) 
 CURVE ( )  GEOMETRIC_REPRESENTATION_ITEM ( )  RATIONAL_B_SPLINE_CURVE ( ( 0.9999999999999880096, 0.8660254037844506980, 1.000000000000000000, 0.8660254037844387076, 1.000000000000000000, 0.8660254037844148378, 1.000000000000023981 ) ) 
 REPRESENTATION_ITEM ( '' )  );
#9338=LINE ( 'NONE', #15584, #34187 ) ;
#9342=CARTESIAN_POINT ( 'NONE',  ( -10.81189881249999729, 6.242252689847871849, -17.21875000204836681 ) ) ;
#9345=CARTESIAN_POINT ( 'NONE',  ( 9.999999999999998224, 0.000000000000000000, -44.37500000409677625 ) ) ;
#9347=CARTESIAN_POINT ( 'NONE',  ( 10.81189881249999551, -6.242252689847874514, -73.46875000204835260 ) ) ;
#9348=CARTESIAN_POINT ( 'NONE',  ( 7.644554776091147741E-16, 12.48450537969573659, -52.15625000204838813 ) ) ;
#9352=CARTESIAN_POINT ( 'NONE',  ( 4.999999999999992006, -8.660254037844389075, -140.2500000000000000 ) ) ;
#9353=CARTESIAN_POINT ( 'NONE',  ( 5.405949406249992428, -9.363379034771808662, -150.2812500020483810 ) ) ;
#9354=CARTESIAN_POINT ( 'NONE',  ( 9.999999999999998224, 0.000000000000000000, -28.99999999999997158 ) ) ;
#9355=CARTESIAN_POINT ( 'NONE',  ( 7.070501591499377789E-16, 11.54700538379251284, -125.0000000040967763 ) ) ;
#9358=ORIENTED_EDGE ( 'NONE', *, *, #1245, .T. ) ;
#9362=CARTESIAN_POINT ( 'NONE',  ( -5.405949406249996869, 9.363379034771805109, -169.0312500020484094 ) ) ;
#9363=CARTESIAN_POINT ( 'NONE',  ( -5.000000000000003553, -8.660254037844383745, -49.37500000409678336 ) ) ;
#9364=CYLINDRICAL_SURFACE ( 'NONE', #29730, 9.999999999999998224 ) ;
#9366=CARTESIAN_POINT ( 'NONE',  ( 5.000000000000000000, 8.660254037844385522, -73.74999999999998579 ) ) ;
#9367=CARTESIAN_POINT ( 'NONE',  ( -10.81189881249999907, -6.242252689847864744, -170.1562500020483810 ) ) ;
#9368=CARTESIAN_POINT ( 'NONE',  ( 10.81189881249999907, 6.242252689847868297, -142.2187500020484094 ) ) ;
#9369=FACE_OUTER_BOUND ( 'NONE', #42542, .T. ) ;
#9370=CARTESIAN_POINT ( 'NONE',  ( 9.999999999999479527, 5.773502691896553074, -80.25000000409676204 ) ) ;
#9372=DIRECTION ( 'NONE',  ( -0.000000000000000000, -0.000000000000000000, 1.000000000000000000 ) ) ;
#9373=VECTOR ( 'NONE', #11714, 1000.000000000000000 ) ;
#9374=( BOUNDED_CURVE ( )  B_SPLINE_CURVE ( 2, ( #41367, #31045, #4488, #17630, #28232, #1263, #11583 ),
 .UNSPECIFIED., .F., .F. ) 
 B_SPLINE_CURVE_WITH_KNOTS ( ( 3, 2, 2, 3 ),
 ( 0.1082089552238805485, 0.1094527363184079616, 0.1106965174129353746, 0.1119402985074627876 ),
 .UNSPECIFIED. ) 
 CURVE ( )  GEOMETRIC_REPRESENTATION_ITEM ( )  RATIONAL_B_SPLINE_CURVE ( ( 1.000000000000004441, 0.8660254037844343777, 1.000000000000000000, 0.8660254037844387076, 1.000000000000000000, 0.8660254037844282715, 1.000000000000010436 ) ) 
 REPRESENTATION_ITEM ( '' )  );
#9375=EDGE_CURVE ( 'NONE', #8957, #37898, #6691, .T. ) ;
#9376=CARTESIAN_POINT ( 'NONE',  ( 5.405949406249992428, -9.363379034771808662, -69.28125000204838102 ) ) ;
#9377=ORIENTED_EDGE ( 'NONE', *, *, #11053, .T. ) ;
#9379=CARTESIAN_POINT ( 'NONE',  ( 9.999999999999998224, 0.000000000000000000, -143.0000000000000000 ) ) ;
#9380=ORIENTED_EDGE ( 'NONE', *, *, #28564, .T. ) ;
#9381=VECTOR ( 'NONE', #39901, 1000.000000000000000 ) ;
#9382=ORIENTED_EDGE ( 'NONE', *, *, #31803, .T. ) ;
#9383=CARTESIAN_POINT ( 'NONE',  ( 7.644554776091147741E-16, 12.48450537969573659, -29.46875000204835970 ) ) ;
#9384=( BOUNDED_CURVE ( )  B_SPLINE_CURVE ( 2, ( #10079, #27341, #40475, #24117, #33194, #37253, #7069 ),
 .UNSPECIFIED., .F., .F. ) 
 B_SPLINE_CURVE_WITH_KNOTS ( ( 3, 2, 2, 3 ),
 ( 0.9179104477611943480, 0.9191542288557217333, 0.9203980099502490075, 0.9216417910447763928 ),
 .UNSPECIFIED. ) 
 CURVE ( )  GEOMETRIC_REPRESENTATION_ITEM ( )  RATIONAL_B_SPLINE_CURVE ( ( 0.9999999999999641398, 0.8660254037844745678, 1.000000000000000000, 0.8660254037844387076, 1.000000000000000000, 0.8660254037844148378, 1.000000000000023981 ) ) 
 REPRESENTATION_ITEM ( '' )  );
#9385=CARTESIAN_POINT ( 'NONE',  ( 9.999999999999479527, 5.773502691896553074, -114.3749999999999716 ) ) ;
#9386=CARTESIAN_POINT ( 'NONE',  ( 5.405949406249999534, 9.363379034771803333, -5.781250002048377468 ) ) ;
#9387=CARTESIAN_POINT ( 'NONE',  ( 10.81189881249999551, -6.242252689847874514, -58.46875000204836681 ) ) ;
#9390=CARTESIAN_POINT ( 'NONE',  ( -5.405949406249996869, 9.363379034771805109, -185.3437500020483810 ) ) ;
#9391=CARTESIAN_POINT ( 'NONE',  ( 7.644554776091147741E-16, 12.48450537969573659, -167.4687500020483810 ) ) ;
#9394=CARTESIAN_POINT ( 'NONE',  ( 9.999999999999998224, 0.000000000000000000, -200.0000000000000000 ) ) ;
#9396=CARTESIAN_POINT ( 'NONE',  ( -9.999999999999998224, 1.224646799147353059E-15, -25.24999999999996803 ) ) ;
#9398=CARTESIAN_POINT ( 'NONE',  ( 5.405949406249992428, -9.363379034771808662, -105.0937500020483810 ) ) ;
#9400=CARTESIAN_POINT ( 'NONE',  ( -2.293366432827344421E-15, -12.48450537969573659, -72.40625000204836681 ) ) ;
#9401=CARTESIAN_POINT ( 'NONE',  ( 5.000000000000000000, 8.660254037844385522, -96.62500000409677625 ) ) ;
#9402=CARTESIAN_POINT ( 'NONE',  ( -2.293366432827344421E-15, -12.48450537969573659, -87.21875000204838102 ) ) ;
#9403=VECTOR ( 'NONE', #38328, 1000.000000000000000 ) ;
#9405=CARTESIAN_POINT ( 'NONE',  ( 4.999999999999992006, -8.660254037844389075, -143.6250000040967905 ) ) ;
#9410=CARTESIAN_POINT ( 'NONE',  ( -2.293366432827344421E-15, -12.48450537969573659, -193.9062500020484094 ) ) ;
#9411=LINE ( 'NONE', #15653, #41265 ) ;
#9413=ORIENTED_EDGE ( 'NONE', *, *, #10491, .T. ) ;
#9414=CARTESIAN_POINT ( 'NONE',  ( 5.000000000000000000, 8.660254037844385522, -57.24999999999996447 ) ) ;
#9416=CARTESIAN_POINT ( 'NONE',  ( -5.000000000000003553, -8.660254037844383745, -77.87500000409677625 ) ) ;
#9417=CARTESIAN_POINT ( 'NONE',  ( 5.000000000000000000, 8.660254037844385522, -102.2500000000000000 ) ) ;
#9418=CARTESIAN_POINT ( 'NONE',  ( 5.000000000000000000, 8.660254037844385522, -12.62500000409674783 ) ) ;
#9420=CARTESIAN_POINT ( 'NONE',  ( -10.81189881249999729, 1.324075727343319199E-15, -69.78125000204838102 ) ) ;
#9423=DIRECTION ( 'NONE',  ( -0.000000000000000000, -0.000000000000000000, 1.000000000000000000 ) ) ;
#9424=CARTESIAN_POINT ( 'NONE',  ( -2.293366432827344421E-15, -12.48450537969573659, -195.4062500020484094 ) ) ;
#9425=EDGE_CURVE ( 'NONE', #12898, #12699, #8084, .T. ) ;
#9427=CARTESIAN_POINT ( 'NONE',  ( -2.293366432827344421E-15, -12.48450537969573659, -9.218750002048359704 ) ) ;
#9428=DIRECTION ( 'NONE',  ( -0.000000000000000000, -0.000000000000000000, 1.000000000000000000 ) ) ;
#9430=CYLINDRICAL_SURFACE ( 'NONE', #4544, 9.999999999999998224 ) ;
#9431=CARTESIAN_POINT ( 'NONE',  ( 9.999999999999996447, -5.773502691896262640, -176.1250000000000000 ) ) ;
#9432=CARTESIAN_POINT ( 'NONE',  ( 0.000000000000000000, 0.000000000000000000, -200.0000000000000000 ) ) ;
#9433=CARTESIAN_POINT ( 'NONE',  ( -10.81189881249999729, 1.324075727343319199E-15, -101.2812500020483952 ) ) ;
#9434=ORIENTED_EDGE ( 'NONE', *, *, #1670, .T. ) ;
#9435=LINE ( 'NONE', #22600, #33124 ) ;
#9436=EDGE_LOOP ( 'NONE', ( #6363, #19699, #18010, #5297 ) ) ;
#9438=ADVANCED_FACE ( 'NONE', ( #42296 ), #39279, .T. ) ;
#9439=CARTESIAN_POINT ( 'NONE',  ( -5.405949406249996869, 9.363379034771805109, -36.84375000204836681 ) ) ;
#9440=CARTESIAN_POINT ( 'NONE',  ( -10.81189881249999729, 1.324075727343319199E-15, -33.78125000204837391 ) ) ;
#9443=CARTESIAN_POINT ( 'NONE',  ( -10.81189881249999729, 6.242252689847871849, -83.21875000204838102 ) ) ;
#9444=CARTESIAN_POINT ( 'NONE',  ( 9.999999999999998224, 0.000000000000000000, -34.99999999999997868 ) ) ;
#9446=CARTESIAN_POINT ( 'NONE',  ( -10.81189881249999729, 1.324075727343319199E-15, -198.5937500020484094 ) ) ;
#9448=CARTESIAN_POINT ( 'NONE',  ( 9.999999999999479527, 5.773502691896553074, -49.87499999999996447 ) ) ;
#9450=CARTESIAN_POINT ( 'NONE',  ( -9.999999999999998224, 1.224646799147353059E-15, -9.125000004096744277 ) ) ;
#9452=CARTESIAN_POINT ( 'NONE',  ( 5.405949406249992428, -9.363379034771808662, -126.0937500020483668 ) ) ;
#9453=CARTESIAN_POINT ( 'NONE',  ( 10.81189881249999551, -6.242252689847874514, -96.15625000204838102 ) ) ;
#9454=CARTESIAN_POINT ( 'NONE',  ( 10.81189881249999551, -6.242252689847874514, -110.9687500020483810 ) ) ;
#9457=CARTESIAN_POINT ( 'NONE',  ( 4.999999999999992006, -8.660254037844389075, -170.6250000040968189 ) ) ;
#9458=DIRECTION ( 'NONE',  ( 1.000000000000000000, 0.000000000000000000, 0.000000000000000000 ) ) ;
#9462=CARTESIAN_POINT ( 'NONE',  ( 14.84614977916193190, 1.301042606982605321E-14, 52.14285714285716011 ) ) ;
#9465=CARTESIAN_POINT ( 'NONE',  ( -10.00000000000000000, -5.773502691896251982, -88.12499999999998579 ) ) ;
#9467=CARTESIAN_POINT ( 'NONE',  ( 9.999999999999996447, -5.773502691896262640, -95.50000000409677625 ) ) ;
#9469=FACE_OUTER_BOUND ( 'NONE', #2299, .T. ) ;
#9471=CARTESIAN_POINT ( 'NONE',  ( 10.81189881249999729, 6.242252689847867408, -91.40625000204836681 ) ) ;
#9473=EDGE_CURVE ( 'NONE', #41377, #3757, #30148, .T. ) ;
#9475=CARTESIAN_POINT ( 'NONE',  ( 9.999999999999998224, 0.000000000000000000, -4.999999999999976907 ) ) ;
#9477=ORIENTED_EDGE ( 'NONE', *, *, #39350, .T. ) ;
#9478=CARTESIAN_POINT ( 'NONE',  ( -9.999999999999998224, 1.224646799147353059E-15, -19.24999999999996092 ) ) ;
#9479=CARTESIAN_POINT ( 'NONE',  ( -9.999999999999998224, 1.224646799147353059E-15, -154.2500000000000000 ) ) ;
#9482=CARTESIAN_POINT ( 'NONE',  ( 10.81189881249999729, 0.000000000000000000, -126.0312500020483952 ) ) ;
#9483=ORIENTED_EDGE ( 'NONE', *, *, #28564, .F. ) ;
#9484=AXIS2_PLACEMENT_3D ( 'NONE', #35580, #8819, #11604 ) ;
#9485=CARTESIAN_POINT ( 'NONE',  ( 10.00000000000154010, -5.773502691895370020, -21.62499999999993250 ) ) ;
#9486=EDGE_CURVE ( 'NONE', #7623, #41888, #12711, .T. ) ;
#9487=ORIENTED_EDGE ( 'NONE', *, *, #40899, .T. ) ;
#9488=CARTESIAN_POINT ( 'NONE',  ( 10.81189881249999907, 6.242252689847868297, -56.90625000204837391 ) ) ;
#9490=CARTESIAN_POINT ( 'NONE',  ( 5.405949406249999534, 9.363379034771803333, -101.5937500020483810 ) ) ;
#9493=CARTESIAN_POINT ( 'NONE',  ( 0.000000000000000000, 0.000000000000000000, -200.0000000000000000 ) ) ;
#9496=CARTESIAN_POINT ( 'NONE',  ( -9.999999999999998224, 1.224646799147353059E-15, -175.2500000000000284 ) ) ;
#9497=CARTESIAN_POINT ( 'NONE',  ( 9.999999999999998224, 0.000000000000000000, -177.5000000000000000 ) ) ;
#9498=CARTESIAN_POINT ( 'NONE',  ( -2.293366432827344421E-15, -12.48450537969573659, -129.2187500020483810 ) ) ;
#9500=CARTESIAN_POINT ( 'NONE',  ( 10.00000000000051159, -5.773502691895965988, -147.6249999999999716 ) ) ;
#9502=CARTESIAN_POINT ( 'NONE',  ( 7.070501591499377789E-16, 11.54700538379251284, -192.5000000040968189 ) ) ;
#9504=CARTESIAN_POINT ( 'NONE',  ( -10.81189881249999729, 6.242252689847871849, -188.4062500020484094 ) ) ;
#9506=DIRECTION ( 'NONE',  ( -0.000000000000000000, -0.000000000000000000, 1.000000000000000000 ) ) ;
#9509=CARTESIAN_POINT ( 'NONE',  ( 10.81189881249999729, 6.242252689847867408, -70.21875000204839523 ) ) ;
#9510=CARTESIAN_POINT ( 'NONE',  ( -10.81189881249999907, -6.242252689847864744, -51.46875000204837391 ) ) ;
#9512=CARTESIAN_POINT ( 'NONE',  ( -10.81189881249999907, -6.242252689847864744, -24.65625000204838457 ) ) ;
#9513=AXIS2_PLACEMENT_3D ( 'NONE', #16695, #32704, #26855 ) ;
#9515=CARTESIAN_POINT ( 'NONE',  ( 4.999999999999992006, -8.660254037844389075, -8.249999999999952038 ) ) ;
#9517=CARTESIAN_POINT ( 'NONE',  ( -10.00000000000000000, -5.773502691896251982, -110.6249999999999858 ) ) ;
#9518=VECTOR ( 'NONE', #35365, 1000.000000000000000 ) ;
#9521=CARTESIAN_POINT ( 'NONE',  ( -5.405949406250003975, -9.363379034771801557, -116.0312500020483952 ) ) ;
#9522=ORIENTED_EDGE ( 'NONE', *, *, #7513, .T. ) ;
#9523=DIRECTION ( 'NONE',  ( -0.000000000000000000, -1.000000000000000000, -0.000000000000000000 ) ) ;
#9525=CARTESIAN_POINT ( 'NONE',  ( 9.999999999999998224, 0.000000000000000000, -183.8750000040967905 ) ) ;
#9527=EDGE_LOOP ( 'NONE', ( #33700, #9745, #25892, #31406 ) ) ;
#9528=CARTESIAN_POINT ( 'NONE',  ( 10.00000000000000000, 5.773502691896255534, -42.37499999999997158 ) ) ;
#9529=CARTESIAN_POINT ( 'NONE',  ( 5.000000000000000000, 8.660254037844385522, -20.12500000409675494 ) ) ;
#9530=CARTESIAN_POINT ( 'NONE',  ( 10.81189881249999729, 6.242252689847867408, -41.90625000204836681 ) ) ;
#9531=DIRECTION ( 'NONE',  ( 0.000000000000000000, 0.000000000000000000, 1.000000000000000000 ) ) ;
#9534=CARTESIAN_POINT ( 'NONE',  ( 10.81189881249999907, 6.242252689847868297, -134.9062500020483810 ) ) ;
#9535=CARTESIAN_POINT ( 'NONE',  ( -10.81189881249999907, -6.242252689847864744, -149.1562500020483810 ) ) ;
#9536=EDGE_LOOP ( 'NONE', ( #16580, #30089, #2343, #8308 ) ) ;
#9537=ORIENTED_EDGE ( 'NONE', *, *, #35621, .T. ) ;
#9538=EDGE_CURVE ( 'NONE', #41318, #21756, #34561, .T. ) ;
#9540=ADVANCED_FACE ( 'NONE', ( #28950 ), #6278, .F. ) ;
#9541=DIRECTION ( 'NONE',  ( -0.000000000000000000, -0.000000000000000000, 1.000000000000000000 ) ) ;
#9542=CARTESIAN_POINT ( 'NONE',  ( 10.81189881249999729, 0.000000000000000000, -173.8437500020484094 ) ) ;
#9543=CARTESIAN_POINT ( 'NONE',  ( -5.405949406250003975, -9.363379034771801557, -22.84375000204835615 ) ) ;
#9544=CARTESIAN_POINT ( 'NONE',  ( -9.999999999999998224, 1.224646799147353059E-15, -126.1250000040967620 ) ) ;
#9545=CARTESIAN_POINT ( 'NONE',  ( 10.81189881249999551, -6.242252689847874514, -164.9687500020483810 ) ) ;
#9546=CARTESIAN_POINT ( 'NONE',  ( -2.293366432827344421E-15, -12.48450537969573659, -142.7187500020484094 ) ) ;
#9547=DIRECTION ( 'NONE',  ( -0.000000000000000000, -0.000000000000000000, 1.000000000000000000 ) ) ;
#9550=CARTESIAN_POINT ( 'NONE',  ( -2.293366432827344421E-15, -12.48450537969573659, -15.21875000204835615 ) ) ;
#9552=CARTESIAN_POINT ( 'NONE',  ( 0.000000000000000000, 0.000000000000000000, -200.0000000000000000 ) ) ;
#9553=CARTESIAN_POINT ( 'NONE',  ( 9.999999999998456346, 5.773502691897149042, -25.87499999999993960 ) ) ;
#9555=CARTESIAN_POINT ( 'NONE',  ( -9.999999999999998224, 1.224646799147353059E-15, -70.24999999999998579 ) ) ;
#9556=CARTESIAN_POINT ( 'NONE',  ( 10.81189881249999729, 0.000000000000000000, -76.34375000204838102 ) ) ;
#9557=CARTESIAN_POINT ( 'NONE',  ( -10.81189881249999907, -6.242252689847864744, -47.15625000204836681 ) ) ;
#9561=CARTESIAN_POINT ( 'NONE',  ( -2.121150477449813534E-15, -11.54700538379251284, -138.8750000000000000 ) ) ;
#9562=CARTESIAN_POINT ( 'NONE',  ( -10.81189881249999729, -6.242252689847864744, -137.1562500020484094 ) ) ;
#9563=CARTESIAN_POINT ( 'NONE',  ( 4.999999999999992006, -8.660254037844389075, -23.62500000409675849 ) ) ;
#9564=CARTESIAN_POINT ( 'NONE',  ( 7.070501591499377789E-16, 11.54700538379251284, -116.0000000040967763 ) ) ;
#9566=EDGE_LOOP ( 'NONE', ( #12030, #20591, #32015 ) ) ;
#9569=DIRECTION ( 'NONE',  ( 1.000000000000000000, 0.000000000000000000, 0.000000000000000000 ) ) ;
#9570=CARTESIAN_POINT ( 'NONE',  ( 5.405949406249992428, -9.363379034771808662, -174.2812500020484094 ) ) ;
#9571=CARTESIAN_POINT ( 'NONE',  ( -2.121150477449813534E-15, -11.54700538379251284, -49.25000000409676915 ) ) ;
#9572=CARTESIAN_POINT ( 'NONE',  ( 9.999999999999479527, 5.773502691896553074, -48.75000000409676204 ) ) ;
#9574=CARTESIAN_POINT ( 'NONE',  ( 9.999999999999998224, 0.000000000000000000, -101.3750000040967905 ) ) ;
#9575=CARTESIAN_POINT ( 'NONE',  ( 10.81189881249999551, -6.242252689847874514, -157.6562500020484094 ) ) ;
#9576=VECTOR ( 'NONE', #27352, 1000.000000000000000 ) ;
#9577=CARTESIAN_POINT ( 'NONE',  ( 5.405949406249999534, 9.363379034771803333, -146.5937500020483810 ) ) ;
#9579=CARTESIAN_POINT ( 'NONE',  ( -9.999999999999998224, 1.224646799147353059E-15, -74.74999999999998579 ) ) ;
#9580=ORIENTED_EDGE ( 'NONE', *, *, #5930, .F. ) ;
#9581=CARTESIAN_POINT ( 'NONE',  ( 9.999999999999998224, 0.000000000000000000, -78.49999999999998579 ) ) ;
#9582=CARTESIAN_POINT ( 'NONE',  ( -10.81189881249999907, -6.242252689847864744, -71.15625000204839523 ) ) ;
#9583=ORIENTED_EDGE ( 'NONE', *, *, #16948, .F. ) ;
#9584=EDGE_CURVE ( 'NONE', #24932, #27948, #39067, .T. ) ;
#9585=CARTESIAN_POINT ( 'NONE',  ( 10.81189881249999729, 0.000000000000000000, -121.3437500020483952 ) ) ;
#9587=ORIENTED_EDGE ( 'NONE', *, *, #9018, .F. ) ;
#9588=EDGE_CURVE ( 'NONE', #4873, #3545, #41717, .T. ) ;
#9589=CARTESIAN_POINT ( 'NONE',  ( 10.81189881249999729, 6.242252689847867408, -31.21875000204835260 ) ) ;
#9590=CARTESIAN_POINT ( 'NONE',  ( -10.81189881249999729, 1.324075727343319199E-15, -194.0937500020484094 ) ) ;
#9591=CARTESIAN_POINT ( 'NONE',  ( -5.405949406250003975, -9.363379034771801557, -51.34375000204835260 ) ) ;
#9593=LINE ( 'NONE', #39787, #30966 ) ;
#9595=CARTESIAN_POINT ( 'NONE',  ( -10.81189881249999729, -6.242252689847864744, -189.4687500020484094 ) ) ;
#9596=CARTESIAN_POINT ( 'NONE',  ( 10.81189881249999551, -6.242252689847874514, -167.9687500020483810 ) ) ;
#9601=CARTESIAN_POINT ( 'NONE',  ( 7.070501591499376803E-16, 11.54700538379251284, -188.0000000040968189 ) ) ;
#9604=CARTESIAN_POINT ( 'NONE',  ( 5.405949406249999534, 9.363379034771803333, -94.09375000204838102 ) ) ;
#9605=CARTESIAN_POINT ( 'NONE',  ( 9.999999999999479527, 5.773502691896553074, -108.7500000040967620 ) ) ;
#9606=CARTESIAN_POINT ( 'NONE',  ( -10.81189881249999907, -6.242252689847864744, -74.15625000204835260 ) ) ;
#9607=CARTESIAN_POINT ( 'NONE',  ( -9.999999999999998224, 1.224646799147353059E-15, -142.6250000040967905 ) ) ;
#9609=CARTESIAN_POINT ( 'NONE',  ( 7.644554776091147741E-16, 12.48450537969573659, -81.96875000204838102 ) ) ;
#9611=CARTESIAN_POINT ( 'NONE',  ( 10.00000000000000000, 5.773502691896255534, -135.7500000040967905 ) ) ;
#9613=VERTEX_POINT ( 'NONE', #30641 ) ;
#9617=ADVANCED_FACE ( 'NONE', ( #3678 ), #37319, .T. ) ;
#9618=CARTESIAN_POINT ( 'NONE',  ( -10.81189881249999907, -6.242252689847864744, -197.1562500020484379 ) ) ;
#9619=LINE ( 'NONE', #22791, #4070 ) ;
#9622=CARTESIAN_POINT ( 'NONE',  ( 7.070501591499377789E-16, 11.54700538379251284, -60.12499999999997868 ) ) ;
#9624=CARTESIAN_POINT ( 'NONE',  ( -10.00000000000000000, -5.773502691896251982, -70.50000000409677625 ) ) ;
#9625=CARTESIAN_POINT ( 'NONE',  ( 23.09401076758504345, 1.040834085586084257E-14, 49.99999999999998579 ) ) ;
#9628=CARTESIAN_POINT ( 'NONE',  ( -10.81189881249999729, -6.242252689847864744, -65.15625000204838102 ) ) ;
#9629=( BOUNDED_CURVE ( )  B_SPLINE_CURVE ( 2, ( #24953, #28400, #14984, #21477, #8539, #5295, #20832 ),
 .UNSPECIFIED., .F., .F. ) 
 B_SPLINE_CURVE_WITH_KNOTS ( ( 3, 2, 2, 3 ),
 ( 0.01492537313432837180, 0.01616915422885573453, 0.01741293532338310246, 0.01865671641791046345 ),
 .UNSPECIFIED. ) 
 CURVE ( )  GEOMETRIC_REPRESENTATION_ITEM ( )  RATIONAL_B_SPLINE_CURVE ( ( 0.9999999999999984457, 0.8660254037844402619, 1.000000000000000000, 0.8660254037844387076, 1.000000000000000000, 0.8660254037844368202, 1.000000000000001776 ) ) 
 REPRESENTATION_ITEM ( '' )  );
#9632=CARTESIAN_POINT ( 'NONE',  ( -9.999999999999998224, 1.224646799147353059E-15, -151.6250000040967905 ) ) ;
#9633=CARTESIAN_POINT ( 'NONE',  ( 5.405949406249999534, 9.363379034771803333, -181.2812500020483810 ) ) ;
#9636=CYLINDRICAL_SURFACE ( 'NONE', #24889, 9.999999999999998224 ) ;
#9638=DIRECTION ( 'NONE',  ( 0.000000000000000000, 1.000000000000000000, 0.000000000000000000 ) ) ;
#9639=( BOUNDED_CURVE ( )  B_SPLINE_CURVE ( 2, ( #32707, #9605, #19523, #2932, #22778, #6380, #36148 ),
 .UNSPECIFIED., .F., .F. ) 
 B_SPLINE_CURVE_WITH_KNOTS ( ( 3, 2, 2, 3 ),
 ( 0.4477611940298508730, 0.4490049751243782028, 0.4502487562189055881, 0.4514925373134329734 ),
 .UNSPECIFIED. ) 
 CURVE ( )  GEOMETRIC_REPRESENTATION_ITEM ( )  RATIONAL_B_SPLINE_CURVE ( ( 0.9999999999999880096, 0.8660254037844506980, 1.000000000000000000, 0.8660254037844387076, 1.000000000000000000, 0.8660254037844267172, 1.000000000000011990 ) ) 
 REPRESENTATION_ITEM ( '' )  );
#9640=CARTESIAN_POINT ( 'NONE',  ( 5.000000000000000000, 8.660254037844385522, -166.7500000000000000 ) ) ;
#9641=CARTESIAN_POINT ( 'NONE',  ( 9.999999999999998224, 0.000000000000000000, -200.0000000000000000 ) ) ;
#9642=AXIS2_PLACEMENT_3D ( 'NONE', #17157, #26681, #13283 ) ;
#9643=CARTESIAN_POINT ( 'NONE',  ( 5.405949406249992428, -9.363379034771808662, -93.28125000204838102 ) ) ;
#9647=VERTEX_POINT ( 'NONE', #13983 ) ;
#9649=CARTESIAN_POINT ( 'NONE',  ( -10.81189881249999907, -6.242252689847864744, -34.96875000204835260 ) ) ;
#9650=CARTESIAN_POINT ( 'NONE',  ( -10.81189881249999729, 1.324075727343319199E-15, -23.28125000204836326 ) ) ;
#9652=CARTESIAN_POINT ( 'NONE',  ( -5.405949406250003975, -9.363379034771801557, -81.34375000204838102 ) ) ;
#9653=CARTESIAN_POINT ( 'NONE',  ( -2.121150477449813534E-15, -11.54700538379251284, -173.7500000040968189 ) ) ;
#9655=CARTESIAN_POINT ( 'NONE',  ( -5.405949406249996869, 9.363379034771805109, -191.3437500020484094 ) ) ;
#9656=DIRECTION ( 'NONE',  ( -0.000000000000000000, -0.000000000000000000, 1.000000000000000000 ) ) ;
#9659=CARTESIAN_POINT ( 'NONE',  ( 5.000000000000000000, 8.660254037844385522, -3.625000004096767814 ) ) ;
#9660=CARTESIAN_POINT ( 'NONE',  ( 9.999999999999998224, 0.000000000000000000, -102.8750000040967763 ) ) ;
#9661=EDGE_CURVE ( 'NONE', #1760, #6518, #7838, .T. ) ;
#9662=CARTESIAN_POINT ( 'NONE',  ( 10.81189881249999907, 6.242252689847868297, -119.7187500020483810 ) ) ;
#9663=CARTESIAN_POINT ( 'NONE',  ( -5.405949406250003975, -9.363379034771801557, -101.0312500020483952 ) ) ;
#9664=CARTESIAN_POINT ( 'NONE',  ( -5.405949406250003975, -9.363379034771801557, -105.3437500020483810 ) ) ;
#9667=CARTESIAN_POINT ( 'NONE',  ( -4.999999999999996447, 8.660254037844387298, -169.8750000040967905 ) ) ;
#9668=DIRECTION ( 'NONE',  ( -0.000000000000000000, -0.000000000000000000, 1.000000000000000000 ) ) ;
#9674=CARTESIAN_POINT ( 'NONE',  ( -9.999999999999998224, 1.224646799147353059E-15, -60.12500000409676204 ) ) ;
#9676=CARTESIAN_POINT ( 'NONE',  ( -2.121150477449813534E-15, -11.54700538379251284, -81.87500000000000000 ) ) ;
#9678=CARTESIAN_POINT ( 'NONE',  ( 7.070501591499377789E-16, 11.54700538379251284, -99.50000000409677625 ) ) ;
#9681=CARTESIAN_POINT ( 'NONE',  ( -5.405949406250003975, -9.363379034771801557, -92.03125000204838102 ) ) ;
#9682=ORIENTED_EDGE ( 'NONE', *, *, #37564, .T. ) ;
#9686=CARTESIAN_POINT ( 'NONE',  ( 9.999999999999998224, 0.000000000000000000, -19.99999999999996092 ) ) ;
#9687=CARTESIAN_POINT ( 'NONE',  ( 7.070501591499377789E-16, 11.54700538379251284, -147.1250000000000000 ) ) ;
#9689=CARTESIAN_POINT ( 'NONE',  ( 9.999999999999998224, 0.000000000000000000, -197.0000000000000000 ) ) ;
#9690=CARTESIAN_POINT ( 'NONE',  ( 5.405949406249999534, 9.363379034771803333, -118.2812500020483952 ) ) ;
#9692=CARTESIAN_POINT ( 'NONE',  ( -9.999999999999998224, 1.224646799147353059E-15, -64.62500000409676204 ) ) ;
#9693=ORIENTED_EDGE ( 'NONE', *, *, #34252, .T. ) ;
#9694=CARTESIAN_POINT ( 'NONE',  ( 7.644554776091147741E-16, 12.48450537969573659, -52.15625000204838813 ) ) ;
#9696=CARTESIAN_POINT ( 'NONE',  ( 5.405949406249992428, -9.363379034771808662, -106.5937500020483810 ) ) ;
#9697=CARTESIAN_POINT ( 'NONE',  ( -10.81189881249999729, 6.242252689847871849, -122.4062500020483952 ) ) ;
#9701=CARTESIAN_POINT ( 'NONE',  ( 7.070501591499376803E-16, 11.54700538379251284, -78.12500000000000000 ) ) ;
#9703=CARTESIAN_POINT ( 'NONE',  ( -10.81189881249999729, 1.324075727343319199E-15, -2.093750002048366810 ) ) ;
#9704=CARTESIAN_POINT ( 'NONE',  ( 7.070501591499376803E-16, 11.54700538379251284, -0.5000000040967461645 ) ) ;
#9705=CARTESIAN_POINT ( 'NONE',  ( 5.405949406249992428, -9.363379034771808662, -133.5937500020483810 ) ) ;
#9709=CARTESIAN_POINT ( 'NONE',  ( 9.999999999999996447, -5.773502691896262640, -197.5000000040968189 ) ) ;
#9711=CARTESIAN_POINT ( 'NONE',  ( 10.81189881249999551, -6.242252689847874514, -186.1562500020484094 ) ) ;
#9712=CARTESIAN_POINT ( 'NONE',  ( 9.999999999999998224, 0.000000000000000000, -6.875000004096742501 ) ) ;
#9715=CARTESIAN_POINT ( 'NONE',  ( -5.405949406250003975, -9.363379034771801557, -60.34375000204835970 ) ) ;
#9716=CARTESIAN_POINT ( 'NONE',  ( -10.81189881249999907, -6.242252689847864744, -48.46875000204837391 ) ) ;
#9718=CARTESIAN_POINT ( 'NONE',  ( -10.81189881249999729, 1.324075727343319199E-15, -17.28125000204835970 ) ) ;
#9720=CARTESIAN_POINT ( 'NONE',  ( 9.999999999999998224, 0.000000000000000000, -27.87500000409676204 ) ) ;
#9722=CARTESIAN_POINT ( 'NONE',  ( -4.999999999999996447, 8.660254037844387298, -102.0000000000000000 ) ) ;
#9723=CARTESIAN_POINT ( 'NONE',  ( -9.999999999998456346, -5.773502691897145489, -28.12499999999995026 ) ) ;
#9726=CARTESIAN_POINT ( 'NONE',  ( 5.405949406249992428, -9.363379034771808662, -114.2812500020483952 ) ) ;
#9728=ORIENTED_EDGE ( 'NONE', *, *, #16959, .F. ) ;
#9729=AXIS2_PLACEMENT_3D ( 'NONE', #8740, #31199, #27952 ) ;
#9730=DIRECTION ( 'NONE',  ( 1.000000000000000000, 0.000000000000000000, 0.000000000000000000 ) ) ;
#9734=ORIENTED_EDGE ( 'NONE', *, *, #14872, .T. ) ;
#9735=CARTESIAN_POINT ( 'NONE',  ( 4.999999999999992006, -8.660254037844389075, -39.74999999999997868 ) ) ;
#9737=CARTESIAN_POINT ( 'NONE',  ( -10.00000000000000000, -5.773502691896251982, -19.50000000409677270 ) ) ;
#9738=CARTESIAN_POINT ( 'NONE',  ( -5.405949406249996869, 9.363379034771805109, -43.03125000204838102 ) ) ;
#9739=CARTESIAN_POINT ( 'NONE',  ( -10.00000000000102496, 5.773502691895664007, -16.37499999999995381 ) ) ;
#9742=CARTESIAN_POINT ( 'NONE',  ( -10.81189881249999729, 6.242252689847871849, -134.4062500020484094 ) ) ;
#9743=CARTESIAN_POINT ( 'NONE',  ( -10.81189881249999729, 6.242252689847871849, -146.4062500020484094 ) ) ;
#9745=ORIENTED_EDGE ( 'NONE', *, *, #14315, .T. ) ;
#9746=ORIENTED_EDGE ( 'NONE', *, *, #36492, .T. ) ;
#9747=ORIENTED_EDGE ( 'NONE', *, *, #23044, .T. ) ;
#9750=( BOUNDED_CURVE ( )  B_SPLINE_CURVE ( 2, ( #32078, #2928, #5745, #16057, #2306, #38115, #21709 ),
 .UNSPECIFIED., .F., .F. ) 
 B_SPLINE_CURVE_WITH_KNOTS ( ( 3, 2, 2, 3 ),
 ( 0.6156716417910449435, 0.6169154228855723288, 0.6181592039800996030, 0.6194029850746269883 ),
 .UNSPECIFIED. ) 
 CURVE ( )  GEOMETRIC_REPRESENTATION_ITEM ( )  RATIONAL_B_SPLINE_CURVE ( ( 0.9999999999999761302, 0.8660254037844625774, 1.000000000000000000, 0.8660254037844387076, 1.000000000000000000, 0.8660254037844267172, 1.000000000000011990 ) ) 
 REPRESENTATION_ITEM ( '' )  );
#9751=CARTESIAN_POINT ( 'NONE',  ( -10.81189881249999729, 6.242252689847871849, -174.7187500020483810 ) ) ;
#9753=CARTESIAN_POINT ( 'NONE',  ( -5.405949406250003975, -9.363379034771801557, -25.84375000204835970 ) ) ;
#9754=CARTESIAN_POINT ( 'NONE',  ( 4.999999999999992006, -8.660254037844389075, -61.12500000409676204 ) ) ;
#9755=CARTESIAN_POINT ( 'NONE',  ( -2.293366432827344421E-15, -12.48450537969573659, -159.2187500020483526 ) ) ;
#9756=CARTESIAN_POINT ( 'NONE',  ( 5.405949406249999534, 9.363379034771803333, -143.5937500020483810 ) ) ;
#9757=CARTESIAN_POINT ( 'NONE',  ( -9.999999999998456346, -5.773502691897145489, -9.000000004096717632 ) ) ;
#9760=CARTESIAN_POINT ( 'NONE',  ( -10.81189881249999729, 6.242252689847871849, -18.71875000204837391 ) ) ;
#9762=FACE_OUTER_BOUND ( 'NONE', #1107, .T. ) ;
#9763=CARTESIAN_POINT ( 'NONE',  ( 5.000000000000000000, 8.660254037844385522, -44.12500000409677625 ) ) ;
#9766=VECTOR ( 'NONE', #28351, 1000.000000000000000 ) ;
#9767=CARTESIAN_POINT ( 'NONE',  ( -10.81189881249999907, -6.242252689847864744, -70.96875000204840944 ) ) ;
#9768=CARTESIAN_POINT ( 'NONE',  ( -5.405949406249996869, 9.363379034771805109, -38.53125000204838102 ) ) ;
#9770=CARTESIAN_POINT ( 'NONE',  ( 7.070501591499376803E-16, 11.54700538379251284, -90.50000000409677625 ) ) ;
#9772=CARTESIAN_POINT ( 'NONE',  ( 7.070501591499377789E-16, 11.54700538379251284, -136.6250000000000000 ) ) ;
#9773=CARTESIAN_POINT ( 'NONE',  ( 5.405949406249992428, -9.363379034771808662, -141.2812500020483810 ) ) ;
#9774=CARTESIAN_POINT ( 'NONE',  ( 0.000000000000000000, 0.000000000000000000, -200.0000000000000000 ) ) ;
#9775=CARTESIAN_POINT ( 'NONE',  ( 5.000000000000000000, 8.660254037844385522, -113.1250000040967763 ) ) ;
#9777=ORIENTED_EDGE ( 'NONE', *, *, #11801, .T. ) ;
#9780=CARTESIAN_POINT ( 'NONE',  ( -9.999999999999479527, -5.773502691896549521, -141.0000000040967620 ) ) ;
#9781=CARTESIAN_POINT ( 'NONE',  ( -10.81189881249999729, 1.324075727343319199E-15, -173.2812500020484094 ) ) ;
#9782=CARTESIAN_POINT ( 'NONE',  ( 9.999999999999998224, 0.000000000000000000, -42.87500000409677625 ) ) ;
#9783=EDGE_CURVE ( 'NONE', #1402, #32484, #17657, .T. ) ;
#9784=DIRECTION ( 'NONE',  ( 1.000000000000000000, 0.000000000000000000, 0.000000000000000000 ) ) ;
#9787=CARTESIAN_POINT ( 'NONE',  ( 9.999999999999479527, 5.773502691896553074, -101.2500000040967763 ) ) ;
#9788=CARTESIAN_POINT ( 'NONE',  ( 10.81189881249999907, 6.242252689847868297, -160.4062500020484094 ) ) ;
#9789=CARTESIAN_POINT ( 'NONE',  ( -10.81189881249999907, -6.242252689847864744, -145.9687500020484094 ) ) ;
#9790=CYLINDRICAL_SURFACE ( 'NONE', #15982, 9.999999999999998224 ) ;
#9793=CARTESIAN_POINT ( 'NONE',  ( 9.999999999999998224, 0.000000000000000000, -189.8750000040967905 ) ) ;
#9795=CARTESIAN_POINT ( 'NONE',  ( 10.81189881249999729, 0.000000000000000000, -69.03125000204838102 ) ) ;
#9797=CARTESIAN_POINT ( 'NONE',  ( -10.81189881249999729, 1.324075727343319199E-15, -117.5937500020483810 ) ) ;
#9800=CARTESIAN_POINT ( 'NONE',  ( -5.405949406250003975, -9.363379034771801557, -21.34375000204835615 ) ) ;
#9801=CARTESIAN_POINT ( 'NONE',  ( 7.644554776091147741E-16, 12.48450537969573659, -198.9687500020484094 ) ) ;
#9802=CARTESIAN_POINT ( 'NONE',  ( 10.81189881249999907, 6.242252689847868297, -47.71875000204835970 ) ) ;
#9803=CARTESIAN_POINT ( 'NONE',  ( -9.999999999999998224, 1.224646799147353059E-15, -72.12500000409677625 ) ) ;
#9805=CARTESIAN_POINT ( 'NONE',  ( 5.405949406249999534, 9.363379034771803333, -181.0937500020483810 ) ) ;
#9806=CARTESIAN_POINT ( 'NONE',  ( -5.405949406249996869, 9.363379034771805109, -171.8437500020484094 ) ) ;
#9808=VECTOR ( 'NONE', #7453, 1000.000000000000000 ) ;
#9812=CARTESIAN_POINT ( 'NONE',  ( 10.81189881249999907, 6.242252689847868297, -94.21875000204838102 ) ) ;
#9813=CARTESIAN_POINT ( 'NONE',  ( 9.999999999999998224, 0.000000000000000000, -200.0000000000000000 ) ) ;
#9814=CARTESIAN_POINT ( 'NONE',  ( 5.405949406249992428, -9.363379034771808662, -73.78125000204838102 ) ) ;
#9816=CARTESIAN_POINT ( 'NONE',  ( 10.81189881249999729, 6.242252689847867408, -163.4062500020483810 ) ) ;
#9818=CARTESIAN_POINT ( 'NONE',  ( 9.999999999999996447, -5.773502691896262640, -142.0000000040967905 ) ) ;
#9823=VECTOR ( 'NONE', #25142, 1000.000000000000000 ) ;
#9824=DIRECTION ( 'NONE',  ( -0.000000000000000000, -0.000000000000000000, 1.000000000000000000 ) ) ;
#9827=CARTESIAN_POINT ( 'NONE',  ( -2.121150477449813534E-15, -11.54700538379251284, -57.87499999999998579 ) ) ;
#9829=CARTESIAN_POINT ( 'NONE',  ( 5.000000000000000000, 8.660254037844385522, -62.12500000409676204 ) ) ;
#9830=EDGE_CURVE ( 'NONE', #21964, #414, #5058, .T. ) ;
#9831=EDGE_CURVE ( 'NONE', #35094, #6, #40752, .T. ) ;
#9833=CARTESIAN_POINT ( 'NONE',  ( 4.999999999999992006, -8.660254037844389075, -144.7500000000000000 ) ) ;
#9836=CARTESIAN_POINT ( 'NONE',  ( 5.405949406249999534, 9.363379034771803333, -68.78125000204838102 ) ) ;
#9840=CARTESIAN_POINT ( 'NONE',  ( -10.00000000000051337, 5.773502691895962435, -37.75000000409675494 ) ) ;
#9841=CARTESIAN_POINT ( 'NONE',  ( 5.405949406249999534, 9.363379034771803333, -188.7812500020484094 ) ) ;
#9843=CARTESIAN_POINT ( 'NONE',  ( -10.81189881249999729, 6.242252689847871849, -0.7187500020483512664 ) ) ;
#9844=CARTESIAN_POINT ( 'NONE',  ( -9.999999999999998224, 1.224646799147353059E-15, -118.2500000000000000 ) ) ;
#9845=CARTESIAN_POINT ( 'NONE',  ( -5.000000000000003553, -8.660254037844383745, -45.99999999999998579 ) ) ;
#9847=CARTESIAN_POINT ( 'NONE',  ( -9.999999999999998224, 1.836970198721029589E-15, 0.000000000000000000 ) ) ;
#9848=CARTESIAN_POINT ( 'NONE',  ( -4.999999999999996447, 8.660254037844387298, -166.5000000000000000 ) ) ;
#9849=CARTESIAN_POINT ( 'NONE',  ( -5.000000000000003553, -8.660254037844383745, -36.99999999999997868 ) ) ;
#9850=CARTESIAN_POINT ( 'NONE',  ( 5.405949406249992428, -9.363379034771808662, -94.78125000204838102 ) ) ;
#9852=DIRECTION ( 'NONE',  ( 1.000000000000000000, 0.000000000000000000, 0.000000000000000000 ) ) ;
#9855=ORIENTED_EDGE ( 'NONE', *, *, #13702, .F. ) ;
#9856=ORIENTED_EDGE ( 'NONE', *, *, #38885, .T. ) ;
#9857=CARTESIAN_POINT ( 'NONE',  ( -2.293366432827344421E-15, -12.48450537969573659, -33.21875000204834549 ) ) ;
#9858=CARTESIAN_POINT ( 'NONE',  ( -10.81189881249999729, 1.324075727343319199E-15, -24.78125000204836681 ) ) ;
#9860=EDGE_CURVE ( 'NONE', #29087, #29783, #19915, .T. ) ;
#9861=CARTESIAN_POINT ( 'NONE',  ( 10.81189881249999907, 6.242252689847868297, -73.21875000204836681 ) ) ;
#9863=EDGE_CURVE ( 'NONE', #8912, #28824, #31543, .T. ) ;
#9864=CARTESIAN_POINT ( 'NONE',  ( 10.81189881249999729, 0.000000000000000000, -190.3437500020484094 ) ) ;
#9867=CARTESIAN_POINT ( 'NONE',  ( -4.999999999999996447, 8.660254037844387298, -6.375000004096770034 ) ) ;
#9868=FACE_OUTER_BOUND ( 'NONE', #26266, .T. ) ;
#9869=CARTESIAN_POINT ( 'NONE',  ( -5.405949406249996869, 9.363379034771805109, -120.8437500020483952 ) ) ;
#9870=CARTESIAN_POINT ( 'NONE',  ( -10.81189881249999729, 6.242252689847871849, -98.40625000204838102 ) ) ;
#9871=CARTESIAN_POINT ( 'NONE',  ( 10.81189881249999551, -6.242252689847874514, -109.4687500020483952 ) ) ;
#9872=EDGE_CURVE ( 'NONE', #15363, #18023, #40316, .T. ) ;
#9875=CARTESIAN_POINT ( 'NONE',  ( -10.00000000000000000, -5.773502691896251982, -165.0000000040967905 ) ) ;
#9876=( BOUNDED_CURVE ( )  B_SPLINE_CURVE ( 2, ( #25369, #15412, #28608, #35297, #38734, #5727, #18880 ),
 .UNSPECIFIED., .F., .F. ) 
 B_SPLINE_CURVE_WITH_KNOTS ( ( 3, 2, 2, 3 ),
 ( 0.8582089552238808539, 0.8594527363184081281, 0.8606965174129356244, 0.8619402985074630097 ),
 .UNSPECIFIED. ) 
 CURVE ( )  GEOMETRIC_REPRESENTATION_ITEM ( )  RATIONAL_B_SPLINE_CURVE ( ( 0.9999999999999761302, 0.8660254037844625774, 1.000000000000000000, 0.8660254037844387076, 1.000000000000000000, 0.8660254037844028474, 1.000000000000035971 ) ) 
 REPRESENTATION_ITEM ( '' )  );
#9877=CARTESIAN_POINT ( 'NONE',  ( -9.999999999999998224, 1.224646799147353059E-15, -67.24999999999997158 ) ) ;
#9883=CARTESIAN_POINT ( 'NONE',  ( 10.00000000000154010, -5.773502691895370020, -53.50000000409673362 ) ) ;
#9885=CARTESIAN_POINT ( 'NONE',  ( 9.999999999999998224, 0.000000000000000000, -78.49999999999998579 ) ) ;
#9887=CARTESIAN_POINT ( 'NONE',  ( 9.999999999999996447, -5.773502691896262640, -98.50000000409677625 ) ) ;
#9890=CARTESIAN_POINT ( 'NONE',  ( -2.293366432827344421E-15, -12.48450537969573659, -88.90625000204838102 ) ) ;
#9893=CARTESIAN_POINT ( 'NONE',  ( -9.999999999999998224, 1.224646799147353059E-15, -73.62500000409677625 ) ) ;
#9896=CARTESIAN_POINT ( 'NONE',  ( -10.00000000000000000, -5.773502691896251982, -7.124999999999969802 ) ) ;
#9897=CARTESIAN_POINT ( 'NONE',  ( 9.999999999999996447, -5.773502691896262640, -149.1250000000000000 ) ) ;
#9900=CARTESIAN_POINT ( 'NONE',  ( -5.000000000000003553, -8.660254037844383745, -193.0000000000000000 ) ) ;
#9901=CARTESIAN_POINT ( 'NONE',  ( 5.405949406249992428, -9.363379034771808662, -121.7812500020483952 ) ) ;
#9902=VERTEX_POINT ( 'NONE', #21123 ) ;
#9903=CYLINDRICAL_SURFACE ( 'NONE', #16548, 9.999999999999998224 ) ;
#9904=ORIENTED_EDGE ( 'NONE', *, *, #4319, .T. ) ;
#9905=CARTESIAN_POINT ( 'NONE',  ( 10.81189881249999729, 0.000000000000000000, -42.03125000204838102 ) ) ;
#9907=CARTESIAN_POINT ( 'NONE',  ( -10.81189881249999729, 6.242252689847871849, -107.2187500020483810 ) ) ;
#9908=CARTESIAN_POINT ( 'NONE',  ( -5.405949406249996869, 9.363379034771805109, -122.5312500020483952 ) ) ;
#9909=VERTEX_POINT ( 'NONE', #11612 ) ;
#9910=CARTESIAN_POINT ( 'NONE',  ( -9.999999999999227285, -5.773502691896698735, -133.1249999999999716 ) ) ;
#9911=CARTESIAN_POINT ( 'NONE',  ( 9.999999999999479527, 5.773502691896553074, -78.37499999999995737 ) ) ;
#9913=CARTESIAN_POINT ( 'NONE',  ( -9.999999999999998224, 1.224646799147353059E-15, -26.74999999999996803 ) ) ;
#9914=CARTESIAN_POINT ( 'NONE',  ( 9.999999999998969713, 5.773502691896851502, -0.7500000040967217396 ) ) ;
#9915=CARTESIAN_POINT ( 'NONE',  ( -10.81189881249999729, -6.242252689847864744, -129.4687500020483810 ) ) ;
#9919=CARTESIAN_POINT ( 'NONE',  ( 4.999999999999992006, -8.660254037844389075, -184.1250000040967905 ) ) ;
#9921=CARTESIAN_POINT ( 'NONE',  ( 5.405949406249992428, -9.363379034771808662, -183.2812500020484094 ) ) ;
#9924=CARTESIAN_POINT ( 'NONE',  ( 7.644554776091147741E-16, 12.48450537969573659, -57.96875000204836681 ) ) ;
#9925=CARTESIAN_POINT ( 'NONE',  ( -5.405949406250003975, -9.363379034771801557, -46.84375000204838102 ) ) ;
#9927=CARTESIAN_POINT ( 'NONE',  ( 5.405949406249999534, 9.363379034771803333, -14.78125000204835793 ) ) ;
#9931=CARTESIAN_POINT ( 'NONE',  ( -5.000000000000003553, -8.660254037844383745, -104.4999999999999858 ) ) ;
#9933=CARTESIAN_POINT ( 'NONE',  ( 5.000000000000000000, 8.660254037844385522, -119.1250000040967905 ) ) ;
#9936=CARTESIAN_POINT ( 'NONE',  ( 7.644554776091147741E-16, 12.48450537969573659, -119.6562500020484094 ) ) ;
#9937=ORIENTED_EDGE ( 'NONE', *, *, #252, .T. ) ;
#9938=CARTESIAN_POINT ( 'NONE',  ( 9.999999999999998224, 0.000000000000000000, -6.499999999999977796 ) ) ;
#9941=ORIENTED_EDGE ( 'NONE', *, *, #36841, .T. ) ;
#9942=CARTESIAN_POINT ( 'NONE',  ( 9.999999999999998224, 0.000000000000000000, -30.49999999999997158 ) ) ;
#9943=CARTESIAN_POINT ( 'NONE',  ( 7.070501591499377789E-16, 11.54700538379251284, -20.00000000409677625 ) ) ;
#9944=CARTESIAN_POINT ( 'NONE',  ( -10.81189881249999729, 1.324075727343319199E-15, -44.28125000204838102 ) ) ;
#9945=CARTESIAN_POINT ( 'NONE',  ( -9.999999999999998224, 1.224646799147353059E-15, -200.0000000000000000 ) ) ;
#9947=DIRECTION ( 'NONE',  ( 0.000000000000000000, 0.000000000000000000, -1.000000000000000000 ) ) ;
#9948=CARTESIAN_POINT ( 'NONE',  ( -2.293366432827344421E-15, -12.48450537969573659, -136.9062500020484094 ) ) ;
#9949=EDGE_CURVE ( 'NONE', #9613, #23672, #10834, .T. ) ;
#9950=CARTESIAN_POINT ( 'NONE',  ( 5.405949406249992428, -9.363379034771808662, -138.2812500020483810 ) ) ;
#9951=DIRECTION ( 'NONE',  ( 1.000000000000000000, 0.000000000000000000, 0.000000000000000000 ) ) ;
#9952=ORIENTED_EDGE ( 'NONE', *, *, #10185, .F. ) ;
#9954=VERTEX_POINT ( 'NONE', #11832 ) ;
#9955=( BOUNDED_CURVE ( )  B_SPLINE_CURVE ( 2, ( #23684, #34468, #4247, #11347, #10705, #23901, #21282 ),
 .UNSPECIFIED., .F., .F. ) 
 B_SPLINE_CURVE_WITH_KNOTS ( ( 3, 2, 2, 3 ),
 ( 0.6865671641791046831, 0.6878109452736320684, 0.6890547263681594536, 0.6902985074626868389 ),
 .UNSPECIFIED. ) 
 CURVE ( )  GEOMETRIC_REPRESENTATION_ITEM ( )  RATIONAL_B_SPLINE_CURVE ( ( 0.9999999999999761302, 0.8660254037844625774, 1.000000000000000000, 0.8660254037844387076, 1.000000000000000000, 0.8660254037844148378, 1.000000000000023981 ) ) 
 REPRESENTATION_ITEM ( '' )  );
#9957=CARTESIAN_POINT ( 'NONE',  ( 9.999999999999998224, 0.000000000000000000, -200.0000000000000000 ) ) ;
#9958=CARTESIAN_POINT ( 'NONE',  ( -5.405949406249996869, 9.363379034771805109, -173.3437500020484094 ) ) ;
#9959=CARTESIAN_POINT ( 'NONE',  ( 10.81189881249999729, 0.000000000000000000, -22.34375000204835615 ) ) ;
#9960=CARTESIAN_POINT ( 'NONE',  ( -9.999999999999998224, 1.224646799147353059E-15, -129.1250000040967620 ) ) ;
#9961=CARTESIAN_POINT ( 'NONE',  ( -10.81189881249999729, 1.324075727343319199E-15, -156.5937500020483810 ) ) ;
#9962=CARTESIAN_POINT ( 'NONE',  ( 10.81189881249999907, 6.242252689847868297, -148.2187500020484094 ) ) ;
#9963=CARTESIAN_POINT ( 'NONE',  ( -2.121150477449813534E-15, -11.54700538379251284, -9.874999999999982236 ) ) ;
#9966=CARTESIAN_POINT ( 'NONE',  ( 7.644554776091147741E-16, 12.48450537969573659, -18.96875000204837391 ) ) ;
#9968=DIRECTION ( 'NONE',  ( -0.000000000000000000, -0.000000000000000000, 1.000000000000000000 ) ) ;
#9971=CARTESIAN_POINT ( 'NONE',  ( 4.999999999999992006, -8.660254037844389075, -167.6250000040967905 ) ) ;
#9972=CARTESIAN_POINT ( 'NONE',  ( -10.81189881249999729, 6.242252689847871849, -72.71875000204835260 ) ) ;
#9973=CARTESIAN_POINT ( 'NONE',  ( 5.405949406249999534, 9.363379034771803333, -44.78125000204838102 ) ) ;
#9977=CARTESIAN_POINT ( 'NONE',  ( 10.00000000000000000, 5.773502691896255534, -129.3750000000000000 ) ) ;
#9978=CARTESIAN_POINT ( 'NONE',  ( 10.81189881249999551, -6.242252689847874514, -136.6562500020484094 ) ) ;
#9979=CARTESIAN_POINT ( 'NONE',  ( 9.999999999999998224, 0.000000000000000000, -98.37500000409677625 ) ) ;
#9980=CARTESIAN_POINT ( 'NONE',  ( -5.000000000000003553, -8.660254037844383745, -110.8750000040967763 ) ) ;
#9982=EDGE_LOOP ( 'NONE', ( #11520, #19248, #9120, #27863 ) ) ;
#9985=CARTESIAN_POINT ( 'NONE',  ( -9.999999999999998224, 1.224646799147353059E-15, -200.0000000000000000 ) ) ;
#9986=CARTESIAN_POINT ( 'NONE',  ( -2.293366432827344421E-15, -12.48450537969573659, -160.9062500020483810 ) ) ;
#9987=CARTESIAN_POINT ( 'NONE',  ( -9.999999999999998224, 5.773502691896259087, -45.25000000409676915 ) ) ;
#9988=CYLINDRICAL_SURFACE ( 'NONE', #27662, 9.999999999999998224 ) ;
#9990=EDGE_CURVE ( 'NONE', #10829, #24501, #37311, .T. ) ;
#9991=CARTESIAN_POINT ( 'NONE',  ( 10.81189881249999907, 6.242252689847868297, -163.4062500020484094 ) ) ;
#9992=CARTESIAN_POINT ( 'NONE',  ( 10.81189881249999729, 0.000000000000000000, -137.8437500020484094 ) ) ;
#9993=CARTESIAN_POINT ( 'NONE',  ( -9.999999999999998224, 1.224646799147353059E-15, -200.0000000000000000 ) ) ;
#9995=ORIENTED_EDGE ( 'NONE', *, *, #41316, .T. ) ;
#9996=CARTESIAN_POINT ( 'NONE',  ( -12.99038105676666888, -7.500000000000057732, 49.99999999999998579 ) ) ;
#9997=( BOUNDED_CURVE ( )  B_SPLINE_CURVE ( 2, ( #12138, #31379, #41273, #24695, #5253, #22082, #38263 ),
 .UNSPECIFIED., .F., .F. ) 
 B_SPLINE_CURVE_WITH_KNOTS ( ( 3, 2, 2, 3 ),
 ( 0.4402985074626867279, 0.4415422885572141132, 0.4427860696517414429, 0.4440298507462688282 ),
 .UNSPECIFIED. ) 
 CURVE ( )  GEOMETRIC_REPRESENTATION_ITEM ( )  RATIONAL_B_SPLINE_CURVE ( ( 0.9999999999999820144, 0.8660254037844566932, 1.000000000000000000, 0.8660254037844387076, 1.000000000000000000, 0.8660254037844207220, 1.000000000000017986 ) ) 
 REPRESENTATION_ITEM ( '' )  );
#9998=CARTESIAN_POINT ( 'NONE',  ( 10.81189881249999729, 0.000000000000000000, -73.53125000204838102 ) ) ;
#10001=CARTESIAN_POINT ( 'NONE',  ( -5.405949406250003975, -9.363379034771801557, -117.3437500020483810 ) ) ;
#10002=ORIENTED_EDGE ( 'NONE', *, *, #16038, .T. ) ;
#10003=ORIENTED_EDGE ( 'NONE', *, *, #2805, .T. ) ;
#10004=VECTOR ( 'NONE', #10783, 1000.000000000000000 ) ;
#10005=CARTESIAN_POINT ( 'NONE',  ( -2.293366432827344421E-15, -12.48450537969573659, -22.71875000204837391 ) ) ;
#10006=CARTESIAN_POINT ( 'NONE',  ( 5.405949406249992428, -9.363379034771808662, -196.5937500020484094 ) ) ;
#10008=CARTESIAN_POINT ( 'NONE',  ( -5.405949406249996869, 9.363379034771805109, -44.34375000204837391 ) ) ;
#10010=EDGE_CURVE ( 'NONE', #27538, #36032, #19665, .T. ) ;
#10012=CARTESIAN_POINT ( 'NONE',  ( -10.81189881249999729, 1.324075727343319199E-15, -179.0937500020484094 ) ) ;
#10013=VECTOR ( 'NONE', #10164, 1000.000000000000000 ) ;
#10014=CARTESIAN_POINT ( 'NONE',  ( -5.405949406249996869, 9.363379034771805109, -167.3437500020484094 ) ) ;
#10017=LINE ( 'NONE', #33132, #6768 ) ;
#10020=CARTESIAN_POINT ( 'NONE',  ( 10.81189881249999729, 0.000000000000000000, -100.3437500020483810 ) ) ;
#10022=CARTESIAN_POINT ( 'NONE',  ( -10.81189881249999907, -6.242252689847864744, -65.15625000204838102 ) ) ;
#10024=CARTESIAN_POINT ( 'NONE',  ( -5.405949406250003975, -9.363379034771801557, -120.5312500020483952 ) ) ;
#10025=CARTESIAN_POINT ( 'NONE',  ( -5.405949406250003975, -9.363379034771801557, -164.0312500020484094 ) ) ;
#10027=CARTESIAN_POINT ( 'NONE',  ( -9.999999999999998224, 5.773502691896259087, -141.2500000040967905 ) ) ;
#10029=ORIENTED_EDGE ( 'NONE', *, *, #25344, .F. ) ;
#10032=CARTESIAN_POINT ( 'NONE',  ( 10.81189881249999907, 6.242252689847868297, -193.4062500020484094 ) ) ;
#10033=CARTESIAN_POINT ( 'NONE',  ( 10.00000000000000000, 5.773502691896255534, -131.2500000040967905 ) ) ;
#10035=ORIENTED_EDGE ( 'NONE', *, *, #7513, .F. ) ;
#10036=CARTESIAN_POINT ( 'NONE',  ( 9.999999999999998224, 0.000000000000000000, -54.49999999999996447 ) ) ;
#10038=CARTESIAN_POINT ( 'NONE',  ( 7.070501591499377789E-16, 11.54700538379251284, -69.50000000409679046 ) ) ;
#10039=CYLINDRICAL_SURFACE ( 'NONE', #343, 9.999999999999998224 ) ;
#10040=FACE_OUTER_BOUND ( 'NONE', #14721, .T. ) ;
#10042=VECTOR ( 'NONE', #17756, 1000.000000000000000 ) ;
#10043=CARTESIAN_POINT ( 'NONE',  ( 10.81189881249999551, -6.242252689847874514, -60.15625000204838813 ) ) ;
#10044=VECTOR ( 'NONE', #15879, 1000.000000000000000 ) ;
#10047=LINE ( 'NONE', #22803, #23490 ) ;
#10048=CARTESIAN_POINT ( 'NONE',  ( 10.81189881249999729, 0.000000000000000000, -186.0312500020484094 ) ) ;
#10050=LINE ( 'NONE', #39200, #2185 ) ;
#10052=AXIS2_PLACEMENT_3D ( 'NONE', #7855, #10434, #324 ) ;
#10055=CARTESIAN_POINT ( 'NONE',  ( 4.999999999999992006, -8.660254037844389075, -167.2500000000000000 ) ) ;
#10056=CARTESIAN_POINT ( 'NONE',  ( 9.999999999999998224, 0.000000000000000000, -168.8750000040967905 ) ) ;
#10058=CARTESIAN_POINT ( 'NONE',  ( -5.405949406250003975, -9.363379034771801557, -95.03125000204838102 ) ) ;
#10060=CARTESIAN_POINT ( 'NONE',  ( 9.999999999999998224, 0.000000000000000000, -180.8750000040967905 ) ) ;
#10062=EDGE_LOOP ( 'NONE', ( #35120, #639, #26318, #20504 ) ) ;
#10063=ORIENTED_EDGE ( 'NONE', *, *, #26217, .T. ) ;
#10064=CARTESIAN_POINT ( 'NONE',  ( -5.405949406250003975, -9.363379034771801557, -34.84375000204836681 ) ) ;
#10065=CARTESIAN_POINT ( 'NONE',  ( 10.81189881249999551, -6.242252689847874514, -19.65625000204837747 ) ) ;
#10067=CARTESIAN_POINT ( 'NONE',  ( 10.81189881249999907, 6.242252689847868297, -70.21875000204840944 ) ) ;
#10068=CARTESIAN_POINT ( 'NONE',  ( 9.999999999999998224, 0.000000000000000000, -173.3750000040968189 ) ) ;
#10069=EDGE_CURVE ( 'NONE', #38354, #41544, #1723, .T. ) ;
#10070=CARTESIAN_POINT ( 'NONE',  ( -5.405949406249996869, 9.363379034771805109, -195.8437500020484094 ) ) ;
#10071=CARTESIAN_POINT ( 'NONE',  ( 10.81189881249999551, -6.242252689847874514, -152.9687500020484094 ) ) ;
#10072=EDGE_CURVE ( 'NONE', #10798, #22060, #28519, .T. ) ;
#10074=DIRECTION ( 'NONE',  ( -0.000000000000000000, -0.000000000000000000, 1.000000000000000000 ) ) ;
#10077=CARTESIAN_POINT ( 'NONE',  ( 4.999999999999992006, -8.660254037844389075, -7.125000004096743389 ) ) ;
#10078=CARTESIAN_POINT ( 'NONE',  ( 10.81189881249999907, 6.242252689847868297, -122.7187500020483810 ) ) ;
#10079=CARTESIAN_POINT ( 'NONE',  ( 9.999999999999998224, 0.000000000000000000, -15.49999999999995737 ) ) ;
#10080=CARTESIAN_POINT ( 'NONE',  ( -2.293366432827344421E-15, -12.48450537969573659, -87.40625000204838102 ) ) ;
#10081=CARTESIAN_POINT ( 'NONE',  ( -5.405949406250003975, -9.363379034771801557, -109.8437500020483810 ) ) ;
#10084=CARTESIAN_POINT ( 'NONE',  ( 10.00000000000000000, 5.773502691896255534, -164.2500000040967905 ) ) ;
#10085=CARTESIAN_POINT ( 'NONE',  ( -2.121150477449813534E-15, -11.54700538379251284, -11.37499999999995737 ) ) ;
#10091=CARTESIAN_POINT ( 'NONE',  ( 5.000000000000000000, 8.660254037844385522, -81.24999999999998579 ) ) ;
#10093=CARTESIAN_POINT ( 'NONE',  ( 4.999999999999992006, -8.660254037844389075, -92.62500000409677625 ) ) ;
#10094=ADVANCED_FACE ( 'NONE', ( #26293 ), #9037, .T. ) ;
#10097=CARTESIAN_POINT ( 'NONE',  ( -10.81189881249999729, -6.242252689847864744, -84.65625000204836681 ) ) ;
#10098=VERTEX_POINT ( 'NONE', #22202 ) ;
#10100=CARTESIAN_POINT ( 'NONE',  ( 7.070501591499376803E-16, 11.54700538379251284, -48.12499999999997158 ) ) ;
#10102=VERTEX_POINT ( 'NONE', #26079 ) ;
#10103=CARTESIAN_POINT ( 'NONE',  ( -4.999999999999996447, 8.660254037844387298, -10.49999999999995381 ) ) ;
#10104=CARTESIAN_POINT ( 'NONE',  ( 5.000000000000000000, 8.660254037844385522, -147.2500000000000000 ) ) ;
#10105=CARTESIAN_POINT ( 'NONE',  ( -9.999999999999998224, 1.224646799147353059E-15, -15.12500000409674961 ) ) ;
#10106=EDGE_CURVE ( 'NONE', #6565, #22119, #32911, .T. ) ;
#10108=CARTESIAN_POINT ( 'NONE',  ( 10.00000000000000000, 5.773502691896255534, -193.8750000000000284 ) ) ;
#10109=PLANE ( 'NONE',  #22036 ) ;
#10110=CARTESIAN_POINT ( 'NONE',  ( 10.81189881249999729, 0.000000000000000000, -115.5312500020483952 ) ) ;
#10111=ORIENTED_EDGE ( 'NONE', *, *, #1444, .T. ) ;
#10112=LINE ( 'NONE', #19821, #6933 ) ;
#10113=EDGE_LOOP ( 'NONE', ( #33426, #3365, #17108, #36037 ) ) ;
#10114=CARTESIAN_POINT ( 'NONE',  ( -2.293366432827344421E-15, -12.48450537969573659, -49.90625000204838102 ) ) ;
#10116=CARTESIAN_POINT ( 'NONE',  ( 5.405949406249999534, 9.363379034771803333, -97.09375000204838102 ) ) ;
#10117=CARTESIAN_POINT ( 'NONE',  ( -10.81189881249999729, 6.242252689847871849, -123.9062500020483810 ) ) ;
#10118=ADVANCED_FACE ( 'NONE', ( #6643 ), #19793, .T. ) ;
#10120=CARTESIAN_POINT ( 'NONE',  ( 9.999999999999998224, 0.000000000000000000, -84.87500000409677625 ) ) ;
#10121=DIRECTION ( 'NONE',  ( -0.000000000000000000, -0.000000000000000000, 1.000000000000000000 ) ) ;
#10122=( BOUNDED_CURVE ( )  B_SPLINE_CURVE ( 2, ( #33149, #10033, #3579, #26447, #13049, #16713, #29478 ),
 .UNSPECIFIED., .F., .F. ) 
 B_SPLINE_CURVE_WITH_KNOTS ( ( 3, 2, 2, 3 ),
 ( 0.3358208955223880854, 0.3370646766169154707, 0.3383084577114429670, 0.3395522388059703522 ),
 .UNSPECIFIED. ) 
 CURVE ( )  GEOMETRIC_REPRESENTATION_ITEM ( )  RATIONAL_B_SPLINE_CURVE ( ( 1.000000000000000000, 0.8660254037844387076, 1.000000000000000000, 0.8660254037844387076, 1.000000000000000000, 0.8660254037844148378, 1.000000000000023981 ) ) 
 REPRESENTATION_ITEM ( '' )  );
#10123=EDGE_CURVE ( 'NONE', #33268, #33809, #3920, .T. ) ;
#10125=CARTESIAN_POINT ( 'NONE',  ( -10.00000000000102496, 5.773502691895664007, -13.75000000409673184 ) ) ;
#10126=ADVANCED_FACE ( 'NONE', ( #35588 ), #39022, .T. ) ;
#10127=CARTESIAN_POINT ( 'NONE',  ( -10.81189881249999729, 1.324075727343319199E-15, -132.5937500020483810 ) ) ;
#10130=CARTESIAN_POINT ( 'NONE',  ( 10.00000000000000000, 5.773502691896255534, -186.7500000040967905 ) ) ;
#10132=CARTESIAN_POINT ( 'NONE',  ( -5.405949406250003975, -9.363379034771801557, -183.5312500020484094 ) ) ;
#10133=CARTESIAN_POINT ( 'NONE',  ( 9.999999999999998224, 0.000000000000000000, -149.3750000040967905 ) ) ;
#10134=DIRECTION ( 'NONE',  ( -0.4999999999999998890, -0.8660254037844387076, 0.000000000000000000 ) ) ;
#10137=CARTESIAN_POINT ( 'NONE',  ( 10.81189881249999729, 6.242252689847867408, -61.21875000204838813 ) ) ;
#10138=CARTESIAN_POINT ( 'NONE',  ( -2.293366432827344421E-15, -12.48450537969573659, -49.71875000204835970 ) ) ;
#10140=CARTESIAN_POINT ( 'NONE',  ( 7.644554776091147741E-16, 12.48450537969573659, -17.65625000204836681 ) ) ;
#10142=CARTESIAN_POINT ( 'NONE',  ( -9.999999999999998224, 1.224646799147353059E-15, -124.6250000040967763 ) ) ;
#10144=CARTESIAN_POINT ( 'NONE',  ( -9.999999999999998224, 1.224646799147353059E-15, -106.2499999999999858 ) ) ;
#10146=CARTESIAN_POINT ( 'NONE',  ( 9.999999999999998224, 0.000000000000000000, -27.49999999999996803 ) ) ;
#10149=CARTESIAN_POINT ( 'NONE',  ( -10.81189881249999729, 1.324075727343319199E-15, -111.7812500020483810 ) ) ;
#10150=EDGE_CURVE ( 'NONE', #29288, #26359, #17130, .T. ) ;
#10151=ORIENTED_EDGE ( 'NONE', *, *, #23826, .T. ) ;
#10156=VERTEX_POINT ( 'NONE', #2991 ) ;
#10157=CARTESIAN_POINT ( 'NONE',  ( 10.00000000000000000, 5.773502691896255534, -33.37499999999996447 ) ) ;
#10158=CARTESIAN_POINT ( 'NONE',  ( 9.999999999999996447, -5.773502691896262640, -19.00000000409676915 ) ) ;
#10159=CARTESIAN_POINT ( 'NONE',  ( -5.405949406249996869, 9.363379034771805109, -46.03125000204838813 ) ) ;
#10160=DIRECTION ( 'NONE',  ( -0.000000000000000000, -0.000000000000000000, 1.000000000000000000 ) ) ;
#10162=CARTESIAN_POINT ( 'NONE',  ( -9.999999999999998224, 1.224646799147353059E-15, -107.7499999999999858 ) ) ;
#10163=CARTESIAN_POINT ( 'NONE',  ( -10.81189881249999907, -6.242252689847864744, -143.1562500020484094 ) ) ;
#10164=DIRECTION ( 'NONE',  ( -0.000000000000000000, -0.000000000000000000, 1.000000000000000000 ) ) ;
#10166=ORIENTED_EDGE ( 'NONE', *, *, #38108, .T. ) ;
#10167=VERTEX_POINT ( 'NONE', #42457 ) ;
#10168=DIRECTION ( 'NONE',  ( -0.000000000000000000, -0.000000000000000000, 1.000000000000000000 ) ) ;
#10169=CARTESIAN_POINT ( 'NONE',  ( 0.000000000000000000, 0.000000000000000000, -200.0000000000000000 ) ) ;
#10170=CARTESIAN_POINT ( 'NONE',  ( -5.405949406250003975, -9.363379034771801557, -174.3437500020484094 ) ) ;
#10171=CARTESIAN_POINT ( 'NONE',  ( -5.405949406249996869, 9.363379034771805109, -24.84375000204835970 ) ) ;
#10172=FACE_OUTER_BOUND ( 'NONE', #36876, .T. ) ;
#10173=VECTOR ( 'NONE', #24333, 1000.000000000000000 ) ;
#10174=CARTESIAN_POINT ( 'NONE',  ( 10.81189881249999729, 6.242252689847867408, -158.7187500020484094 ) ) ;
#10175=CARTESIAN_POINT ( 'NONE',  ( 10.81189881249999907, 6.242252689847868297, -142.2187500020484094 ) ) ;
#10176=CARTESIAN_POINT ( 'NONE',  ( 10.00000000000102318, -5.773502691895667560, -88.00000000409673362 ) ) ;
#10179=CARTESIAN_POINT ( 'NONE',  ( 5.405949406249992428, -9.363379034771808662, -13.59375000204834905 ) ) ;
#10184=CARTESIAN_POINT ( 'NONE',  ( 4.999999999999992006, -8.660254037844389075, -17.24999999999996092 ) ) ;
#10185=EDGE_CURVE ( 'NONE', #2553, #1094, #22410, .T. ) ;
#10186=CARTESIAN_POINT ( 'NONE',  ( 10.81189881249999729, 0.000000000000000000, -71.84375000204836681 ) ) ;
#10187=CARTESIAN_POINT ( 'NONE',  ( 5.405949406249999534, 9.363379034771803333, -41.78125000204838102 ) ) ;
#10189=CARTESIAN_POINT ( 'NONE',  ( -5.000000000000003553, -8.660254037844383745, -113.8750000040967763 ) ) ;
#10191=CARTESIAN_POINT ( 'NONE',  ( 5.000000000000000000, 8.660254037844385522, -127.7499999999999716 ) ) ;
#10192=CARTESIAN_POINT ( 'NONE',  ( -2.293366432827344421E-15, -12.48450537969573659, -141.4062500020484094 ) ) ;
#10194=CARTESIAN_POINT ( 'NONE',  ( -2.121150477449813534E-15, -11.54700538379251284, -113.7500000040967905 ) ) ;
#10196=VERTEX_POINT ( 'NONE', #15701 ) ;
#10199=DIRECTION ( 'NONE',  ( -0.000000000000000000, -0.000000000000000000, 1.000000000000000000 ) ) ;
#10200=CARTESIAN_POINT ( 'NONE',  ( 10.81189881249999551, -6.242252689847874514, -166.6562500020484094 ) ) ;
#10201=CARTESIAN_POINT ( 'NONE',  ( -10.00000000000000000, -5.773502691896251982, -39.00000000409676915 ) ) ;
#10202=CARTESIAN_POINT ( 'NONE',  ( 9.999999999999998224, 0.000000000000000000, -90.87500000409677625 ) ) ;
#10204=CARTESIAN_POINT ( 'NONE',  ( 9.999999999999998224, 0.000000000000000000, -63.49999999999997158 ) ) ;
#10205=CARTESIAN_POINT ( 'NONE',  ( 5.405949406249992428, -9.363379034771808662, -160.7812500020484094 ) ) ;
#10206=CARTESIAN_POINT ( 'NONE',  ( -5.405949406249996869, 9.363379034771805109, -134.3437500020484094 ) ) ;
#10207=CARTESIAN_POINT ( 'NONE',  ( -9.999999999999998224, 1.224646799147353059E-15, -51.12500000409675494 ) ) ;
#10208=CARTESIAN_POINT ( 'NONE',  ( -9.999999999999918288, -5.773502691896298167, -196.1250000000000284 ) ) ;
#10210=( BOUNDED_CURVE ( )  B_SPLINE_CURVE ( 2, ( #8148, #14594, #1249, #21296, #11148, #30391, #20867 ),
 .UNSPECIFIED., .F., .F. ) 
 B_SPLINE_CURVE_WITH_KNOTS ( ( 3, 2, 2, 3 ),
 ( 0.3880597014925373789, 0.3893034825870647087, 0.3905472636815920939, 0.3917910447761194792 ),
 .UNSPECIFIED. ) 
 CURVE ( )  GEOMETRIC_REPRESENTATION_ITEM ( )  RATIONAL_B_SPLINE_CURVE ( ( 0.9999999999999940048, 0.8660254037844447028, 1.000000000000000000, 0.8660254037844387076, 1.000000000000000000, 0.8660254037844327124, 1.000000000000005995 ) ) 
 REPRESENTATION_ITEM ( '' )  );
#10212=CARTESIAN_POINT ( 'NONE',  ( -5.405949406250003975, -9.363379034771801557, -68.03125000204838102 ) ) ;
#10215=CARTESIAN_POINT ( 'NONE',  ( 10.81189881249999551, -6.242252689847874514, -116.9687500020483952 ) ) ;
#10216=ORIENTED_EDGE ( 'NONE', *, *, #6673, .F. ) ;
#10217=CARTESIAN_POINT ( 'NONE',  ( 5.405949406249992428, -9.363379034771808662, -22.59375000204835615 ) ) ;
#10218=CARTESIAN_POINT ( 'NONE',  ( 7.644554776091147741E-16, 12.48450537969573659, -1.156250002048369474 ) ) ;
#10219=CARTESIAN_POINT ( 'NONE',  ( 10.81189881249999907, 6.242252689847868297, -46.21875000204837391 ) ) ;
#10220=LINE ( 'NONE', #19726, #33020 ) ;
#10221=CARTESIAN_POINT ( 'NONE',  ( 9.999999999999998224, 0.000000000000000000, -0.4999999999999726885 ) ) ;
#10222=CARTESIAN_POINT ( 'NONE',  ( 10.81189881249999551, -6.242252689847874514, -176.9687500020484094 ) ) ;
#10223=CARTESIAN_POINT ( 'NONE',  ( -10.81189881249999729, 1.324075727343319199E-15, -171.5937500020484094 ) ) ;
#10226=CARTESIAN_POINT ( 'NONE',  ( -9.999999999999479527, -5.773502691896549521, -105.0000000040967620 ) ) ;
#10227=CARTESIAN_POINT ( 'NONE',  ( 9.999999999999998224, 0.000000000000000000, -194.3750000040967905 ) ) ;
#10229=CARTESIAN_POINT ( 'NONE',  ( 5.405949406249999534, 9.363379034771803333, -98.59375000204838102 ) ) ;
#10230=CARTESIAN_POINT ( 'NONE',  ( 9.999999999999998224, 0.000000000000000000, -72.49999999999998579 ) ) ;
#10231=CARTESIAN_POINT ( 'NONE',  ( 7.644554776091147741E-16, 12.48450537969573659, -67.15625000204838102 ) ) ;
#10232=CARTESIAN_POINT ( 'NONE',  ( -5.000000000000003553, -8.660254037844383745, -5.499999999999976907 ) ) ;
#10234=CARTESIAN_POINT ( 'NONE',  ( 7.644554776091147741E-16, 12.48450537969573659, -119.6562500020484094 ) ) ;
#10235=CARTESIAN_POINT ( 'NONE',  ( 10.81189881249999729, 6.242252689847867408, -160.4062500020483810 ) ) ;
#10237=CARTESIAN_POINT ( 'NONE',  ( -4.999999999999996447, 8.660254037844387298, -141.3750000040967905 ) ) ;
#10239=ORIENTED_EDGE ( 'NONE', *, *, #6160, .T. ) ;
#10242=CARTESIAN_POINT ( 'NONE',  ( -5.405949406249996869, 9.363379034771805109, -191.5312500020484094 ) ) ;
#10243=CARTESIAN_POINT ( 'NONE',  ( -9.999999999999998224, 1.224646799147353059E-15, -43.62500000409677625 ) ) ;
#10245=VERTEX_POINT ( 'NONE', #6439 ) ;
#10246=CARTESIAN_POINT ( 'NONE',  ( -9.999999999999998224, 1.224646799147353059E-15, -56.74999999999996447 ) ) ;
#10248=CARTESIAN_POINT ( 'NONE',  ( -4.999999999999996447, 8.660254037844387298, -69.37500000409677625 ) ) ;
#10249=ADVANCED_FACE ( 'NONE', ( #19582 ), #42668, .T. ) ;
#10250=CARTESIAN_POINT ( 'NONE',  ( 4.999999999999992006, -8.660254037844389075, -109.1250000040967763 ) ) ;
#10253=CARTESIAN_POINT ( 'NONE',  ( -2.293366432827344421E-15, -12.48450537969573659, -55.90625000204837391 ) ) ;
#10254=( BOUNDED_CURVE ( )  B_SPLINE_CURVE ( 2, ( #35990, #593, #30154, #9653, #13294, #13079, #10068 ),
 .UNSPECIFIED., .F., .F. ) 
 B_SPLINE_CURVE_WITH_KNOTS ( ( 3, 2, 2, 3 ),
 ( 0.1231343283582089221, 0.1243781094527362935, 0.1256218905472636649, 0.1268656716417910224 ),
 .UNSPECIFIED. ) 
 CURVE ( )  GEOMETRIC_REPRESENTATION_ITEM ( )  RATIONAL_B_SPLINE_CURVE ( ( 1.000000000000002887, 0.8660254037844355990, 1.000000000000000000, 0.8660254037844387076, 1.000000000000000000, 0.8660254037844417052, 0.9999999999999970024 ) ) 
 REPRESENTATION_ITEM ( '' )  );
#10258=CARTESIAN_POINT ( 'NONE',  ( -2.293366432827344421E-15, -12.48450537969573659, -183.4062500020483810 ) ) ;
#10260=CARTESIAN_POINT ( 'NONE',  ( -9.999999999999998224, 1.224646799147353059E-15, -79.24999999999998579 ) ) ;
#10262=CARTESIAN_POINT ( 'NONE',  ( 9.999999999999998224, 0.000000000000000000, -200.0000000000000000 ) ) ;
#10263=CYLINDRICAL_SURFACE ( 'NONE', #27268, 9.999999999999998224 ) ;
#10264=( BOUNDED_CURVE ( )  B_SPLINE_CURVE ( 2, ( #13129, #20262, #33449, #39265, #36877, #29560, #26536 ),
 .UNSPECIFIED., .F., .F. ) 
 B_SPLINE_CURVE_WITH_KNOTS ( ( 3, 2, 2, 3 ),
 ( 0.5783582089552241623, 0.5796019900497515476, 0.5808457711442788218, 0.5820895522388062071 ),
 .UNSPECIFIED. ) 
 CURVE ( )  GEOMETRIC_REPRESENTATION_ITEM ( )  RATIONAL_B_SPLINE_CURVE ( ( 0.9999999999999641398, 0.8660254037844745678, 1.000000000000000000, 0.8660254037844387076, 1.000000000000000000, 0.8660254037844148378, 1.000000000000023981 ) ) 
 REPRESENTATION_ITEM ( '' )  );
#10265=CARTESIAN_POINT ( 'NONE',  ( 7.070501591499377789E-16, 11.54700538379251284, -166.6249999999999716 ) ) ;
#10266=CARTESIAN_POINT ( 'NONE',  ( 4.999999999999992006, -8.660254037844389075, -62.24999999999997158 ) ) ;
#10267=CARTESIAN_POINT ( 'NONE',  ( -10.81189881249999729, 1.324075727343319199E-15, -90.78125000204838102 ) ) ;
#10268=ORIENTED_EDGE ( 'NONE', *, *, #16204, .T. ) ;
#10269=CARTESIAN_POINT ( 'NONE',  ( 7.070501591499376803E-16, 11.54700538379251284, -107.0000000040967763 ) ) ;
#10270=CARTESIAN_POINT ( 'NONE',  ( -9.999999999999998224, 1.224646799147353059E-15, -70.24999999999998579 ) ) ;
#10272=ORIENTED_EDGE ( 'NONE', *, *, #14973, .T. ) ;
#10273=CARTESIAN_POINT ( 'NONE',  ( -10.81189881249999907, -6.242252689847864744, -31.96875000204835970 ) ) ;
#10274=CARTESIAN_POINT ( 'NONE',  ( 5.405949406249992428, -9.363379034771808662, -18.28125000204835970 ) ) ;
#10275=AXIS2_PLACEMENT_3D ( 'NONE', #41128, #21294, #1459 ) ;
#10276=CARTESIAN_POINT ( 'NONE',  ( -5.405949406250003975, -9.363379034771801557, -69.34375000204836681 ) ) ;
#10278=CARTESIAN_POINT ( 'NONE',  ( 7.644554776091147741E-16, 12.48450537969573659, -195.9687500020484094 ) ) ;
#10279=CARTESIAN_POINT ( 'NONE',  ( -10.81189881249999729, 6.242252689847871849, -152.2187500020483526 ) ) ;
#10280=DIRECTION ( 'NONE',  ( 1.000000000000000000, 0.000000000000000000, 0.000000000000000000 ) ) ;
#10281=VECTOR ( 'NONE', #11195, 1000.000000000000000 ) ;
#10284=CARTESIAN_POINT ( 'NONE',  ( -2.121150477449813534E-15, -11.54700538379251284, -5.750000004096770923 ) ) ;
#10285=CARTESIAN_POINT ( 'NONE',  ( -9.999999999999479527, -5.773502691896549521, -80.62499999999997158 ) ) ;
#10286=CARTESIAN_POINT ( 'NONE',  ( -2.293366432827344421E-15, -12.48450537969573659, -121.7187500020483952 ) ) ;
#10288=CARTESIAN_POINT ( 'NONE',  ( -2.293366432827344421E-15, -12.48450537969573659, -93.40625000204839523 ) ) ;
#10289=CARTESIAN_POINT ( 'NONE',  ( 10.81189881249999729, 6.242252689847867408, -106.2187500020483810 ) ) ;
#10292=CARTESIAN_POINT ( 'NONE',  ( 7.070501591499377789E-16, 11.54700538379251284, -159.5000000040967905 ) ) ;
#10298=CARTESIAN_POINT ( 'NONE',  ( 9.999999999999998224, 0.000000000000000000, -9.875000004096746054 ) ) ;
#10300=CARTESIAN_POINT ( 'NONE',  ( 10.00000000000000000, 5.773502691896255534, -79.87499999999998579 ) ) ;
#10302=CARTESIAN_POINT ( 'NONE',  ( -9.999999999999998224, 1.224646799147353059E-15, -88.62500000409677625 ) ) ;
#10303=CARTESIAN_POINT ( 'NONE',  ( -10.00000000000000000, -5.773502691896252870, -172.1250000000000284 ) ) ;
#10305=CARTESIAN_POINT ( 'NONE',  ( -10.81189881249999729, 6.242252689847871849, -86.40625000204838102 ) ) ;
#10310=ORIENTED_EDGE ( 'NONE', *, *, #35327, .T. ) ;
#10311=CARTESIAN_POINT ( 'NONE',  ( -9.999999999999998224, 1.224646799147353059E-15, -5.749999999999976907 ) ) ;
#10315=CARTESIAN_POINT ( 'NONE',  ( -5.000000000000003553, -8.660254037844383745, -148.0000000000000000 ) ) ;
#10316=CARTESIAN_POINT ( 'NONE',  ( 10.00000000000102318, -5.773502691895667560, -32.12499999999992895 ) ) ;
#10318=CARTESIAN_POINT ( 'NONE',  ( 9.999999999999996447, -5.773502691896262640, -194.1250000000000284 ) ) ;
#10319=CYLINDRICAL_SURFACE ( 'NONE', #40610, 9.999999999999998224 ) ;
#10320=CARTESIAN_POINT ( 'NONE',  ( 5.405949406249999534, 9.363379034771803333, -119.7812500020483952 ) ) ;
#10323=ORIENTED_EDGE ( 'NONE', *, *, #6971, .T. ) ;
#10324=CARTESIAN_POINT ( 'NONE',  ( -10.81189881249999729, 1.324075727343319199E-15, -44.28125000204838102 ) ) ;
#10326=CARTESIAN_POINT ( 'NONE',  ( 10.81189881249999729, 0.000000000000000000, -94.34375000204838102 ) ) ;
#10327=CARTESIAN_POINT ( 'NONE',  ( -5.405949406249996869, 9.363379034771805109, -125.5312500020483952 ) ) ;
#10328=ORIENTED_EDGE ( 'NONE', *, *, #41868, .T. ) ;
#10329=( BOUNDED_CURVE ( )  B_SPLINE_CURVE ( 2, ( #24832, #8422, #34754, #31518, #1947, #15073, #28274 ),
 .UNSPECIFIED., .F., .F. ) 
 B_SPLINE_CURVE_WITH_KNOTS ( ( 3, 2, 2, 3 ),
 ( 0.5820895522388062071, 0.5833333333333335924, 0.5845771144278607556, 0.5858208955223881409 ),
 .UNSPECIFIED. ) 
 CURVE ( )  GEOMETRIC_REPRESENTATION_ITEM ( )  RATIONAL_B_SPLINE_CURVE ( ( 0.9999999999999761302, 0.8660254037844625774, 1.000000000000000000, 0.8660254037844387076, 1.000000000000000000, 0.8660254037844267172, 1.000000000000011990 ) ) 
 REPRESENTATION_ITEM ( '' )  );
#10330=CARTESIAN_POINT ( 'NONE',  ( -9.999999999999998224, 1.224646799147353059E-15, -5.749999999999976907 ) ) ;
#10332=CYLINDRICAL_SURFACE ( 'NONE', #32138, 9.999999999999998224 ) ;
#10333=AXIS2_PLACEMENT_3D ( 'NONE', #27748, #40883, #34661 ) ;
#10334=CARTESIAN_POINT ( 'NONE',  ( 10.81189881249999551, -6.242252689847874514, -131.9687500020483810 ) ) ;
#10336=CARTESIAN_POINT ( 'NONE',  ( 9.999999999999998224, 0.000000000000000000, -43.99999999999998579 ) ) ;
#10338=CARTESIAN_POINT ( 'NONE',  ( 5.000000000000000000, 8.660254037844385522, -183.6250000040967905 ) ) ;
#10340=CARTESIAN_POINT ( 'NONE',  ( -5.405949406250003975, -9.363379034771801557, -182.0312500020483810 ) ) ;
#10341=CARTESIAN_POINT ( 'NONE',  ( -4.999999999999996447, 8.660254037844387298, -2.999999999999975131 ) ) ;
#10342=CARTESIAN_POINT ( 'NONE',  ( 7.070501591499376803E-16, 11.54700538379251284, -181.6250000000000000 ) ) ;
#10344=CARTESIAN_POINT ( 'NONE',  ( 10.81189881249999729, 6.242252689847867408, -62.71875000204839523 ) ) ;
#10345=CARTESIAN_POINT ( 'NONE',  ( -5.405949406249996869, 9.363379034771805109, -41.34375000204837391 ) ) ;
#10347=CARTESIAN_POINT ( 'NONE',  ( 10.81189881249999907, 6.242252689847868297, -20.90625000204836681 ) ) ;
#10349=FACE_OUTER_BOUND ( 'NONE', #8261, .T. ) ;
#10351=CARTESIAN_POINT ( 'NONE',  ( -2.121150477449813534E-15, -11.54700538379251284, -108.8749999999999858 ) ) ;
#10355=CARTESIAN_POINT ( 'NONE',  ( 10.81189881249999729, 0.000000000000000000, -108.0312500020483810 ) ) ;
#10356=ORIENTED_EDGE ( 'NONE', *, *, #41809, .T. ) ;
#10361=CARTESIAN_POINT ( 'NONE',  ( -4.999999999999996447, 8.660254037844387298, -29.99999999999997158 ) ) ;
#10362=ADVANCED_FACE ( 'NONE', ( #28900 ), #12885, .T. ) ;
#10363=ADVANCED_FACE ( 'NONE', ( #32356 ), #2780, .T. ) ;
#10364=CARTESIAN_POINT ( 'NONE',  ( 5.405949406249992428, -9.363379034771808662, -31.78125000204837391 ) ) ;
#10365=EDGE_CURVE ( 'NONE', #39621, #4388, #1185, .T. ) ;
#10369=CARTESIAN_POINT ( 'NONE',  ( -10.81189881249999907, -6.242252689847864744, -141.6562500020483810 ) ) ;
#10371=CARTESIAN_POINT ( 'NONE',  ( 9.999999999999998224, 0.000000000000000000, -167.3750000040967905 ) ) ;
#10373=( BOUNDED_CURVE ( )  B_SPLINE_CURVE ( 2, ( #35514, #29030, #9167, #8543, #21695, #2698, #2074 ),
 .UNSPECIFIED., .F., .F. ) 
 B_SPLINE_CURVE_WITH_KNOTS ( ( 3, 2, 2, 3 ),
 ( 0.3992537313432836799, 0.4004975124378110651, 0.4017412935323383949, 0.4029850746268657802 ),
 .UNSPECIFIED. ) 
 CURVE ( )  GEOMETRIC_REPRESENTATION_ITEM ( )  RATIONAL_B_SPLINE_CURVE ( ( 0.9999999999999880096, 0.8660254037844506980, 1.000000000000000000, 0.8660254037844387076, 1.000000000000000000, 0.8660254037844267172, 1.000000000000011990 ) ) 
 REPRESENTATION_ITEM ( '' )  );
#10375=CARTESIAN_POINT ( 'NONE',  ( 5.000000000000000000, 8.660254037844385522, -114.2499999999999858 ) ) ;
#10376=CARTESIAN_POINT ( 'NONE',  ( 0.000000000000000000, 0.000000000000000000, -200.0000000000000000 ) ) ;
#10377=CARTESIAN_POINT ( 'NONE',  ( 10.81189881249999907, 6.242252689847868297, -163.2187500020483810 ) ) ;
#10380=CARTESIAN_POINT ( 'NONE',  ( -10.81189881249999729, 6.242252689847871849, -20.21875000204836326 ) ) ;
#10383=CARTESIAN_POINT ( 'NONE',  ( 7.644554776091147741E-16, 12.48450537969573659, -155.4687500020484094 ) ) ;
#10384=CARTESIAN_POINT ( 'NONE',  ( 10.81189881249999907, 6.242252689847868297, -139.2187500020484094 ) ) ;
#10385=CARTESIAN_POINT ( 'NONE',  ( -9.999999999999998224, 1.224646799147353059E-15, -172.6250000040968189 ) ) ;
#10389=CARTESIAN_POINT ( 'NONE',  ( -10.81189881249999729, 1.324075727343319199E-15, -8.093750002048343717 ) ) ;
#10391=CARTESIAN_POINT ( 'NONE',  ( -9.999999999999998224, 1.224646799147353059E-15, -172.6250000040968189 ) ) ;
#10395=CARTESIAN_POINT ( 'NONE',  ( 10.81189881249999551, -6.242252689847874514, -80.96875000204838102 ) ) ;
#10396=CARTESIAN_POINT ( 'NONE',  ( -10.81189881249999729, 6.242252689847871849, -63.71875000204838102 ) ) ;
#10397=CARTESIAN_POINT ( 'NONE',  ( -2.293366432827344421E-15, -12.48450537969573659, -40.90625000204836681 ) ) ;
#10399=CARTESIAN_POINT ( 'NONE',  ( 10.00000000000051159, -5.773502691895965988, -113.5000000040967620 ) ) ;
#10401=CARTESIAN_POINT ( 'NONE',  ( -10.00000000000000000, -5.773502691896251982, -128.6250000000000000 ) ) ;
#10402=CARTESIAN_POINT ( 'NONE',  ( -10.81189881249999729, -6.242252689847864744, -138.6562500020484094 ) ) ;
#10403=EDGE_CURVE ( 'NONE', #25696, #35021, #19162, .T. ) ;
#10404=CARTESIAN_POINT ( 'NONE',  ( 10.00000000000154010, -5.773502691895370020, -23.50000000409674072 ) ) ;
#10406=CARTESIAN_POINT ( 'NONE',  ( 10.81189881249999551, -6.242252689847874514, -19.65625000204837391 ) ) ;
#10411=CARTESIAN_POINT ( 'NONE',  ( -2.121150477449813534E-15, -11.54700538379251284, -44.75000000409676204 ) ) ;
#10412=LINE ( 'NONE', #33104, #38688 ) ;
#10414=CARTESIAN_POINT ( 'NONE',  ( 4.999999999999992006, -8.660254037844389075, -191.2500000000000000 ) ) ;
#10415=CARTESIAN_POINT ( 'NONE',  ( -5.405949406249996869, 9.363379034771805109, -158.5312500020484094 ) ) ;
#10416=CARTESIAN_POINT ( 'NONE',  ( -10.81189881249999729, 1.324075727343319199E-15, -137.0937500020483810 ) ) ;
#10418=CARTESIAN_POINT ( 'NONE',  ( 4.999999999999992006, -8.660254037844389075, -115.1250000040967905 ) ) ;
#10420=DIRECTION ( 'NONE',  ( -0.6123724356957962467, -0.3535533905932750631, 0.7071067811865454633 ) ) ;
#10422=EDGE_CURVE ( 'NONE', #33095, #795, #20008, .T. ) ;
#10423=CARTESIAN_POINT ( 'NONE',  ( 10.81189881249999907, 6.242252689847868297, -61.40625000204838102 ) ) ;
#10426=CARTESIAN_POINT ( 'NONE',  ( 10.81189881249999551, -6.242252689847874514, -115.4687500020483810 ) ) ;
#10427=ORIENTED_EDGE ( 'NONE', *, *, #12999, .T. ) ;
#10428=CARTESIAN_POINT ( 'NONE',  ( 10.81189881249999551, -6.242252689847874514, -20.96875000204836681 ) ) ;
#10430=CARTESIAN_POINT ( 'NONE',  ( 10.81189881249999729, 0.000000000000000000, -194.8437500020484094 ) ) ;
#10431=AXIS2_PLACEMENT_3D ( 'NONE', #16513, #33166, #16728 ) ;
#10432=CARTESIAN_POINT ( 'NONE',  ( -10.81189881249999729, 6.242252689847871849, -50.21875000204836681 ) ) ;
#10433=CARTESIAN_POINT ( 'NONE',  ( -8.659811548901195977, -5.000849327365069819, 0.000000000000000000 ) ) ;
#10434=DIRECTION ( 'NONE',  ( -0.000000000000000000, -0.000000000000000000, 1.000000000000000000 ) ) ;
#10435=CARTESIAN_POINT ( 'NONE',  ( -10.81189881249999729, 6.242252689847871849, -176.2187500020483810 ) ) ;
#10436=CARTESIAN_POINT ( 'NONE',  ( -10.81189881249999907, -6.242252689847864744, -157.9687500020484379 ) ) ;
#10439=FACE_OUTER_BOUND ( 'NONE', #25934, .T. ) ;
#10442=CARTESIAN_POINT ( 'NONE',  ( -5.405949406250003975, -9.363379034771801557, -96.34375000204838102 ) ) ;
#10443=CARTESIAN_POINT ( 'NONE',  ( 9.999999999999998224, 0.000000000000000000, -183.5000000000000000 ) ) ;
#10444=CARTESIAN_POINT ( 'NONE',  ( 5.405949406249992428, -9.363379034771808662, -67.78125000204838102 ) ) ;
#10445=CARTESIAN_POINT ( 'NONE',  ( 4.999999999999992006, -8.660254037844389075, -97.12500000409677625 ) ) ;
#10447=CARTESIAN_POINT ( 'NONE',  ( -2.293366432827344421E-15, -12.48450537969573659, -120.4062500020483952 ) ) ;
#10448=CARTESIAN_POINT ( 'NONE',  ( 10.81189881249999729, 0.000000000000000000, -159.0312500020484094 ) ) ;
#10450=CARTESIAN_POINT ( 'NONE',  ( -4.999999999999996447, 8.660254037844387298, -138.3750000040967905 ) ) ;
#10453=ORIENTED_EDGE ( 'NONE', *, *, #34124, .T. ) ;
#10456=CARTESIAN_POINT ( 'NONE',  ( 10.81189881249999729, 0.000000000000000000, -187.5312500020484094 ) ) ;
#10458=VERTEX_POINT ( 'NONE', #17985 ) ;
#10459=CARTESIAN_POINT ( 'NONE',  ( 9.999999999999998224, 0.000000000000000000, -48.49999999999998579 ) ) ;
#10461=CARTESIAN_POINT ( 'NONE',  ( -2.121150477449813534E-15, -11.54700538379251284, -65.75000000409679046 ) ) ;
#10463=( BOUNDED_CURVE ( )  B_SPLINE_CURVE ( 2, ( #6607, #42631, #13061, #26255, #39404, #9840, #32944 ),
 .UNSPECIFIED., .F., .F. ) 
 B_SPLINE_CURVE_WITH_KNOTS ( ( 3, 2, 2, 3 ),
 ( 0.7985074626865673597, 0.7997512437810947450, 0.8009950248756220192, 0.8022388059701494045 ),
 .UNSPECIFIED. ) 
 CURVE ( )  GEOMETRIC_REPRESENTATION_ITEM ( )  RATIONAL_B_SPLINE_CURVE ( ( 0.9999999999999761302, 0.8660254037844625774, 1.000000000000000000, 0.8660254037844387076, 1.000000000000000000, 0.8660254037844267172, 1.000000000000011990 ) ) 
 REPRESENTATION_ITEM ( '' )  );
#10465=CARTESIAN_POINT ( 'NONE',  ( -10.81189881249999729, 1.324075727343319199E-15, -62.28125000204837391 ) ) ;
#10469=CARTESIAN_POINT ( 'NONE',  ( -5.405949406249996869, 9.363379034771805109, -185.5312500020484094 ) ) ;
#10470=AXIS2_PLACEMENT_3D ( 'NONE', #22539, #29230, #3324 ) ;
#10473=CARTESIAN_POINT ( 'NONE',  ( 9.999999999999998224, 0.000000000000000000, -88.99999999999998579 ) ) ;
#10475=CARTESIAN_POINT ( 'NONE',  ( 9.999999999999998224, 0.000000000000000000, -200.0000000000000000 ) ) ;
#10476=CARTESIAN_POINT ( 'NONE',  ( 5.405949406249992428, -9.363379034771808662, -90.28125000204838102 ) ) ;
#10478=CARTESIAN_POINT ( 'NONE',  ( -2.121150477449813534E-15, -11.54700538379251284, -162.8750000000000000 ) ) ;
#10479=DIRECTION ( 'NONE',  ( 1.000000000000000000, 0.000000000000000000, 0.000000000000000000 ) ) ;
#10480=VERTEX_POINT ( 'NONE', #11511 ) ;
#10481=ORIENTED_EDGE ( 'NONE', *, *, #10010, .T. ) ;
#10482=AXIS2_PLACEMENT_3D ( 'NONE', #15050, #5151, #7960 ) ;
#10483=CARTESIAN_POINT ( 'NONE',  ( 10.81189881249999551, -6.242252689847874514, -22.46875000204837391 ) ) ;
#10484=CARTESIAN_POINT ( 'NONE',  ( 10.81189881249999907, 6.242252689847868297, -22.40625000204837747 ) ) ;
#10486=CARTESIAN_POINT ( 'NONE',  ( -10.81189881249999729, 6.242252689847871849, -68.21875000204838102 ) ) ;
#10487=CARTESIAN_POINT ( 'NONE',  ( 0.000000000000000000, 0.000000000000000000, -200.0000000000000000 ) ) ;
#10489=CARTESIAN_POINT ( 'NONE',  ( -10.81189881249999907, -6.242252689847864744, -195.4687500020484094 ) ) ;
#10490=CARTESIAN_POINT ( 'NONE',  ( -5.405949406250003975, -9.363379034771801557, -150.3437500020483810 ) ) ;
#10491=EDGE_CURVE ( 'NONE', #27538, #8850, #31396, .T. ) ;
#10492=CARTESIAN_POINT ( 'NONE',  ( 7.070501591499376803E-16, 11.54700538379251284, -72.50000000409677625 ) ) ;
#10495=CARTESIAN_POINT ( 'NONE',  ( -9.999999999999998224, 1.224646799147353059E-15, -4.625000004096769146 ) ) ;
#10496=CARTESIAN_POINT ( 'NONE',  ( -9.999999999999998224, 1.224646799147353059E-15, -200.0000000000000000 ) ) ;
#10497=CARTESIAN_POINT ( 'NONE',  ( 7.644554776091147741E-16, 12.48450537969573659, -119.4687500020483952 ) ) ;
#10498=DIRECTION ( 'NONE',  ( 1.000000000000000000, 0.000000000000000000, 0.000000000000000000 ) ) ;
#10499=CARTESIAN_POINT ( 'NONE',  ( 5.405949406249999534, 9.363379034771803333, -88.28125000204838102 ) ) ;
#10500=CARTESIAN_POINT ( 'NONE',  ( -10.81189881249999729, 6.242252689847871849, -102.7187500020483810 ) ) ;
#10503=CARTESIAN_POINT ( 'NONE',  ( -4.999999999999996447, 8.660254037844387298, -160.8750000040967905 ) ) ;
#10504=( BOUNDED_CURVE ( )  B_SPLINE_CURVE ( 2, ( #4802, #37396, #7839, #34814, #20986, #4591, #11265 ),
 .UNSPECIFIED., .F., .F. ) 
 B_SPLINE_CURVE_WITH_KNOTS ( ( 3, 2, 2, 3 ),
 ( 0.2537313432835822113, 0.2549751243781095411, 0.2562189054726369264, 0.2574626865671643117 ),
 .UNSPECIFIED. ) 
 CURVE ( )  GEOMETRIC_REPRESENTATION_ITEM ( )  RATIONAL_B_SPLINE_CURVE ( ( 0.9999999999999880096, 0.8660254037844506980, 1.000000000000000000, 0.8660254037844387076, 1.000000000000000000, 0.8660254037844267172, 1.000000000000011990 ) ) 
 REPRESENTATION_ITEM ( '' )  );
#10508=FACE_OUTER_BOUND ( 'NONE', #24152, .T. ) ;
#10509=CARTESIAN_POINT ( 'NONE',  ( 9.999999999999998224, 0.000000000000000000, -79.99999999999998579 ) ) ;
#10511=CARTESIAN_POINT ( 'NONE',  ( -10.00000000000000000, -5.773502691896251982, -79.12499999999998579 ) ) ;
#10513=CARTESIAN_POINT ( 'NONE',  ( -5.000000000000003553, -8.660254037844383745, -86.87500000409677625 ) ) ;
#10514=DIRECTION ( 'NONE',  ( -0.000000000000000000, -0.000000000000000000, 1.000000000000000000 ) ) ;
#10516=CARTESIAN_POINT ( 'NONE',  ( -5.405949406249996869, 9.363379034771805109, -80.53125000204838102 ) ) ;
#10517=( BOUNDED_CURVE ( )  B_SPLINE_CURVE ( 2, ( #647, #9910, #33659, #39686, #22878, #30425, #26745 ),
 .UNSPECIFIED., .F., .F. ) 
 B_SPLINE_CURVE_WITH_KNOTS ( ( 3, 2, 2, 3 ),
 ( 0.3320895522388061516, 0.3333333333333334259, 0.3345771144278607556, 0.3358208955223880854 ),
 .UNSPECIFIED. ) 
 CURVE ( )  GEOMETRIC_REPRESENTATION_ITEM ( )  RATIONAL_B_SPLINE_CURVE ( ( 0.9999999999999820144, 0.8660254037844566932, 1.000000000000000000, 0.8660254037844387076, 1.000000000000000000, 0.8660254037844387076, 1.000000000000000000 ) ) 
 REPRESENTATION_ITEM ( '' )  );
#10519=DIRECTION ( 'NONE',  ( 0.000000000000000000, -0.000000000000000000, -1.000000000000000000 ) ) ;
#10521=ORIENTED_EDGE ( 'NONE', *, *, #2444, .T. ) ;
#10522=CARTESIAN_POINT ( 'NONE',  ( 5.000000000000000000, 8.660254037844385522, -12.24999999999995559 ) ) ;
#10525=CARTESIAN_POINT ( 'NONE',  ( -9.999999999999998224, 5.773502691896259087, -145.3750000000000000 ) ) ;
#10526=DIRECTION ( 'NONE',  ( -0.000000000000000000, -0.000000000000000000, 1.000000000000000000 ) ) ;
#10529=CARTESIAN_POINT ( 'NONE',  ( 4.999999999999992006, -8.660254037844389075, -192.7500000000000000 ) ) ;
#10531=CARTESIAN_POINT ( 'NONE',  ( -10.81189881249999729, 6.242252689847871849, -114.9062500020483952 ) ) ;
#10533=ORIENTED_EDGE ( 'NONE', *, *, #32563, .F. ) ;
#10535=CARTESIAN_POINT ( 'NONE',  ( 10.81189881249999907, 6.242252689847868297, -47.90625000204836681 ) ) ;
#10537=CARTESIAN_POINT ( 'NONE',  ( -10.81189881249999729, 1.324075727343319199E-15, -95.09375000204838102 ) ) ;
#10538=CARTESIAN_POINT ( 'NONE',  ( 10.81189881249999729, 0.000000000000000000, -121.5312500020483952 ) ) ;
#10541=CARTESIAN_POINT ( 'NONE',  ( 5.405949406249992428, -9.363379034771808662, -198.0937500020484094 ) ) ;
#10543=LINE ( 'NONE', #23521, #9381 ) ;
#10545=CARTESIAN_POINT ( 'NONE',  ( -10.81189881249999729, 6.242252689847871849, -120.7187500020483952 ) ) ;
#10549=CARTESIAN_POINT ( 'NONE',  ( 4.999999999999992006, -8.660254037844389075, -182.6250000040967905 ) ) ;
#10551=CARTESIAN_POINT ( 'NONE',  ( 5.405949406249999534, 9.363379034771803333, -179.7812500020484094 ) ) ;
#10554=CARTESIAN_POINT ( 'NONE',  ( 5.405949406249992428, -9.363379034771808662, -58.59375000204835970 ) ) ;
#10555=CARTESIAN_POINT ( 'NONE',  ( 5.405949406249999534, 9.363379034771803333, -40.09375000204837391 ) ) ;
#10557=CARTESIAN_POINT ( 'NONE',  ( 5.405949406249992428, -9.363379034771808662, -15.28125000204835793 ) ) ;
#10561=CARTESIAN_POINT ( 'NONE',  ( 4.999999999999992006, -8.660254037844389075, -104.2499999999999858 ) ) ;
#10563=LINE ( 'NONE', #7779, #33461 ) ;
#10566=CARTESIAN_POINT ( 'NONE',  ( -10.81189881249999729, 1.324075727343319199E-15, -108.7812500020483810 ) ) ;
#10567=ORIENTED_EDGE ( 'NONE', *, *, #17511, .T. ) ;
#10568=CARTESIAN_POINT ( 'NONE',  ( -9.999999999999998224, 1.224646799147353059E-15, -7.249999999999978684 ) ) ;
#10570=CARTESIAN_POINT ( 'NONE',  ( 9.999999999999994671, -5.773502691896262640, -136.0000000040967905 ) ) ;
#10572=ORIENTED_EDGE ( 'NONE', *, *, #35256, .F. ) ;
#10573=CARTESIAN_POINT ( 'NONE',  ( -9.999999999999998224, 1.224646799147353059E-15, -35.74999999999997868 ) ) ;
#10574=CARTESIAN_POINT ( 'NONE',  ( -10.81189881249999729, 6.242252689847871849, -38.40625000204835260 ) ) ;
#10578=CARTESIAN_POINT ( 'NONE',  ( -10.81189881249999729, 1.324075727343319199E-15, -144.7812500020483810 ) ) ;
#10579=( BOUNDED_CURVE ( )  B_SPLINE_CURVE ( 2, ( #37013, #20602, #986, #26667, #27305, #20387, #20818 ),
 .UNSPECIFIED., .F., .F. ) 
 B_SPLINE_CURVE_WITH_KNOTS ( ( 3, 2, 2, 3 ),
 ( 0.1007462686567163757, 0.1019900497512437887, 0.1032338308457712017, 0.1044776119402986148 ),
 .UNSPECIFIED. ) 
 CURVE ( )  GEOMETRIC_REPRESENTATION_ITEM ( )  RATIONAL_B_SPLINE_CURVE ( ( 1.000000000000004441, 0.8660254037844342667, 1.000000000000000000, 0.8660254037844387076, 1.000000000000000000, 0.8660254037844267172, 1.000000000000011990 ) ) 
 REPRESENTATION_ITEM ( '' )  );
#10580=CARTESIAN_POINT ( 'NONE',  ( -10.00000000000012434, 5.773502691896184480, -166.7500000040967905 ) ) ;
#10583=CARTESIAN_POINT ( 'NONE',  ( -10.00000000000012434, 5.773502691896184480, -158.8750000000000000 ) ) ;
#10584=LINE ( 'NONE', #36926, #22172 ) ;
#10585=CARTESIAN_POINT ( 'NONE',  ( 10.81189881249999551, -6.242252689847874514, -169.4687500020483810 ) ) ;
#10588=CARTESIAN_POINT ( 'NONE',  ( 10.81189881249999551, -6.242252689847874514, -17.96875000204837036 ) ) ;
#10591=CARTESIAN_POINT ( 'NONE',  ( -5.405949406250003975, -9.363379034771801557, -157.8437500020483810 ) ) ;
#10592=CARTESIAN_POINT ( 'NONE',  ( 10.81189881249999729, 0.000000000000000000, -136.3437500020484094 ) ) ;
#10598=CARTESIAN_POINT ( 'NONE',  ( -2.293366432827344421E-15, -12.48450537969573659, -9.218750002048359704 ) ) ;
#10600=CARTESIAN_POINT ( 'NONE',  ( 0.000000000000000000, 0.000000000000000000, -200.0000000000000000 ) ) ;
#10603=CARTESIAN_POINT ( 'NONE',  ( -10.81189881249999729, 6.242252689847871849, -84.71875000204836681 ) ) ;
#10604=CARTESIAN_POINT ( 'NONE',  ( 7.644554776091147741E-16, 12.48450537969573659, -65.46875000204836681 ) ) ;
#10605=CARTESIAN_POINT ( 'NONE',  ( -9.999999999999998224, 1.224646799147353059E-15, -118.6250000040967905 ) ) ;
#10606=CARTESIAN_POINT ( 'NONE',  ( -5.405949406250003975, -9.363379034771801557, -44.03125000204838102 ) ) ;
#10608=LINE ( 'NONE', #13838, #28881 ) ;
#10610=CARTESIAN_POINT ( 'NONE',  ( -9.999999999999998224, 1.224646799147353059E-15, -133.2499999999999716 ) ) ;
#10611=CARTESIAN_POINT ( 'NONE',  ( -10.81189881249999729, -6.242252689847864744, -131.1562500020483810 ) ) ;
#10614=CARTESIAN_POINT ( 'NONE',  ( 10.81189881249999729, 6.242252689847867408, -20.90625000204836681 ) ) ;
#10615=VERTEX_POINT ( 'NONE', #15599 ) ;
#10618=DIRECTION ( 'NONE',  ( -0.000000000000000000, -0.000000000000000000, 1.000000000000000000 ) ) ;
#10619=CARTESIAN_POINT ( 'NONE',  ( -9.999999999999998224, 5.773502691896259087, -43.75000000409676204 ) ) ;
#10621=CARTESIAN_POINT ( 'NONE',  ( -9.999999999999998224, 1.224646799147353059E-15, -43.62500000409677625 ) ) ;
#10623=( BOUNDED_CURVE ( )  B_SPLINE_CURVE ( 2, ( #37586, #1559, #17710, #14032, #14690, #30905, #27879 ),
 .UNSPECIFIED., .F., .F. ) 
 B_SPLINE_CURVE_WITH_KNOTS ( ( 3, 2, 2, 3 ),
 ( 0.7201492537313435305, 0.7213930348258709158, 0.7226368159203983010, 0.7238805970149256863 ),
 .UNSPECIFIED. ) 
 CURVE ( )  GEOMETRIC_REPRESENTATION_ITEM ( )  RATIONAL_B_SPLINE_CURVE ( ( 0.9999999999999761302, 0.8660254037844625774, 1.000000000000000000, 0.8660254037844387076, 1.000000000000000000, 0.8660254037844028474, 1.000000000000035971 ) ) 
 REPRESENTATION_ITEM ( '' )  );
#10625=CARTESIAN_POINT ( 'NONE',  ( 5.405949406249999534, 9.363379034771803333, -149.7812500020483810 ) ) ;
#10626=CARTESIAN_POINT ( 'NONE',  ( -2.293366432827344421E-15, -12.48450537969573659, -133.7187500020483810 ) ) ;
#10630=DIRECTION ( 'NONE',  ( -0.8660254037844439257, 0.000000000000000000, 0.4999999999999907296 ) ) ;
#10632=CARTESIAN_POINT ( 'NONE',  ( -5.405949406250003975, -9.363379034771801557, -60.53125000204836681 ) ) ;
#10633=VERTEX_POINT ( 'NONE', #2676 ) ;
#10635=CARTESIAN_POINT ( 'NONE',  ( 5.405949406249992428, -9.363379034771808662, -111.0937500020483810 ) ) ;
#10636=ORIENTED_EDGE ( 'NONE', *, *, #22174, .F. ) ;
#10637=CARTESIAN_POINT ( 'NONE',  ( -10.81189881249999729, 1.324075727343319199E-15, -18.59375000204835260 ) ) ;
#10638=CARTESIAN_POINT ( 'NONE',  ( 10.81189881249999551, -6.242252689847874514, -191.9687500020484379 ) ) ;
#10639=CARTESIAN_POINT ( 'NONE',  ( 10.81189881249999729, 0.000000000000000000, -50.84375000204835260 ) ) ;
#10641=CARTESIAN_POINT ( 'NONE',  ( -5.000000000000003553, -8.660254037844383745, -31.37500000409676559 ) ) ;
#10642=CARTESIAN_POINT ( 'NONE',  ( -10.81189881249999729, 6.242252689847871849, -179.2187500020484379 ) ) ;
#10643=CARTESIAN_POINT ( 'NONE',  ( 10.81189881249999729, 0.000000000000000000, -163.3437500020484094 ) ) ;
#10646=EDGE_CURVE ( 'NONE', #37675, #3284, #18021, .T. ) ;
#10647=CARTESIAN_POINT ( 'NONE',  ( 10.00000000000051159, -5.773502691895965988, -93.62499999999997158 ) ) ;
#10648=CYLINDRICAL_SURFACE ( 'NONE', #10880, 9.999999999999998224 ) ;
#10650=EDGE_CURVE ( 'NONE', #3605, #41097, #29887, .T. ) ;
#10651=CARTESIAN_POINT ( 'NONE',  ( -5.405949406249996869, 9.363379034771805109, -92.34375000204838102 ) ) ;
#10652=CARTESIAN_POINT ( 'NONE',  ( 9.999999999999998224, 0.000000000000000000, -100.9999999999999858 ) ) ;
#10653=CARTESIAN_POINT ( 'NONE',  ( 10.81189881249999551, -6.242252689847874514, -69.15625000204839523 ) ) ;
#10654=CARTESIAN_POINT ( 'NONE',  ( 0.000000000000000000, 0.000000000000000000, -200.0000000000000000 ) ) ;
#10656=CARTESIAN_POINT ( 'NONE',  ( 5.405949406249992428, -9.363379034771808662, -126.2812500020483668 ) ) ;
#10657=CARTESIAN_POINT ( 'NONE',  ( 5.405949406249999534, 9.363379034771803333, -163.2812500020484094 ) ) ;
#10659=CARTESIAN_POINT ( 'NONE',  ( 10.00000000000000000, 5.773502691896255534, -132.7500000040967905 ) ) ;
#10661=VERTEX_POINT ( 'NONE', #38281 ) ;
#10665=CARTESIAN_POINT ( 'NONE',  ( 10.81189881249999729, 0.000000000000000000, -192.0312500020484094 ) ) ;
#10667=ORIENTED_EDGE ( 'NONE', *, *, #20133, .F. ) ;
#10668=CARTESIAN_POINT ( 'NONE',  ( -9.999999999999998224, 1.224646799147353059E-15, -49.24999999999998579 ) ) ;
#10670=CARTESIAN_POINT ( 'NONE',  ( -5.000000000000003553, -8.660254037844383745, -65.87500000409676204 ) ) ;
#10671=CARTESIAN_POINT ( 'NONE',  ( 9.999999999999998224, 0.000000000000000000, -21.87500000409675494 ) ) ;
#10672=CARTESIAN_POINT ( 'NONE',  ( -2.121150477449813534E-15, -11.54700538379251284, -165.8750000000000000 ) ) ;
#10674=CARTESIAN_POINT ( 'NONE',  ( -2.293366432827344421E-15, -12.48450537969573659, -63.40625000204837391 ) ) ;
#10675=ADVANCED_FACE ( 'NONE', ( #24928 ), #18422, .T. ) ;
#10678=CARTESIAN_POINT ( 'NONE',  ( -9.999999999998969713, -5.773502691896847949, -30.00000000409673717 ) ) ;
#10679=CARTESIAN_POINT ( 'NONE',  ( 10.81189881249999551, -6.242252689847874514, -174.1562500020484094 ) ) ;
#10683=CARTESIAN_POINT ( 'NONE',  ( 9.999999999999998224, 0.000000000000000000, -155.0000000000000000 ) ) ;
#10684=CARTESIAN_POINT ( 'NONE',  ( 10.00000000000038369, -5.773502691896038819, -153.6250000000000284 ) ) ;
#10685=VECTOR ( 'NONE', #10134, 1000.000000000000000 ) ;
#10687=CARTESIAN_POINT ( 'NONE',  ( 5.405949406249992428, -9.363379034771808662, -88.78125000204838102 ) ) ;
#10688=ORIENTED_EDGE ( 'NONE', *, *, #34402, .T. ) ;
#10690=ORIENTED_EDGE ( 'NONE', *, *, #15931, .T. ) ;
#10692=CARTESIAN_POINT ( 'NONE',  ( 10.81189881249999729, 0.000000000000000000, -25.34375000204835970 ) ) ;
#10694=CARTESIAN_POINT ( 'NONE',  ( 5.405949406249999534, 9.363379034771803333, -17.78125000204835970 ) ) ;
#10696=CARTESIAN_POINT ( 'NONE',  ( -5.405949406249996869, 9.363379034771805109, -74.34375000204838102 ) ) ;
#10697=CARTESIAN_POINT ( 'NONE',  ( 9.999999999999872102, 5.773502691896329253, -164.2500000040968189 ) ) ;
#10699=CARTESIAN_POINT ( 'NONE',  ( 10.81189881249999551, -6.242252689847874514, -187.4687500020484094 ) ) ;
#10701=CARTESIAN_POINT ( 'NONE',  ( 7.644554776091147741E-16, 12.48450537969573659, -2.468750002048359704 ) ) ;
#10705=CARTESIAN_POINT ( 'NONE',  ( -4.999999999999996447, 8.660254037844387298, -60.37500000409676204 ) ) ;
#10706=CARTESIAN_POINT ( 'NONE',  ( 10.81189881249999551, -6.242252689847874514, -109.4687500020483810 ) ) ;
#10707=CARTESIAN_POINT ( 'NONE',  ( 9.999999999999998224, 0.000000000000000000, -200.0000000000000000 ) ) ;
#10708=CARTESIAN_POINT ( 'NONE',  ( 7.644554776091147741E-16, 12.48450537969573659, -94.15625000204839523 ) ) ;
#10709=CARTESIAN_POINT ( 'NONE',  ( -10.81189881249999729, 6.242252689847871849, -96.71875000204836681 ) ) ;
#10710=( BOUNDED_CURVE ( )  B_SPLINE_CURVE ( 2, ( #34659, #11534, #27533, #37230, #24738, #24517, #27963 ),
 .UNSPECIFIED., .F., .F. ) 
 B_SPLINE_CURVE_WITH_KNOTS ( ( 3, 2, 2, 3 ),
 ( 0.6902985074626868389, 0.6915422885572141132, 0.6927860696517414985, 0.6940298507462688837 ),
 .UNSPECIFIED. ) 
 CURVE ( )  GEOMETRIC_REPRESENTATION_ITEM ( )  RATIONAL_B_SPLINE_CURVE ( ( 0.9999999999999761302, 0.8660254037844625774, 1.000000000000000000, 0.8660254037844387076, 1.000000000000000000, 0.8660254037844148378, 1.000000000000023981 ) ) 
 REPRESENTATION_ITEM ( '' )  );
#10712=AXIS2_PLACEMENT_3D ( 'NONE', #2030, #11929, #15794 ) ;
#10714=CARTESIAN_POINT ( 'NONE',  ( 9.999999999999996447, -5.773502691896262640, -166.0000000040967905 ) ) ;
#10715=VECTOR ( 'NONE', #23764, 1000.000000000000000 ) ;
#10718=ADVANCED_FACE ( 'NONE', ( #32249 ), #38714, .T. ) ;
#10723=CARTESIAN_POINT ( 'NONE',  ( -4.999999999999996447, 8.660254037844387298, -71.99999999999998579 ) ) ;
#10725=CARTESIAN_POINT ( 'NONE',  ( -5.000000000000003553, -8.660254037844383745, -92.87500000409677625 ) ) ;
#10726=VECTOR ( 'NONE', #5463, 1000.000000000000000 ) ;
#10727=CARTESIAN_POINT ( 'NONE',  ( -9.999999999999998224, 1.224646799147353059E-15, -168.1250000040967905 ) ) ;
#10729=CARTESIAN_POINT ( 'NONE',  ( 10.81189881249999551, -6.242252689847874514, -87.15625000204838102 ) ) ;
#10733=EDGE_LOOP ( 'NONE', ( #19249, #40144, #1869, #14383 ) ) ;
#10734=CARTESIAN_POINT ( 'NONE',  ( -9.999999999999998224, 1.224646799147353059E-15, -4.249999999999976019 ) ) ;
#10736=CARTESIAN_POINT ( 'NONE',  ( 10.81189881249999729, 0.000000000000000000, -14.84375000204835082 ) ) ;
#10737=CARTESIAN_POINT ( 'NONE',  ( -5.000000000000003553, -8.660254037844383745, -32.49999999999997158 ) ) ;
#10739=CARTESIAN_POINT ( 'NONE',  ( 10.81189881249999551, -6.242252689847874514, -139.6562500020484094 ) ) ;
#10740=ADVANCED_FACE ( 'NONE', ( #41933 ), #38494, .T. ) ;
#10741=CARTESIAN_POINT ( 'NONE',  ( -4.999999999999996447, 8.660254037844387298, -187.5000000000000000 ) ) ;
#10742=CARTESIAN_POINT ( 'NONE',  ( 6.760415694317262479E-15, -15.00000000000010303, 49.99999999999998579 ) ) ;
#10743=CARTESIAN_POINT ( 'NONE',  ( 5.405949406249992428, -9.363379034771808662, -108.2812500020483810 ) ) ;
#10744=VERTEX_POINT ( 'NONE', #8728 ) ;
#10745=CARTESIAN_POINT ( 'NONE',  ( -9.999999999999998224, 1.224646799147353059E-15, -75.12500000409677625 ) ) ;
#10746=EDGE_LOOP ( 'NONE', ( #10035, #31673, #39351, #18511 ) ) ;
#10747=ORIENTED_EDGE ( 'NONE', *, *, #19331, .T. ) ;
#10748=CARTESIAN_POINT ( 'NONE',  ( 10.81189881249999907, 6.242252689847868297, -44.90625000204836681 ) ) ;
#10750=CARTESIAN_POINT ( 'NONE',  ( -2.293366432827344421E-15, -12.48450537969573659, -99.21875000204839523 ) ) ;
#10752=CARTESIAN_POINT ( 'NONE',  ( -5.405949406249996869, 9.363379034771805109, -192.8437500020484094 ) ) ;
#10755=CARTESIAN_POINT ( 'NONE',  ( 0.000000000000000000, 0.000000000000000000, -200.0000000000000000 ) ) ;
#10756=CARTESIAN_POINT ( 'NONE',  ( 10.81189881249999551, -6.242252689847874514, -124.4687500020483952 ) ) ;
#10761=CARTESIAN_POINT ( 'NONE',  ( -2.121150477449813534E-15, -11.54700538379251284, -187.2500000040967905 ) ) ;
#10763=CARTESIAN_POINT ( 'NONE',  ( 5.405949406249992428, -9.363379034771808662, -177.2812500020484094 ) ) ;
#10764=EDGE_CURVE ( 'NONE', #11999, #33637, #7320, .T. ) ;
#10765=( BOUNDED_CURVE ( )  B_SPLINE_CURVE ( 2, ( #8898, #22063, #25523, #6087, #18818, #32002, #22275 ),
 .UNSPECIFIED., .F., .F. ) 
 B_SPLINE_CURVE_WITH_KNOTS ( ( 3, 2, 2, 3 ),
 ( 0.7947761194029852039, 0.7960199004975125892, 0.7972636815920399744, 0.7985074626865673597 ),
 .UNSPECIFIED. ) 
 CURVE ( )  GEOMETRIC_REPRESENTATION_ITEM ( )  RATIONAL_B_SPLINE_CURVE ( ( 0.9999999999999880096, 0.8660254037844506980, 1.000000000000000000, 0.8660254037844387076, 1.000000000000000000, 0.8660254037844148378, 1.000000000000023981 ) ) 
 REPRESENTATION_ITEM ( '' )  );
#10766=CARTESIAN_POINT ( 'NONE',  ( 5.000000000000000000, 8.660254037844385522, -180.2500000000000284 ) ) ;
#10767=CARTESIAN_POINT ( 'NONE',  ( -9.999999999999740652, 5.773502691896409189, -181.3749999999999716 ) ) ;
#10769=CARTESIAN_POINT ( 'NONE',  ( -5.405949406250003975, -9.363379034771801557, -54.34375000204835970 ) ) ;
#10770=CARTESIAN_POINT ( 'NONE',  ( -10.81189881249999729, 6.242252689847871849, -39.71875000204835970 ) ) ;
#10772=CARTESIAN_POINT ( 'NONE',  ( 10.81189881249999907, 6.242252689847868297, -11.90625000204835615 ) ) ;
#10776=CARTESIAN_POINT ( 'NONE',  ( 7.070501591499377789E-16, 11.54700538379251284, -94.62499999999997158 ) ) ;
#10778=CARTESIAN_POINT ( 'NONE',  ( -9.999999999998456346, -5.773502691897145489, -27.00000000409673717 ) ) ;
#10781=CARTESIAN_POINT ( 'NONE',  ( 10.81189881249999729, 6.242252689847867408, -104.9062500020483952 ) ) ;
#10782=ORIENTED_EDGE ( 'NONE', *, *, #35792, .T. ) ;
#10783=DIRECTION ( 'NONE',  ( -0.000000000000000000, -0.000000000000000000, 1.000000000000000000 ) ) ;
#10785=CARTESIAN_POINT ( 'NONE',  ( -4.999999999999996447, 8.660254037844387298, -91.49999999999998579 ) ) ;
#10789=CARTESIAN_POINT ( 'NONE',  ( -4.999999999999996447, 8.660254037844387298, -31.49999999999997158 ) ) ;
#10790=CARTESIAN_POINT ( 'NONE',  ( -5.405949406250003975, -9.363379034771801557, -33.53125000204837391 ) ) ;
#10791=EDGE_CURVE ( 'NONE', #14676, #4387, #29006, .T. ) ;
#10792=CARTESIAN_POINT ( 'NONE',  ( -4.999999999999996447, 8.660254037844387298, -111.3750000040967763 ) ) ;
#10795=CARTESIAN_POINT ( 'NONE',  ( -10.81189881249999907, -6.242252689847864744, -144.6562500020484094 ) ) ;
#10796=DIRECTION ( 'NONE',  ( 1.000000000000000000, 0.000000000000000000, 0.000000000000000000 ) ) ;
#10798=VERTEX_POINT ( 'NONE', #11729 ) ;
#10799=ORIENTED_EDGE ( 'NONE', *, *, #40243, .T. ) ;
#10801=CARTESIAN_POINT ( 'NONE',  ( -5.405949406249996869, 9.363379034771805109, -167.3437500020484094 ) ) ;
#10803=CARTESIAN_POINT ( 'NONE',  ( 7.644554776091147741E-16, 12.48450537969573659, -12.96875000204836148 ) ) ;
#10804=DIRECTION ( 'NONE',  ( -0.000000000000000000, -0.000000000000000000, 1.000000000000000000 ) ) ;
#10805=CARTESIAN_POINT ( 'NONE',  ( 7.644554776091147741E-16, 12.48450537969573659, -146.4687500020484094 ) ) ;
#10806=CARTESIAN_POINT ( 'NONE',  ( -10.81189881249999729, 1.324075727343319199E-15, -140.0937500020483810 ) ) ;
#10807=CARTESIAN_POINT ( 'NONE',  ( 10.81189881249999551, -6.242252689847874514, -105.1562500020483810 ) ) ;
#10811=CARTESIAN_POINT ( 'NONE',  ( 10.81189881249999729, 0.000000000000000000, -13.34375000204834905 ) ) ;
#10813=CARTESIAN_POINT ( 'NONE',  ( 5.000000000000000000, 8.660254037844385522, -63.62500000409676204 ) ) ;
#10817=CARTESIAN_POINT ( 'NONE',  ( 10.81189881249999729, 0.000000000000000000, -79.34375000204838102 ) ) ;
#10818=CARTESIAN_POINT ( 'NONE',  ( -5.405949406249996869, 9.363379034771805109, -63.84375000204836681 ) ) ;
#10820=CARTESIAN_POINT ( 'NONE',  ( -5.405949406250003975, -9.363379034771801557, -30.53125000204837036 ) ) ;
#10822=CARTESIAN_POINT ( 'NONE',  ( 9.999999999999998224, 0.000000000000000000, -9.499999999999953815 ) ) ;
#10824=CARTESIAN_POINT ( 'NONE',  ( 9.999999999999996447, -5.773502691896262640, -128.1249999999999716 ) ) ;
#10825=CARTESIAN_POINT ( 'NONE',  ( 5.405949406249999534, 9.363379034771803333, -133.2812500020483810 ) ) ;
#10826=CARTESIAN_POINT ( 'NONE',  ( -9.999999999999776179, -5.773502691896382544, -187.5000000040967905 ) ) ;
#10828=CARTESIAN_POINT ( 'NONE',  ( -2.293366432827344421E-15, -12.48450537969573659, -16.90625000204838102 ) ) ;
#10829=VERTEX_POINT ( 'NONE', #15390 ) ;
#10832=CARTESIAN_POINT ( 'NONE',  ( -9.999999999999998224, 1.224646799147353059E-15, -38.74999999999997868 ) ) ;
#10833=CARTESIAN_POINT ( 'NONE',  ( -9.999999999999998224, 5.773502691896259087, -36.25000000409675494 ) ) ;
#10834=( BOUNDED_CURVE ( )  B_SPLINE_CURVE ( 2, ( #24598, #2149, #37747, #18097, #28260, #31073, #41398 ),
 .UNSPECIFIED., .F., .F. ) 
 B_SPLINE_CURVE_WITH_KNOTS ( ( 3, 2, 2, 3 ),
 ( 0.9813432835820897759, 0.9825870646766171612, 0.9838308457711445465, 0.9850746268656718208 ),
 .UNSPECIFIED. ) 
 CURVE ( )  GEOMETRIC_REPRESENTATION_ITEM ( )  RATIONAL_B_SPLINE_CURVE ( ( 0.9999999999999761302, 0.8660254037844625774, 1.000000000000000000, 0.8660254037844387076, 1.000000000000000000, 0.8660254037844148378, 1.000000000000023981 ) ) 
 REPRESENTATION_ITEM ( '' )  );
#10835=CARTESIAN_POINT ( 'NONE',  ( 0.000000000000000000, 0.000000000000000000, -200.0000000000000000 ) ) ;
#10838=CARTESIAN_POINT ( 'NONE',  ( -5.405949406250003975, -9.363379034771801557, -150.5312500020483810 ) ) ;
#10839=CARTESIAN_POINT ( 'NONE',  ( 7.644554776091147741E-16, 12.48450537969573659, -138.9687500020484094 ) ) ;
#10840=LINE ( 'NONE', #31369, #39250 ) ;
#10841=EDGE_CURVE ( 'NONE', #5330, #848, #16112, .T. ) ;
#10842=VERTEX_POINT ( 'NONE', #29215 ) ;
#10843=ADVANCED_FACE ( 'NONE', ( #36740 ), #33091, .T. ) ;
#10845=ORIENTED_EDGE ( 'NONE', *, *, #11941, .F. ) ;
#10846=EDGE_LOOP ( 'NONE', ( #11332, #5663, #16276, #15558 ) ) ;
#10849=CARTESIAN_POINT ( 'NONE',  ( 5.405949406249992428, -9.363379034771808662, -109.5937500020483810 ) ) ;
#10850=ORIENTED_EDGE ( 'NONE', *, *, #28324, .F. ) ;
#10852=CARTESIAN_POINT ( 'NONE',  ( -10.81189881249999729, 1.324075727343319199E-15, -192.5937500020484094 ) ) ;
#10853=CARTESIAN_POINT ( 'NONE',  ( -2.293366432827344421E-15, -12.48450537969573659, -39.21875000204835970 ) ) ;
#10854=CARTESIAN_POINT ( 'NONE',  ( -4.519005929163725455, -9.200975322961610914, 1.142019215729700943E-14 ) ) ;
#10855=CARTESIAN_POINT ( 'NONE',  ( 7.070501591499376803E-16, 11.54700538379251284, -0.1249999999999685391 ) ) ;
#10856=CARTESIAN_POINT ( 'NONE',  ( 10.81189881249999729, 0.000000000000000000, -172.3437500020484094 ) ) ;
#10857=CARTESIAN_POINT ( 'NONE',  ( -5.405949406249996869, 9.363379034771805109, -161.3437500020484094 ) ) ;
#10858=LINE ( 'NONE', #41276, #9373 ) ;
#10861=CARTESIAN_POINT ( 'NONE',  ( -2.121150477449813534E-15, -11.54700538379251284, -93.87500000000000000 ) ) ;
#10862=CARTESIAN_POINT ( 'NONE',  ( 5.000000000000000000, 8.660254037844385522, -66.62500000409676204 ) ) ;
#10864=CARTESIAN_POINT ( 'NONE',  ( 5.405949406249992428, -9.363379034771808662, -87.09375000204836681 ) ) ;
#10865=DIRECTION ( 'NONE',  ( -0.000000000000000000, -0.000000000000000000, 1.000000000000000000 ) ) ;
#10866=CARTESIAN_POINT ( 'NONE',  ( -10.81189881249999907, -6.242252689847864744, -63.65625000204836681 ) ) ;
#10869=CARTESIAN_POINT ( 'NONE',  ( -10.81189881249999729, 1.324075727343319199E-15, -120.7812500020483952 ) ) ;
#10870=CARTESIAN_POINT ( 'NONE',  ( -10.81189881249999729, 1.324075727343319199E-15, -153.7812500020484094 ) ) ;
#10872=CARTESIAN_POINT ( 'NONE',  ( 7.070501591499377789E-16, 11.54700538379251284, -132.5000000040967620 ) ) ;
#10874=( BOUNDED_CURVE ( )  B_SPLINE_CURVE ( 2, ( #5016, #11252, #18377, #34586, #22052, #2418, #41460 ),
 .UNSPECIFIED., .F., .F. ) 
 B_SPLINE_CURVE_WITH_KNOTS ( ( 3, 2, 2, 3 ),
 ( 0.7238805970149256863, 0.7251243781094530716, 0.7263681592039803459, 0.7276119402985077311 ),
 .UNSPECIFIED. ) 
 CURVE ( )  GEOMETRIC_REPRESENTATION_ITEM ( )  RATIONAL_B_SPLINE_CURVE ( ( 0.9999999999999641398, 0.8660254037844745678, 1.000000000000000000, 0.8660254037844387076, 1.000000000000000000, 0.8660254037844148378, 1.000000000000023981 ) ) 
 REPRESENTATION_ITEM ( '' )  );
#10875=ORIENTED_EDGE ( 'NONE', *, *, #1993, .T. ) ;
#10879=CARTESIAN_POINT ( 'NONE',  ( -10.81189881249999729, 1.324075727343319199E-15, -185.2812500020484094 ) ) ;
#10880=AXIS2_PLACEMENT_3D ( 'NONE', #40215, #17334, #23841 ) ;
#10882=CARTESIAN_POINT ( 'NONE',  ( 5.000000000000000000, 8.660254037844385522, -46.74999999999998579 ) ) ;
#10884=CARTESIAN_POINT ( 'NONE',  ( 9.999999999999996447, -5.773502691896262640, -61.00000000409677625 ) ) ;
#10887=CARTESIAN_POINT ( 'NONE',  ( 9.999999999999998224, 0.000000000000000000, -119.3750000040967905 ) ) ;
#10889=CARTESIAN_POINT ( 'NONE',  ( -5.405949406250003975, -9.363379034771801557, -62.03125000204837391 ) ) ;
#10892=CARTESIAN_POINT ( 'NONE',  ( 5.000000000000000000, 8.660254037844385522, -88.74999999999998579 ) ) ;
#10893=CARTESIAN_POINT ( 'NONE',  ( -10.81189881249999907, -6.242252689847864744, -177.6562500020484094 ) ) ;
#10895=CARTESIAN_POINT ( 'NONE',  ( 10.00000000000102318, -5.773502691895667560, -87.62499999999995737 ) ) ;
#10897=EDGE_CURVE ( 'NONE', #12865, #12739, #29637, .T. ) ;
#10898=CARTESIAN_POINT ( 'NONE',  ( 9.999999999999742428, 5.773502691896404748, -117.3749999999999716 ) ) ;
#10899=CARTESIAN_POINT ( 'NONE',  ( 9.999999999999548805, 5.773502691896514882, -177.3749999999999716 ) ) ;
#10901=DIRECTION ( 'NONE',  ( -1.000000000000000000, -1.502314598737160017E-16, 0.000000000000000000 ) ) ;
#10903=CARTESIAN_POINT ( 'NONE',  ( 10.81189881249999551, -6.242252689847874514, -84.15625000204838102 ) ) ;
#10906=ORIENTED_EDGE ( 'NONE', *, *, #3109, .F. ) ;
#10909=CARTESIAN_POINT ( 'NONE',  ( -5.405949406249996869, 9.363379034771805109, -33.84375000204836681 ) ) ;
#10910=CARTESIAN_POINT ( 'NONE',  ( -5.405949406249996869, 9.363379034771805109, -29.34375000204836326 ) ) ;
#10911=CARTESIAN_POINT ( 'NONE',  ( -10.81189881249999729, 1.324075727343319199E-15, -14.28125000204835615 ) ) ;
#10912=CARTESIAN_POINT ( 'NONE',  ( 10.81189881249999907, 6.242252689847868297, -67.21875000204838102 ) ) ;
#10915=CARTESIAN_POINT ( 'NONE',  ( -10.81189881249999729, 1.324075727343319199E-15, -186.5937500020483810 ) ) ;
#10917=CARTESIAN_POINT ( 'NONE',  ( -9.999999999998456346, -5.773502691897145489, -26.62499999999994316 ) ) ;
#10920=EDGE_CURVE ( 'NONE', #41097, #39297, #13204, .T. ) ;
#10921=DIRECTION ( 'NONE',  ( -1.000000000000000000, 0.000000000000000000, -0.000000000000000000 ) ) ;
#10922=CARTESIAN_POINT ( 'NONE',  ( -10.81189881249999907, -6.242252689847864744, -112.9687500020483810 ) ) ;
#10923=CARTESIAN_POINT ( 'NONE',  ( 9.999999999999998224, 0.000000000000000000, -18.49999999999996092 ) ) ;
#10924=CARTESIAN_POINT ( 'NONE',  ( -5.405949406249996869, 9.363379034771805109, -92.53125000204838102 ) ) ;
#10925=CARTESIAN_POINT ( 'NONE',  ( -5.405949406250003975, -9.363379034771801557, -99.34375000204838102 ) ) ;
#10928=CARTESIAN_POINT ( 'NONE',  ( 5.000000000000000000, 8.660254037844385522, -155.1250000040967905 ) ) ;
#10933=CARTESIAN_POINT ( 'NONE',  ( -9.999999999999998224, 1.224646799147353059E-15, -101.7500000000000000 ) ) ;
#10935=CARTESIAN_POINT ( 'NONE',  ( -9.999999999999998224, 1.224646799147353059E-15, -62.74999999999997158 ) ) ;
#10936=CARTESIAN_POINT ( 'NONE',  ( -10.00000000000000000, -5.773502691896251982, -71.62500000000000000 ) ) ;
#10938=CARTESIAN_POINT ( 'NONE',  ( -5.000000000000003553, -8.660254037844383745, -82.37500000409676204 ) ) ;
#10939=CARTESIAN_POINT ( 'NONE',  ( -2.121150477449813534E-15, -11.54700538379251284, -171.8750000000000284 ) ) ;
#10941=CARTESIAN_POINT ( 'NONE',  ( 10.81189881249999551, -6.242252689847874514, -84.15625000204838102 ) ) ;
#10943=CARTESIAN_POINT ( 'NONE',  ( 7.070501591499376803E-16, 11.54700538379251284, -168.1250000000000000 ) ) ;
#10945=ORIENTED_EDGE ( 'NONE', *, *, #40984, .F. ) ;
#10946=CARTESIAN_POINT ( 'NONE',  ( 7.070501591499377789E-16, 11.54700538379251284, -1.624999999999975575 ) ) ;
#10948=CARTESIAN_POINT ( 'NONE',  ( -2.293366432827344421E-15, -12.48450537969573659, -13.71875000204836503 ) ) ;
#10950=AXIS2_PLACEMENT_3D ( 'NONE', #4577, #40380, #925 ) ;
#10952=CARTESIAN_POINT ( 'NONE',  ( 10.81189881249999729, 0.000000000000000000, -132.0312500020484094 ) ) ;
#10953=CARTESIAN_POINT ( 'NONE',  ( 9.999999999999998224, 0.000000000000000000, -180.5000000000000000 ) ) ;
#10954=DIRECTION ( 'NONE',  ( 1.000000000000000000, 0.000000000000000000, 0.000000000000000000 ) ) ;
#10955=CARTESIAN_POINT ( 'NONE',  ( -10.81189881249999907, -6.242252689847864744, -111.6562500020483952 ) ) ;
#10956=ORIENTED_EDGE ( 'NONE', *, *, #39430, .F. ) ;
#10957=ORIENTED_EDGE ( 'NONE', *, *, #36194, .T. ) ;
#10959=CARTESIAN_POINT ( 'NONE',  ( 10.81189881249999729, 0.000000000000000000, -39.03125000204838102 ) ) ;
#10962=CARTESIAN_POINT ( 'NONE',  ( -10.81189881249999907, -6.242252689847864744, -87.46875000204838102 ) ) ;
#10965=CARTESIAN_POINT ( 'NONE',  ( -10.81189881249999729, -6.242252689847864744, -193.9687500020484094 ) ) ;
#10967=CARTESIAN_POINT ( 'NONE',  ( 9.999999999998969713, 5.773502691896851502, -58.87499999999997158 ) ) ;
#10968=CARTESIAN_POINT ( 'NONE',  ( 5.405949406249992428, -9.363379034771808662, -126.0937500020483668 ) ) ;
#10970=CARTESIAN_POINT ( 'NONE',  ( 5.405949406249992428, -9.363379034771808662, -4.781250002048375691 ) ) ;
#10973=CARTESIAN_POINT ( 'NONE',  ( -10.00000000000000000, -5.773502691896251982, -177.0000000040967620 ) ) ;
#10975=CARTESIAN_POINT ( 'NONE',  ( -2.293366432827344421E-15, -12.48450537969573659, -181.9062500020483810 ) ) ;
#10979=CARTESIAN_POINT ( 'NONE',  ( -2.293366432827344421E-15, -12.48450537969573659, -52.71875000204836681 ) ) ;
#10980=VECTOR ( 'NONE', #7737, 1000.000000000000000 ) ;
#10981=CARTESIAN_POINT ( 'NONE',  ( -2.293366432827344421E-15, -12.48450537969573659, -43.71875000204835970 ) ) ;
#10983=CARTESIAN_POINT ( 'NONE',  ( -5.405949406249996869, 9.363379034771805109, -7.031250002048378356 ) ) ;
#10985=CARTESIAN_POINT ( 'NONE',  ( 10.00000000000025402, -5.773502691896113426, -124.0000000040967620 ) ) ;
#10987=CARTESIAN_POINT ( 'NONE',  ( -9.999999999999998224, 5.773502691896259087, -100.3750000000000000 ) ) ;
#10989=CARTESIAN_POINT ( 'NONE',  ( -2.121150477449813534E-15, -11.54700538379251284, -110.7500000040967763 ) ) ;
#10990=CARTESIAN_POINT ( 'NONE',  ( -10.00000000000000000, -5.773502691896252870, -169.1249999999999716 ) ) ;
#10993=CARTESIAN_POINT ( 'NONE',  ( 5.405949406249992428, -9.363379034771808662, -103.7812500020483810 ) ) ;
#10995=AXIS2_PLACEMENT_3D ( 'NONE', #22315, #41718, #15810 ) ;
#10996=CARTESIAN_POINT ( 'NONE',  ( -9.999999999999998224, 1.224646799147353059E-15, -68.74999999999997158 ) ) ;
#10999=CARTESIAN_POINT ( 'NONE',  ( 5.405949406249999534, 9.363379034771803333, -164.7812500020484094 ) ) ;
#11001=ORIENTED_EDGE ( 'NONE', *, *, #39889, .T. ) ;
#11002=CARTESIAN_POINT ( 'NONE',  ( -9.999999999999998224, 1.224646799147353059E-15, -26.74999999999996803 ) ) ;
#11003=CARTESIAN_POINT ( 'NONE',  ( 5.405949406249992428, -9.363379034771808662, -39.28125000204838102 ) ) ;
#11004=CARTESIAN_POINT ( 'NONE',  ( 5.000000000000000000, 8.660254037844385522, -163.7500000000000000 ) ) ;
#11007=( BOUNDED_CURVE ( )  B_SPLINE_CURVE ( 2, ( #15470, #21962, #15262, #28671, #32540, #5353, #38156 ),
 .UNSPECIFIED., .F., .F. ) 
 B_SPLINE_CURVE_WITH_KNOTS ( ( 3, 2, 2, 3 ),
 ( 0.1828358208955224162, 0.1840796019900497738, 0.1853233830845771313, 0.1865671641791045166 ),
 .UNSPECIFIED. ) 
 CURVE ( )  GEOMETRIC_REPRESENTATION_ITEM ( )  RATIONAL_B_SPLINE_CURVE ( ( 0.9999999999999970024, 0.8660254037844417052, 1.000000000000000000, 0.8660254037844387076, 1.000000000000000000, 0.8660254037844357100, 1.000000000000002887 ) ) 
 REPRESENTATION_ITEM ( '' )  );
#11008=CARTESIAN_POINT ( 'NONE',  ( 7.644554776091147741E-16, 12.48450537969573659, -131.6562500020483810 ) ) ;
#11009=CARTESIAN_POINT ( 'NONE',  ( -9.999999999999998224, 1.224646799147353059E-15, -75.12500000409677625 ) ) ;
#11010=EDGE_LOOP ( 'NONE', ( #25015, #6558, #20255, #41155 ) ) ;
#11011=( BOUNDED_CURVE ( )  B_SPLINE_CURVE ( 2, ( #19438, #23548, #16395, #6711, #680, #14002, #20290 ),
 .UNSPECIFIED., .F., .F. ) 
 B_SPLINE_CURVE_WITH_KNOTS ( ( 3, 2, 2, 3 ),
 ( 0.1940298507462686894, 0.1952736318407960470, 0.1965174129353234322, 0.1977611940298507898 ),
 .UNSPECIFIED. ) 
 CURVE ( )  GEOMETRIC_REPRESENTATION_ITEM ( )  RATIONAL_B_SPLINE_CURVE ( ( 0.9999999999999970024, 0.8660254037844417052, 1.000000000000000000, 0.8660254037844387076, 1.000000000000000000, 0.8660254037844327124, 1.000000000000005995 ) ) 
 REPRESENTATION_ITEM ( '' )  );
#11012=ORIENTED_EDGE ( 'NONE', *, *, #27480, .T. ) ;
#11014=CARTESIAN_POINT ( 'NONE',  ( 5.000000000000000000, 8.660254037844385522, -182.1250000040967905 ) ) ;
#11015=CARTESIAN_POINT ( 'NONE',  ( -5.000000000000003553, -8.660254037844383745, -134.5000000000000000 ) ) ;
#11016=CARTESIAN_POINT ( 'NONE',  ( 7.644554776091147741E-16, 12.48450537969573659, -162.9687500020483810 ) ) ;
#11017=( BOUNDED_CURVE ( )  B_SPLINE_CURVE ( 2, ( #32857, #36505, #6728, #39312, #3286, #33497, #33067 ),
 .UNSPECIFIED., .F., .F. ) 
 B_SPLINE_CURVE_WITH_KNOTS ( ( 3, 2, 2, 3 ),
 ( 0.3470149253731344974, 0.3482587064676618271, 0.3495024875621891569, 0.3507462686567164867 ),
 .UNSPECIFIED. ) 
 CURVE ( )  GEOMETRIC_REPRESENTATION_ITEM ( )  RATIONAL_B_SPLINE_CURVE ( ( 0.9999999999999820144, 0.8660254037844566932, 1.000000000000000000, 0.8660254037844387076, 1.000000000000000000, 0.8660254037844327124, 1.000000000000005995 ) ) 
 REPRESENTATION_ITEM ( '' )  );
#11019=CARTESIAN_POINT ( 'NONE',  ( -10.81189881249999729, 6.242252689847871849, -17.21875000204836681 ) ) ;
#11020=CARTESIAN_POINT ( 'NONE',  ( -10.81189881249999729, -6.242252689847864744, -145.9687500020484094 ) ) ;
#11021=CARTESIAN_POINT ( 'NONE',  ( 10.81189881249999551, -6.242252689847874514, -140.9687500020483810 ) ) ;
#11022=CARTESIAN_POINT ( 'NONE',  ( 7.644554776091147741E-16, 12.48450537969573659, -106.1562500020483952 ) ) ;
#11026=CARTESIAN_POINT ( 'NONE',  ( -5.405949406249996869, 9.363379034771805109, -11.34375000204834727 ) ) ;
#11028=EDGE_CURVE ( 'NONE', #10480, #21964, #26397, .T. ) ;
#11029=CARTESIAN_POINT ( 'NONE',  ( -10.81189881249999729, -6.242252689847864744, -198.6562500020484094 ) ) ;
#11030=CARTESIAN_POINT ( 'NONE',  ( 4.999999999999992006, -8.660254037844389075, -196.1250000040967905 ) ) ;
#11033=CARTESIAN_POINT ( 'NONE',  ( -10.81189881249999729, -6.242252689847864744, -79.96875000204838102 ) ) ;
#11034=CARTESIAN_POINT ( 'NONE',  ( 10.81189881249999907, 6.242252689847868297, -61.21875000204838102 ) ) ;
#11036=CARTESIAN_POINT ( 'NONE',  ( 10.81189881249999551, -6.242252689847874514, -37.65625000204836681 ) ) ;
#11038=CARTESIAN_POINT ( 'NONE',  ( -4.999999999999996447, 8.660254037844387298, -186.0000000000000000 ) ) ;
#11040=CARTESIAN_POINT ( 'NONE',  ( -5.000000000000003553, -8.660254037844383745, -121.0000000000000000 ) ) ;
#11041=CARTESIAN_POINT ( 'NONE',  ( -10.81189881249999729, 1.324075727343319199E-15, -128.2812500020483810 ) ) ;
#11042=CARTESIAN_POINT ( 'NONE',  ( 9.999999999999998224, 0.000000000000000000, -186.8750000040967905 ) ) ;
#11044=CARTESIAN_POINT ( 'NONE',  ( 10.81189881249999729, 0.000000000000000000, -15.03125000204835793 ) ) ;
#11048=CARTESIAN_POINT ( 'NONE',  ( -4.999999999999996447, 8.660254037844387298, -8.999999999999952038 ) ) ;
#11049=CARTESIAN_POINT ( 'NONE',  ( 5.000000000000000000, 8.660254037844385522, -33.62500000409676915 ) ) ;
#11050=CARTESIAN_POINT ( 'NONE',  ( -10.00000000000051337, 5.773502691895962435, -74.87499999999997158 ) ) ;
#11052=CARTESIAN_POINT ( 'NONE',  ( 10.81189881249999551, -6.242252689847874514, -151.6562500020484094 ) ) ;
#11053=EDGE_CURVE ( 'NONE', #26894, #39570, #13628, .T. ) ;
#11054=CARTESIAN_POINT ( 'NONE',  ( -5.405949406249996869, 9.363379034771805109, -126.8437500020483952 ) ) ;
#11055=ORIENTED_EDGE ( 'NONE', *, *, #13238, .F. ) ;
#11056=CARTESIAN_POINT ( 'NONE',  ( 0.000000000000000000, 0.000000000000000000, -200.0000000000000000 ) ) ;
#11057=ORIENTED_EDGE ( 'NONE', *, *, #26285, .T. ) ;
#11059=CARTESIAN_POINT ( 'NONE',  ( -5.405949406249996869, 9.363379034771805109, -113.3437500020483810 ) ) ;
#11061=CARTESIAN_POINT ( 'NONE',  ( -5.000000000000003553, -8.660254037844383745, -41.87500000409677625 ) ) ;
#11062=CARTESIAN_POINT ( 'NONE',  ( -5.405949406250003975, -9.363379034771801557, -186.3437500020483810 ) ) ;
#11064=CARTESIAN_POINT ( 'NONE',  ( 5.405949406249999534, 9.363379034771803333, -41.59375000204837391 ) ) ;
#11066=CARTESIAN_POINT ( 'NONE',  ( 9.999999999999612754, 5.773502691896477579, -152.2500000040967336 ) ) ;
#11067=CARTESIAN_POINT ( 'NONE',  ( 10.81189881249999551, -6.242252689847874514, -173.9687500020483810 ) ) ;
#11068=CARTESIAN_POINT ( 'NONE',  ( 5.405949406249999534, 9.363379034771803333, -163.0937500020484094 ) ) ;
#11069=CARTESIAN_POINT ( 'NONE',  ( -2.121150477449813534E-15, -11.54700538379251284, -76.25000000409676204 ) ) ;
#11074=CARTESIAN_POINT ( 'NONE',  ( -10.81189881249999907, -6.242252689847864744, -88.96875000204836681 ) ) ;
#11075=DIRECTION ( 'NONE',  ( -0.000000000000000000, -0.000000000000000000, 1.000000000000000000 ) ) ;
#11076=CARTESIAN_POINT ( 'NONE',  ( 10.81189881249999907, 6.242252689847868297, -58.40625000204838102 ) ) ;
#11077=CARTESIAN_POINT ( 'NONE',  ( -9.999999999999479527, -5.773502691896549521, -97.50000000409676204 ) ) ;
#11080=CARTESIAN_POINT ( 'NONE',  ( 10.81189881249999907, 6.242252689847868297, -118.4062500020484094 ) ) ;
#11081=CARTESIAN_POINT ( 'NONE',  ( -5.405949406250003975, -9.363379034771801557, -150.5312500020483810 ) ) ;
#11082=( BOUNDED_CURVE ( )  B_SPLINE_CURVE ( 2, ( #40169, #23787, #20531, #4143, #30490, #918, #4360 ),
 .UNSPECIFIED., .F., .F. ) 
 B_SPLINE_CURVE_WITH_KNOTS ( ( 3, 2, 2, 3 ),
 ( 0.5111940298507463565, 0.5124378109452737418, 0.5136815920398011270, 0.5149253731343285123 ),
 .UNSPECIFIED. ) 
 CURVE ( )  GEOMETRIC_REPRESENTATION_ITEM ( )  RATIONAL_B_SPLINE_CURVE ( ( 0.9999999999999880096, 0.8660254037844506980, 1.000000000000000000, 0.8660254037844387076, 1.000000000000000000, 0.8660254037844267172, 1.000000000000011990 ) ) 
 REPRESENTATION_ITEM ( '' )  );
#11085=CARTESIAN_POINT ( 'NONE',  ( -9.999999999999998224, 1.224646799147353059E-15, -130.6250000040967620 ) ) ;
#11090=CARTESIAN_POINT ( 'NONE',  ( 10.81189881249999551, -6.242252689847874514, -187.6562500020484379 ) ) ;
#11091=ORIENTED_EDGE ( 'NONE', *, *, #1313, .T. ) ;
#11092=CARTESIAN_POINT ( 'NONE',  ( -5.000000000000003553, -8.660254037844383745, -53.49999999999996447 ) ) ;
#11094=CARTESIAN_POINT ( 'NONE',  ( 7.070501591499377789E-16, 11.54700538379251284, -59.00000000409676915 ) ) ;
#11098=CARTESIAN_POINT ( 'NONE',  ( -10.81189881249999729, 6.242252689847871849, -54.90625000204836681 ) ) ;
#11101=CARTESIAN_POINT ( 'NONE',  ( -9.999999999999998224, 1.224646799147353059E-15, -135.1250000040967620 ) ) ;
#11102=CARTESIAN_POINT ( 'NONE',  ( -10.81189881249999729, 1.324075727343319199E-15, -176.2812500020484094 ) ) ;
#11107=CARTESIAN_POINT ( 'NONE',  ( 7.070501591499376803E-16, 11.54700538379251284, -177.1250000000000000 ) ) ;
#11108=LINE ( 'NONE', #24091, #6895 ) ;
#11109=VECTOR ( 'NONE', #1761, 1000.000000000000000 ) ;
#11110=CARTESIAN_POINT ( 'NONE',  ( 10.81189881249999729, 0.000000000000000000, -88.53125000204838102 ) ) ;
#11111=ORIENTED_EDGE ( 'NONE', *, *, #2221, .T. ) ;
#11112=DIRECTION ( 'NONE',  ( 0.000000000000000000, 0.000000000000000000, 1.000000000000000000 ) ) ;
#11114=ORIENTED_EDGE ( 'NONE', *, *, #33743, .T. ) ;
#11116=CARTESIAN_POINT ( 'NONE',  ( 10.81189881249999729, 6.242252689847867408, -40.21875000204835970 ) ) ;
#11117=CARTESIAN_POINT ( 'NONE',  ( -10.81189881249999729, 1.324075727343319199E-15, -24.59375000204835970 ) ) ;
#11118=CARTESIAN_POINT ( 'NONE',  ( -10.81189881249999729, 1.324075727343319199E-15, -12.78125000204835615 ) ) ;
#11119=CARTESIAN_POINT ( 'NONE',  ( 5.405949406249999534, 9.363379034771803333, -61.09375000204836681 ) ) ;
#11122=CARTESIAN_POINT ( 'NONE',  ( 10.81189881249999907, 6.242252689847868297, -181.2187500020484094 ) ) ;
#11124=AXIS2_PLACEMENT_3D ( 'NONE', #14446, #27638, #21367 ) ;
#11127=CYLINDRICAL_SURFACE ( 'NONE', #14284, 9.999999999999998224 ) ;
#11128=FACE_OUTER_BOUND ( 'NONE', #34239, .T. ) ;
#11129=CARTESIAN_POINT ( 'NONE',  ( -9.999999999999998224, 1.224646799147353059E-15, -140.7500000000000000 ) ) ;
#11130=LINE ( 'NONE', #37691, #10173 ) ;
#11132=CARTESIAN_POINT ( 'NONE',  ( -10.81189881249999729, 1.324075727343319199E-15, -116.0937500020483810 ) ) ;
#11134=CARTESIAN_POINT ( 'NONE',  ( 10.81189881249999907, 6.242252689847868297, -82.40625000204836681 ) ) ;
#11136=CARTESIAN_POINT ( 'NONE',  ( -5.405949406250003975, -9.363379034771801557, -103.8437500020483810 ) ) ;
#11138=ADVANCED_FACE ( 'NONE', ( #19906 ), #39548, .T. ) ;
#11140=CARTESIAN_POINT ( 'NONE',  ( 9.999999999999996447, -5.773502691896262640, -151.0000000040967905 ) ) ;
#11142=EDGE_CURVE ( 'NONE', #8957, #25614, #28004, .T. ) ;
#11145=VECTOR ( 'NONE', #6142, 1000.000000000000000 ) ;
#11148=CARTESIAN_POINT ( 'NONE',  ( -4.999999999999996447, 8.660254037844387298, -120.3750000040967905 ) ) ;
#11149=CARTESIAN_POINT ( 'NONE',  ( -2.121150477449813534E-15, -11.54700538379251284, -71.37499999999997158 ) ) ;
#11151=CARTESIAN_POINT ( 'NONE',  ( 5.000000000000000000, 8.660254037844385522, -84.62500000409677625 ) ) ;
#11154=CARTESIAN_POINT ( 'NONE',  ( -2.293366432827344421E-15, -12.48450537969573659, -73.90625000204836681 ) ) ;
#11156=CARTESIAN_POINT ( 'NONE',  ( 9.999999999999998224, 0.000000000000000000, -97.99999999999998579 ) ) ;
#11158=ORIENTED_EDGE ( 'NONE', *, *, #19624, .T. ) ;
#11159=CARTESIAN_POINT ( 'NONE',  ( -10.81189881249999907, -6.242252689847864744, -198.6562500020484094 ) ) ;
#11161=CARTESIAN_POINT ( 'NONE',  ( 10.81189881249999551, -6.242252689847874514, -16.46875000204836326 ) ) ;
#11165=CARTESIAN_POINT ( 'NONE',  ( 5.405949406249992428, -9.363379034771808662, -127.7812500020483810 ) ) ;
#11167=EDGE_CURVE ( 'NONE', #38243, #36297, #4294, .T. ) ;
#11168=CARTESIAN_POINT ( 'NONE',  ( 9.999999999999996447, -5.773502691896262640, -185.1250000000000284 ) ) ;
#11169=CARTESIAN_POINT ( 'NONE',  ( -10.00000000000051337, 5.773502691895962435, -106.3749999999999716 ) ) ;
#11170=CARTESIAN_POINT ( 'NONE',  ( -5.405949406250003975, -9.363379034771801557, -111.5312500020483810 ) ) ;
#11171=ORIENTED_EDGE ( 'NONE', *, *, #34958, .F. ) ;
#11173=EDGE_CURVE ( 'NONE', #41888, #12272, #11713, .T. ) ;
#11175=ORIENTED_EDGE ( 'NONE', *, *, #42683, .F. ) ;
#11176=CARTESIAN_POINT ( 'NONE',  ( 5.405949406249999534, 9.363379034771803333, -38.78125000204838102 ) ) ;
#11179=CARTESIAN_POINT ( 'NONE',  ( 7.644554776091147741E-16, 12.48450537969573659, -87.96875000204838102 ) ) ;
#11180=FACE_OUTER_BOUND ( 'NONE', #15179, .T. ) ;
#11185=DIRECTION ( 'NONE',  ( 1.000000000000000000, 0.000000000000000000, 0.000000000000000000 ) ) ;
#11186=CARTESIAN_POINT ( 'NONE',  ( 5.405949406249992428, -9.363379034771808662, -121.5937500020483952 ) ) ;
#11188=CARTESIAN_POINT ( 'NONE',  ( 10.81189881249999729, 6.242252689847867408, -2.906250002048345493 ) ) ;
#11191=CARTESIAN_POINT ( 'NONE',  ( 7.070501591499377789E-16, 11.54700538379251284, -174.5000000040967905 ) ) ;
#11193=CARTESIAN_POINT ( 'NONE',  ( 5.405949406249999534, 9.363379034771803333, -181.2812500020483810 ) ) ;
#11194=ADVANCED_FACE ( 'NONE', ( #37387 ), #1573, .F. ) ;
#11195=DIRECTION ( 'NONE',  ( -0.000000000000000000, -0.000000000000000000, 1.000000000000000000 ) ) ;
#11197=CARTESIAN_POINT ( 'NONE',  ( -10.81189881249999729, 6.242252689847871849, -51.71875000204836681 ) ) ;
#11199=CARTESIAN_POINT ( 'NONE',  ( -10.81189881249999729, 6.242252689847871849, -6.906250002048365033 ) ) ;
#11201=CARTESIAN_POINT ( 'NONE',  ( -5.000000000000003553, -8.660254037844383745, -193.3750000040967905 ) ) ;
#11203=CARTESIAN_POINT ( 'NONE',  ( -10.00000000000000000, -5.773502691896251982, -97.12500000000000000 ) ) ;
#11205=CARTESIAN_POINT ( 'NONE',  ( 7.070501591499377789E-16, 11.54700538379251284, -107.0000000040967763 ) ) ;
#11209=CARTESIAN_POINT ( 'NONE',  ( 5.405949406249999534, 9.363379034771803333, -110.7812500020483810 ) ) ;
#11210=ORIENTED_EDGE ( 'NONE', *, *, #25689, .T. ) ;
#11212=CARTESIAN_POINT ( 'NONE',  ( 10.81189881249999907, 6.242252689847868297, -164.9062500020484094 ) ) ;
#11214=ORIENTED_EDGE ( 'NONE', *, *, #36754, .F. ) ;
#11215=CARTESIAN_POINT ( 'NONE',  ( -2.121150477449813534E-15, -11.54700538379251284, -29.37499999999994671 ) ) ;
#11216=AXIS2_PLACEMENT_3D ( 'NONE', #6458, #13326, #20448 ) ;
#11217=CARTESIAN_POINT ( 'NONE',  ( 10.81189881249999729, 0.000000000000000000, -33.03125000204837391 ) ) ;
#11218=CARTESIAN_POINT ( 'NONE',  ( -9.999999999999998224, 5.773502691896259087, -164.8749999999999716 ) ) ;
#11221=EDGE_CURVE ( 'NONE', #8276, #40345, #41475, .T. ) ;
#11222=CARTESIAN_POINT ( 'NONE',  ( -9.999999999999998224, 1.224646799147353059E-15, -27.12500000409676204 ) ) ;
#11223=CARTESIAN_POINT ( 'NONE',  ( 10.81189881249999729, 0.000000000000000000, -130.5312500020484094 ) ) ;
#11224=CARTESIAN_POINT ( 'NONE',  ( -9.999999999999998224, 1.224646799147353059E-15, -46.24999999999998579 ) ) ;
#11225=CARTESIAN_POINT ( 'NONE',  ( 10.00000000000051159, -5.773502691895965988, -119.5000000040967905 ) ) ;
#11226=ORIENTED_EDGE ( 'NONE', *, *, #8320, .T. ) ;
#11227=ORIENTED_EDGE ( 'NONE', *, *, #37760, .F. ) ;
#11228=ORIENTED_EDGE ( 'NONE', *, *, #31748, .F. ) ;
#11229=LINE ( 'NONE', #37571, #4543 ) ;
#11230=CARTESIAN_POINT ( 'NONE',  ( 9.999999999999998224, 0.000000000000000000, -134.0000000000000000 ) ) ;
#11231=CARTESIAN_POINT ( 'NONE',  ( -2.293366432827344421E-15, -12.48450537969573659, -166.7187500020484094 ) ) ;
#11233=CARTESIAN_POINT ( 'NONE',  ( -2.293366432827344421E-15, -12.48450537969573659, -12.21875000204837391 ) ) ;
#11235=CARTESIAN_POINT ( 'NONE',  ( -5.405949406249996869, 9.363379034771805109, -147.8437500020483810 ) ) ;
#11236=CARTESIAN_POINT ( 'NONE',  ( 5.405949406249992428, -9.363379034771808662, -133.5937500020483810 ) ) ;
#11237=CARTESIAN_POINT ( 'NONE',  ( -10.81189881249999729, 1.324075727343319199E-15, -107.2812500020483810 ) ) ;
#11241=CARTESIAN_POINT ( 'NONE',  ( 10.81189881249999729, 0.000000000000000000, -2.843750002048367698 ) ) ;
#11243=FACE_OUTER_BOUND ( 'NONE', #2022, .T. ) ;
#11244=CARTESIAN_POINT ( 'NONE',  ( -5.000000000000003553, -8.660254037844383745, -196.3750000040967905 ) ) ;
#11247=CARTESIAN_POINT ( 'NONE',  ( -10.81189881249999729, 1.324075727343319199E-15, -74.09375000204838102 ) ) ;
#11248=CARTESIAN_POINT ( 'NONE',  ( -10.81189881249999907, -6.242252689847864744, -66.46875000204838102 ) ) ;
#11250=CARTESIAN_POINT ( 'NONE',  ( -10.81189881249999729, 1.324075727343319199E-15, -38.28125000204838102 ) ) ;
#11252=CARTESIAN_POINT ( 'NONE',  ( 9.999999999998456346, 5.773502691897149042, -53.25000000409673362 ) ) ;
#11254=CARTESIAN_POINT ( 'NONE',  ( -2.121150477449813534E-15, -11.54700538379251284, -117.8749999999999858 ) ) ;
#11255=CARTESIAN_POINT ( 'NONE',  ( -10.81189881249999729, -6.242252689847864744, -128.1562500020483810 ) ) ;
#11256=CARTESIAN_POINT ( 'NONE',  ( -2.121150477449813534E-15, -11.54700538379251284, -67.25000000409676204 ) ) ;
#11258=CARTESIAN_POINT ( 'NONE',  ( -10.81189881249999729, -6.242252689847864744, -18.65625000204837036 ) ) ;
#11262=CYLINDRICAL_SURFACE ( 'NONE', #16675, 9.999999999999998224 ) ;
#11263=ADVANCED_FACE ( 'NONE', ( #723 ), #7830, .T. ) ;
#11264=CARTESIAN_POINT ( 'NONE',  ( -5.000000000000003553, -8.660254037844383745, -37.37500000409676915 ) ) ;
#11265=CARTESIAN_POINT ( 'NONE',  ( -9.999999999999998224, 1.224646799147353059E-15, -148.2500000000000000 ) ) ;
#11268=CARTESIAN_POINT ( 'NONE',  ( -5.405949406249996869, 9.363379034771805109, -154.0312500020484094 ) ) ;
#11269=CARTESIAN_POINT ( 'NONE',  ( 5.405949406249999534, 9.363379034771803333, -130.0937500020483810 ) ) ;
#11270=CARTESIAN_POINT ( 'NONE',  ( -9.999999999999998224, 1.224646799147353059E-15, -151.2500000000000000 ) ) ;
#11271=ORIENTED_EDGE ( 'NONE', *, *, #19605, .T. ) ;
#11272=DIRECTION ( 'NONE',  ( -0.000000000000000000, -0.000000000000000000, 1.000000000000000000 ) ) ;
#11274=EDGE_CURVE ( 'NONE', #31274, #41628, #34304, .T. ) ;
#11275=ORIENTED_EDGE ( 'NONE', *, *, #10422, .T. ) ;
#11276=ORIENTED_EDGE ( 'NONE', *, *, #4580, .T. ) ;
#11277=FACE_OUTER_BOUND ( 'NONE', #27644, .T. ) ;
#11278=CARTESIAN_POINT ( 'NONE',  ( 5.405949406249999534, 9.363379034771803333, -190.0937500020483810 ) ) ;
#11279=CARTESIAN_POINT ( 'NONE',  ( 5.405949406249992428, -9.363379034771808662, -37.59375000204837391 ) ) ;
#11280=CARTESIAN_POINT ( 'NONE',  ( -2.121150477449813534E-15, -11.54700538379251284, -155.7500000040968189 ) ) ;
#11281=CARTESIAN_POINT ( 'NONE',  ( -9.999999999999998224, 1.224646799147353059E-15, -34.24999999999997158 ) ) ;
#11282=CARTESIAN_POINT ( 'NONE',  ( 10.81189881249999551, -6.242252689847874514, -172.4687500020483810 ) ) ;
#11283=CARTESIAN_POINT ( 'NONE',  ( 5.405949406249992428, -9.363379034771808662, -159.0937500020484094 ) ) ;
#11284=CARTESIAN_POINT ( 'NONE',  ( 9.999999999999998224, 0.000000000000000000, -200.0000000000000000 ) ) ;
#11288=CARTESIAN_POINT ( 'NONE',  ( 9.999999999999742428, 5.773502691896404748, -134.2500000040967905 ) ) ;
#11289=LINE ( 'NONE', #33555, #23996 ) ;
#11291=CARTESIAN_POINT ( 'NONE',  ( -2.293366432827344421E-15, -12.48450537969573659, -91.71875000204838102 ) ) ;
#11293=CARTESIAN_POINT ( 'NONE',  ( 5.405949406249999534, 9.363379034771803333, -55.28125000204836681 ) ) ;
#11296=CARTESIAN_POINT ( 'NONE',  ( 5.405949406249999534, 9.363379034771803333, -113.7812500020483952 ) ) ;
#11297=CARTESIAN_POINT ( 'NONE',  ( 10.81189881249999729, 6.242252689847867408, -155.9062500020483810 ) ) ;
#11300=CARTESIAN_POINT ( 'NONE',  ( 7.070501591499377789E-16, 11.54700538379251284, -128.0000000040967620 ) ) ;
#11306=CARTESIAN_POINT ( 'NONE',  ( 9.999999999999998224, 0.000000000000000000, -6.499999999999977796 ) ) ;
#11307=CARTESIAN_POINT ( 'NONE',  ( -5.405949406249996869, 9.363379034771805109, -178.0312500020483810 ) ) ;
#11308=ORIENTED_EDGE ( 'NONE', *, *, #13750, .F. ) ;
#11309=CARTESIAN_POINT ( 'NONE',  ( 5.000000000000000000, 8.660254037844385522, -49.74999999999998579 ) ) ;
#11311=CARTESIAN_POINT ( 'NONE',  ( -4.999999999999996447, 8.660254037844387298, -60.37500000409676204 ) ) ;
#11313=CARTESIAN_POINT ( 'NONE',  ( -9.999999999999998224, 1.224646799147353059E-15, -130.2499999999999716 ) ) ;
#11315=CARTESIAN_POINT ( 'NONE',  ( 10.81189881249999551, -6.242252689847874514, -55.65625000204837391 ) ) ;
#11318=CARTESIAN_POINT ( 'NONE',  ( -4.999999999999996447, 8.660254037844387298, -157.8750000040967905 ) ) ;
#11319=CARTESIAN_POINT ( 'NONE',  ( 10.81189881249999907, 6.242252689847868297, -179.9062500020484094 ) ) ;
#11320=CARTESIAN_POINT ( 'NONE',  ( 4.999999999999992006, -8.660254037844389075, -87.74999999999998579 ) ) ;
#11323=CARTESIAN_POINT ( 'NONE',  ( 9.999999999999998224, 0.000000000000000000, -58.99999999999997158 ) ) ;
#11324=DIRECTION ( 'NONE',  ( -0.000000000000000000, -0.000000000000000000, 1.000000000000000000 ) ) ;
#11325=DIRECTION ( 'NONE',  ( 1.000000000000000000, 0.000000000000000000, 0.000000000000000000 ) ) ;
#11326=CARTESIAN_POINT ( 'NONE',  ( -2.293366432827344421E-15, -12.48450537969573659, -88.90625000204838102 ) ) ;
#11327=ORIENTED_EDGE ( 'NONE', *, *, #353, .F. ) ;
#11328=DIRECTION ( 'NONE',  ( 1.000000000000000000, 0.000000000000000000, 0.000000000000000000 ) ) ;
#11329=EDGE_CURVE ( 'NONE', #17679, #5036, #15553, .T. ) ;
#11330=CARTESIAN_POINT ( 'NONE',  ( 9.999999999999479527, 5.773502691896553074, -92.25000000409676204 ) ) ;
#11332=ORIENTED_EDGE ( 'NONE', *, *, #15911, .F. ) ;
#11333=CARTESIAN_POINT ( 'NONE',  ( 5.405949406249992428, -9.363379034771808662, -37.59375000204837391 ) ) ;
#11334=CARTESIAN_POINT ( 'NONE',  ( -10.81189881249999729, 6.242252689847871849, -27.71875000204838102 ) ) ;
#11335=CARTESIAN_POINT ( 'NONE',  ( -5.405949406250003975, -9.363379034771801557, -12.53125000204835615 ) ) ;
#11336=CARTESIAN_POINT ( 'NONE',  ( -5.405949406249996869, 9.363379034771805109, -60.84375000204836681 ) ) ;
#11337=VERTEX_POINT ( 'NONE', #8683 ) ;
#11338=CARTESIAN_POINT ( 'NONE',  ( -10.00000000000051337, 5.773502691895962435, -92.87499999999998579 ) ) ;
#11340=CARTESIAN_POINT ( 'NONE',  ( 10.81189881249999729, 0.000000000000000000, -187.3437500020483810 ) ) ;
#11344=CARTESIAN_POINT ( 'NONE',  ( 5.000000000000000000, 8.660254037844385522, -132.2499999999999716 ) ) ;
#11346=CARTESIAN_POINT ( 'NONE',  ( 9.999999999999998224, 0.000000000000000000, -20.37500000409675494 ) ) ;
#11347=CARTESIAN_POINT ( 'NONE',  ( 7.070501591499376803E-16, 11.54700538379251284, -60.50000000409677625 ) ) ;
#11348=CARTESIAN_POINT ( 'NONE',  ( -10.81189881249999907, -6.242252689847864744, -111.4687500020483810 ) ) ;
#11349=DIRECTION ( 'NONE',  ( 1.000000000000000000, 0.000000000000000000, 0.000000000000000000 ) ) ;
#11350=CARTESIAN_POINT ( 'NONE',  ( 10.81189881249999907, 6.242252689847868297, -83.90625000204836681 ) ) ;
#11351=CARTESIAN_POINT ( 'NONE',  ( 10.81189881249999551, -6.242252689847874514, -98.96875000204838102 ) ) ;
#11354=CARTESIAN_POINT ( 'NONE',  ( 7.070501591499377789E-16, 11.54700538379251284, -158.0000000040968189 ) ) ;
#11359=LINE ( 'NONE', #24554, #22011 ) ;
#11361=CARTESIAN_POINT ( 'NONE',  ( 5.000000000000000000, 8.660254037844385522, -42.62500000409677625 ) ) ;
#11362=CARTESIAN_POINT ( 'NONE',  ( 9.999999999999998224, 0.000000000000000000, -76.99999999999998579 ) ) ;
#11364=CARTESIAN_POINT ( 'NONE',  ( -9.999999999999998224, 5.773502691896259087, -79.75000000409677625 ) ) ;
#11365=CARTESIAN_POINT ( 'NONE',  ( -9.999999999999998224, 1.224646799147353059E-15, -25.62500000409675849 ) ) ;
#11367=CARTESIAN_POINT ( 'NONE',  ( 5.405949406249999534, 9.363379034771803333, -76.28125000204838102 ) ) ;
#11371=CARTESIAN_POINT ( 'NONE',  ( 10.81189881249999729, 0.000000000000000000, -199.5312500020484094 ) ) ;
#11373=CARTESIAN_POINT ( 'NONE',  ( -10.81189881249999729, 6.242252689847871849, -11.21875000204837036 ) ) ;
#11374=CARTESIAN_POINT ( 'NONE',  ( 10.00000000000102318, -5.773502691895667560, -64.00000000409674783 ) ) ;
#11376=CARTESIAN_POINT ( 'NONE',  ( -10.81189881249999907, -6.242252689847864744, -131.1562500020483810 ) ) ;
#11378=CARTESIAN_POINT ( 'NONE',  ( -9.999999999999998224, 5.773502691896259087, -185.8750000000000000 ) ) ;
#11380=CARTESIAN_POINT ( 'NONE',  ( 10.81189881249999551, -6.242252689847874514, -106.6562500020483952 ) ) ;
#11381=ORIENTED_EDGE ( 'NONE', *, *, #4319, .F. ) ;
#11386=EDGE_LOOP ( 'NONE', ( #31271, #42436, #9162, #26269 ) ) ;
#11387=( BOUNDED_CURVE ( )  B_SPLINE_CURVE ( 2, ( #41964, #34885, #38954, #12604, #5951, #32072, #8760 ),
 .UNSPECIFIED., .F., .F. ) 
 B_SPLINE_CURVE_WITH_KNOTS ( ( 3, 2, 2, 3 ),
 ( 0.9738805970149255753, 0.9751243781094529606, 0.9763681592039802348, 0.9776119402985076201 ),
 .UNSPECIFIED. ) 
 CURVE ( )  GEOMETRIC_REPRESENTATION_ITEM ( )  RATIONAL_B_SPLINE_CURVE ( ( 0.9999999999999761302, 0.8660254037844625774, 1.000000000000000000, 0.8660254037844387076, 1.000000000000000000, 0.8660254037844267172, 1.000000000000011990 ) ) 
 REPRESENTATION_ITEM ( '' )  );
#11388=CARTESIAN_POINT ( 'NONE',  ( -5.405949406249996869, 9.363379034771805109, -40.03125000204838102 ) ) ;
#11390=CARTESIAN_POINT ( 'NONE',  ( 10.81189881249999907, 6.242252689847868297, -85.21875000204836681 ) ) ;
#11393=VECTOR ( 'NONE', #29049, 1000.000000000000000 ) ;
#11397=CARTESIAN_POINT ( 'NONE',  ( -10.81189881249999729, 6.242252689847871849, -122.2187500020483810 ) ) ;
#11399=CARTESIAN_POINT ( 'NONE',  ( 10.81189881249999729, 0.000000000000000000, -3.031250002048374803 ) ) ;
#11402=CARTESIAN_POINT ( 'NONE',  ( 5.000000000000000000, 8.660254037844385522, -176.1250000040968189 ) ) ;
#11403=CARTESIAN_POINT ( 'NONE',  ( 5.405949406249992428, -9.363379034771808662, -172.7812500020484094 ) ) ;
#11404=CARTESIAN_POINT ( 'NONE',  ( 10.00000000000102318, -5.773502691895667560, -70.00000000409676204 ) ) ;
#11407=CARTESIAN_POINT ( 'NONE',  ( 7.644554776091147741E-16, 12.48450537969573659, -53.46875000204838102 ) ) ;
#11409=CARTESIAN_POINT ( 'NONE',  ( -2.293366432827344421E-15, -12.48450537969573659, -12.40625000204835970 ) ) ;
#11411=CARTESIAN_POINT ( 'NONE',  ( -9.999999999999612754, -5.773502691896474914, -153.0000000040967620 ) ) ;
#11413=CARTESIAN_POINT ( 'NONE',  ( -2.121150477449813534E-15, -11.54700538379251284, -96.87500000000000000 ) ) ;
#11415=CARTESIAN_POINT ( 'NONE',  ( 10.00000000000000000, 5.773502691896255534, -105.7500000040967905 ) ) ;
#11417=CARTESIAN_POINT ( 'NONE',  ( 10.00000000000021672, -5.773502691896130301, -190.0000000040968189 ) ) ;
#11420=CARTESIAN_POINT ( 'NONE',  ( -5.405949406250003975, -9.363379034771801557, -96.53125000204839523 ) ) ;
#11423=CARTESIAN_POINT ( 'NONE',  ( -2.121150477449813534E-15, -11.54700538379251284, -166.2500000040968189 ) ) ;
#11424=CARTESIAN_POINT ( 'NONE',  ( 7.644554776091147741E-16, 12.48450537969573659, -163.1562500020484094 ) ) ;
#11426=ORIENTED_EDGE ( 'NONE', *, *, #17223, .T. ) ;
#11427=CARTESIAN_POINT ( 'NONE',  ( 9.999999999999996447, -5.773502691896262640, -29.12499999999997513 ) ) ;
#11428=CARTESIAN_POINT ( 'NONE',  ( -5.405949406250003975, -9.363379034771801557, -30.53125000204837036 ) ) ;
#11429=CARTESIAN_POINT ( 'NONE',  ( 9.999999999999998224, 0.000000000000000000, -158.0000000000000000 ) ) ;
#11433=CARTESIAN_POINT ( 'NONE',  ( 4.999999999999992006, -8.660254037844389075, -23.24999999999996447 ) ) ;
#11434=CARTESIAN_POINT ( 'NONE',  ( -5.405949406250003975, -9.363379034771801557, -131.0312500020484094 ) ) ;
#11439=CARTESIAN_POINT ( 'NONE',  ( 10.81189881249999729, 0.000000000000000000, -64.53125000204836681 ) ) ;
#11440=EDGE_CURVE ( 'NONE', #35715, #34507, #25724, .T. ) ;
#11442=ORIENTED_EDGE ( 'NONE', *, *, #9661, .T. ) ;
#11443=CARTESIAN_POINT ( 'NONE',  ( -9.999999999999479527, -5.773502691896549521, -46.50000000409676204 ) ) ;
#11444=CARTESIAN_POINT ( 'NONE',  ( -10.81189881249999907, -6.242252689847864744, -157.9687500020484379 ) ) ;
#11446=CARTESIAN_POINT ( 'NONE',  ( 5.405949406249999534, 9.363379034771803333, -19.09375000204835260 ) ) ;
#11447=CARTESIAN_POINT ( 'NONE',  ( -9.999999999999998224, 1.224646799147353059E-15, -200.0000000000000000 ) ) ;
#11448=CARTESIAN_POINT ( 'NONE',  ( 5.405949406249999534, 9.363379034771803333, -149.5937500020483810 ) ) ;
#11449=CARTESIAN_POINT ( 'NONE',  ( -10.81189881249999907, -6.242252689847864744, -127.9687500020483810 ) ) ;
#11450=CARTESIAN_POINT ( 'NONE',  ( 10.81189881249999729, 0.000000000000000000, -106.5312500020483810 ) ) ;
#11452=CARTESIAN_POINT ( 'NONE',  ( 9.999999999999998224, 0.000000000000000000, -2.375000004096766482 ) ) ;
#11454=CARTESIAN_POINT ( 'NONE',  ( 5.405949406249992428, -9.363379034771808662, -4.593750002048368586 ) ) ;
#11456=EDGE_CURVE ( 'NONE', #3313, #8277, #23594, .T. ) ;
#11460=CARTESIAN_POINT ( 'NONE',  ( -10.81189881249999729, -6.242252689847864744, -78.46875000204838102 ) ) ;
#11461=CARTESIAN_POINT ( 'NONE',  ( 5.405949406249999534, 9.363379034771803333, -59.59375000204835970 ) ) ;
#11463=CARTESIAN_POINT ( 'NONE',  ( -10.81189881249999729, 1.324075727343319199E-15, -36.78125000204837391 ) ) ;
#11465=FACE_OUTER_BOUND ( 'NONE', #267, .T. ) ;
#11467=CARTESIAN_POINT ( 'NONE',  ( 7.070501591499377789E-16, 11.54700538379251284, -120.1249999999999858 ) ) ;
#11468=CARTESIAN_POINT ( 'NONE',  ( 4.999999999999992006, -8.660254037844389075, -67.12500000409676204 ) ) ;
#11470=CARTESIAN_POINT ( 'NONE',  ( 7.644554776091147741E-16, 12.48450537969573659, -8.656250002048372139 ) ) ;
#11471=ORIENTED_EDGE ( 'NONE', *, *, #36313, .T. ) ;
#11476=CARTESIAN_POINT ( 'NONE',  ( 4.999999999999992006, -8.660254037844389075, -31.12500000409676559 ) ) ;
#11477=CARTESIAN_POINT ( 'NONE',  ( -5.000000000000003553, -8.660254037844383745, -14.49999999999995737 ) ) ;
#11480=CARTESIAN_POINT ( 'NONE',  ( -5.405949406250003975, -9.363379034771801557, -143.0312500020483810 ) ) ;
#11481=CARTESIAN_POINT ( 'NONE',  ( 10.81189881249999907, 6.242252689847868297, -124.2187500020483952 ) ) ;
#11482=CARTESIAN_POINT ( 'NONE',  ( 5.000000000000000000, 8.660254037844385522, -104.1250000040967763 ) ) ;
#11483=CARTESIAN_POINT ( 'NONE',  ( 9.999999999999998224, 0.000000000000000000, -32.37500000409676204 ) ) ;
#11484=ORIENTED_EDGE ( 'NONE', *, *, #5611, .T. ) ;
#11486=ORIENTED_EDGE ( 'NONE', *, *, #1701, .F. ) ;
#11489=CARTESIAN_POINT ( 'NONE',  ( 10.81189881249999729, 0.000000000000000000, -187.3437500020483810 ) ) ;
#11490=CARTESIAN_POINT ( 'NONE',  ( -2.293366432827344421E-15, -12.48450537969573659, -37.71875000204836681 ) ) ;
#11494=CARTESIAN_POINT ( 'NONE',  ( -10.81189881249999729, 6.242252689847871849, -173.2187500020483810 ) ) ;
#11495=CARTESIAN_POINT ( 'NONE',  ( 5.405949406249992428, -9.363379034771808662, -150.0937500020483810 ) ) ;
#11496=CARTESIAN_POINT ( 'NONE',  ( -9.999999999998456346, -5.773502691897145489, -25.50000000409673007 ) ) ;
#11501=CARTESIAN_POINT ( 'NONE',  ( 7.070501591499376803E-16, 11.54700538379251284, -87.12500000000000000 ) ) ;
#11502=CARTESIAN_POINT ( 'NONE',  ( 5.000000000000000000, 8.660254037844385522, -36.24999999999997868 ) ) ;
#11504=CARTESIAN_POINT ( 'NONE',  ( -5.405949406250003975, -9.363379034771801557, -87.34375000204836681 ) ) ;
#11505=CARTESIAN_POINT ( 'NONE',  ( -9.999999999999740652, 5.773502691896409189, -180.2500000040967905 ) ) ;
#11506=CARTESIAN_POINT ( 'NONE',  ( 10.81189881249999729, 0.000000000000000000, -57.03125000204836681 ) ) ;
#11509=CARTESIAN_POINT ( 'NONE',  ( 10.81189881249999551, -6.242252689847874514, -117.1562500020483810 ) ) ;
#11510=CARTESIAN_POINT ( 'NONE',  ( -5.405949406250003975, -9.363379034771801557, -152.0312500020484094 ) ) ;
#11511=CARTESIAN_POINT ( 'NONE',  ( 9.999999999999998224, 0.000000000000000000, -3.875000004096768258 ) ) ;
#11513=CARTESIAN_POINT ( 'NONE',  ( -5.000000000000003553, -8.660254037844383745, -127.3750000040967905 ) ) ;
#11518=FACE_OUTER_BOUND ( 'NONE', #9017, .T. ) ;
#11519=CARTESIAN_POINT ( 'NONE',  ( -10.81189881249999907, -6.242252689847864744, -179.1562500020484094 ) ) ;
#11520=ORIENTED_EDGE ( 'NONE', *, *, #33333, .F. ) ;
#11522=CARTESIAN_POINT ( 'NONE',  ( -10.00000000000000000, -5.773502691896251982, -58.50000000409676204 ) ) ;
#11523=CARTESIAN_POINT ( 'NONE',  ( -2.121150477449813534E-15, -11.54700538379251284, -18.87499999999997868 ) ) ;
#11524=CARTESIAN_POINT ( 'NONE',  ( 5.000000000000000000, 8.660254037844385522, -171.6250000040968189 ) ) ;
#11526=CARTESIAN_POINT ( 'NONE',  ( 10.81189881249999729, 0.000000000000000000, -54.03125000204836681 ) ) ;
#11529=CARTESIAN_POINT ( 'NONE',  ( 4.999999999999992006, -8.660254037844389075, -29.62500000409676204 ) ) ;
#11530=CARTESIAN_POINT ( 'NONE',  ( 10.81189881249999907, 6.242252689847868297, -176.9062500020484094 ) ) ;
#11531=CARTESIAN_POINT ( 'NONE',  ( 9.999999999999998224, 0.000000000000000000, -200.0000000000000000 ) ) ;
#11532=CARTESIAN_POINT ( 'NONE',  ( 9.999999999999998224, 0.000000000000000000, -173.0000000000000284 ) ) ;
#11533=ORIENTED_EDGE ( 'NONE', *, *, #10069, .F. ) ;
#11534=CARTESIAN_POINT ( 'NONE',  ( -9.999999999998969713, -5.773502691896847949, -61.12499999999996447 ) ) ;
#11535=CARTESIAN_POINT ( 'NONE',  ( 10.81189881249999907, 6.242252689847868297, -85.40625000204839523 ) ) ;
#11537=( LENGTH_UNIT ( ) NAMED_UNIT ( * ) SI_UNIT ( .MILLI., .METRE. ) );
#11538=CARTESIAN_POINT ( 'NONE',  ( 5.000000000000000000, 8.660254037844385522, -92.12500000409677625 ) ) ;
#11539=VERTEX_POINT ( 'NONE', #16818 ) ;
#11540=ORIENTED_EDGE ( 'NONE', *, *, #17511, .F. ) ;
#11541=CARTESIAN_POINT ( 'NONE',  ( -10.81189881249999729, -6.242252689847864744, -40.96875000204835260 ) ) ;
#11542=CARTESIAN_POINT ( 'NONE',  ( -4.999999999999996447, 8.660254037844387298, -76.87500000409677625 ) ) ;
#11543=CARTESIAN_POINT ( 'NONE',  ( 7.644554776091147741E-16, 12.48450537969573659, -11.65625000204835438 ) ) ;
#11544=CARTESIAN_POINT ( 'NONE',  ( -5.405949406250003975, -9.363379034771801557, -66.34375000204836681 ) ) ;
#11545=ORIENTED_EDGE ( 'NONE', *, *, #34606, .F. ) ;
#11547=CARTESIAN_POINT ( 'NONE',  ( 5.405949406249992428, -9.363379034771808662, -187.5937500020483810 ) ) ;
#11550=CARTESIAN_POINT ( 'NONE',  ( -2.121150477449813534E-15, -11.54700538379251284, -182.7500000040967905 ) ) ;
#11554=CARTESIAN_POINT ( 'NONE',  ( -2.293366432827344421E-15, -12.48450537969573659, -115.7187500020483952 ) ) ;
#11555=CARTESIAN_POINT ( 'NONE',  ( 9.999999999999998224, 0.000000000000000000, -200.0000000000000000 ) ) ;
#11556=AXIS2_PLACEMENT_3D ( 'NONE', #24433, #1766, #29099 ) ;
#11557=CARTESIAN_POINT ( 'NONE',  ( 5.405949406249999534, 9.363379034771803333, -83.78125000204838102 ) ) ;
#11558=CARTESIAN_POINT ( 'NONE',  ( 5.405949406249992428, -9.363379034771808662, -90.09375000204838102 ) ) ;
#11562=CARTESIAN_POINT ( 'NONE',  ( 4.999999999999992006, -8.660254037844389075, -155.6250000040967905 ) ) ;
#11564=EDGE_CURVE ( 'NONE', #11901, #14343, #38713, .T. ) ;
#11567=CARTESIAN_POINT ( 'NONE',  ( 9.999999999999866773, -5.773502691896336358, -174.6249999999999716 ) ) ;
#11568=DIRECTION ( 'NONE',  ( -0.000000000000000000, -0.000000000000000000, 1.000000000000000000 ) ) ;
#11570=CARTESIAN_POINT ( 'NONE',  ( -9.999999999999998224, 1.224646799147353059E-15, -42.12500000409677625 ) ) ;
#11571=CARTESIAN_POINT ( 'NONE',  ( -4.999999999999996447, 8.660254037844387298, -74.99999999999998579 ) ) ;
#11573=CARTESIAN_POINT ( 'NONE',  ( -9.999999999999998224, 5.773502691896259087, -78.25000000409677625 ) ) ;
#11576=CARTESIAN_POINT ( 'NONE',  ( -10.81189881249999729, 6.242252689847871849, -72.90625000204836681 ) ) ;
#11579=ORIENTED_EDGE ( 'NONE', *, *, #39797, .T. ) ;
#11580=CARTESIAN_POINT ( 'NONE',  ( -9.999999999999998224, 1.224646799147353059E-15, -1.249999999999973355 ) ) ;
#11582=CARTESIAN_POINT ( 'NONE',  ( 10.81189881249999729, 0.000000000000000000, -13.34375000204834905 ) ) ;
#11583=CARTESIAN_POINT ( 'NONE',  ( 9.999999999999998224, 0.000000000000000000, -176.3750000040967905 ) ) ;
#11584=CARTESIAN_POINT ( 'NONE',  ( -10.81189881249999729, 1.324075727343319199E-15, -143.0937500020483810 ) ) ;
#11587=CARTESIAN_POINT ( 'NONE',  ( 10.81189881249999729, 0.000000000000000000, -130.5312500020484094 ) ) ;
#11588=CARTESIAN_POINT ( 'NONE',  ( 7.070501591499377789E-16, 11.54700538379251284, -181.6250000000000000 ) ) ;
#11589=DIRECTION ( 'NONE',  ( -0.000000000000000000, -0.000000000000000000, 1.000000000000000000 ) ) ;
#11590=CARTESIAN_POINT ( 'NONE',  ( 5.405949406249999534, 9.363379034771803333, -110.7812500020483810 ) ) ;
#11592=CARTESIAN_POINT ( 'NONE',  ( -4.999999999999996447, 8.660254037844387298, -195.0000000000000000 ) ) ;
#11593=VECTOR ( 'NONE', #15163, 1000.000000000000000 ) ;
#11594=ORIENTED_EDGE ( 'NONE', *, *, #21376, .T. ) ;
#11595=( BOUNDED_CURVE ( )  B_SPLINE_CURVE ( 2, ( #26848, #17114, #10641, #30530, #14290, #27066, #21004 ),
 .UNSPECIFIED., .F., .F. ) 
 B_SPLINE_CURVE_WITH_KNOTS ( ( 3, 2, 2, 3 ),
 ( 0.8320895522388060961, 0.8333333333333334814, 0.8345771144278608666, 0.8358208955223882519 ),
 .UNSPECIFIED. ) 
 CURVE ( )  GEOMETRIC_REPRESENTATION_ITEM ( )  RATIONAL_B_SPLINE_CURVE ( ( 0.9999999999999880096, 0.8660254037844506980, 1.000000000000000000, 0.8660254037844387076, 1.000000000000000000, 0.8660254037844148378, 1.000000000000023981 ) ) 
 REPRESENTATION_ITEM ( '' )  );
#11597=CARTESIAN_POINT ( 'NONE',  ( -10.81189881249999907, -6.242252689847864744, -41.15625000204836681 ) ) ;
#11599=CARTESIAN_POINT ( 'NONE',  ( 5.405949406249999534, 9.363379034771803333, -86.59375000204836681 ) ) ;
#11602=CARTESIAN_POINT ( 'NONE',  ( -5.000000000000003553, -8.660254037844383745, -32.87500000409676915 ) ) ;
#11604=DIRECTION ( 'NONE',  ( 1.000000000000000000, 0.000000000000000000, 0.000000000000000000 ) ) ;
#11605=CARTESIAN_POINT ( 'NONE',  ( 10.81189881249999729, 0.000000000000000000, -112.3437500020483810 ) ) ;
#11607=CARTESIAN_POINT ( 'NONE',  ( 5.405949406249999534, 9.363379034771803333, -4.281250002048375691 ) ) ;
#11610=CARTESIAN_POINT ( 'NONE',  ( -10.00000000000000000, -5.773502691896251982, -180.0000000040967905 ) ) ;
#11611=CARTESIAN_POINT ( 'NONE',  ( 10.81189881249999551, -6.242252689847874514, -172.6562500020484094 ) ) ;
#11612=CARTESIAN_POINT ( 'NONE',  ( -9.999999999999998224, 1.224646799147353059E-15, -144.1250000040967905 ) ) ;
#11615=CARTESIAN_POINT ( 'NONE',  ( -10.81189881249999729, 6.242252689847871849, -50.21875000204835970 ) ) ;
#11617=CARTESIAN_POINT ( 'NONE',  ( -5.405949406250003975, -9.363379034771801557, -8.031250002048350822 ) ) ;
#11619=CARTESIAN_POINT ( 'NONE',  ( -9.999999999999998224, 1.224646799147353059E-15, -165.1250000040967905 ) ) ;
#11621=ADVANCED_FACE ( 'NONE', ( #3470 ), #3261, .T. ) ;
#11622=CARTESIAN_POINT ( 'NONE',  ( -2.121150477449813534E-15, -11.54700538379251284, -93.87499999999997158 ) ) ;
#11624=CARTESIAN_POINT ( 'NONE',  ( 5.000000000000000000, 8.660254037844385522, -107.1250000040967763 ) ) ;
#11625=CARTESIAN_POINT ( 'NONE',  ( 9.999999999999998224, 0.000000000000000000, -197.0000000000000000 ) ) ;
#11629=CARTESIAN_POINT ( 'NONE',  ( 10.81189881249999729, 0.000000000000000000, -100.5312500020483952 ) ) ;
#11633=CARTESIAN_POINT ( 'NONE',  ( 10.81189881249999907, 6.242252689847868297, -157.4062500020483810 ) ) ;
#11635=ORIENTED_EDGE ( 'NONE', *, *, #35860, .T. ) ;
#11636=CARTESIAN_POINT ( 'NONE',  ( -10.00000000000000000, -5.773502691896251982, -26.62499999999998224 ) ) ;
#11637=VECTOR ( 'NONE', #40674, 1000.000000000000000 ) ;
#11638=CARTESIAN_POINT ( 'NONE',  ( -10.81189881249999729, 6.242252689847871849, -29.40625000204835615 ) ) ;
#11639=CARTESIAN_POINT ( 'NONE',  ( -9.999999999999998224, 5.773502691896259087, -161.8750000000000000 ) ) ;
#11640=CARTESIAN_POINT ( 'NONE',  ( 9.999999999999998224, 0.000000000000000000, -90.49999999999998579 ) ) ;
#11645=CARTESIAN_POINT ( 'NONE',  ( 5.405949406249999534, 9.363379034771803333, -134.7812500020483810 ) ) ;
#11646=CARTESIAN_POINT ( 'NONE',  ( 3.170450507625008019, 9.888387355072444151, 1.028787474604544383E-14 ) ) ;
#11647=CARTESIAN_POINT ( 'NONE',  ( 9.999999999999998224, 0.000000000000000000, -68.37500000409677625 ) ) ;
#11649=( BOUNDED_CURVE ( )  B_SPLINE_CURVE ( 2, ( #9475, #38616, #42262, #32159, #25051, #9053, #5606 ),
 .UNSPECIFIED., .F., .F. ) 
 B_SPLINE_CURVE_WITH_KNOTS ( ( 3, 2, 2, 3 ),
 ( 0.9701492537313435305, 0.9713930348258709158, 0.9726368159203981900, 0.9738805970149255753 ),
 .UNSPECIFIED. ) 
 CURVE ( )  GEOMETRIC_REPRESENTATION_ITEM ( )  RATIONAL_B_SPLINE_CURVE ( ( 0.9999999999999761302, 0.8660254037844625774, 1.000000000000000000, 0.8660254037844387076, 1.000000000000000000, 0.8660254037844148378, 1.000000000000023981 ) ) 
 REPRESENTATION_ITEM ( '' )  );
#11650=CARTESIAN_POINT ( 'NONE',  ( -10.81189881249999729, 1.324075727343319199E-15, -65.28125000204838102 ) ) ;
#11652=ORIENTED_EDGE ( 'NONE', *, *, #22674, .F. ) ;
#11653=ORIENTED_EDGE ( 'NONE', *, *, #33333, .T. ) ;
#11654=CARTESIAN_POINT ( 'NONE',  ( 10.00000000000102318, -5.773502691895667560, -46.00000000409674072 ) ) ;
#11656=CARTESIAN_POINT ( 'NONE',  ( 5.405949406249999534, 9.363379034771803333, -161.5937500020484094 ) ) ;
#11658=CARTESIAN_POINT ( 'NONE',  ( 5.405949406249999534, 9.363379034771803333, -7.093750002048371250 ) ) ;
#11660=CARTESIAN_POINT ( 'NONE',  ( -10.81189881249999729, 1.324075727343319199E-15, -146.0937500020483810 ) ) ;
#11661=CARTESIAN_POINT ( 'NONE',  ( -10.81189881249999907, -6.242252689847864744, -95.15625000204839523 ) ) ;
#11665=CARTESIAN_POINT ( 'NONE',  ( -2.293366432827344421E-15, -12.48450537969573659, -4.718750002048369474 ) ) ;
#11667=CARTESIAN_POINT ( 'NONE',  ( -10.81189881249999729, 1.324075727343319199E-15, -191.2812500020484094 ) ) ;
#11672=CARTESIAN_POINT ( 'NONE',  ( 10.81189881249999729, 0.000000000000000000, -74.84375000204838102 ) ) ;
#11673=CARTESIAN_POINT ( 'NONE',  ( -5.405949406250003975, -9.363379034771801557, -60.34375000204835970 ) ) ;
#11675=CARTESIAN_POINT ( 'NONE',  ( 10.81189881249999907, 6.242252689847868297, -31.40625000204834905 ) ) ;
#11677=DIRECTION ( 'NONE',  ( 1.000000000000000000, 0.000000000000000000, 0.000000000000000000 ) ) ;
#11679=EDGE_CURVE ( 'NONE', #24959, #28547, #157, .T. ) ;
#11680=CARTESIAN_POINT ( 'NONE',  ( -9.999999999999998224, 5.773502691896259087, -124.3750000000000000 ) ) ;
#11681=ADVANCED_FACE ( 'NONE', ( #248 ), #15972, .T. ) ;
#11682=CARTESIAN_POINT ( 'NONE',  ( -4.999999999999996447, 8.660254037844387298, -41.99999999999997868 ) ) ;
#11683=EDGE_CURVE ( 'NONE', #12029, #30470, #20543, .T. ) ;
#11686=CARTESIAN_POINT ( 'NONE',  ( -5.405949406250003975, -9.363379034771801557, -9.531250002048352599 ) ) ;
#11688=ORIENTED_EDGE ( 'NONE', *, *, #12166, .F. ) ;
#11691=FACE_OUTER_BOUND ( 'NONE', #28980, .T. ) ;
#11693=CARTESIAN_POINT ( 'NONE',  ( 9.999999999999998224, 0.000000000000000000, -24.87500000409675849 ) ) ;
#11694=LINE ( 'NONE', #41252, #24901 ) ;
#11698=CARTESIAN_POINT ( 'NONE',  ( 10.81189881249999907, 6.242252689847868297, -148.4062500020484094 ) ) ;
#11699=CARTESIAN_POINT ( 'NONE',  ( -5.405949406249996869, 9.363379034771805109, -125.3437500020483952 ) ) ;
#11700=CARTESIAN_POINT ( 'NONE',  ( 5.000000000000000000, 8.660254037844385522, -51.24999999999996447 ) ) ;
#11702=CARTESIAN_POINT ( 'NONE',  ( -5.000000000000003553, -8.660254037844383745, -57.99999999999997158 ) ) ;
#11704=EDGE_CURVE ( 'NONE', #8850, #34991, #40083, .T. ) ;
#11705=ORIENTED_EDGE ( 'NONE', *, *, #20399, .T. ) ;
#11707=CARTESIAN_POINT ( 'NONE',  ( 4.999999999999992006, -8.660254037844389075, -145.1250000040967905 ) ) ;
#11708=CARTESIAN_POINT ( 'NONE',  ( -10.81189881249999729, 6.242252689847871849, -180.7187500020483810 ) ) ;
#11709=CARTESIAN_POINT ( 'NONE',  ( -10.81189881249999729, 1.324075727343319199E-15, -29.09375000204836326 ) ) ;
#11710=CARTESIAN_POINT ( 'NONE',  ( 10.81189881249999729, 6.242252689847867408, -172.2187500020483810 ) ) ;
#11711=CARTESIAN_POINT ( 'NONE',  ( -5.405949406250003975, -9.363379034771801557, -153.3437500020483810 ) ) ;
#11712=ADVANCED_FACE ( 'NONE', ( #4741 ), #27410, .T. ) ;
#11713=( BOUNDED_CURVE ( )  B_SPLINE_CURVE ( 2, ( #27037, #20977, #24019, #17941, #31140, #37160, #7396 ),
 .UNSPECIFIED., .F., .F. ) 
 B_SPLINE_CURVE_WITH_KNOTS ( ( 3, 2, 2, 3 ),
 ( 0.5223880597014926019, 0.5236318407960199872, 0.5248756218905473725, 0.5261194029850747578 ),
 .UNSPECIFIED. ) 
 CURVE ( )  GEOMETRIC_REPRESENTATION_ITEM ( )  RATIONAL_B_SPLINE_CURVE ( ( 0.9999999999999880096, 0.8660254037844506980, 1.000000000000000000, 0.8660254037844387076, 1.000000000000000000, 0.8660254037844267172, 1.000000000000011990 ) ) 
 REPRESENTATION_ITEM ( '' )  );
#11714=DIRECTION ( 'NONE',  ( -0.000000000000000000, -0.000000000000000000, 1.000000000000000000 ) ) ;
#11718=DIRECTION ( 'NONE',  ( -0.000000000000000000, -0.000000000000000000, 1.000000000000000000 ) ) ;
#11719=CARTESIAN_POINT ( 'NONE',  ( 7.070501591499376803E-16, 11.54700538379251284, -11.00000000409676382 ) ) ;
#11722=CARTESIAN_POINT ( 'NONE',  ( -10.81189881249999729, 1.324075727343319199E-15, -80.09375000204838102 ) ) ;
#11723=CARTESIAN_POINT ( 'NONE',  ( 4.999999999999992006, -8.660254037844389075, -135.7499999999999716 ) ) ;
#11724=CARTESIAN_POINT ( 'NONE',  ( 7.644554776091147741E-16, 12.48450537969573659, -61.15625000204838102 ) ) ;
#11727=CARTESIAN_POINT ( 'NONE',  ( -10.81189881249999729, 1.324075727343319199E-15, -117.7812500020483952 ) ) ;
#11728=CARTESIAN_POINT ( 'NONE',  ( 7.644554776091147741E-16, 12.48450537969573659, -155.6562500020483810 ) ) ;
#11729=CARTESIAN_POINT ( 'NONE',  ( 9.999999999999998224, 0.000000000000000000, -103.9999999999999858 ) ) ;
#11731=CARTESIAN_POINT ( 'NONE',  ( 9.999999999999996447, -5.773502691896262640, -124.0000000040967763 ) ) ;
#11733=ORIENTED_EDGE ( 'NONE', *, *, #27221, .F. ) ;
#11736=DIRECTION ( 'NONE',  ( -0.000000000000000000, -0.000000000000000000, 1.000000000000000000 ) ) ;
#11737=CARTESIAN_POINT ( 'NONE',  ( 10.81189881249999729, 0.000000000000000000, -180.0312500020483810 ) ) ;
#11740=CARTESIAN_POINT ( 'NONE',  ( 10.00000000000000000, 5.773502691896255534, -57.75000000409677625 ) ) ;
#11741=FACE_OUTER_BOUND ( 'NONE', #9536, .T. ) ;
#11746=CARTESIAN_POINT ( 'NONE',  ( 5.000000000000000000, 8.660254037844385522, -9.625000004096746054 ) ) ;
#11747=CARTESIAN_POINT ( 'NONE',  ( 10.81189881249999907, 6.242252689847868297, -172.4062500020484094 ) ) ;
#11749=CARTESIAN_POINT ( 'NONE',  ( 7.071067811865472841, 7.071067811865472841, -200.0000000000000000 ) ) ;
#11751=CARTESIAN_POINT ( 'NONE',  ( 5.000000000000000000, 8.660254037844385522, -123.6250000040967905 ) ) ;
#11752=CARTESIAN_POINT ( 'NONE',  ( -10.00000000000051337, 5.773502691895962435, -39.25000000409674072 ) ) ;
#11753=VECTOR ( 'NONE', #40513, 1000.000000000000000 ) ;
#11754=CARTESIAN_POINT ( 'NONE',  ( 10.81189881249999551, -6.242252689847874514, -79.65625000204838102 ) ) ;
#11755=ORIENTED_EDGE ( 'NONE', *, *, #23564, .T. ) ;
#11757=CARTESIAN_POINT ( 'NONE',  ( -5.000000000000003553, -8.660254037844383745, -140.5000000000000000 ) ) ;
#11760=( BOUNDED_CURVE ( )  B_SPLINE_CURVE ( 2, ( #38939, #9370, #22540, #35713, #32480, #2906, #33327 ),
 .UNSPECIFIED., .F., .F. ) 
 B_SPLINE_CURVE_WITH_KNOTS ( ( 3, 2, 2, 3 ),
 ( 0.5895522388059702967, 0.5907960199004975710, 0.5920398009950249563, 0.5932835820895523415 ),
 .UNSPECIFIED. ) 
 CURVE ( )  GEOMETRIC_REPRESENTATION_ITEM ( )  RATIONAL_B_SPLINE_CURVE ( ( 0.9999999999999880096, 0.8660254037844506980, 1.000000000000000000, 0.8660254037844387076, 1.000000000000000000, 0.8660254037844267172, 1.000000000000011990 ) ) 
 REPRESENTATION_ITEM ( '' )  );
#11761=CARTESIAN_POINT ( 'NONE',  ( 10.81189881249999729, 0.000000000000000000, -35.84375000204836681 ) ) ;
#11762=CARTESIAN_POINT ( 'NONE',  ( 9.999999999999998224, 0.000000000000000000, -77.37500000409677625 ) ) ;
#11763=CARTESIAN_POINT ( 'NONE',  ( 10.81189881249999907, 6.242252689847868297, -8.906250002048375691 ) ) ;
#11764=CARTESIAN_POINT ( 'NONE',  ( 5.405949406249992428, -9.363379034771808662, -66.09375000204836681 ) ) ;
#11765=VERTEX_POINT ( 'NONE', #17248 ) ;
#11768=CARTESIAN_POINT ( 'NONE',  ( 10.81189881249999729, 6.242252689847867408, -199.2187500020484094 ) ) ;
#11769=CARTESIAN_POINT ( 'NONE',  ( -5.405949406249996869, 9.363379034771805109, -174.8437500020484094 ) ) ;
#11772=CARTESIAN_POINT ( 'NONE',  ( 7.070501591499376803E-16, 11.54700538379251284, -18.50000000409676559 ) ) ;
#11775=CARTESIAN_POINT ( 'NONE',  ( 10.81189881249999551, -6.242252689847874514, -103.4687500020483810 ) ) ;
#11777=CARTESIAN_POINT ( 'NONE',  ( 7.644554776091147741E-16, 12.48450537969573659, -80.65625000204839523 ) ) ;
#11778=CARTESIAN_POINT ( 'NONE',  ( 10.81189881249999729, 0.000000000000000000, -91.34375000204838102 ) ) ;
#11780=CARTESIAN_POINT ( 'NONE',  ( -4.999999999999996447, 8.660254037844387298, -156.3750000040967905 ) ) ;
#11786=DIRECTION ( 'NONE',  ( 1.000000000000000000, 0.000000000000000000, 0.000000000000000000 ) ) ;
#11788=ORIENTED_EDGE ( 'NONE', *, *, #14049, .T. ) ;
#11789=CARTESIAN_POINT ( 'NONE',  ( 5.000000000000000000, 8.660254037844385522, -67.74999999999997158 ) ) ;
#11791=CARTESIAN_POINT ( 'NONE',  ( 4.999999999999992006, -8.660254037844389075, -85.12500000409677625 ) ) ;
#11795=CARTESIAN_POINT ( 'NONE',  ( -5.405949406250003975, -9.363379034771801557, -77.03125000204838102 ) ) ;
#11797=CARTESIAN_POINT ( 'NONE',  ( -9.999999999999998224, 1.224646799147353059E-15, -78.12500000409677625 ) ) ;
#11800=CARTESIAN_POINT ( 'NONE',  ( 5.405949406249999534, 9.363379034771803333, -190.2812500020484094 ) ) ;
#11801=EDGE_CURVE ( 'NONE', #16199, #25687, #37063, .T. ) ;
#11803=CARTESIAN_POINT ( 'NONE',  ( -10.81189881249999729, 1.324075727343319199E-15, -6.593750002048370362 ) ) ;
#11804=CARTESIAN_POINT ( 'NONE',  ( -5.000000000000003553, -8.660254037844383745, -94.37500000409677625 ) ) ;
#11805=CARTESIAN_POINT ( 'NONE',  ( -2.293366432827344421E-15, -12.48450537969573659, -145.7187500020484094 ) ) ;
#11806=CARTESIAN_POINT ( 'NONE',  ( 9.999999999999872102, 5.773502691896329253, -161.2500000040967905 ) ) ;
#11807=CARTESIAN_POINT ( 'NONE',  ( 10.00000000000000000, 5.773502691896255534, -180.3750000000000284 ) ) ;
#11808=CARTESIAN_POINT ( 'NONE',  ( 9.999999999999548805, 5.773502691896514882, -176.2500000040967905 ) ) ;
#11809=CARTESIAN_POINT ( 'NONE',  ( 10.81189881249999729, 0.000000000000000000, -100.5312500020483952 ) ) ;
#11810=ORIENTED_EDGE ( 'NONE', *, *, #26407, .F. ) ;
#11811=CARTESIAN_POINT ( 'NONE',  ( 9.999999999999998224, 0.000000000000000000, -200.0000000000000000 ) ) ;
#11813=ORIENTED_EDGE ( 'NONE', *, *, #37255, .T. ) ;
#11814=EDGE_CURVE ( 'NONE', #5330, #38561, #10563, .T. ) ;
#11815=CARTESIAN_POINT ( 'NONE',  ( -10.81189881249999729, 1.324075727343319199E-15, -39.78125000204838102 ) ) ;
#11818=CARTESIAN_POINT ( 'NONE',  ( -10.81189881249999729, 6.242252689847871849, -84.71875000204836681 ) ) ;
#11820=DIRECTION ( 'NONE',  ( -0.000000000000000000, -0.000000000000000000, 1.000000000000000000 ) ) ;
#11821=CARTESIAN_POINT ( 'NONE',  ( 9.999999999999998224, 0.000000000000000000, -63.87500000409676915 ) ) ;
#11824=CARTESIAN_POINT ( 'NONE',  ( -2.121150477449813534E-15, -11.54700538379251284, -86.37500000000000000 ) ) ;
#11825=CARTESIAN_POINT ( 'NONE',  ( 10.81189881249999729, 6.242252689847867408, -119.7187500020483810 ) ) ;
#11827=CARTESIAN_POINT ( 'NONE',  ( -5.405949406249996869, 9.363379034771805109, -2.531250002048373915 ) ) ;
#11830=CARTESIAN_POINT ( 'NONE',  ( -9.999999999999998224, 5.773502691896259087, -177.2500000040967905 ) ) ;
#11831=CARTESIAN_POINT ( 'NONE',  ( -2.293366432827344421E-15, -12.48450537969573659, -172.9062500020484379 ) ) ;
#11832=CARTESIAN_POINT ( 'NONE',  ( -9.999999999999998224, 1.224646799147353059E-15, -169.6250000040967905 ) ) ;
#11835=CARTESIAN_POINT ( 'NONE',  ( -10.81189881249999729, 1.324075727343319199E-15, -42.59375000204837391 ) ) ;
#11837=CARTESIAN_POINT ( 'NONE',  ( -10.81189881249999729, 1.324075727343319199E-15, -2.281250002048373915 ) ) ;
#11839=CARTESIAN_POINT ( 'NONE',  ( -10.00000000000000000, -5.773502691896252870, -165.0000000040967905 ) ) ;
#11841=CARTESIAN_POINT ( 'NONE',  ( -9.999999999999998224, 5.773502691896259087, -86.87499999999998579 ) ) ;
#11843=CARTESIAN_POINT ( 'NONE',  ( -5.000000000000003553, -8.660254037844383745, -103.3750000040967763 ) ) ;
#11844=CARTESIAN_POINT ( 'NONE',  ( -2.121150477449813534E-15, -11.54700538379251284, -149.7500000040968189 ) ) ;
#11847=CARTESIAN_POINT ( 'NONE',  ( -5.405949406249996869, 9.363379034771805109, -101.5312500020483952 ) ) ;
#11848=ORIENTED_EDGE ( 'NONE', *, *, #25689, .F. ) ;
#11849=AXIS2_PLACEMENT_3D ( 'NONE', #15685, #35574, #31920 ) ;
#11850=EDGE_CURVE ( 'NONE', #13534, #38098, #39829, .T. ) ;
#11852=CARTESIAN_POINT ( 'NONE',  ( 7.070501591499376803E-16, 11.54700538379251284, -29.00000000409674783 ) ) ;
#11853=CARTESIAN_POINT ( 'NONE',  ( -10.81189881249999729, 1.324075727343319199E-15, -155.2812500020484094 ) ) ;
#11855=VERTEX_POINT ( 'NONE', #23542 ) ;
#11856=CARTESIAN_POINT ( 'NONE',  ( 4.999999999999992006, -8.660254037844389075, -27.74999999999996803 ) ) ;
#11858=CARTESIAN_POINT ( 'NONE',  ( 5.405949406249999534, 9.363379034771803333, -29.78125000204837036 ) ) ;
#11859=CARTESIAN_POINT ( 'NONE',  ( 5.000000000000000000, 8.660254037844385522, -165.2500000000000000 ) ) ;
#11860=( BOUNDED_CURVE ( )  B_SPLINE_CURVE ( 2, ( #41530, #2689, #9158, #38298, #18440, #15822, #28816 ),
 .UNSPECIFIED., .F., .F. ) 
 B_SPLINE_CURVE_WITH_KNOTS ( ( 3, 2, 2, 3 ),
 ( 0.5746268656716420065, 0.5758706467661693917, 0.5771144278606968880, 0.5783582089552241623 ),
 .UNSPECIFIED. ) 
 CURVE ( )  GEOMETRIC_REPRESENTATION_ITEM ( )  RATIONAL_B_SPLINE_CURVE ( ( 0.9999999999999761302, 0.8660254037844625774, 1.000000000000000000, 0.8660254037844387076, 1.000000000000000000, 0.8660254037844028474, 1.000000000000035971 ) ) 
 REPRESENTATION_ITEM ( '' )  );
#11863=CARTESIAN_POINT ( 'NONE',  ( -10.81189881249999907, -6.242252689847864744, -123.6562500020484094 ) ) ;
#11864=CARTESIAN_POINT ( 'NONE',  ( -4.265126633838427495, 9.090591124651073329, 7.031793886498073594E-15 ) ) ;
#11866=ORIENTED_EDGE ( 'NONE', *, *, #7750, .T. ) ;
#11867=CARTESIAN_POINT ( 'NONE',  ( 5.405949406249992428, -9.363379034771808662, -64.78125000204838102 ) ) ;
#11869=CARTESIAN_POINT ( 'NONE',  ( 10.81189881249999551, -6.242252689847874514, -107.9687500020483810 ) ) ;
#11871=VERTEX_POINT ( 'NONE', #17035 ) ;
#11872=ORIENTED_EDGE ( 'NONE', *, *, #16038, .F. ) ;
#11873=CARTESIAN_POINT ( 'NONE',  ( -10.00000000000038547, 5.773502691896036154, -181.7500000040967905 ) ) ;
#11874=CARTESIAN_POINT ( 'NONE',  ( -2.121150477449813534E-15, -11.54700538379251284, -183.8750000000000000 ) ) ;
#11875=CARTESIAN_POINT ( 'NONE',  ( -5.405949406250003975, -9.363379034771801557, -157.8437500020483810 ) ) ;
#11877=CARTESIAN_POINT ( 'NONE',  ( -10.81189881249999729, 1.324075727343319199E-15, -5.093750002048369474 ) ) ;
#11878=CARTESIAN_POINT ( 'NONE',  ( 10.81189881249999551, -6.242252689847874514, -136.4687500020483810 ) ) ;
#11879=CARTESIAN_POINT ( 'NONE',  ( -10.81189881249999907, -6.242252689847864744, -98.15625000204839523 ) ) ;
#11883=CARTESIAN_POINT ( 'NONE',  ( -5.405949406249996869, 9.363379034771805109, 0.6562499979516356330 ) ) ;
#11885=CARTESIAN_POINT ( 'NONE',  ( 10.81189881249999551, -6.242252689847874514, -195.1562500020484094 ) ) ;
#11886=CARTESIAN_POINT ( 'NONE',  ( -5.000000000000003553, -8.660254037844383745, -5.875000004096770034 ) ) ;
#11890=CARTESIAN_POINT ( 'NONE',  ( 10.81189881249999729, 0.000000000000000000, -64.34375000204836681 ) ) ;
#11891=CARTESIAN_POINT ( 'NONE',  ( 10.81189881249999907, 6.242252689847868297, -59.71875000204838102 ) ) ;
#11893=CARTESIAN_POINT ( 'NONE',  ( -10.81189881249999729, 6.242252689847871849, -27.90625000204838102 ) ) ;
#11897=CARTESIAN_POINT ( 'NONE',  ( 9.999999999999996447, -5.773502691896262640, -119.1249999999999858 ) ) ;
#11900=CARTESIAN_POINT ( 'NONE',  ( -5.405949406250003975, -9.363379034771801557, -11.03125000204835438 ) ) ;
#11901=VERTEX_POINT ( 'NONE', #30235 ) ;
#11902=( BOUNDED_CURVE ( )  B_SPLINE_CURVE ( 2, ( #3065, #42321, #16191, #42530, #12955, #9739, #7569 ),
 .UNSPECIFIED., .F., .F. ) 
 B_SPLINE_CURVE_WITH_KNOTS ( ( 3, 2, 2, 3 ),
 ( 0.9104477611940301474, 0.9116915422885575326, 0.9129353233830848069, 0.9141791044776121922 ),
 .UNSPECIFIED. ) 
 CURVE ( )  GEOMETRIC_REPRESENTATION_ITEM ( )  RATIONAL_B_SPLINE_CURVE ( ( 0.9999999999999641398, 0.8660254037844745678, 1.000000000000000000, 0.8660254037844387076, 1.000000000000000000, 0.8660254037844148378, 1.000000000000023981 ) ) 
 REPRESENTATION_ITEM ( '' )  );
#11907=CARTESIAN_POINT ( 'NONE',  ( -2.121150477449813534E-15, -11.54700538379251284, -23.75000000409677270 ) ) ;
#11908=CARTESIAN_POINT ( 'NONE',  ( 9.999999999999998224, 0.000000000000000000, -93.49999999999998579 ) ) ;
#11911=FACE_OUTER_BOUND ( 'NONE', #14278, .T. ) ;
#11912=CARTESIAN_POINT ( 'NONE',  ( -5.405949406250003975, -9.363379034771801557, -144.5312500020483810 ) ) ;
#11913=CARTESIAN_POINT ( 'NONE',  ( 10.81189881249999907, 6.242252689847868297, -127.2187500020483668 ) ) ;
#11916=LINE ( 'NONE', #18830, #1796 ) ;
#11917=ORIENTED_EDGE ( 'NONE', *, *, #353, .T. ) ;
#11919=ORIENTED_EDGE ( 'NONE', *, *, #32567, .F. ) ;
#11920=EDGE_CURVE ( 'NONE', #11855, #31902, #26851, .T. ) ;
#11921=ORIENTED_EDGE ( 'NONE', *, *, #38642, .T. ) ;
#11922=EDGE_CURVE ( 'NONE', #34185, #22125, #30449, .T. ) ;
#11923=CARTESIAN_POINT ( 'NONE',  ( -5.000000000000003553, -8.660254037844383745, -7.375000004096743389 ) ) ;
#11924=CARTESIAN_POINT ( 'NONE',  ( -5.405949406250003975, -9.363379034771801557, -181.8437500020483810 ) ) ;
#11925=CARTESIAN_POINT ( 'NONE',  ( -5.405949406250003975, -9.363379034771801557, -34.84375000204836681 ) ) ;
#11926=DIRECTION ( 'NONE',  ( -0.000000000000000000, -0.000000000000000000, 1.000000000000000000 ) ) ;
#11927=CARTESIAN_POINT ( 'NONE',  ( 10.81189881249999729, 0.000000000000000000, -166.3437500020484094 ) ) ;
#11928=CARTESIAN_POINT ( 'NONE',  ( -10.81189881249999907, -6.242252689847864744, -151.9687500020484094 ) ) ;
#11929=DIRECTION ( 'NONE',  ( -0.000000000000000000, -0.000000000000000000, 1.000000000000000000 ) ) ;
#11933=CARTESIAN_POINT ( 'NONE',  ( 7.070501591499376803E-16, 11.54700538379251284, -135.1250000000000000 ) ) ;
#11934=CARTESIAN_POINT ( 'NONE',  ( 7.070501591499376803E-16, 11.54700538379251284, -169.6250000000000000 ) ) ;
#11936=CARTESIAN_POINT ( 'NONE',  ( -5.405949406249996869, 9.363379034771805109, -78.84375000204838102 ) ) ;
#11938=CARTESIAN_POINT ( 'NONE',  ( -10.81189881249999907, -6.242252689847864744, -59.15625000204838813 ) ) ;
#11941=EDGE_CURVE ( 'NONE', #31963, #20180, #25883, .T. ) ;
#11942=CARTESIAN_POINT ( 'NONE',  ( 7.644554776091147741E-16, 12.48450537969573659, -113.6562500020483952 ) ) ;
#11943=CARTESIAN_POINT ( 'NONE',  ( 10.81189881249999729, 0.000000000000000000, -148.5312500020483810 ) ) ;
#11944=CARTESIAN_POINT ( 'NONE',  ( -10.00000000000102496, 5.773502691895664007, -15.25000000409674250 ) ) ;
#11946=CARTESIAN_POINT ( 'NONE',  ( -9.999999999999998224, 1.224646799147353059E-15, -120.1250000040967905 ) ) ;
#11948=VERTEX_POINT ( 'NONE', #4107 ) ;
#11951=LINE ( 'NONE', #36842, #9823 ) ;
#11952=CARTESIAN_POINT ( 'NONE',  ( -10.81189881249999907, -6.242252689847864744, -183.6562500020483810 ) ) ;
#11953=ORIENTED_EDGE ( 'NONE', *, *, #39430, .T. ) ;
#11955=CARTESIAN_POINT ( 'NONE',  ( 10.00000000000000000, 5.773502691896255534, -51.75000000409676204 ) ) ;
#11960=CARTESIAN_POINT ( 'NONE',  ( -5.000000000000003553, -8.660254037844383745, -148.3750000040967905 ) ) ;
#11961=CARTESIAN_POINT ( 'NONE',  ( -5.405949406250003975, -9.363379034771801557, -168.5312500020484094 ) ) ;
#11962=CARTESIAN_POINT ( 'NONE',  ( 7.070501591499376803E-16, 11.54700538379251284, -2.000000004096753159 ) ) ;
#11963=CARTESIAN_POINT ( 'NONE',  ( 4.999999999999992006, -8.660254037844389075, -34.12500000409676915 ) ) ;
#11967=CARTESIAN_POINT ( 'NONE',  ( 5.405949406249992428, -9.363379034771808662, -79.78125000204838102 ) ) ;
#11968=ORIENTED_EDGE ( 'NONE', *, *, #15619, .T. ) ;
#11969=EDGE_CURVE ( 'NONE', #5733, #41318, #36811, .T. ) ;
#11970=CARTESIAN_POINT ( 'NONE',  ( 9.999999999999998224, 0.000000000000000000, -188.3750000040967905 ) ) ;
#11971=ORIENTED_EDGE ( 'NONE', *, *, #34132, .F. ) ;
#11973=ORIENTED_EDGE ( 'NONE', *, *, #24630, .T. ) ;
#11975=CARTESIAN_POINT ( 'NONE',  ( -5.405949406249996869, 9.363379034771805109, -30.84375000204836326 ) ) ;
#11977=CARTESIAN_POINT ( 'NONE',  ( 10.81189881249999551, -6.242252689847874514, -4.656250002048353487 ) ) ;
#11978=CARTESIAN_POINT ( 'NONE',  ( -10.81189881249999729, 6.242252689847871849, -54.71875000204838102 ) ) ;
#11979=ORIENTED_EDGE ( 'NONE', *, *, #12507, .F. ) ;
#11980=EDGE_CURVE ( 'NONE', #33268, #8658, #35390, .T. ) ;
#11983=CARTESIAN_POINT ( 'NONE',  ( -5.405949406249996869, 9.363379034771805109, -194.3437500020484094 ) ) ;
#11984=CARTESIAN_POINT ( 'NONE',  ( 10.81189881249999729, 0.000000000000000000, -178.3437500020483810 ) ) ;
#11988=LINE ( 'NONE', #12404, #19188 ) ;
#11991=CARTESIAN_POINT ( 'NONE',  ( -5.405949406249996869, 9.363379034771805109, -105.8437500020483810 ) ) ;
#11993=CARTESIAN_POINT ( 'NONE',  ( -10.81189881249999729, 1.324075727343319199E-15, -83.28125000204838102 ) ) ;
#11994=CARTESIAN_POINT ( 'NONE',  ( -2.293366432827344421E-15, -12.48450537969573659, -90.21875000204838102 ) ) ;
#11996=CARTESIAN_POINT ( 'NONE',  ( -9.999999999999998224, 5.773502691896259087, -145.7500000040967905 ) ) ;
#11999=VERTEX_POINT ( 'NONE', #38187 ) ;
#12002=CARTESIAN_POINT ( 'NONE',  ( 9.999999999999998224, 0.000000000000000000, -96.49999999999998579 ) ) ;
#12003=DIRECTION ( 'NONE',  ( -0.000000000000000000, -0.000000000000000000, 1.000000000000000000 ) ) ;
#12006=CARTESIAN_POINT ( 'NONE',  ( -2.121150477449813534E-15, -11.54700538379251284, -63.87499999999999289 ) ) ;
#12008=CARTESIAN_POINT ( 'NONE',  ( -10.00000000000000000, -5.773502691896251982, -72.00000000409674783 ) ) ;
#12009=CARTESIAN_POINT ( 'NONE',  ( 10.00000000000102318, -5.773502691895667560, -11.50000000409674072 ) ) ;
#12011=CARTESIAN_POINT ( 'NONE',  ( 10.81189881249999729, 0.000000000000000000, -76.53125000204838102 ) ) ;
#12015=ORIENTED_EDGE ( 'NONE', *, *, #3158, .T. ) ;
#12016=CARTESIAN_POINT ( 'NONE',  ( 10.81189881249999729, 0.000000000000000000, -195.0312500020484094 ) ) ;
#12018=CARTESIAN_POINT ( 'NONE',  ( 5.405949406249999534, 9.363379034771803333, -5.593750002048370362 ) ) ;
#12020=CARTESIAN_POINT ( 'NONE',  ( -10.81189881249999907, -6.242252689847864744, -142.9687500020484094 ) ) ;
#12022=CARTESIAN_POINT ( 'NONE',  ( 4.999999999999992006, -8.660254037844389075, -173.2500000000000284 ) ) ;
#12023=( BOUNDED_CURVE ( )  B_SPLINE_CURVE ( 2, ( #16651, #12986, #15805, #13411, #42562, #42142, #29211 ),
 .UNSPECIFIED., .F., .F. ) 
 B_SPLINE_CURVE_WITH_KNOTS ( ( 3, 2, 2, 3 ),
 ( 0.7089552238805972850, 0.7101990049751245593, 0.7114427860696519446, 0.7126865671641793298 ),
 .UNSPECIFIED. ) 
 CURVE ( )  GEOMETRIC_REPRESENTATION_ITEM ( )  RATIONAL_B_SPLINE_CURVE ( ( 0.9999999999999761302, 0.8660254037844625774, 1.000000000000000000, 0.8660254037844387076, 1.000000000000000000, 0.8660254037844148378, 1.000000000000023981 ) ) 
 REPRESENTATION_ITEM ( '' )  );
#12024=CARTESIAN_POINT ( 'NONE',  ( 10.00000000000000000, 5.773502691896255534, -175.8750000000000000 ) ) ;
#12026=CARTESIAN_POINT ( 'NONE',  ( 10.81189881249999907, 6.242252689847868297, -103.4062500020483952 ) ) ;
#12027=ORIENTED_EDGE ( 'NONE', *, *, #1670, .F. ) ;
#12028=CYLINDRICAL_SURFACE ( 'NONE', #9004, 9.999999999999998224 ) ;
#12029=VERTEX_POINT ( 'NONE', #21352 ) ;
#12030=ORIENTED_EDGE ( 'NONE', *, *, #24028, .F. ) ;
#12031=CARTESIAN_POINT ( 'NONE',  ( -5.405949406250003975, -9.363379034771801557, -29.03125000204837036 ) ) ;
#12033=CARTESIAN_POINT ( 'NONE',  ( -10.81189881249999907, -6.242252689847864744, -78.46875000204838102 ) ) ;
#12034=CARTESIAN_POINT ( 'NONE',  ( -4.999999999999996447, 8.660254037844387298, -127.8750000040967905 ) ) ;
#12035=CARTESIAN_POINT ( 'NONE',  ( -9.999999999999998224, 1.224646799147353059E-15, -180.1250000040968189 ) ) ;
#12036=CARTESIAN_POINT ( 'NONE',  ( 0.000000000000000000, 0.000000000000000000, -200.0000000000000000 ) ) ;
#12038=CARTESIAN_POINT ( 'NONE',  ( -2.121150477449813534E-15, -11.54700538379251284, -10.25000000409676026 ) ) ;
#12040=EDGE_CURVE ( 'NONE', #42590, #25379, #18109, .T. ) ;
#12041=CARTESIAN_POINT ( 'NONE',  ( 10.81189881249999729, 6.242252689847867408, -118.2187500020483810 ) ) ;
#12045=CARTESIAN_POINT ( 'NONE',  ( 10.00000000000000000, 5.773502691896255534, -167.2500000040968189 ) ) ;
#12046=CARTESIAN_POINT ( 'NONE',  ( -10.81189881249999729, 6.242252689847871849, -171.9062500020484094 ) ) ;
#12050=CARTESIAN_POINT ( 'NONE',  ( -5.405949406250003975, -9.363379034771801557, -42.34375000204837391 ) ) ;
#12052=CARTESIAN_POINT ( 'NONE',  ( 10.81189881249999729, 0.000000000000000000, -1.531250002048373249 ) ) ;
#12054=CARTESIAN_POINT ( 'NONE',  ( 9.999999999999998224, 0.000000000000000000, -158.3750000040967905 ) ) ;
#12056=CARTESIAN_POINT ( 'NONE',  ( 7.070501591499377789E-16, 11.54700538379251284, -93.12500000000000000 ) ) ;
#12058=CARTESIAN_POINT ( 'NONE',  ( -4.999999999999996447, 8.660254037844387298, -105.3750000040967763 ) ) ;
#12061=CARTESIAN_POINT ( 'NONE',  ( 5.405949406249999534, 9.363379034771803333, -100.2812500020483952 ) ) ;
#12062=ADVANCED_FACE ( 'NONE', ( #31304 ), #25466, .T. ) ;
#12064=AXIS2_PLACEMENT_3D ( 'NONE', #13530, #33423, #20654 ) ;
#12067=CARTESIAN_POINT ( 'NONE',  ( 10.81189881249999551, -6.242252689847874514, -156.1562500020484094 ) ) ;
#12069=EDGE_LOOP ( 'NONE', ( #40888, #39155, #10799, #30781 ) ) ;
#12070=CARTESIAN_POINT ( 'NONE',  ( 7.070501591499377789E-16, 11.54700538379251284, -15.12499999999997691 ) ) ;
#12071=CARTESIAN_POINT ( 'NONE',  ( 10.81189881249999551, -6.242252689847874514, -30.15625000204836326 ) ) ;
#12072=CARTESIAN_POINT ( 'NONE',  ( -9.999999999999998224, 5.773502691896259087, -155.8749999999999716 ) ) ;
#12074=CARTESIAN_POINT ( 'NONE',  ( -5.000000000000003553, -8.660254037844383745, -196.0000000000000000 ) ) ;
#12075=CARTESIAN_POINT ( 'NONE',  ( -10.81189881249999729, 1.324075727343319199E-15, -123.7812500020483952 ) ) ;
#12077=CARTESIAN_POINT ( 'NONE',  ( 4.999999999999992006, -8.660254037844389075, -21.74999999999996447 ) ) ;
#12079=VECTOR ( 'NONE', #28965, 1000.000000000000000 ) ;
#12081=CARTESIAN_POINT ( 'NONE',  ( -10.81189881249999907, -6.242252689847864744, -54.65625000204838102 ) ) ;
#12083=CARTESIAN_POINT ( 'NONE',  ( -10.81189881249999729, 1.324075727343319199E-15, -113.0937500020483810 ) ) ;
#12085=ORIENTED_EDGE ( 'NONE', *, *, #26407, .T. ) ;
#12088=LINE ( 'NONE', #1977, #820 ) ;
#12089=CARTESIAN_POINT ( 'NONE',  ( 7.644554776091147741E-16, 12.48450537969573659, -153.9687500020484094 ) ) ;
#12090=ADVANCED_FACE ( 'NONE', ( #1736 ), #5814, .T. ) ;
#12092=CARTESIAN_POINT ( 'NONE',  ( -5.405949406249996869, 9.363379034771805109, -5.343750002048369474 ) ) ;
#12093=CARTESIAN_POINT ( 'NONE',  ( -5.405949406249996869, 9.363379034771805109, -138.8437500020484094 ) ) ;
#12095=CARTESIAN_POINT ( 'NONE',  ( 5.000000000000000000, 8.660254037844385522, -187.7500000000000000 ) ) ;
#12097=CARTESIAN_POINT ( 'NONE',  ( 10.81189881249999907, 6.242252689847868297, -2.718750002048360592 ) ) ;
#12099=CARTESIAN_POINT ( 'NONE',  ( 7.644554776091147741E-16, 12.48450537969573659, -196.1562500020484094 ) ) ;
#12102=CARTESIAN_POINT ( 'NONE',  ( -5.405949406249996869, 9.363379034771805109, -68.34375000204836681 ) ) ;
#12103=CARTESIAN_POINT ( 'NONE',  ( -2.293366432827344421E-15, -12.48450537969573659, -57.21875000204835970 ) ) ;
#12105=CARTESIAN_POINT ( 'NONE',  ( -10.81189881249999729, 6.242252689847871849, -29.40625000204835615 ) ) ;
#12107=CARTESIAN_POINT ( 'NONE',  ( -9.999999999999998224, 1.224646799147353059E-15, -136.2499999999999716 ) ) ;
#12109=CARTESIAN_POINT ( 'NONE',  ( -2.121150477449813534E-15, -11.54700538379251284, -116.3749999999999858 ) ) ;
#12111=CARTESIAN_POINT ( 'NONE',  ( 9.999999999999998224, 0.000000000000000000, -200.0000000000000000 ) ) ;
#12112=VECTOR ( 'NONE', #9547, 1000.000000000000000 ) ;
#12115=CARTESIAN_POINT ( 'NONE',  ( 5.405949406249999534, 9.363379034771803333, -8.781250002048352599 ) ) ;
#12118=LINE ( 'NONE', #38670, #17578 ) ;
#12120=CARTESIAN_POINT ( 'NONE',  ( -9.999999999999998224, 1.224646799147353059E-15, -128.7499999999999716 ) ) ;
#12122=CARTESIAN_POINT ( 'NONE',  ( -5.000000000000003553, -8.660254037844383745, -44.49999999999998579 ) ) ;
#12123=CARTESIAN_POINT ( 'NONE',  ( -9.999999999999998224, 5.773502691896259087, -22.75000000409677270 ) ) ;
#12125=CARTESIAN_POINT ( 'NONE',  ( 4.999999999999992006, -8.660254037844389075, -141.7500000000000000 ) ) ;
#12127=FACE_OUTER_BOUND ( 'NONE', #34129, .T. ) ;
#12128=CARTESIAN_POINT ( 'NONE',  ( -10.81189881249999729, 1.324075727343319199E-15, -147.7812500020483810 ) ) ;
#12129=CARTESIAN_POINT ( 'NONE',  ( 10.81189881249999729, 0.000000000000000000, -150.0312500020483810 ) ) ;
#12130=CARTESIAN_POINT ( 'NONE',  ( 9.999999999999998224, 0.000000000000000000, -51.49999999999996447 ) ) ;
#12131=FACE_OUTER_BOUND ( 'NONE', #31522, .T. ) ;
#12132=ORIENTED_EDGE ( 'NONE', *, *, #22674, .T. ) ;
#12134=ORIENTED_EDGE ( 'NONE', *, *, #19400, .F. ) ;
#12135=CARTESIAN_POINT ( 'NONE',  ( 10.00000000000205347, -5.773502691895071592, -7.000000004096692763 ) ) ;
#12136=CARTESIAN_POINT ( 'NONE',  ( 5.405949406249999534, 9.363379034771803333, -178.0937500020484094 ) ) ;
#12137=CARTESIAN_POINT ( 'NONE',  ( 10.81189881249999551, -6.242252689847874514, -28.46875000204837036 ) ) ;
#12138=CARTESIAN_POINT ( 'NONE',  ( 9.999999999999998224, 0.000000000000000000, -110.3750000040967763 ) ) ;
#12139=CARTESIAN_POINT ( 'NONE',  ( 7.644554776091147741E-16, 12.48450537969573659, -167.4687500020483526 ) ) ;
#12140=CARTESIAN_POINT ( 'NONE',  ( -10.81189881249999907, -6.242252689847864744, -156.4687500020484379 ) ) ;
#12141=DIRECTION ( 'NONE',  ( -0.000000000000000000, -0.000000000000000000, 1.000000000000000000 ) ) ;
#12145=( BOUNDED_CURVE ( )  B_SPLINE_CURVE ( 2, ( #33826, #6849, #20855, #16969, #17181, #30379, #811 ),
 .UNSPECIFIED., .F., .F. ) 
 B_SPLINE_CURVE_WITH_KNOTS ( ( 3, 2, 2, 3 ),
 ( 0.4477611940298508730, 0.4490049751243782028, 0.4502487562189055881, 0.4514925373134329734 ),
 .UNSPECIFIED. ) 
 CURVE ( )  GEOMETRIC_REPRESENTATION_ITEM ( )  RATIONAL_B_SPLINE_CURVE ( ( 0.9999999999999880096, 0.8660254037844506980, 1.000000000000000000, 0.8660254037844387076, 1.000000000000000000, 0.8660254037844267172, 1.000000000000011990 ) ) 
 REPRESENTATION_ITEM ( '' )  );
#12146=CARTESIAN_POINT ( 'NONE',  ( -9.999999999999998224, 1.224646799147353059E-15, -70.24999999999998579 ) ) ;
#12148=CARTESIAN_POINT ( 'NONE',  ( 10.81189881249999729, 0.000000000000000000, -77.84375000204838102 ) ) ;
#12150=CARTESIAN_POINT ( 'NONE',  ( 5.405949406249999534, 9.363379034771803333, -50.78125000204835970 ) ) ;
#12153=CARTESIAN_POINT ( 'NONE',  ( 10.00000000000000000, 5.773502691896255534, -133.8750000000000000 ) ) ;
#12154=CARTESIAN_POINT ( 'NONE',  ( -10.81189881249999729, 1.324075727343319199E-15, -149.2812500020483810 ) ) ;
#12155=CARTESIAN_POINT ( 'NONE',  ( -2.121150477449813534E-15, -11.54700538379251284, -29.37499999999994671 ) ) ;
#12157=CARTESIAN_POINT ( 'NONE',  ( 5.000000000000000000, 8.660254037844385522, -122.1250000040967905 ) ) ;
#12159=VERTEX_POINT ( 'NONE', #11625 ) ;
#12164=CARTESIAN_POINT ( 'NONE',  ( -5.405949406250003975, -9.363379034771801557, -182.0312500020483810 ) ) ;
#12165=CARTESIAN_POINT ( 'NONE',  ( -4.999999999999996447, 8.660254037844387298, -46.87500000409677625 ) ) ;
#12166=EDGE_CURVE ( 'NONE', #26513, #32487, #31285, .T. ) ;
#12168=EDGE_CURVE ( 'NONE', #11337, #15716, #10329, .T. ) ;
#12170=CARTESIAN_POINT ( 'NONE',  ( 9.999999999999998224, 0.000000000000000000, -23.37500000409675849 ) ) ;
#12171=CARTESIAN_POINT ( 'NONE',  ( -10.81189881249999729, 6.242252689847871849, -168.9062500020483810 ) ) ;
#12172=CARTESIAN_POINT ( 'NONE',  ( 0.000000000000000000, 0.000000000000000000, -200.0000000000000000 ) ) ;
#12173=CYLINDRICAL_SURFACE ( 'NONE', #15106, 9.999999999999998224 ) ;
#12174=VERTEX_POINT ( 'NONE', #41410 ) ;
#12175=CARTESIAN_POINT ( 'NONE',  ( 0.000000000000000000, 0.000000000000000000, -200.0000000000000000 ) ) ;
#12176=CARTESIAN_POINT ( 'NONE',  ( 9.999999999999998224, 0.000000000000000000, -123.8750000040967905 ) ) ;
#12177=CARTESIAN_POINT ( 'NONE',  ( -5.000000000000003553, -8.660254037844383745, -71.49999999999998579 ) ) ;
#12178=CARTESIAN_POINT ( 'NONE',  ( 5.405949406249999534, 9.363379034771803333, -74.78125000204838102 ) ) ;
#12179=ORIENTED_EDGE ( 'NONE', *, *, #21511, .F. ) ;
#12181=CARTESIAN_POINT ( 'NONE',  ( 10.00000000000025402, -5.773502691896113426, -140.1250000000000000 ) ) ;
#12182=VERTEX_POINT ( 'NONE', #25045 ) ;
#12184=CARTESIAN_POINT ( 'NONE',  ( -10.81189881249999729, -6.242252689847864744, -31.96875000204835970 ) ) ;
#12185=CARTESIAN_POINT ( 'NONE',  ( -9.999999999998969713, -5.773502691896847949, -53.62499999999995737 ) ) ;
#12186=CARTESIAN_POINT ( 'NONE',  ( 10.81189881249999907, 6.242252689847868297, -2.906250002048345937 ) ) ;
#12187=CARTESIAN_POINT ( 'NONE',  ( -10.81189881249999729, 1.324075727343319199E-15, -59.09375000204835970 ) ) ;
#12188=ORIENTED_EDGE ( 'NONE', *, *, #11814, .F. ) ;
#12189=LINE ( 'NONE', #2083, #34636 ) ;
#12191=CARTESIAN_POINT ( 'NONE',  ( 10.81189881249999729, 6.242252689847867408, -190.2187500020484094 ) ) ;
#12192=CARTESIAN_POINT ( 'NONE',  ( -5.405949406249996869, 9.363379034771805109, -176.3437500020483810 ) ) ;
#12195=LINE ( 'NONE', #28419, #30896 ) ;
#12196=CARTESIAN_POINT ( 'NONE',  ( -9.999999999999998224, 1.224646799147353059E-15, -102.1250000040967905 ) ) ;
#12198=CARTESIAN_POINT ( 'NONE',  ( -5.405949406250003975, -9.363379034771801557, -102.3437500020483810 ) ) ;
#12199=CARTESIAN_POINT ( 'NONE',  ( 4.999999999999992006, -8.660254037844389075, -84.74999999999997158 ) ) ;
#12200=CARTESIAN_POINT ( 'NONE',  ( -2.293366432827344421E-15, -12.48450537969573659, -75.40625000204838102 ) ) ;
#12201=CARTESIAN_POINT ( 'NONE',  ( -10.81189881249999729, 6.242252689847871849, -92.21875000204839523 ) ) ;
#12203=CARTESIAN_POINT ( 'NONE',  ( -10.00000000000000000, -5.773502691896251982, -150.0000000040967905 ) ) ;
#12205=ORIENTED_EDGE ( 'NONE', *, *, #24444, .T. ) ;
#12208=CARTESIAN_POINT ( 'NONE',  ( 0.000000000000000000, 0.000000000000000000, -200.0000000000000000 ) ) ;
#12209=CARTESIAN_POINT ( 'NONE',  ( -2.121150477449813534E-15, -11.54700538379251284, -38.37499999999995737 ) ) ;
#12211=ORIENTED_EDGE ( 'NONE', *, *, #37433, .F. ) ;
#12212=CARTESIAN_POINT ( 'NONE',  ( 4.999999999999992006, -8.660254037844389075, -62.24999999999997158 ) ) ;
#12214=CARTESIAN_POINT ( 'NONE',  ( 10.00000000000000000, 5.773502691896255534, -72.75000000409674783 ) ) ;
#12216=CARTESIAN_POINT ( 'NONE',  ( -9.999999999999998224, 1.224646799147353059E-15, -151.2500000000000000 ) ) ;
#12219=CARTESIAN_POINT ( 'NONE',  ( -5.405949406249996869, 9.363379034771805109, -70.03125000204838102 ) ) ;
#12220=EDGE_CURVE ( 'NONE', #40396, #5733, #31033, .T. ) ;
#12222=CARTESIAN_POINT ( 'NONE',  ( -9.999999999999998224, 1.224646799147353059E-15, -26.74999999999996803 ) ) ;
#12224=DIRECTION ( 'NONE',  ( 1.000000000000000000, 0.000000000000000000, 0.000000000000000000 ) ) ;
#12225=CARTESIAN_POINT ( 'NONE',  ( -10.81189881249999907, -6.242252689847864744, -195.6562500020484094 ) ) ;
#12227=CARTESIAN_POINT ( 'NONE',  ( 10.81189881249999551, -6.242252689847874514, -4.468750002048368586 ) ) ;
#12228=LINE ( 'NONE', #26050, #34496 ) ;
#12229=( BOUNDED_CURVE ( )  B_SPLINE_CURVE ( 2, ( #20577, #7214, #11502, #30537, #20366, #17542, #33766 ),
 .UNSPECIFIED., .F., .F. ) 
 B_SPLINE_CURVE_WITH_KNOTS ( ( 3, 2, 2, 3 ),
 ( 0.8134328358208956500, 0.8146766169154230353, 0.8159203980099504205, 0.8171641791044778058 ),
 .UNSPECIFIED. ) 
 CURVE ( )  GEOMETRIC_REPRESENTATION_ITEM ( )  RATIONAL_B_SPLINE_CURVE ( ( 0.9999999999999880096, 0.8660254037844506980, 1.000000000000000000, 0.8660254037844387076, 1.000000000000000000, 0.8660254037844148378, 1.000000000000023981 ) ) 
 REPRESENTATION_ITEM ( '' )  );
#12230=CARTESIAN_POINT ( 'NONE',  ( -5.000000000000003553, -8.660254037844383745, -181.0000000000000000 ) ) ;
#12232=CARTESIAN_POINT ( 'NONE',  ( -10.00000000000025580, 5.773502691896109873, -159.2500000040968189 ) ) ;
#12233=CARTESIAN_POINT ( 'NONE',  ( -4.999999999999996447, 8.660254037844387298, -174.0000000000000284 ) ) ;
#12234=CARTESIAN_POINT ( 'NONE',  ( 10.81189881249999551, -6.242252689847874514, -102.1562500020483952 ) ) ;
#12235=ORIENTED_EDGE ( 'NONE', *, *, #2805, .F. ) ;
#12238=ORIENTED_EDGE ( 'NONE', *, *, #17223, .F. ) ;
#12239=CARTESIAN_POINT ( 'NONE',  ( 10.81189881249999551, -6.242252689847874514, -30.15625000204836326 ) ) ;
#12242=CARTESIAN_POINT ( 'NONE',  ( 5.405949406249992428, -9.363379034771808662, -81.09375000204838102 ) ) ;
#12244=AXIS2_PLACEMENT_3D ( 'NONE', #7807, #14239, #14462 ) ;
#12245=VECTOR ( 'NONE', #13395, 1000.000000000000000 ) ;
#12246=CARTESIAN_POINT ( 'NONE',  ( 10.81189881249999551, -6.242252689847874514, -197.9687500020484094 ) ) ;
#12248=DIRECTION ( 'NONE',  ( -0.000000000000000000, -0.000000000000000000, 1.000000000000000000 ) ) ;
#12250=CARTESIAN_POINT ( 'NONE',  ( 9.999999999999996447, -5.773502691896262640, -10.00000000409676026 ) ) ;
#12251=FACE_OUTER_BOUND ( 'NONE', #12069, .T. ) ;
#12252=CARTESIAN_POINT ( 'NONE',  ( -10.81189881249999729, 6.242252689847871849, -129.7187500020483810 ) ) ;
#12253=CARTESIAN_POINT ( 'NONE',  ( -10.81189881249999729, -6.242252689847864744, -114.4687500020483810 ) ) ;
#12256=CARTESIAN_POINT ( 'NONE',  ( -10.00000000000000000, -5.773502691896251982, -174.0000000040967905 ) ) ;
#12257=CARTESIAN_POINT ( 'NONE',  ( 10.81189881249999729, 6.242252689847867408, -167.9062500020484094 ) ) ;
#12260=CARTESIAN_POINT ( 'NONE',  ( -5.405949406249996869, 9.363379034771805109, -42.84375000204837391 ) ) ;
#12262=CARTESIAN_POINT ( 'NONE',  ( 5.405949406249999534, 9.363379034771803333, -2.781250002048374359 ) ) ;
#12266=CARTESIAN_POINT ( 'NONE',  ( -9.999999999999998224, 5.773502691896259087, -91.37499999999998579 ) ) ;
#12268=CARTESIAN_POINT ( 'NONE',  ( -4.999999999999996447, 8.660254037844387298, -100.8750000040967905 ) ) ;
#12271=CARTESIAN_POINT ( 'NONE',  ( 10.81189881249999729, 6.242252689847867408, -92.90625000204839523 ) ) ;
#12272=VERTEX_POINT ( 'NONE', #38824 ) ;
#12273=( BOUNDED_CURVE ( )  B_SPLINE_CURVE ( 2, ( #35743, #33138, #35941, #19739, #15851, #36361, #16063 ),
 .UNSPECIFIED., .F., .F. ) 
 B_SPLINE_CURVE_WITH_KNOTS ( ( 3, 2, 2, 3 ),
 ( 0.1977611940298507898, 0.1990049751243781750, 0.2002487562189055326, 0.2014925373134328901 ),
 .UNSPECIFIED. ) 
 CURVE ( )  GEOMETRIC_REPRESENTATION_ITEM ( )  RATIONAL_B_SPLINE_CURVE ( ( 0.9999999999999940048, 0.8660254037844447028, 1.000000000000000000, 0.8660254037844387076, 1.000000000000000000, 0.8660254037844327124, 1.000000000000005995 ) ) 
 REPRESENTATION_ITEM ( '' )  );
#12276=CARTESIAN_POINT ( 'NONE',  ( -10.81189881249999729, 1.324075727343319199E-15, -158.2812500020484094 ) ) ;
#12278=ORIENTED_EDGE ( 'NONE', *, *, #17483, .F. ) ;
#12279=CARTESIAN_POINT ( 'NONE',  ( 10.00000000000000000, 5.773502691896255534, -13.87499999999997158 ) ) ;
#12280=CARTESIAN_POINT ( 'NONE',  ( 5.405949406249992428, -9.363379034771808662, -24.28125000204836681 ) ) ;
#12281=CARTESIAN_POINT ( 'NONE',  ( 9.999999999999996447, -5.773502691896262640, -150.6250000000000000 ) ) ;
#12284=FACE_OUTER_BOUND ( 'NONE', #16828, .T. ) ;
#12286=CARTESIAN_POINT ( 'NONE',  ( -5.405949406249996869, 9.363379034771805109, -128.5312500020484094 ) ) ;
#12288=ORIENTED_EDGE ( 'NONE', *, *, #13812, .T. ) ;
#12289=CARTESIAN_POINT ( 'NONE',  ( -2.293366432827344421E-15, -12.48450537969573659, -57.40625000204838102 ) ) ;
#12291=CARTESIAN_POINT ( 'NONE',  ( 7.644554776091147741E-16, 12.48450537969573659, -101.4687500020483668 ) ) ;
#12293=VERTEX_POINT ( 'NONE', #19178 ) ;
#12295=CARTESIAN_POINT ( 'NONE',  ( -9.999999999999998224, 1.224646799147353059E-15, -198.1250000040967905 ) ) ;
#12296=CARTESIAN_POINT ( 'NONE',  ( -10.81189881249999729, 1.324075727343319199E-15, -161.0937500020484094 ) ) ;
#12298=CARTESIAN_POINT ( 'NONE',  ( 10.81189881249999907, 6.242252689847868297, -4.218750002048367698 ) ) ;
#12300=CARTESIAN_POINT ( 'NONE',  ( 7.644554776091147741E-16, 12.48450537969573659, -143.4687500020484094 ) ) ;
#12304=CARTESIAN_POINT ( 'NONE',  ( 4.999999999999992006, -8.660254037844389075, -194.6250000040967905 ) ) ;
#12306=CARTESIAN_POINT ( 'NONE',  ( -2.293366432827344421E-15, -12.48450537969573659, -196.9062500020484094 ) ) ;
#12310=CARTESIAN_POINT ( 'NONE',  ( 5.405949406249999534, 9.363379034771803333, -71.59375000204836681 ) ) ;
#12311=CARTESIAN_POINT ( 'NONE',  ( 10.81189881249999729, 0.000000000000000000, -53.84375000204835970 ) ) ;
#12313=CARTESIAN_POINT ( 'NONE',  ( 10.81189881249999551, -6.242252689847874514, -30.15625000204836326 ) ) ;
#12317=CARTESIAN_POINT ( 'NONE',  ( -10.00000000000000000, -5.773502691896251982, -113.6249999999999858 ) ) ;
#12321=CARTESIAN_POINT ( 'NONE',  ( -5.405949406249996869, 9.363379034771805109, -8.531250002048352599 ) ) ;
#12323=CARTESIAN_POINT ( 'NONE',  ( 10.00000000000051159, -5.773502691895965988, -176.1250000000000000 ) ) ;
#12325=CARTESIAN_POINT ( 'NONE',  ( -9.999999999999998224, 1.224646799147353059E-15, -87.12500000409677625 ) ) ;
#12327=CARTESIAN_POINT ( 'NONE',  ( 5.000000000000000000, 8.660254037844385522, -42.24999999999997868 ) ) ;
#12328=CARTESIAN_POINT ( 'NONE',  ( -9.999999999999998224, 5.773502691896259087, -24.25000000409676204 ) ) ;
#12329=CARTESIAN_POINT ( 'NONE',  ( -2.293366432827344421E-15, -12.48450537969573659, -51.40625000204838102 ) ) ;
#12330=CARTESIAN_POINT ( 'NONE',  ( 9.999999999999998224, 0.000000000000000000, -12.87500000409674783 ) ) ;
#12332=DIRECTION ( 'NONE',  ( -0.4999999999999997224, -0.8660254037844388186, -0.000000000000000000 ) ) ;
#12333=CARTESIAN_POINT ( 'NONE',  ( 10.81189881249999551, -6.242252689847874514, -147.1562500020484094 ) ) ;
#12334=CARTESIAN_POINT ( 'NONE',  ( -2.293366432827344421E-15, -12.48450537969573659, -150.4062500020483810 ) ) ;
#12337=ORIENTED_EDGE ( 'NONE', *, *, #41795, .F. ) ;
#12338=ORIENTED_EDGE ( 'NONE', *, *, #31811, .F. ) ;
#12339=ORIENTED_EDGE ( 'NONE', *, *, #34353, .T. ) ;
#12341=CARTESIAN_POINT ( 'NONE',  ( -1.040834085586084257E-14, 20.00000000000000711, 22.49999999999999289 ) ) ;
#12342=CARTESIAN_POINT ( 'NONE',  ( -10.81189881249999729, 6.242252689847871849, -185.2187500020483810 ) ) ;
#12343=CARTESIAN_POINT ( 'NONE',  ( -5.405949406250003975, -9.363379034771801557, -28.84375000204836326 ) ) ;
#12344=FACE_OUTER_BOUND ( 'NONE', #42526, .T. ) ;
#12345=CARTESIAN_POINT ( 'NONE',  ( 5.405949406249999534, 9.363379034771803333, -167.5937500020484094 ) ) ;
#12346=CARTESIAN_POINT ( 'NONE',  ( -2.293366432827344421E-15, -12.48450537969573659, -154.7187500020483810 ) ) ;
#12347=( BOUNDED_CURVE ( )  B_SPLINE_CURVE ( 2, ( #30928, #40825, #1363, #3957, #4165, #1584, #7188 ),
 .UNSPECIFIED., .F., .F. ) 
 B_SPLINE_CURVE_WITH_KNOTS ( ( 3, 2, 2, 3 ),
 ( 0.2611940298507463565, 0.2624378109452737418, 0.2636815920398011270, 0.2649253731343284568 ),
 .UNSPECIFIED. ) 
 CURVE ( )  GEOMETRIC_REPRESENTATION_ITEM ( )  RATIONAL_B_SPLINE_CURVE ( ( 0.9999999999999880096, 0.8660254037844506980, 1.000000000000000000, 0.8660254037844387076, 1.000000000000000000, 0.8660254037844267172, 1.000000000000011990 ) ) 
 REPRESENTATION_ITEM ( '' )  );
#12351=CARTESIAN_POINT ( 'NONE',  ( 7.644554776091147741E-16, 12.48450537969573659, -15.96875000204835615 ) ) ;
#12353=CARTESIAN_POINT ( 'NONE',  ( 10.00000000000051159, -5.773502691895965988, -152.1250000000000000 ) ) ;
#12354=CARTESIAN_POINT ( 'NONE',  ( 9.999999999998969713, 5.773502691896851502, -11.25000000409674072 ) ) ;
#12356=CARTESIAN_POINT ( 'NONE',  ( -10.81189881249999729, 6.242252689847871849, -84.71875000204836681 ) ) ;
#12358=CARTESIAN_POINT ( 'NONE',  ( -5.405949406250003975, -9.363379034771801557, -48.53125000204838813 ) ) ;
#12360=DIRECTION ( 'NONE',  ( 1.000000000000000000, 0.000000000000000000, 0.000000000000000000 ) ) ;
#12362=CARTESIAN_POINT ( 'NONE',  ( -4.999999999999996447, 8.660254037844387298, -138.0000000000000000 ) ) ;
#12363=CARTESIAN_POINT ( 'NONE',  ( 10.81189881249999729, 0.000000000000000000, -142.5312500020483810 ) ) ;
#12364=CARTESIAN_POINT ( 'NONE',  ( -5.000000000000003553, -8.660254037844383745, -29.49999999999997158 ) ) ;
#12366=CARTESIAN_POINT ( 'NONE',  ( 5.000000000000000000, 8.660254037844385522, -123.6250000040967905 ) ) ;
#12372=AXIS2_PLACEMENT_3D ( 'NONE', #28237, #11589, #8168 ) ;
#12374=CARTESIAN_POINT ( 'NONE',  ( 5.405949406249992428, -9.363379034771808662, -169.7812500020484094 ) ) ;
#12375=CARTESIAN_POINT ( 'NONE',  ( -2.121150477449813534E-15, -11.54700538379251284, -46.25000000409676915 ) ) ;
#12376=DIRECTION ( 'NONE',  ( -0.000000000000000000, -0.000000000000000000, 1.000000000000000000 ) ) ;
#12379=CARTESIAN_POINT ( 'NONE',  ( 10.81189881249999551, -6.242252689847874514, -168.1562500020484094 ) ) ;
#12380=CARTESIAN_POINT ( 'NONE',  ( 9.999999999999998224, 0.000000000000000000, -183.8750000040967905 ) ) ;
#12381=CARTESIAN_POINT ( 'NONE',  ( 10.00000000000044764, -5.773502691896004180, -177.6249999999999716 ) ) ;
#12383=CARTESIAN_POINT ( 'NONE',  ( 9.999999999999998224, 0.000000000000000000, -51.87500000409675494 ) ) ;
#12384=( BOUNDED_CURVE ( )  B_SPLINE_CURVE ( 2, ( #22123, #42164, #12177, #12385, #2289, #41952, #15828 ),
 .UNSPECIFIED., .F., .F. ) 
 B_SPLINE_CURVE_WITH_KNOTS ( ( 3, 2, 2, 3 ),
 ( 0.6380597014925374344, 0.6393034825870648197, 0.6405472636815923160, 0.6417910447761195902 ),
 .UNSPECIFIED. ) 
 CURVE ( )  GEOMETRIC_REPRESENTATION_ITEM ( )  RATIONAL_B_SPLINE_CURVE ( ( 0.9999999999999880096, 0.8660254037844506980, 1.000000000000000000, 0.8660254037844387076, 1.000000000000000000, 0.8660254037844148378, 1.000000000000023981 ) ) 
 REPRESENTATION_ITEM ( '' )  );
#12385=CARTESIAN_POINT ( 'NONE',  ( -2.121150477449813534E-15, -11.54700538379251284, -71.37499999999998579 ) ) ;
#12386=CARTESIAN_POINT ( 'NONE',  ( -10.81189881249999729, 6.242252689847871849, -74.40625000204836681 ) ) ;
#12387=EDGE_LOOP ( 'NONE', ( #11540, #31481, #17855, #38948 ) ) ;
#12388=CARTESIAN_POINT ( 'NONE',  ( 4.999999999999992006, -8.660254037844389075, -188.6250000040967905 ) ) ;
#12391=CARTESIAN_POINT ( 'NONE',  ( -5.405949406250003975, -9.363379034771801557, -31.84375000204836681 ) ) ;
#12392=( BOUNDED_CURVE ( )  B_SPLINE_CURVE ( 2, ( #23013, #35761, #19970, #32939, #9833, #29701, #147 ),
 .UNSPECIFIED., .F., .F. ) 
 B_SPLINE_CURVE_WITH_KNOTS ( ( 3, 2, 2, 3 ),
 ( 0.2723880597014926574, 0.2736318407960199872, 0.2748756218905473725, 0.2761194029850747578 ),
 .UNSPECIFIED. ) 
 CURVE ( )  GEOMETRIC_REPRESENTATION_ITEM ( )  RATIONAL_B_SPLINE_CURVE ( ( 0.9999999999999880096, 0.8660254037844506980, 1.000000000000000000, 0.8660254037844387076, 1.000000000000000000, 0.8660254037844267172, 1.000000000000011990 ) ) 
 REPRESENTATION_ITEM ( '' )  );
#12393=CARTESIAN_POINT ( 'NONE',  ( 4.999999999999992006, -8.660254037844389075, -170.6250000040968189 ) ) ;
#12394=CARTESIAN_POINT ( 'NONE',  ( 7.644554776091147741E-16, 12.48450537969573659, -7.156250002048365921 ) ) ;
#12395=CARTESIAN_POINT ( 'NONE',  ( -10.81189881249999729, 1.324075727343319199E-15, -54.59375000204835970 ) ) ;
#12396=ORIENTED_EDGE ( 'NONE', *, *, #31200, .F. ) ;
#12398=ADVANCED_FACE ( 'NONE', ( #39453 ), #28912, .T. ) ;
#12400=CARTESIAN_POINT ( 'NONE',  ( -10.81189881249999729, 1.324075727343319199E-15, -186.5937500020483810 ) ) ;
#12401=CARTESIAN_POINT ( 'NONE',  ( 5.405949406249992428, -9.363379034771808662, -174.0937500020484094 ) ) ;
#12404=CARTESIAN_POINT ( 'NONE',  ( 9.999999999999998224, 0.000000000000000000, -200.0000000000000000 ) ) ;
#12407=CARTESIAN_POINT ( 'NONE',  ( 7.644554776091147741E-16, 12.48450537969573659, -105.9687500020483668 ) ) ;
#12408=CARTESIAN_POINT ( 'NONE',  ( 0.000000000000000000, 0.000000000000000000, -200.0000000000000000 ) ) ;
#12409=CARTESIAN_POINT ( 'NONE',  ( -5.405949406250003975, -9.363379034771801557, -74.03125000204838102 ) ) ;
#12410=CARTESIAN_POINT ( 'NONE',  ( 10.81189881249999551, -6.242252689847874514, -95.96875000204838102 ) ) ;
#12412=CARTESIAN_POINT ( 'NONE',  ( -4.999999999999996447, 8.660254037844387298, -145.8750000040967905 ) ) ;
#12414=ORIENTED_EDGE ( 'NONE', *, *, #30168, .T. ) ;
#12417=CARTESIAN_POINT ( 'NONE',  ( 10.81189881249999551, -6.242252689847874514, -195.1562500020484379 ) ) ;
#12418=FACE_OUTER_BOUND ( 'NONE', #40832, .T. ) ;
#12420=ORIENTED_EDGE ( 'NONE', *, *, #24247, .T. ) ;
#12421=CARTESIAN_POINT ( 'NONE',  ( -9.999999999999998224, 5.773502691896259087, -65.87499999999998579 ) ) ;
#12423=CARTESIAN_POINT ( 'NONE',  ( 9.999999999999996447, -5.773502691896262640, -71.50000000409676204 ) ) ;
#12427=CARTESIAN_POINT ( 'NONE',  ( 10.81189881249999729, 6.242252689847867408, -68.90625000204840944 ) ) ;
#12430=CARTESIAN_POINT ( 'NONE',  ( -10.00000000000051337, 5.773502691895962435, -46.75000000409676915 ) ) ;
#12431=CARTESIAN_POINT ( 'NONE',  ( 5.405949406249992428, -9.363379034771808662, -195.2812500020484094 ) ) ;
#12433=CARTESIAN_POINT ( 'NONE',  ( -10.81189881249999729, 1.324075727343319199E-15, -3.593750002048368142 ) ) ;
#12434=CARTESIAN_POINT ( 'NONE',  ( 5.000000000000000000, 8.660254037844385522, -140.1250000040967905 ) ) ;
#12435=VECTOR ( 'NONE', #3531, 1000.000000000000000 ) ;
#12436=CARTESIAN_POINT ( 'NONE',  ( -10.00000000000025757, -5.773502691896102768, -181.1250000000000000 ) ) ;
#12437=CARTESIAN_POINT ( 'NONE',  ( -5.000000000000003553, -8.660254037844383745, -137.5000000000000000 ) ) ;
#12438=CARTESIAN_POINT ( 'NONE',  ( -9.999999999999998224, 5.773502691896259087, -173.8749999999999716 ) ) ;
#12439=LINE ( 'NONE', #16303, #32433 ) ;
#12440=CARTESIAN_POINT ( 'NONE',  ( -10.81189881249999907, -6.242252689847864744, -99.65625000204839523 ) ) ;
#12443=ORIENTED_EDGE ( 'NONE', *, *, #7820, .T. ) ;
#12445=CARTESIAN_POINT ( 'NONE',  ( 10.81189881249999729, 0.000000000000000000, -31.53125000204837391 ) ) ;
#12447=CARTESIAN_POINT ( 'NONE',  ( -10.81189881249999729, 6.242252689847871849, -78.71875000204838102 ) ) ;
#12449=ADVANCED_FACE ( 'NONE', ( #9469 ), #35810, .T. ) ;
#12451=EDGE_CURVE ( 'NONE', #9613, #40457, #13105, .T. ) ;
#12452=ADVANCED_FACE ( 'NONE', ( #19386 ), #20018, .T. ) ;
#12454=CARTESIAN_POINT ( 'NONE',  ( 9.999999999999998224, 0.000000000000000000, -72.87500000409677625 ) ) ;
#12456=CARTESIAN_POINT ( 'NONE',  ( -9.999999999999998224, 1.224646799147353059E-15, -7.625000004096743389 ) ) ;
#12459=CARTESIAN_POINT ( 'NONE',  ( -5.405949406249996869, 9.363379034771805109, -129.8437500020484094 ) ) ;
#12460=CARTESIAN_POINT ( 'NONE',  ( -5.405949406249996869, 9.363379034771805109, -114.8437500020483810 ) ) ;
#12463=CARTESIAN_POINT ( 'NONE',  ( 7.070501591499377789E-16, 11.54700538379251284, -173.0000000040967905 ) ) ;
#12464=DIRECTION ( 'NONE',  ( -0.000000000000000000, -0.000000000000000000, 1.000000000000000000 ) ) ;
#12467=CARTESIAN_POINT ( 'NONE',  ( -5.405949406250003975, -9.363379034771801557, -45.34375000204838102 ) ) ;
#12469=CARTESIAN_POINT ( 'NONE',  ( -2.293366432827344421E-15, -12.48450537969573659, -4.906250002048355263 ) ) ;
#12472=CARTESIAN_POINT ( 'NONE',  ( -9.999999999999998224, 5.773502691896259087, -92.87500000000000000 ) ) ;
#12474=CARTESIAN_POINT ( 'NONE',  ( 10.00000000000000000, 5.773502691896255534, -95.25000000409679046 ) ) ;
#12475=EDGE_CURVE ( 'NONE', #25614, #19247, #3003, .T. ) ;
#12476=( BOUNDED_CURVE ( )  B_SPLINE_CURVE ( 2, ( #22091, #38485, #5700, #41281, #18851, #15800, #21656 ),
 .UNSPECIFIED., .F., .F. ) 
 B_SPLINE_CURVE_WITH_KNOTS ( ( 3, 2, 2, 3 ),
 ( 0.8208955223880598506, 0.8221393034825871249, 0.8233830845771146212, 0.8246268656716420065 ),
 .UNSPECIFIED. ) 
 CURVE ( )  GEOMETRIC_REPRESENTATION_ITEM ( )  RATIONAL_B_SPLINE_CURVE ( ( 0.9999999999999880096, 0.8660254037844506980, 1.000000000000000000, 0.8660254037844387076, 1.000000000000000000, 0.8660254037844148378, 1.000000000000023981 ) ) 
 REPRESENTATION_ITEM ( '' )  );
#12479=CARTESIAN_POINT ( 'NONE',  ( -10.81189881249999729, -6.242252689847864744, -92.15625000204836681 ) ) ;
#12482=CARTESIAN_POINT ( 'NONE',  ( 11.54700538379250396, 20.00000000000000711, 0.000000000000000000 ) ) ;
#12484=ORIENTED_EDGE ( 'NONE', *, *, #8111, .T. ) ;
#12485=ADVANCED_FACE ( 'NONE', ( #16127 ), #32776, .T. ) ;
#12486=CARTESIAN_POINT ( 'NONE',  ( 5.000000000000000000, 8.660254037844385522, -19.74999999999996092 ) ) ;
#12487=CARTESIAN_POINT ( 'NONE',  ( 10.81189881249999729, 6.242252689847867408, -22.40625000204837747 ) ) ;
#12488=CARTESIAN_POINT ( 'NONE',  ( -9.999999999999998224, 5.773502691896259087, -149.8750000000000000 ) ) ;
#12489=ADVANCED_FACE ( 'NONE', ( #30396 ), #33842, .F. ) ;
#12493=CARTESIAN_POINT ( 'NONE',  ( -2.121150477449813534E-15, -11.54700538379251284, -195.8750000000000284 ) ) ;
#12494=CARTESIAN_POINT ( 'NONE',  ( -2.293366432827344421E-15, -12.48450537969573659, -126.4062500020483952 ) ) ;
#12495=ORIENTED_EDGE ( 'NONE', *, *, #20226, .F. ) ;
#12496=CARTESIAN_POINT ( 'NONE',  ( 10.00000000000102318, -5.773502691895667560, -12.62499999999993605 ) ) ;
#12497=VERTEX_POINT ( 'NONE', #39869 ) ;
#12498=CARTESIAN_POINT ( 'NONE',  ( -10.81189881249999729, 6.242252689847871849, -50.40625000204837391 ) ) ;
#12500=VECTOR ( 'NONE', #41088, 1000.000000000000000 ) ;
#12501=CARTESIAN_POINT ( 'NONE',  ( 10.81189881249999551, -6.242252689847874514, -104.9687500020483810 ) ) ;
#12502=EDGE_LOOP ( 'NONE', ( #31371, #19317, #9377, #18993 ) ) ;
#12503=EDGE_LOOP ( 'NONE', ( #36489, #27113, #2761, #29347 ) ) ;
#12506=CARTESIAN_POINT ( 'NONE',  ( 5.405949406249992428, -9.363379034771808662, -150.0937500020483810 ) ) ;
#12507=EDGE_CURVE ( 'NONE', #35463, #9647, #29388, .T. ) ;
#12509=CARTESIAN_POINT ( 'NONE',  ( 5.405949406249999534, 9.363379034771803333, -8.593750002048345493 ) ) ;
#12510=DIRECTION ( 'NONE',  ( -0.000000000000000000, -0.000000000000000000, 1.000000000000000000 ) ) ;
#12511=EDGE_CURVE ( 'NONE', #21406, #39053, #6199, .T. ) ;
#12512=CARTESIAN_POINT ( 'NONE',  ( -5.405949406250003975, -9.363379034771801557, -141.3437500020483810 ) ) ;
#12516=CARTESIAN_POINT ( 'NONE',  ( -5.000000000000003553, -8.660254037844383745, -190.3750000040967905 ) ) ;
#12518=CARTESIAN_POINT ( 'NONE',  ( 10.81189881249999551, -6.242252689847874514, -187.6562500020484094 ) ) ;
#12519=( BOUNDED_CURVE ( )  B_SPLINE_CURVE ( 2, ( #24273, #37420, #4829, #11501, #963, #24703, #27071 ),
 .UNSPECIFIED., .F., .F. ) 
 B_SPLINE_CURVE_WITH_KNOTS ( ( 3, 2, 2, 3 ),
 ( 0.5597014925373136052, 0.5609452736318409904, 0.5621890547263683757, 0.5634328358208957610 ),
 .UNSPECIFIED. ) 
 CURVE ( )  GEOMETRIC_REPRESENTATION_ITEM ( )  RATIONAL_B_SPLINE_CURVE ( ( 0.9999999999999761302, 0.8660254037844625774, 1.000000000000000000, 0.8660254037844387076, 1.000000000000000000, 0.8660254037844148378, 1.000000000000023981 ) ) 
 REPRESENTATION_ITEM ( '' )  );
#12523=CARTESIAN_POINT ( 'NONE',  ( 5.405949406249992428, -9.363379034771808662, -64.59375000204836681 ) ) ;
#12524=CARTESIAN_POINT ( 'NONE',  ( -10.81189881249999907, -6.242252689847864744, -45.46875000204837391 ) ) ;
#12526=CARTESIAN_POINT ( 'NONE',  ( -5.405949406250003975, -9.363379034771801557, -26.03125000204836681 ) ) ;
#12530=CARTESIAN_POINT ( 'NONE',  ( -9.999999999999998224, 5.773502691896259087, -112.3749999999999858 ) ) ;
#12531=CARTESIAN_POINT ( 'NONE',  ( -9.999999999999998224, 1.224646799147353059E-15, -200.0000000000000000 ) ) ;
#12534=CARTESIAN_POINT ( 'NONE',  ( -2.293366432827344421E-15, -12.48450537969573659, -114.4062500020483952 ) ) ;
#12539=CARTESIAN_POINT ( 'NONE',  ( 10.00000000000051159, -5.773502691895965988, -128.1250000000000000 ) ) ;
#12541=CARTESIAN_POINT ( 'NONE',  ( -10.00000000000000000, -5.773502691896251982, -44.62499999999997158 ) ) ;
#12542=AXIS2_PLACEMENT_3D ( 'NONE', #19922, #2905, #6556 ) ;
#12543=CARTESIAN_POINT ( 'NONE',  ( 7.070501591499377789E-16, 11.54700538379251284, -27.50000000409677980 ) ) ;
#12544=CARTESIAN_POINT ( 'NONE',  ( 10.81189881249999551, -6.242252689847874514, -51.15625000204837391 ) ) ;
#12545=CARTESIAN_POINT ( 'NONE',  ( -2.121150477449813534E-15, -11.54700538379251284, -141.8750000000000000 ) ) ;
#12548=CARTESIAN_POINT ( 'NONE',  ( -2.293366432827344421E-15, -12.48450537969573659, -133.9062500020483810 ) ) ;
#12549=CARTESIAN_POINT ( 'NONE',  ( 5.405949406249992428, -9.363379034771808662, -151.7812500020484094 ) ) ;
#12551=ORIENTED_EDGE ( 'NONE', *, *, #32029, .T. ) ;
#12552=ORIENTED_EDGE ( 'NONE', *, *, #27477, .T. ) ;
#12553=ORIENTED_EDGE ( 'NONE', *, *, #14304, .T. ) ;
#12554=FACE_OUTER_BOUND ( 'NONE', #14318, .T. ) ;
#12555=CARTESIAN_POINT ( 'NONE',  ( 10.81189881249999551, -6.242252689847874514, -181.4687500020484094 ) ) ;
#12556=VECTOR ( 'NONE', #18115, 1000.000000000000000 ) ;
#12557=CARTESIAN_POINT ( 'NONE',  ( -5.405949406250003975, -9.363379034771801557, -27.34375000204835970 ) ) ;
#12559=CARTESIAN_POINT ( 'NONE',  ( -10.81189881249999729, 6.242252689847871849, -165.7187500020483810 ) ) ;
#12560=CARTESIAN_POINT ( 'NONE',  ( -5.405949406249996869, 9.363379034771805109, -143.3437500020483810 ) ) ;
#12561=CYLINDRICAL_SURFACE ( 'NONE', #34871, 9.999999999999998224 ) ;
#12564=CARTESIAN_POINT ( 'NONE',  ( -5.405949406249996869, 9.363379034771805109, -20.34375000204835615 ) ) ;
#12569=EDGE_CURVE ( 'NONE', #26056, #3950, #22197, .T. ) ;
#12570=CARTESIAN_POINT ( 'NONE',  ( -2.293366432827344421E-15, -12.48450537969573659, -84.21875000204835260 ) ) ;
#12571=CARTESIAN_POINT ( 'NONE',  ( -10.81189881249999729, 6.242252689847871849, -51.90625000204838813 ) ) ;
#12575=CARTESIAN_POINT ( 'NONE',  ( 9.999999999999996447, -5.773502691896262640, -138.6250000000000000 ) ) ;
#12576=CARTESIAN_POINT ( 'NONE',  ( -10.81189881249999729, 6.242252689847871849, -144.9062500020484094 ) ) ;
#12577=CARTESIAN_POINT ( 'NONE',  ( -9.999999999998456346, -5.773502691897145489, -24.00000000409674428 ) ) ;
#12578=CARTESIAN_POINT ( 'NONE',  ( -2.121150477449813534E-15, -11.54700538379251284, -124.2500000040967763 ) ) ;
#12583=DIRECTION ( 'NONE',  ( 1.000000000000000000, 0.000000000000000000, 0.000000000000000000 ) ) ;
#12584=CARTESIAN_POINT ( 'NONE',  ( 5.405949406249999534, 9.363379034771803333, -169.2812500020484094 ) ) ;
#12585=CARTESIAN_POINT ( 'NONE',  ( -4.999999999999996447, 8.660254037844387298, -52.87500000409675494 ) ) ;
#12586=CARTESIAN_POINT ( 'NONE',  ( 4.999999999999992006, -8.660254037844389075, -98.24999999999998579 ) ) ;
#12588=EDGE_CURVE ( 'NONE', #28849, #12029, #35696, .T. ) ;
#12590=CARTESIAN_POINT ( 'NONE',  ( 5.405949406249999534, 9.363379034771803333, -170.7812500020484094 ) ) ;
#12591=CARTESIAN_POINT ( 'NONE',  ( 11.54700538379253061, -15.00000000000009770, 49.99999999999998579 ) ) ;
#12592=CARTESIAN_POINT ( 'NONE',  ( -9.999999999999998224, 1.224646799147353059E-15, -34.62500000409676915 ) ) ;
#12595=CARTESIAN_POINT ( 'NONE',  ( -10.81189881249999729, 1.324075727343319199E-15, -69.78125000204838102 ) ) ;
#12599=CARTESIAN_POINT ( 'NONE',  ( 5.405949406249992428, -9.363379034771808662, -31.59375000204836681 ) ) ;
#12600=CARTESIAN_POINT ( 'NONE',  ( 5.000000000000000000, 8.660254037844385522, -108.2499999999999858 ) ) ;
#12601=CARTESIAN_POINT ( 'NONE',  ( -10.81189881249999907, -6.242252689847864744, -5.156250002048356151 ) ) ;
#12602=CARTESIAN_POINT ( 'NONE',  ( -5.405949406249996869, 9.363379034771805109, -51.84375000204835260 ) ) ;
#12604=CARTESIAN_POINT ( 'NONE',  ( -2.121150477449813534E-15, -11.54700538379251284, -3.874999999999953815 ) ) ;
#12606=CARTESIAN_POINT ( 'NONE',  ( -2.293366432827344421E-15, -12.48450537969573659, -186.2187500020484094 ) ) ;
#12607=CARTESIAN_POINT ( 'NONE',  ( 10.81189881249999729, 0.000000000000000000, -173.8437500020484094 ) ) ;
#12610=ADVANCED_FACE ( 'NONE', ( #7084 ), #30814, .T. ) ;
#12611=CARTESIAN_POINT ( 'NONE',  ( -10.00000000000051337, 5.773502691895962435, -124.3749999999999858 ) ) ;
#12612=CARTESIAN_POINT ( 'NONE',  ( -2.121150477449813534E-15, -11.54700538379251284, -24.87499999999998934 ) ) ;
#12614=CARTESIAN_POINT ( 'NONE',  ( -10.81189881249999907, -6.242252689847864744, -105.4687500020483668 ) ) ;
#12615=CARTESIAN_POINT ( 'NONE',  ( -2.121150477449813534E-15, -11.54700538379251284, -47.75000000409676204 ) ) ;
#12616=CARTESIAN_POINT ( 'NONE',  ( -2.293366432827344421E-15, -12.48450537969573659, -76.90625000204839523 ) ) ;
#12618=CARTESIAN_POINT ( 'NONE',  ( -5.405949406249996869, 9.363379034771805109, -81.84375000204838102 ) ) ;
#12620=CARTESIAN_POINT ( 'NONE',  ( -4.999999999999996447, 8.660254037844387298, -147.3750000040967905 ) ) ;
#12622=ORIENTED_EDGE ( 'NONE', *, *, #39913, .F. ) ;
#12625=CARTESIAN_POINT ( 'NONE',  ( -10.81189881249999907, -6.242252689847864744, -194.1562500020484094 ) ) ;
#12626=CARTESIAN_POINT ( 'NONE',  ( -5.000000000000003553, -8.660254037844383745, -38.49999999999997868 ) ) ;
#12628=EDGE_LOOP ( 'NONE', ( #13764, #28670, #6474, #1472 ) ) ;
#12629=CARTESIAN_POINT ( 'NONE',  ( 5.000000000000000000, 8.660254037844385522, -63.24999999999997158 ) ) ;
#12631=CARTESIAN_POINT ( 'NONE',  ( -9.999999999999998224, 5.773502691896259087, -73.75000000409676204 ) ) ;
#12632=CYLINDRICAL_SURFACE ( 'NONE', #18972, 9.999999999999998224 ) ;
#12633=DIRECTION ( 'NONE',  ( 0.000000000000000000, -0.9961946980917455452, -0.08715574274765837404 ) ) ;
#12635=CARTESIAN_POINT ( 'NONE',  ( 5.405949406249999534, 9.363379034771803333, -64.28125000204836681 ) ) ;
#12636=( BOUNDED_CURVE ( )  B_SPLINE_CURVE ( 2, ( #18450, #37232, #24739, #37886, #1213, #27536, #40668 ),
 .UNSPECIFIED., .F., .F. ) 
 B_SPLINE_CURVE_WITH_KNOTS ( ( 3, 2, 2, 3 ),
 ( 0.8917910447761197013, 0.8930348258706470865, 0.8942786069651743608, 0.8955223880597017461 ),
 .UNSPECIFIED. ) 
 CURVE ( )  GEOMETRIC_REPRESENTATION_ITEM ( )  RATIONAL_B_SPLINE_CURVE ( ( 0.9999999999999641398, 0.8660254037844745678, 1.000000000000000000, 0.8660254037844387076, 1.000000000000000000, 0.8660254037844148378, 1.000000000000023981 ) ) 
 REPRESENTATION_ITEM ( '' )  );
#12640=CARTESIAN_POINT ( 'NONE',  ( 5.405949406249992428, -9.363379034771808662, -193.7812500020484094 ) ) ;
#12642=ADVANCED_FACE ( 'NONE', ( #24351 ), #40084, .T. ) ;
#12643=CARTESIAN_POINT ( 'NONE',  ( 5.405949406249992428, -9.363379034771808662, -1.593750002048366365 ) ) ;
#12644=CARTESIAN_POINT ( 'NONE',  ( -2.121150477449813534E-15, -11.54700538379251284, -110.7500000040967620 ) ) ;
#12646=CARTESIAN_POINT ( 'NONE',  ( 4.999999999999992006, -8.660254037844389075, -137.2499999999999716 ) ) ;
#12647=( BOUNDED_CURVE ( )  B_SPLINE_CURVE ( 2, ( #28889, #41601, #5362, #18518, #25644, #41383, #2137 ),
 .UNSPECIFIED., .F., .F. ) 
 B_SPLINE_CURVE_WITH_KNOTS ( ( 3, 2, 2, 3 ),
 ( 0.3656716417910448325, 0.3669154228855722732, 0.3681592039800996030, 0.3694029850746270438 ),
 .UNSPECIFIED. ) 
 CURVE ( )  GEOMETRIC_REPRESENTATION_ITEM ( )  RATIONAL_B_SPLINE_CURVE ( ( 0.9999999999999940048, 0.8660254037844447028, 1.000000000000000000, 0.8660254037844387076, 1.000000000000000000, 0.8660254037844207220, 1.000000000000017986 ) ) 
 REPRESENTATION_ITEM ( '' )  );
#12648=CARTESIAN_POINT ( 'NONE',  ( 10.00000000000000000, 5.773502691896255534, -177.3750000000000000 ) ) ;
#12649=CARTESIAN_POINT ( 'NONE',  ( -9.999999999999998224, 1.224646799147353059E-15, -37.24999999999997868 ) ) ;
#12650=CARTESIAN_POINT ( 'NONE',  ( -5.405949406249996869, 9.363379034771805109, -98.53125000204839523 ) ) ;
#12652=CARTESIAN_POINT ( 'NONE',  ( -10.00000000000102496, 5.773502691895664007, -37.37499999999992184 ) ) ;
#12655=CARTESIAN_POINT ( 'NONE',  ( -5.405949406249996869, 9.363379034771805109, -38.34375000204837391 ) ) ;
#12656=CARTESIAN_POINT ( 'NONE',  ( -10.81189881249999729, 6.242252689847871849, -29.40625000204835615 ) ) ;
#12658=CARTESIAN_POINT ( 'NONE',  ( -2.293366432827344421E-15, -12.48450537969573659, -78.21875000204838102 ) ) ;
#12659=CARTESIAN_POINT ( 'NONE',  ( -5.405949406249996869, 9.363379034771805109, -198.8437500020484094 ) ) ;
#12661=CARTESIAN_POINT ( 'NONE',  ( -4.999999999999996447, 8.660254037844387298, -49.49999999999998579 ) ) ;
#12663=CARTESIAN_POINT ( 'NONE',  ( 4.999999999999992006, -8.660254037844389075, -13.12500000409674783 ) ) ;
#12664=CYLINDRICAL_SURFACE ( 'NONE', #561, 9.999999999999998224 ) ;
#12665=CARTESIAN_POINT ( 'NONE',  ( -10.81189881249999907, -6.242252689847864744, -130.9687500020483810 ) ) ;
#12666=CARTESIAN_POINT ( 'NONE',  ( -2.293366432827344421E-15, -12.48450537969573659, -94.90625000204838102 ) ) ;
#12667=CARTESIAN_POINT ( 'NONE',  ( 5.405949406249999534, 9.363379034771803333, -110.5937500020483810 ) ) ;
#12670=CARTESIAN_POINT ( 'NONE',  ( 4.999999999999992006, -8.660254037844389075, -167.6250000040967905 ) ) ;
#12671=CARTESIAN_POINT ( 'NONE',  ( 0.000000000000000000, 0.000000000000000000, -200.0000000000000000 ) ) ;
#12675=CARTESIAN_POINT ( 'NONE',  ( 10.81189881249999729, 0.000000000000000000, -6.031250002048377468 ) ) ;
#12677=CARTESIAN_POINT ( 'NONE',  ( 0.000000000000000000, 0.000000000000000000, -200.0000000000000000 ) ) ;
#12679=CARTESIAN_POINT ( 'NONE',  ( 7.070501591499377789E-16, 11.54700538379251284, -88.62500000000000000 ) ) ;
#12681=CARTESIAN_POINT ( 'NONE',  ( 10.00000000000000000, 5.773502691896255534, -98.25000000409677625 ) ) ;
#12682=CARTESIAN_POINT ( 'NONE',  ( -10.00000000000051337, 5.773502691895962435, -150.2500000040967620 ) ) ;
#12684=CARTESIAN_POINT ( 'NONE',  ( -2.293366432827344421E-15, -12.48450537969573659, -93.40625000204838102 ) ) ;
#12685=ORIENTED_EDGE ( 'NONE', *, *, #3222, .T. ) ;
#12689=ORIENTED_EDGE ( 'NONE', *, *, #30835, .T. ) ;
#12690=CARTESIAN_POINT ( 'NONE',  ( -2.121150477449813534E-15, -11.54700538379251284, -17.37499999999997158 ) ) ;
#12692=CARTESIAN_POINT ( 'NONE',  ( -10.00000000000000000, -5.773502691896251982, -157.1250000000000284 ) ) ;
#12694=EDGE_CURVE ( 'NONE', #25687, #26580, #8963, .T. ) ;
#12696=CARTESIAN_POINT ( 'NONE',  ( -10.81189881249999729, 1.324075727343319199E-15, -122.2812500020483952 ) ) ;
#12698=CARTESIAN_POINT ( 'NONE',  ( -9.999999999998969713, -5.773502691896847949, -22.12499999999995026 ) ) ;
#12699=VERTEX_POINT ( 'NONE', #34912 ) ;
#12700=CARTESIAN_POINT ( 'NONE',  ( 7.644554776091147741E-16, 12.48450537969573659, -55.15625000204837391 ) ) ;
#12702=CARTESIAN_POINT ( 'NONE',  ( 5.405949406249992428, -9.363379034771808662, -103.5937500020483668 ) ) ;
#12704=ORIENTED_EDGE ( 'NONE', *, *, #3546, .F. ) ;
#12705=CARTESIAN_POINT ( 'NONE',  ( -9.999999999999998224, 1.224646799147353059E-15, -185.7500000000000000 ) ) ;
#12706=CARTESIAN_POINT ( 'NONE',  ( -7.071067811865472841, -7.071067811865472841, -200.0000000000000000 ) ) ;
#12709=CARTESIAN_POINT ( 'NONE',  ( 9.999999999999998224, 0.000000000000000000, -161.3750000040967905 ) ) ;
#12710=CARTESIAN_POINT ( 'NONE',  ( -5.405949406249996869, 9.363379034771805109, -137.3437500020484094 ) ) ;
#12711=( BOUNDED_CURVE ( )  B_SPLINE_CURVE ( 2, ( #36467, #26549, #39697, #15961, #22461, #25915, #39489 ),
 .UNSPECIFIED., .F., .F. ) 
 B_SPLINE_CURVE_WITH_KNOTS ( ( 3, 2, 2, 3 ),
 ( 0.5186567164179105571, 0.5199004975124379424, 0.5211442786069653277, 0.5223880597014926019 ),
 .UNSPECIFIED. ) 
 CURVE ( )  GEOMETRIC_REPRESENTATION_ITEM ( )  RATIONAL_B_SPLINE_CURVE ( ( 0.9999999999999880096, 0.8660254037844506980, 1.000000000000000000, 0.8660254037844387076, 1.000000000000000000, 0.8660254037844267172, 1.000000000000011990 ) ) 
 REPRESENTATION_ITEM ( '' )  );
#12713=DIRECTION ( 'NONE',  ( 1.000000000000000000, 0.000000000000000000, -0.000000000000000000 ) ) ;
#12715=CARTESIAN_POINT ( 'NONE',  ( -10.00000000000000000, -5.773502691896251982, -190.5000000040967905 ) ) ;
#12717=CARTESIAN_POINT ( 'NONE',  ( 5.405949406249992428, -9.363379034771808662, -184.7812500020484094 ) ) ;
#12721=CARTESIAN_POINT ( 'NONE',  ( 10.81189881249999729, 6.242252689847867408, -71.71875000204836681 ) ) ;
#12722=CARTESIAN_POINT ( 'NONE',  ( -5.405949406250003975, -9.363379034771801557, -49.84375000204838102 ) ) ;
#12725=CARTESIAN_POINT ( 'NONE',  ( -2.293366432827344421E-15, -12.48450537969573659, -25.90625000204838813 ) ) ;
#12727=CARTESIAN_POINT ( 'NONE',  ( 5.000000000000000000, 8.660254037844385522, -27.62500000409676204 ) ) ;
#12729=CARTESIAN_POINT ( 'NONE',  ( -9.999999999999998224, 5.773502691896259087, -116.8750000000000000 ) ) ;
#12730=CARTESIAN_POINT ( 'NONE',  ( -9.999999999999998224, 1.224646799147353059E-15, -163.2500000000000000 ) ) ;
#12733=CARTESIAN_POINT ( 'NONE',  ( -5.405949406249996869, 9.363379034771805109, -118.0312500020483952 ) ) ;
#12734=VERTEX_POINT ( 'NONE', #8787 ) ;
#12735=CARTESIAN_POINT ( 'NONE',  ( 9.999999999999998224, 0.000000000000000000, -122.0000000000000000 ) ) ;
#12739=VERTEX_POINT ( 'NONE', #5123 ) ;
#12740=CARTESIAN_POINT ( 'NONE',  ( 10.00000000000000000, 5.773502691896255534, -45.37499999999997158 ) ) ;
#12741=CARTESIAN_POINT ( 'NONE',  ( 9.999999999999996447, -5.773502691896262640, -16.00000000409677270 ) ) ;
#12742=EDGE_CURVE ( 'NONE', #32685, #12182, #24561, .T. ) ;
#12743=CARTESIAN_POINT ( 'NONE',  ( 7.644554776091147741E-16, 12.48450537969573659, -46.15625000204837391 ) ) ;
#12744=DIRECTION ( 'NONE',  ( -0.000000000000000000, 1.000000000000000000, -0.000000000000000000 ) ) ;
#12748=EDGE_CURVE ( 'NONE', #33637, #8113, #14729, .T. ) ;
#12750=CARTESIAN_POINT ( 'NONE',  ( 7.644554776091147741E-16, 12.48450537969573659, -139.1562500020483810 ) ) ;
#12752=CARTESIAN_POINT ( 'NONE',  ( -10.81189881249999729, 1.324075727343319199E-15, -146.2812500020483810 ) ) ;
#12754=CARTESIAN_POINT ( 'NONE',  ( -5.000000000000003553, -8.660254037844383745, -15.99999999999995914 ) ) ;
#12755=ORIENTED_EDGE ( 'NONE', *, *, #3158, .F. ) ;
#12756=AXIS2_PLACEMENT_3D ( 'NONE', #27241, #4372, #30284 ) ;
#12757=EDGE_LOOP ( 'NONE', ( #16677, #38454 ) ) ;
#12759=ORIENTED_EDGE ( 'NONE', *, *, #30711, .F. ) ;
#12761=CARTESIAN_POINT ( 'NONE',  ( 9.999999999999998224, 0.000000000000000000, -120.5000000000000000 ) ) ;
#12763=CARTESIAN_POINT ( 'NONE',  ( -10.81189881249999907, -6.242252689847864744, -174.4687500020484094 ) ) ;
#12764=CARTESIAN_POINT ( 'NONE',  ( 10.81189881249999729, 0.000000000000000000, -19.34375000204835260 ) ) ;
#12765=LINE ( 'NONE', #6318, #12245 ) ;
#12766=CARTESIAN_POINT ( 'NONE',  ( -10.81189881249999729, 6.242252689847871849, -162.7187500020483810 ) ) ;
#12767=CARTESIAN_POINT ( 'NONE',  ( 10.81189881249999907, 6.242252689847868297, -145.2187500020484094 ) ) ;
#12772=CARTESIAN_POINT ( 'NONE',  ( 10.81189881249999729, 0.000000000000000000, -19.34375000204835260 ) ) ;
#12776=CARTESIAN_POINT ( 'NONE',  ( -9.999999999999998224, 1.224646799147353059E-15, -43.62500000409677625 ) ) ;
#12779=CARTESIAN_POINT ( 'NONE',  ( 10.81189881249999729, 0.000000000000000000, -74.84375000204838102 ) ) ;
#12780=CARTESIAN_POINT ( 'NONE',  ( 5.405949406249999534, 9.363379034771803333, -47.78125000204838813 ) ) ;
#12782=CARTESIAN_POINT ( 'NONE',  ( 9.999999999999479527, 5.773502691896553074, -90.75000000409674783 ) ) ;
#12784=CARTESIAN_POINT ( 'NONE',  ( 5.000000000000000000, 8.660254037844385522, -139.7499999999999716 ) ) ;
#12785=VECTOR ( 'NONE', #21593, 1000.000000000000000 ) ;
#12786=CARTESIAN_POINT ( 'NONE',  ( -5.405949406249996869, 9.363379034771805109, -149.5312500020483810 ) ) ;
#12788=CARTESIAN_POINT ( 'NONE',  ( -10.00000000000000000, -5.773502691896251982, -111.0000000040967763 ) ) ;
#12793=CARTESIAN_POINT ( 'NONE',  ( -9.999999999999998224, 1.224646799147353059E-15, -52.24999999999996447 ) ) ;
#12794=CARTESIAN_POINT ( 'NONE',  ( 10.81189881249999729, 0.000000000000000000, -172.5312500020484094 ) ) ;
#12795=CARTESIAN_POINT ( 'NONE',  ( -10.00000000000000000, -5.773502691896251982, -54.00000000409676915 ) ) ;
#12796=FACE_OUTER_BOUND ( 'NONE', #41376, .T. ) ;
#12798=PLANE ( 'NONE',  #6265 ) ;
#12799=CARTESIAN_POINT ( 'NONE',  ( 5.405949406249992428, -9.363379034771808662, -157.7812500020484094 ) ) ;
#12800=CARTESIAN_POINT ( 'NONE',  ( -5.405949406250003975, -9.363379034771801557, -142.8437500020483810 ) ) ;
#12801=CARTESIAN_POINT ( 'NONE',  ( -10.00000000000051337, 5.773502691895962435, -100.3750000000000000 ) ) ;
#12802=CARTESIAN_POINT ( 'NONE',  ( 9.999999999999998224, 0.000000000000000000, -177.5000000000000000 ) ) ;
#12803=VERTEX_POINT ( 'NONE', #21944 ) ;
#12804=CARTESIAN_POINT ( 'NONE',  ( -10.00000000000019185, 5.773502691896147176, -189.2500000040968189 ) ) ;
#12805=VECTOR ( 'NONE', #13720, 1000.000000000000000 ) ;
#12807=CARTESIAN_POINT ( 'NONE',  ( -2.293366432827344421E-15, -12.48450537969573659, -67.90625000204840944 ) ) ;
#12810=CARTESIAN_POINT ( 'NONE',  ( 5.405949406249999534, 9.363379034771803333, -121.0937500020483952 ) ) ;
#12812=ORIENTED_EDGE ( 'NONE', *, *, #31197, .T. ) ;
#12813=CARTESIAN_POINT ( 'NONE',  ( 10.81189881249999729, 6.242252689847867408, -28.21875000204838813 ) ) ;
#12814=FACE_OUTER_BOUND ( 'NONE', #52, .T. ) ;
#12815=CARTESIAN_POINT ( 'NONE',  ( -5.405949406249996869, 9.363379034771805109, -195.8437500020484094 ) ) ;
#12817=CARTESIAN_POINT ( 'NONE',  ( -10.81189881249999729, 1.324075727343319199E-15, -57.59375000204835970 ) ) ;
#12818=DIRECTION ( 'NONE',  ( -0.000000000000000000, -0.000000000000000000, 1.000000000000000000 ) ) ;
#12820=CARTESIAN_POINT ( 'NONE',  ( 10.81189881249999729, 0.000000000000000000, -191.8437500020484094 ) ) ;
#12821=CARTESIAN_POINT ( 'NONE',  ( -5.405949406249996869, 9.363379034771805109, -168.8437500020484094 ) ) ;
#12824=CARTESIAN_POINT ( 'NONE',  ( 9.999999999999998224, 0.000000000000000000, -177.8750000040967905 ) ) ;
#12827=CARTESIAN_POINT ( 'NONE',  ( 7.644554776091147741E-16, 12.48450537969573659, -93.96875000204838102 ) ) ;
#12828=CARTESIAN_POINT ( 'NONE',  ( -2.121150477449813534E-15, -11.54700538379251284, -84.87500000000000000 ) ) ;
#12829=CARTESIAN_POINT ( 'NONE',  ( 10.81189881249999551, -6.242252689847874514, -72.15625000204836681 ) ) ;
#12830=CARTESIAN_POINT ( 'NONE',  ( 9.999999999999998224, 0.000000000000000000, -198.5000000000000000 ) ) ;
#12832=CARTESIAN_POINT ( 'NONE',  ( 7.644554776091147741E-16, 12.48450537969573659, -83.46875000204838102 ) ) ;
#12835=CARTESIAN_POINT ( 'NONE',  ( -9.999999999999998224, 5.773502691896259087, -147.2500000040967905 ) ) ;
#12840=CARTESIAN_POINT ( 'NONE',  ( -5.405949406250003975, -9.363379034771801557, -197.0312500020484094 ) ) ;
#12841=CARTESIAN_POINT ( 'NONE',  ( -9.999999999998456346, -5.773502691897145489, -52.12499999999994316 ) ) ;
#12843=ORIENTED_EDGE ( 'NONE', *, *, #25949, .T. ) ;
#12844=CARTESIAN_POINT ( 'NONE',  ( 7.070501591499377789E-16, 11.54700538379251284, -58.62499999999998579 ) ) ;
#12846=CARTESIAN_POINT ( 'NONE',  ( -9.999999999999998224, 5.773502691896259087, -76.75000000409676204 ) ) ;
#12848=DIRECTION ( 'NONE',  ( 1.000000000000000000, 0.000000000000000000, 0.000000000000000000 ) ) ;
#12850=CARTESIAN_POINT ( 'NONE',  ( -10.81189881249999729, 6.242252689847871849, -65.40625000204839523 ) ) ;
#12854=CARTESIAN_POINT ( 'NONE',  ( 10.81189881249999551, -6.242252689847874514, -181.6562500020484379 ) ) ;
#12856=CARTESIAN_POINT ( 'NONE',  ( -10.00000000000000000, -5.773502691896252870, -172.5000000040967905 ) ) ;
#12857=CARTESIAN_POINT ( 'NONE',  ( 9.999999999999998224, 0.000000000000000000, -152.0000000000000000 ) ) ;
#12858=CARTESIAN_POINT ( 'NONE',  ( -9.999999999999998224, 1.224646799147353059E-15, -137.7499999999999716 ) ) ;
#12859=CARTESIAN_POINT ( 'NONE',  ( -4.999999999999996447, 8.660254037844387298, -178.5000000000000000 ) ) ;
#12860=CARTESIAN_POINT ( 'NONE',  ( -10.00000000000102496, 5.773502691895664007, -1.374999999999948486 ) ) ;
#12861=CARTESIAN_POINT ( 'NONE',  ( -5.405949406250003975, -9.363379034771801557, -93.53125000204838102 ) ) ;
#12862=ORIENTED_EDGE ( 'NONE', *, *, #2974, .T. ) ;
#12863=CARTESIAN_POINT ( 'NONE',  ( 9.999999999999998224, 0.000000000000000000, -200.0000000000000000 ) ) ;
#12864=ORIENTED_EDGE ( 'NONE', *, *, #27809, .T. ) ;
#12865=VERTEX_POINT ( 'NONE', #12216 ) ;
#12866=CARTESIAN_POINT ( 'NONE',  ( -10.81189881249999729, 6.242252689847871849, -36.71875000204835970 ) ) ;
#12867=CARTESIAN_POINT ( 'NONE',  ( -5.405949406250003975, -9.363379034771801557, -33.53125000204837391 ) ) ;
#12868=SHAPE_DEFINITION_REPRESENTATION ( #33876, #31964 ) ;
#12869=CARTESIAN_POINT ( 'NONE',  ( 10.81189881249999907, 6.242252689847868297, -79.21875000204838102 ) ) ;
#12870=CARTESIAN_POINT ( 'NONE',  ( 10.00000000000102318, -5.773502691895667560, -83.50000000409673362 ) ) ;
#12871=CARTESIAN_POINT ( 'NONE',  ( -10.81189881249999729, 1.324075727343319199E-15, -195.5937500020484094 ) ) ;
#12872=ADVANCED_FACE ( 'NONE', ( #34274 ), #42625, .T. ) ;
#12874=CARTESIAN_POINT ( 'NONE',  ( 9.999999999999227285, 5.773502691896701400, -112.8749999999999716 ) ) ;
#12876=CARTESIAN_POINT ( 'NONE',  ( -10.00000000000000000, -5.773502691896251982, -13.50000000409675849 ) ) ;
#12878=CARTESIAN_POINT ( 'NONE',  ( 10.81189881249999907, 6.242252689847868297, -128.7187500020483810 ) ) ;
#12879=CARTESIAN_POINT ( 'NONE',  ( 10.81189881249999551, -6.242252689847874514, -102.1562500020483952 ) ) ;
#12880=CARTESIAN_POINT ( 'NONE',  ( -10.81189881249999729, 6.242252689847871849, -108.7187500020483810 ) ) ;
#12883=CARTESIAN_POINT ( 'NONE',  ( -10.00000000000000000, -5.773502691896251982, -171.0000000040967905 ) ) ;
#12885=CYLINDRICAL_SURFACE ( 'NONE', #41985, 9.999999999999998224 ) ;
#12891=CARTESIAN_POINT ( 'NONE',  ( 9.999999999999998224, 0.000000000000000000, -128.0000000000000000 ) ) ;
#12893=CARTESIAN_POINT ( 'NONE',  ( 5.000000000000000000, 8.660254037844385522, -79.74999999999998579 ) ) ;
#12895=CARTESIAN_POINT ( 'NONE',  ( -9.999999999999998224, 1.224646799147353059E-15, -100.6250000040967905 ) ) ;
#12897=CARTESIAN_POINT ( 'NONE',  ( 5.405949406249999534, 9.363379034771803333, -94.28125000204838102 ) ) ;
#12898=VERTEX_POINT ( 'NONE', #5765 ) ;
#12902=ORIENTED_EDGE ( 'NONE', *, *, #32403, .F. ) ;
#12903=CARTESIAN_POINT ( 'NONE',  ( 7.070501591499377789E-16, 11.54700538379251284, -18.12499999999997513 ) ) ;
#12904=CARTESIAN_POINT ( 'NONE',  ( 9.999999999999998224, 0.000000000000000000, -153.5000000000000000 ) ) ;
#12906=CARTESIAN_POINT ( 'NONE',  ( -2.121150477449813534E-15, -11.54700538379251284, -198.8750000000000284 ) ) ;
#12907=CARTESIAN_POINT ( 'NONE',  ( -2.293366432827344421E-15, -12.48450537969573659, -118.9062500020483952 ) ) ;
#12910=CARTESIAN_POINT ( 'NONE',  ( 7.070501591499376803E-16, 11.54700538379251284, -117.5000000040967905 ) ) ;
#12912=CARTESIAN_POINT ( 'NONE',  ( -10.81189881249999907, -6.242252689847864744, -57.65625000204838102 ) ) ;
#12914=CARTESIAN_POINT ( 'NONE',  ( -10.81189881249999729, 6.242252689847871849, -99.71875000204839523 ) ) ;
#12916=CARTESIAN_POINT ( 'NONE',  ( -4.999999999999996447, 8.660254037844387298, -51.37500000409675494 ) ) ;
#12917=CARTESIAN_POINT ( 'NONE',  ( 9.999999999999998224, 0.000000000000000000, -54.49999999999996447 ) ) ;
#12919=CARTESIAN_POINT ( 'NONE',  ( 5.405949406249992428, -9.363379034771808662, -3.093750002048367698 ) ) ;
#12921=EDGE_CURVE ( 'NONE', #22119, #7656, #33800, .T. ) ;
#12922=CARTESIAN_POINT ( 'NONE',  ( 5.405949406249999534, 9.363379034771803333, -134.5937500020483810 ) ) ;
#12924=LINE ( 'NONE', #14, #14574 ) ;
#12926=CARTESIAN_POINT ( 'NONE',  ( -4.999999999999996447, 8.660254037844387298, -195.3750000040967905 ) ) ;
#12928=CARTESIAN_POINT ( 'NONE',  ( -10.81189881249999729, -6.242252689847864744, -188.1562500020484094 ) ) ;
#12929=CARTESIAN_POINT ( 'NONE',  ( 9.999999999999998224, 0.000000000000000000, -185.3750000040967905 ) ) ;
#12932=CARTESIAN_POINT ( 'NONE',  ( 10.81189881249999551, -6.242252689847874514, -56.96875000204838102 ) ) ;
#12933=CARTESIAN_POINT ( 'NONE',  ( 5.405949406249992428, -9.363379034771808662, -48.09375000204838102 ) ) ;
#12935=CARTESIAN_POINT ( 'NONE',  ( -10.81189881249999729, 6.242252689847871849, -18.90625000204837391 ) ) ;
#12936=VECTOR ( 'NONE', #15433, 1000.000000000000000 ) ;
#12938=CARTESIAN_POINT ( 'NONE',  ( -7.216878364870405349, -17.50000000000005684, 49.99999999999998579 ) ) ;
#12940=CARTESIAN_POINT ( 'NONE',  ( 5.000000000000000000, 8.660254037844385522, -117.2500000000000000 ) ) ;
#12941=VECTOR ( 'NONE', #21864, 1000.000000000000000 ) ;
#12945=CARTESIAN_POINT ( 'NONE',  ( 5.405949406249992428, -9.363379034771808662, -117.2812500020483952 ) ) ;
#12946=ORIENTED_EDGE ( 'NONE', *, *, #2253, .F. ) ;
#12947=CARTESIAN_POINT ( 'NONE',  ( -9.999999999999998224, 1.224646799147353059E-15, -82.62500000409676204 ) ) ;
#12949=DIRECTION ( 'NONE',  ( 1.000000000000000000, 0.000000000000000000, 0.000000000000000000 ) ) ;
#12951=ORIENTED_EDGE ( 'NONE', *, *, #20669, .F. ) ;
#12952=CARTESIAN_POINT ( 'NONE',  ( -9.999999999999998224, 1.224646799147353059E-15, -41.74999999999997868 ) ) ;
#12953=CARTESIAN_POINT ( 'NONE',  ( -5.000000000000003553, -8.660254037844383745, -19.37500000409675494 ) ) ;
#12954=CARTESIAN_POINT ( 'NONE',  ( -5.405949406250003975, -9.363379034771801557, -45.53125000204838102 ) ) ;
#12955=CARTESIAN_POINT ( 'NONE',  ( -4.999999999999996447, 8.660254037844387298, -16.49999999999995737 ) ) ;
#12959=CARTESIAN_POINT ( 'NONE',  ( 10.81189881249999729, 0.000000000000000000, -141.0312500020483810 ) ) ;
#12960=CARTESIAN_POINT ( 'NONE',  ( -10.81189881249999729, 6.242252689847871849, -153.9062500020483810 ) ) ;
#12962=VERTEX_POINT ( 'NONE', #38776 ) ;
#12963=ORIENTED_EDGE ( 'NONE', *, *, #25277, .T. ) ;
#12964=ORIENTED_EDGE ( 'NONE', *, *, #20399, .F. ) ;
#12965=VECTOR ( 'NONE', #2513, 1000.000000000000000 ) ;
#12968=CARTESIAN_POINT ( 'NONE',  ( -2.293366432827344421E-15, -12.48450537969573659, -175.7187500020483810 ) ) ;
#12969=CARTESIAN_POINT ( 'NONE',  ( 5.405949406249999534, 9.363379034771803333, -23.59375000204835970 ) ) ;
#12972=CARTESIAN_POINT ( 'NONE',  ( -5.405949406249996869, 9.363379034771805109, -156.8437500020483810 ) ) ;
#12973=CARTESIAN_POINT ( 'NONE',  ( -5.405949406249996869, 9.363379034771805109, -141.8437500020483810 ) ) ;
#12977=CARTESIAN_POINT ( 'NONE',  ( 5.405949406249999534, 9.363379034771803333, -20.59375000204835615 ) ) ;
#12983=CARTESIAN_POINT ( 'NONE',  ( -5.405949406250003975, -9.363379034771801557, -69.34375000204836681 ) ) ;
#12984=CARTESIAN_POINT ( 'NONE',  ( 10.81189881249999907, 6.242252689847868297, -38.90625000204835970 ) ) ;
#12986=CARTESIAN_POINT ( 'NONE',  ( 9.999999999998969713, 5.773502691896851502, -57.37499999999996447 ) ) ;
#12988=CARTESIAN_POINT ( 'NONE',  ( 5.000000000000000000, 8.660254037844385522, -141.2500000000000000 ) ) ;
#12989=CARTESIAN_POINT ( 'NONE',  ( -10.81189881249999729, 1.324075727343319199E-15, -138.7812500020483810 ) ) ;
#12992=CARTESIAN_POINT ( 'NONE',  ( 4.999999999999992006, -8.660254037844389075, -110.6250000040967763 ) ) ;
#12997=CARTESIAN_POINT ( 'NONE',  ( -10.81189881249999729, 1.324075727343319199E-15, -176.2812500020484094 ) ) ;
#12998=CARTESIAN_POINT ( 'NONE',  ( -9.999999999999998224, 5.773502691896259087, -39.25000000409676915 ) ) ;
#12999=EDGE_CURVE ( 'NONE', #4387, #17690, #32725, .T. ) ;
#13000=AXIS2_PLACEMENT_3D ( 'NONE', #38277, #14954, #12360 ) ;
#13001=DIRECTION ( 'NONE',  ( -0.000000000000000000, -0.000000000000000000, 1.000000000000000000 ) ) ;
#13003=CARTESIAN_POINT ( 'NONE',  ( -9.999999999999998224, 1.224646799147353059E-15, -155.7500000000000000 ) ) ;
#13004=CARTESIAN_POINT ( 'NONE',  ( 10.81189881249999551, -6.242252689847874514, -165.1562500020483526 ) ) ;
#13006=AXIS2_PLACEMENT_3D ( 'NONE', #8781, #2528, #6182 ) ;
#13007=CARTESIAN_POINT ( 'NONE',  ( -10.81189881249999729, 1.324075727343319199E-15, -141.5937500020483810 ) ) ;
#13009=CYLINDRICAL_SURFACE ( 'NONE', #1365, 9.999999999999998224 ) ;
#13011=ORIENTED_EDGE ( 'NONE', *, *, #36194, .F. ) ;
#13013=( BOUNDED_CURVE ( )  B_SPLINE_CURVE ( 2, ( #24844, #24627, #17902, #20937, #37774, #37559, #31099 ),
 .UNSPECIFIED., .F., .F. ) 
 B_SPLINE_CURVE_WITH_KNOTS ( ( 3, 2, 2, 3 ),
 ( 0.5335820895522389584, 0.5348258706467662327, 0.5360696517412936180, 0.5373134328358210032 ),
 .UNSPECIFIED. ) 
 CURVE ( )  GEOMETRIC_REPRESENTATION_ITEM ( )  RATIONAL_B_SPLINE_CURVE ( ( 0.9999999999999880096, 0.8660254037844506980, 1.000000000000000000, 0.8660254037844387076, 1.000000000000000000, 0.8660254037844267172, 1.000000000000011990 ) ) 
 REPRESENTATION_ITEM ( '' )  );
#13015=CARTESIAN_POINT ( 'NONE',  ( -5.405949406250003975, -9.363379034771801557, -71.03125000204838102 ) ) ;
#13016=ORIENTED_EDGE ( 'NONE', *, *, #8670, .F. ) ;
#13017=CARTESIAN_POINT ( 'NONE',  ( -10.81189881249999907, -6.242252689847864744, -120.4687500020483810 ) ) ;
#13020=VERTEX_POINT ( 'NONE', #29068 ) ;
#13021=CARTESIAN_POINT ( 'NONE',  ( 5.405949406249992428, -9.363379034771808662, -18.09375000204835260 ) ) ;
#13022=CARTESIAN_POINT ( 'NONE',  ( 10.81189881249999907, 6.242252689847868297, -199.2187500020484094 ) ) ;
#13023=( BOUNDED_CURVE ( )  B_SPLINE_CURVE ( 2, ( #32863, #3295, #39533, #9963, #23141, #19890, #33073 ),
 .UNSPECIFIED., .F., .F. ) 
 B_SPLINE_CURVE_WITH_KNOTS ( ( 3, 2, 2, 3 ),
 ( 0.9440298507462689948, 0.9452736318407963800, 0.9465174129353237653, 0.9477611940298510396 ),
 .UNSPECIFIED. ) 
 CURVE ( )  GEOMETRIC_REPRESENTATION_ITEM ( )  RATIONAL_B_SPLINE_CURVE ( ( 0.9999999999999641398, 0.8660254037844745678, 1.000000000000000000, 0.8660254037844387076, 1.000000000000000000, 0.8660254037844028474, 1.000000000000035971 ) ) 
 REPRESENTATION_ITEM ( '' )  );
#13024=CARTESIAN_POINT ( 'NONE',  ( -2.293366432827344421E-15, -12.48450537969573659, -48.21875000204836681 ) ) ;
#13027=CARTESIAN_POINT ( 'NONE',  ( -5.405949406250003975, -9.363379034771801557, -184.8437500020483810 ) ) ;
#13028=CARTESIAN_POINT ( 'NONE',  ( -10.81189881249999729, 6.242252689847871849, -167.2187500020483810 ) ) ;
#13032=CARTESIAN_POINT ( 'NONE',  ( -10.00000000000015987, 5.773502691896167605, -193.3750000000000853 ) ) ;
#13035=CARTESIAN_POINT ( 'NONE',  ( -10.81189881249999907, -6.242252689847864744, -96.46875000204838102 ) ) ;
#13036=CARTESIAN_POINT ( 'NONE',  ( 10.81189881249999551, -6.242252689847874514, -78.15625000204838102 ) ) ;
#13037=CARTESIAN_POINT ( 'NONE',  ( -5.000000000000003553, -8.660254037844383745, -131.8750000040967905 ) ) ;
#13039=CARTESIAN_POINT ( 'NONE',  ( 5.405949406249999534, 9.363379034771803333, -166.2812500020484094 ) ) ;
#13041=CARTESIAN_POINT ( 'NONE',  ( -5.000000000000003553, -8.660254037844383745, -137.8750000040967905 ) ) ;
#13043=ORIENTED_EDGE ( 'NONE', *, *, #17790, .F. ) ;
#13047=ADVANCED_FACE ( 'NONE', ( #42206 ), #12632, .T. ) ;
#13048=CARTESIAN_POINT ( 'NONE',  ( -10.81189881249999907, -6.242252689847864744, -198.6562500020484094 ) ) ;
#13049=CARTESIAN_POINT ( 'NONE',  ( -4.999999999999996447, 8.660254037844387298, -130.8750000040967905 ) ) ;
#13052=CARTESIAN_POINT ( 'NONE',  ( -10.00000000000000000, -5.773502691896251982, -53.62499999999997868 ) ) ;
#13054=CARTESIAN_POINT ( 'NONE',  ( -4.999999999999996447, 8.660254037844387298, -64.87500000409676204 ) ) ;
#13056=CARTESIAN_POINT ( 'NONE',  ( 7.070501591499376803E-16, 11.54700538379251284, -12.50000000409677092 ) ) ;
#13058=CARTESIAN_POINT ( 'NONE',  ( 10.81189881249999729, 0.000000000000000000, -70.53125000204838102 ) ) ;
#13061=CARTESIAN_POINT ( 'NONE',  ( 5.000000000000000000, 8.660254037844385522, -38.12500000409676915 ) ) ;
#13062=CARTESIAN_POINT ( 'NONE',  ( -10.81189881249999729, 1.324075727343319199E-15, -188.2812500020484094 ) ) ;
#13064=CARTESIAN_POINT ( 'NONE',  ( -2.121150477449813534E-15, -11.54700538379251284, -172.2500000040968189 ) ) ;
#13065=DIRECTION ( 'NONE',  ( -0.000000000000000000, -0.000000000000000000, 1.000000000000000000 ) ) ;
#13067=CARTESIAN_POINT ( 'NONE',  ( -2.121150477449813534E-15, -11.54700538379251284, -167.3750000000000000 ) ) ;
#13068=CARTESIAN_POINT ( 'NONE',  ( 5.000000000000000000, 8.660254037844385522, -97.74999999999998579 ) ) ;
#13069=AXIS2_PLACEMENT_3D ( 'NONE', #20665, #4277, #30406 ) ;
#13070=CARTESIAN_POINT ( 'NONE',  ( -5.405949406250003975, -9.363379034771801557, -92.03125000204838102 ) ) ;
#13071=ORIENTED_EDGE ( 'NONE', *, *, #1972, .T. ) ;
#13072=CARTESIAN_POINT ( 'NONE',  ( -9.999999999999872102, -5.773502691896326589, -163.1250000000000000 ) ) ;
#13074=ORIENTED_EDGE ( 'NONE', *, *, #24533, .F. ) ;
#13075=EDGE_LOOP ( 'NONE', ( #34062, #12812, #2969, #31590 ) ) ;
#13076=CARTESIAN_POINT ( 'NONE',  ( 10.81189881249999907, 6.242252689847868297, -31.21875000204835260 ) ) ;
#13077=CARTESIAN_POINT ( 'NONE',  ( 10.81189881249999907, 6.242252689847868297, -20.90625000204836681 ) ) ;
#13078=CARTESIAN_POINT ( 'NONE',  ( -2.293366432827344421E-15, -12.48450537969573659, -75.21875000204839523 ) ) ;
#13079=CARTESIAN_POINT ( 'NONE',  ( 9.999999999999866773, -5.773502691896336358, -173.5000000040967905 ) ) ;
#13080=CARTESIAN_POINT ( 'NONE',  ( 5.405949406249992428, -9.363379034771808662, -190.5937500020484094 ) ) ;
#13081=CARTESIAN_POINT ( 'NONE',  ( -4.999999999999996447, 8.660254037844387298, -98.99999999999998579 ) ) ;
#13082=CARTESIAN_POINT ( 'NONE',  ( -5.000000000000003553, -8.660254037844383745, -143.8750000040967905 ) ) ;
#13084=CARTESIAN_POINT ( 'NONE',  ( -4.999999999999996447, 8.660254037844387298, -4.875000004096769146 ) ) ;
#13086=CARTESIAN_POINT ( 'NONE',  ( 5.405949406249992428, -9.363379034771808662, -123.0937500020483952 ) ) ;
#13087=CARTESIAN_POINT ( 'NONE',  ( -10.81189881249999729, 6.242252689847871849, -96.90625000204838102 ) ) ;
#13088=CARTESIAN_POINT ( 'NONE',  ( -5.405949406250003975, -9.363379034771801557, -111.3437500020483810 ) ) ;
#13091=CARTESIAN_POINT ( 'NONE',  ( 9.999999999999996447, -5.773502691896262640, -163.0000000040967905 ) ) ;
#13092=CARTESIAN_POINT ( 'NONE',  ( -9.999999999998456346, -5.773502691897145489, -67.12499999999997158 ) ) ;
#13096=EDGE_CURVE ( 'NONE', #25538, #36134, #38205, .T. ) ;
#13098=CARTESIAN_POINT ( 'NONE',  ( -9.999999999999804601, -5.773502691896363892, -190.1250000000000284 ) ) ;
#13100=CARTESIAN_POINT ( 'NONE',  ( 10.00000000000025402, -5.773502691896113426, -126.6249999999999858 ) ) ;
#13102=CARTESIAN_POINT ( 'NONE',  ( -4.999999999999996447, 8.660254037844387298, -80.99999999999998579 ) ) ;
#13104=CARTESIAN_POINT ( 'NONE',  ( 5.000000000000000000, 8.660254037844385522, -96.62500000409677625 ) ) ;
#13105=LINE ( 'NONE', #36014, #28630 ) ;
#13107=CARTESIAN_POINT ( 'NONE',  ( 5.405949406249999534, 9.363379034771803333, -89.78125000204838102 ) ) ;
#13108=ORIENTED_EDGE ( 'NONE', *, *, #20159, .F. ) ;
#13112=EDGE_LOOP ( 'NONE', ( #18446, #16681, #13256, #6045 ) ) ;
#13113=CARTESIAN_POINT ( 'NONE',  ( -2.121150477449813534E-15, -11.54700538379251284, -6.874999999999968026 ) ) ;
#13114=CARTESIAN_POINT ( 'NONE',  ( -9.999999999999998224, 5.773502691896259087, -146.8750000000000000 ) ) ;
#13116=EDGE_CURVE ( 'NONE', #9902, #14006, #4801, .T. ) ;
#13117=CARTESIAN_POINT ( 'NONE',  ( 7.070501591499377789E-16, 11.54700538379251284, -193.6250000000000000 ) ) ;
#13118=CARTESIAN_POINT ( 'NONE',  ( -10.81189881249999729, 6.242252689847871849, -120.9062500020483952 ) ) ;
#13119=ORIENTED_EDGE ( 'NONE', *, *, #13096, .T. ) ;
#13121=ORIENTED_EDGE ( 'NONE', *, *, #19118, .F. ) ;
#13122=CARTESIAN_POINT ( 'NONE',  ( -5.405949406249996869, 9.363379034771805109, -46.03125000204838813 ) ) ;
#13125=CARTESIAN_POINT ( 'NONE',  ( -5.405949406250003975, -9.363379034771801557, -103.8437500020483810 ) ) ;
#13126=CARTESIAN_POINT ( 'NONE',  ( 5.405949406249992428, -9.363379034771808662, -126.2812500020483668 ) ) ;
#13127=ORIENTED_EDGE ( 'NONE', *, *, #38472, .F. ) ;
#13128=AXIS2_PLACEMENT_3D ( 'NONE', #15193, #35076, #35289 ) ;
#13129=CARTESIAN_POINT ( 'NONE',  ( -9.999999999999998224, 1.224646799147353059E-15, -83.74999999999997158 ) ) ;
#13130=FACE_OUTER_BOUND ( 'NONE', #35779, .T. ) ;
#13133=CARTESIAN_POINT ( 'NONE',  ( -2.293366432827344421E-15, -12.48450537969573659, -0.2187500020483489072 ) ) ;
#13135=CARTESIAN_POINT ( 'NONE',  ( 5.405949406249992428, -9.363379034771808662, -130.5937500020483810 ) ) ;
#13137=CARTESIAN_POINT ( 'NONE',  ( 9.999999999999998224, 0.000000000000000000, -158.0000000000000000 ) ) ;
#13139=CARTESIAN_POINT ( 'NONE',  ( 7.070501591499377789E-16, 11.54700538379251284, -191.0000000040968189 ) ) ;
#13141=CARTESIAN_POINT ( 'NONE',  ( 10.81189881249999729, 0.000000000000000000, -189.0312500020484094 ) ) ;
#13142=EDGE_CURVE ( 'NONE', #17371, #15042, #33789, .T. ) ;
#13146=CARTESIAN_POINT ( 'NONE',  ( 10.81189881249999729, 6.242252689847867408, -58.21875000204836681 ) ) ;
#13147=CARTESIAN_POINT ( 'NONE',  ( -10.81189881249999729, 6.242252689847871849, -51.71875000204836681 ) ) ;
#13149=CARTESIAN_POINT ( 'NONE',  ( 10.81189881249999907, 6.242252689847868297, -22.40625000204837747 ) ) ;
#13153=CARTESIAN_POINT ( 'NONE',  ( 9.999999999999996447, -5.773502691896262640, -107.1249999999999858 ) ) ;
#13155=CARTESIAN_POINT ( 'NONE',  ( 7.070501591499376803E-16, 11.54700538379251284, -119.0000000040967763 ) ) ;
#13158=CARTESIAN_POINT ( 'NONE',  ( 10.81189881249999551, -6.242252689847874514, -117.1562500020483952 ) ) ;
#13160=VECTOR ( 'NONE', #33278, 1000.000000000000000 ) ;
#13166=CARTESIAN_POINT ( 'NONE',  ( 7.070501591499377789E-16, 11.54700538379251284, -30.12499999999995026 ) ) ;
#13168=CARTESIAN_POINT ( 'NONE',  ( -5.000000000000003553, -8.660254037844383745, -17.87500000409675138 ) ) ;
#13169=CARTESIAN_POINT ( 'NONE',  ( 10.81189881249999729, 6.242252689847867408, -40.40625000204836681 ) ) ;
#13170=CARTESIAN_POINT ( 'NONE',  ( -10.00000000000076916, 5.773502691895813221, -111.2500000040967620 ) ) ;
#13173=CARTESIAN_POINT ( 'NONE',  ( 10.81189881249999551, -6.242252689847874514, -138.1562500020484094 ) ) ;
#13174=AXIS2_PLACEMENT_3D ( 'NONE', #32440, #31591, #32228 ) ;
#13175=CARTESIAN_POINT ( 'NONE',  ( -5.405949406249996869, 9.363379034771805109, -140.5312500020484094 ) ) ;
#13176=EDGE_CURVE ( 'NONE', #37116, #34874, #26609, .T. ) ;
#13177=CARTESIAN_POINT ( 'NONE',  ( -1.040834085586084257E-14, -20.00000000000000355, 22.49999999999999289 ) ) ;
#13178=ORIENTED_EDGE ( 'NONE', *, *, #1177, .F. ) ;
#13180=ORIENTED_EDGE ( 'NONE', *, *, #8656, .F. ) ;
#13181=CARTESIAN_POINT ( 'NONE',  ( -9.999999999999742428, -5.773502691896402084, -121.5000000040967905 ) ) ;
#13182=CARTESIAN_POINT ( 'NONE',  ( -2.293366432827344421E-15, -12.48450537969573659, -174.2187500020484094 ) ) ;
#13184=CARTESIAN_POINT ( 'NONE',  ( 10.81189881249999551, -6.242252689847874514, -26.96875000204837747 ) ) ;
#13186=CARTESIAN_POINT ( 'NONE',  ( 10.81189881249999729, 6.242252689847867408, -154.2187500020483810 ) ) ;
#13187=CARTESIAN_POINT ( 'NONE',  ( -2.293366432827344421E-15, -12.48450537969573659, -148.7187500020484094 ) ) ;
#13191=CARTESIAN_POINT ( 'NONE',  ( 5.405949406249999534, 9.363379034771803333, -22.09375000204835615 ) ) ;
#13193=DIRECTION ( 'NONE',  ( 1.000000000000000000, 0.000000000000000000, 0.000000000000000000 ) ) ;
#13196=CARTESIAN_POINT ( 'NONE',  ( 7.070501591499376803E-16, 11.54700538379251284, -56.00000000409676915 ) ) ;
#13197=CARTESIAN_POINT ( 'NONE',  ( 10.81189881249999551, -6.242252689847874514, -70.46875000204840944 ) ) ;
#13198=CARTESIAN_POINT ( 'NONE',  ( 5.405949406249992428, -9.363379034771808662, -43.78125000204838102 ) ) ;
#13200=CARTESIAN_POINT ( 'NONE',  ( 9.999999999999998224, 0.000000000000000000, -90.87500000409677625 ) ) ;
#13202=CARTESIAN_POINT ( 'NONE',  ( -4.999999999999996447, 8.660254037844387298, -129.0000000000000000 ) ) ;
#13203=CARTESIAN_POINT ( 'NONE',  ( 10.81189881249999551, -6.242252689847874514, -138.1562500020484094 ) ) ;
#13204=LINE ( 'NONE', #23595, #17176 ) ;
#13205=CARTESIAN_POINT ( 'NONE',  ( 9.999999999999996447, -5.773502691896262640, -112.0000000040967763 ) ) ;
#13207=ORIENTED_EDGE ( 'NONE', *, *, #35723, .F. ) ;
#13210=CARTESIAN_POINT ( 'NONE',  ( -9.999999999999998224, 1.224646799147353059E-15, -34.62500000409676915 ) ) ;
#13211=CARTESIAN_POINT ( 'NONE',  ( -2.293366432827344421E-15, -12.48450537969573659, -162.4062500020483810 ) ) ;
#13212=CARTESIAN_POINT ( 'NONE',  ( 5.000000000000000000, 8.660254037844385522, -38.12500000409676915 ) ) ;
#13215=AXIS2_PLACEMENT_3D ( 'NONE', #2287, #38303, #28179 ) ;
#13216=CYLINDRICAL_SURFACE ( 'NONE', #34519, 9.999999999999998224 ) ;
#13217=CARTESIAN_POINT ( 'NONE',  ( 7.644554776091147741E-16, 12.48450537969573659, -163.1562500020484094 ) ) ;
#13218=CARTESIAN_POINT ( 'NONE',  ( 5.405949406249999534, 9.363379034771803333, -131.5937500020483810 ) ) ;
#13220=CARTESIAN_POINT ( 'NONE',  ( 10.00000000000011013, -5.773502691896197803, -195.6250000000000284 ) ) ;
#13222=ORIENTED_EDGE ( 'NONE', *, *, #12694, .F. ) ;
#13223=( BOUNDED_CURVE ( )  B_SPLINE_CURVE ( 2, ( #17751, #30947, #18786, #14510, #24696, #40842, #37627 ),
 .UNSPECIFIED., .F., .F. ) 
 B_SPLINE_CURVE_WITH_KNOTS ( ( 3, 2, 2, 3 ),
 ( 0.6231343283582090331, 0.6243781094527364184, 0.6256218905472638037, 0.6268656716417911889 ),
 .UNSPECIFIED. ) 
 CURVE ( )  GEOMETRIC_REPRESENTATION_ITEM ( )  RATIONAL_B_SPLINE_CURVE ( ( 0.9999999999999880096, 0.8660254037844506980, 1.000000000000000000, 0.8660254037844387076, 1.000000000000000000, 0.8660254037844267172, 1.000000000000011990 ) ) 
 REPRESENTATION_ITEM ( '' )  );
#13224=ADVANCED_FACE ( 'NONE', ( #23221 ), #17565, .T. ) ;
#13226=VECTOR ( 'NONE', #36020, 1000.000000000000000 ) ;
#13227=CARTESIAN_POINT ( 'NONE',  ( -5.405949406249996869, 9.363379034771805109, -67.03125000204838102 ) ) ;
#13228=ORIENTED_EDGE ( 'NONE', *, *, #1014, .T. ) ;
#13230=CARTESIAN_POINT ( 'NONE',  ( -5.405949406250003975, -9.363379034771801557, -115.8437500020483810 ) ) ;
#13231=ORIENTED_EDGE ( 'NONE', *, *, #6966, .T. ) ;
#13232=ORIENTED_EDGE ( 'NONE', *, *, #31490, .F. ) ;
#13233=CARTESIAN_POINT ( 'NONE',  ( -10.81189881249999729, 1.324075727343319199E-15, -20.09375000204835615 ) ) ;
#13234=CARTESIAN_POINT ( 'NONE',  ( 5.405949406249992428, -9.363379034771808662, -198.0937500020484094 ) ) ;
#13235=CARTESIAN_POINT ( 'NONE',  ( 5.405949406249992428, -9.363379034771808662, -49.59375000204838102 ) ) ;
#13236=DIRECTION ( 'NONE',  ( -0.000000000000000000, -0.000000000000000000, 1.000000000000000000 ) ) ;
#13238=EDGE_CURVE ( 'NONE', #29783, #38740, #10579, .T. ) ;
#13239=CARTESIAN_POINT ( 'NONE',  ( -10.81189881249999729, 1.324075727343319199E-15, -182.0937500020483810 ) ) ;
#13240=CARTESIAN_POINT ( 'NONE',  ( 7.644554776091147741E-16, 12.48450537969573659, -165.9687500020483810 ) ) ;
#13243=CARTESIAN_POINT ( 'NONE',  ( -5.000000000000003553, -8.660254037844383745, -118.3750000040967905 ) ) ;
#13244=CARTESIAN_POINT ( 'NONE',  ( 7.070501591499376803E-16, 11.54700538379251284, -193.6250000000000284 ) ) ;
#13246=CARTESIAN_POINT ( 'NONE',  ( 7.644554776091147741E-16, 12.48450537969573659, -95.46875000204839523 ) ) ;
#13248=CARTESIAN_POINT ( 'NONE',  ( 10.81189881249999907, 6.242252689847868297, -68.90625000204839523 ) ) ;
#13249=CARTESIAN_POINT ( 'NONE',  ( -9.999999999998969713, -5.773502691896847949, -5.624999999999936939 ) ) ;
#13252=CARTESIAN_POINT ( 'NONE',  ( -2.293366432827344421E-15, -12.48450537969573659, -163.9062500020483810 ) ) ;
#13254=CARTESIAN_POINT ( 'NONE',  ( 9.999999999999998224, 0.000000000000000000, -135.8750000040967905 ) ) ;
#13256=ORIENTED_EDGE ( 'NONE', *, *, #18175, .T. ) ;
#13260=CARTESIAN_POINT ( 'NONE',  ( -10.81189881249999907, -6.242252689847864744, -195.6562500020484094 ) ) ;
#13261=DIRECTION ( 'NONE',  ( -1.000000000000000000, -0.000000000000000000, -0.000000000000000000 ) ) ;
#13263=ORIENTED_EDGE ( 'NONE', *, *, #5249, .T. ) ;
#13264=CARTESIAN_POINT ( 'NONE',  ( -4.999999999999996447, 8.660254037844387298, -56.99999999999996447 ) ) ;
#13266=CARTESIAN_POINT ( 'NONE',  ( 9.999999999999998224, 0.000000000000000000, -62.37500000409676204 ) ) ;
#13269=CARTESIAN_POINT ( 'NONE',  ( -2.293366432827344421E-15, -12.48450537969573659, -61.90625000204838813 ) ) ;
#13270=( BOUNDED_CURVE ( )  B_SPLINE_CURVE ( 2, ( #1361, #14493, #37824, #8266, #21849, #31364, #8482 ),
 .UNSPECIFIED., .F., .F. ) 
 B_SPLINE_CURVE_WITH_KNOTS ( ( 3, 2, 2, 3 ),
 ( 0.6865671641791046831, 0.6878109452736320684, 0.6890547263681594536, 0.6902985074626868389 ),
 .UNSPECIFIED. ) 
 CURVE ( )  GEOMETRIC_REPRESENTATION_ITEM ( )  RATIONAL_B_SPLINE_CURVE ( ( 0.9999999999999761302, 0.8660254037844625774, 1.000000000000000000, 0.8660254037844387076, 1.000000000000000000, 0.8660254037844148378, 1.000000000000023981 ) ) 
 REPRESENTATION_ITEM ( '' )  );
#13273=CARTESIAN_POINT ( 'NONE',  ( -10.81189881249999907, -6.242252689847864744, -183.6562500020483810 ) ) ;
#13275=CARTESIAN_POINT ( 'NONE',  ( 9.999999999999866773, -5.773502691896336358, -172.0000000040967620 ) ) ;
#13276=CYLINDRICAL_SURFACE ( 'NONE', #2053, 9.999999999999998224 ) ;
#13277=EDGE_CURVE ( 'NONE', #15678, #33229, #35452, .T. ) ;
#13278=CARTESIAN_POINT ( 'NONE',  ( 9.999999999999998224, 0.000000000000000000, -48.49999999999998579 ) ) ;
#13279=CYLINDRICAL_SURFACE ( 'NONE', #18303, 9.999999999999998224 ) ;
#13280=ADVANCED_FACE ( 'NONE', ( #39605 ), #10039, .T. ) ;
#13281=( BOUNDED_CURVE ( )  B_SPLINE_CURVE ( 2, ( #11762, #31864, #34670, #18888, #11542, #8338, #25376 ),
 .UNSPECIFIED., .F., .F. ) 
 B_SPLINE_CURVE_WITH_KNOTS ( ( 3, 2, 2, 3 ),
 ( 0.6044776119402985870, 0.6057213930348259723, 0.6069651741293533576, 0.6082089552238807428 ),
 .UNSPECIFIED. ) 
 CURVE ( )  GEOMETRIC_REPRESENTATION_ITEM ( )  RATIONAL_B_SPLINE_CURVE ( ( 0.9999999999999880096, 0.8660254037844506980, 1.000000000000000000, 0.8660254037844387076, 1.000000000000000000, 0.8660254037844267172, 1.000000000000011990 ) ) 
 REPRESENTATION_ITEM ( '' )  );
#13282=CARTESIAN_POINT ( 'NONE',  ( 9.999999999999996447, -5.773502691896262640, -165.6250000000000000 ) ) ;
#13283=DIRECTION ( 'NONE',  ( 1.000000000000000000, 0.000000000000000000, 0.000000000000000000 ) ) ;
#13285=CARTESIAN_POINT ( 'NONE',  ( 10.81189881249999551, -6.242252689847874514, -91.65625000204838102 ) ) ;
#13287=DIRECTION ( 'NONE',  ( 1.000000000000000000, 0.000000000000000000, 0.000000000000000000 ) ) ;
#13289=VERTEX_POINT ( 'NONE', #41526 ) ;
#13290=ORIENTED_EDGE ( 'NONE', *, *, #11679, .T. ) ;
#13291=CARTESIAN_POINT ( 'NONE',  ( -10.81189881249999729, 6.242252689847871849, -30.71875000204834905 ) ) ;
#13292=CARTESIAN_POINT ( 'NONE',  ( 10.81189881249999551, -6.242252689847874514, -21.15625000204836681 ) ) ;
#13293=CARTESIAN_POINT ( 'NONE',  ( -2.293366432827344421E-15, -12.48450537969573659, -70.71875000204839523 ) ) ;
#13294=CARTESIAN_POINT ( 'NONE',  ( 4.999999999999992006, -8.660254037844389075, -173.6250000040968189 ) ) ;
#13295=CARTESIAN_POINT ( 'NONE',  ( 10.81189881249999551, -6.242252689847874514, -194.9687500020484094 ) ) ;
#13296=CARTESIAN_POINT ( 'NONE',  ( 7.644554776091147741E-16, 12.48450537969573659, -147.9687500020484094 ) ) ;
#13297=ADVANCED_FACE ( 'NONE', ( #11741 ), #17786, .T. ) ;
#13301=CARTESIAN_POINT ( 'NONE',  ( 4.999999999999992006, -8.660254037844389075, -5.625000004096769146 ) ) ;
#13302=CARTESIAN_POINT ( 'NONE',  ( 4.999999999999992006, -8.660254037844389075, -80.24999999999998579 ) ) ;
#13303=CARTESIAN_POINT ( 'NONE',  ( 5.405949406249992428, -9.363379034771808662, -121.5937500020483952 ) ) ;
#13304=CARTESIAN_POINT ( 'NONE',  ( -9.999999999999998224, 1.224646799147353059E-15, -103.2500000000000000 ) ) ;
#13305=CARTESIAN_POINT ( 'NONE',  ( 10.81189881249999907, 6.242252689847868297, -88.40625000204839523 ) ) ;
#13306=CARTESIAN_POINT ( 'NONE',  ( -5.405949406249996869, 9.363379034771805109, -104.3437500020483810 ) ) ;
#13309=CARTESIAN_POINT ( 'NONE',  ( -4.999999999999996447, 8.660254037844387298, -165.3750000040967905 ) ) ;
#13310=DIRECTION ( 'NONE',  ( -0.000000000000000000, -0.000000000000000000, 1.000000000000000000 ) ) ;
#13314=CARTESIAN_POINT ( 'NONE',  ( -9.999999999999742428, -5.773502691896402084, -157.1250000000000000 ) ) ;
#13316=DIRECTION ( 'NONE',  ( 1.000000000000000000, 0.000000000000000000, 0.000000000000000000 ) ) ;
#13318=CARTESIAN_POINT ( 'NONE',  ( -9.999999999999998224, 1.224646799147353059E-15, -80.74999999999998579 ) ) ;
#13320=CARTESIAN_POINT ( 'NONE',  ( 9.999999999999998224, 0.000000000000000000, -89.37500000409677625 ) ) ;
#13323=CARTESIAN_POINT ( 'NONE',  ( 5.405949406249999534, 9.363379034771803333, -82.28125000204838102 ) ) ;
#13324=ORIENTED_EDGE ( 'NONE', *, *, #21485, .T. ) ;
#13326=DIRECTION ( 'NONE',  ( -0.000000000000000000, -0.000000000000000000, 1.000000000000000000 ) ) ;
#13329=CARTESIAN_POINT ( 'NONE',  ( 9.999999999999998224, 0.000000000000000000, -6.499999999999977796 ) ) ;
#13330=CARTESIAN_POINT ( 'NONE',  ( 9.999999999999998224, 0.000000000000000000, -144.5000000000000000 ) ) ;
#13331=CARTESIAN_POINT ( 'NONE',  ( 9.999999999999998224, 0.000000000000000000, -31.99999999999997158 ) ) ;
#13333=CARTESIAN_POINT ( 'NONE',  ( 4.999999999999992006, -8.660254037844389075, -191.2500000000000000 ) ) ;
#13335=CARTESIAN_POINT ( 'NONE',  ( -10.81189881249999729, 1.324075727343319199E-15, -119.2812500020483952 ) ) ;
#13336=ORIENTED_EDGE ( 'NONE', *, *, #431, .T. ) ;
#13337=CARTESIAN_POINT ( 'NONE',  ( 11.54700538379250396, 20.00000000000000711, 45.00000000000009237 ) ) ;
#13339=CARTESIAN_POINT ( 'NONE',  ( 5.405949406249992428, -9.363379034771808662, -46.78125000204838813 ) ) ;
#13341=EDGE_CURVE ( 'NONE', #21669, #22182, #34055, .T. ) ;
#13342=CARTESIAN_POINT ( 'NONE',  ( -5.405949406250003975, -9.363379034771801557, -91.84375000204838102 ) ) ;
#13343=CARTESIAN_POINT ( 'NONE',  ( 10.81189881249999551, -6.242252689847874514, -121.6562500020483952 ) ) ;
#13346=CARTESIAN_POINT ( 'NONE',  ( -9.999999999999227285, -5.773502691896698735, -112.1249999999999574 ) ) ;
#13347=CARTESIAN_POINT ( 'NONE',  ( 10.00000000000051159, -5.773502691895965988, -116.1249999999999716 ) ) ;
#13350=CARTESIAN_POINT ( 'NONE',  ( 10.81189881249999729, 0.000000000000000000, -128.8437500020484094 ) ) ;
#13352=CARTESIAN_POINT ( 'NONE',  ( -4.999999999999996447, 8.660254037844387298, -115.8750000040967905 ) ) ;
#13354=CARTESIAN_POINT ( 'NONE',  ( 9.999999999999996447, -5.773502691896262640, -190.0000000040968189 ) ) ;
#13356=CARTESIAN_POINT ( 'NONE',  ( -5.405949406249996869, 9.363379034771805109, -185.5312500020484094 ) ) ;
#13357=CARTESIAN_POINT ( 'NONE',  ( 5.000000000000000000, 8.660254037844385522, -6.625000004096770923 ) ) ;
#13361=CARTESIAN_POINT ( 'NONE',  ( -10.81189881249999729, 6.242252689847871849, -63.71875000204838102 ) ) ;
#13362=CARTESIAN_POINT ( 'NONE',  ( 5.405949406249999534, 9.363379034771803333, -49.09375000204838102 ) ) ;
#13364=CARTESIAN_POINT ( 'NONE',  ( 5.405949406249999534, 9.363379034771803333, -17.78125000204835970 ) ) ;
#13366=CARTESIAN_POINT ( 'NONE',  ( 9.999999999999998224, 0.000000000000000000, -158.3750000040967905 ) ) ;
#13368=CARTESIAN_POINT ( 'NONE',  ( -9.999999999999998224, 5.773502691896259087, -101.8749999999999858 ) ) ;
#13373=CARTESIAN_POINT ( 'NONE',  ( 10.81189881249999551, -6.242252689847874514, -118.6562500020483952 ) ) ;
#13374=VERTEX_POINT ( 'NONE', #15188 ) ;
#13380=CARTESIAN_POINT ( 'NONE',  ( -2.121150477449813534E-15, -11.54700538379251284, -36.87499999999996447 ) ) ;
#13381=CARTESIAN_POINT ( 'NONE',  ( -10.00000000000000000, -5.773502691896251982, -18.00000000409676559 ) ) ;
#13382=CARTESIAN_POINT ( 'NONE',  ( -10.81189881249999729, 1.324075727343319199E-15, -39.78125000204838102 ) ) ;
#13383=DIRECTION ( 'NONE',  ( -0.000000000000000000, -0.000000000000000000, 1.000000000000000000 ) ) ;
#13385=DIRECTION ( 'NONE',  ( -0.000000000000000000, -0.000000000000000000, 1.000000000000000000 ) ) ;
#13386=CARTESIAN_POINT ( 'NONE',  ( 10.81189881249999907, 6.242252689847868297, -142.4062500020484094 ) ) ;
#13388=ORIENTED_EDGE ( 'NONE', *, *, #39942, .T. ) ;
#13390=ORIENTED_EDGE ( 'NONE', *, *, #6442, .T. ) ;
#13391=ORIENTED_EDGE ( 'NONE', *, *, #40732, .T. ) ;
#13392=DIRECTION ( 'NONE',  ( -0.000000000000000000, -0.000000000000000000, 1.000000000000000000 ) ) ;
#13393=CARTESIAN_POINT ( 'NONE',  ( 10.81189881249999729, 0.000000000000000000, -172.3437500020484094 ) ) ;
#13394=CARTESIAN_POINT ( 'NONE',  ( -10.81189881249999907, -6.242252689847864744, -22.96875000204837747 ) ) ;
#13395=DIRECTION ( 'NONE',  ( -0.000000000000000000, -0.000000000000000000, 1.000000000000000000 ) ) ;
#13396=CARTESIAN_POINT ( 'NONE',  ( -5.405949406249996869, 9.363379034771805109, -152.3437500020483810 ) ) ;
#13397=CARTESIAN_POINT ( 'NONE',  ( 7.644554776091147741E-16, 12.48450537969573659, -143.4687500020483810 ) ) ;
#13399=CARTESIAN_POINT ( 'NONE',  ( -9.999999999999998224, 1.224646799147353059E-15, -22.24999999999996447 ) ) ;
#13402=CARTESIAN_POINT ( 'NONE',  ( -10.81189881249999729, 1.324075727343319199E-15, -6.593750002048370362 ) ) ;
#13405=CARTESIAN_POINT ( 'NONE',  ( -9.999999999999998224, 1.224646799147353059E-15, -182.7500000000000000 ) ) ;
#13407=CARTESIAN_POINT ( 'NONE',  ( -9.999999999999998224, 1.224646799147353059E-15, -99.12500000409677625 ) ) ;
#13408=CARTESIAN_POINT ( 'NONE',  ( 5.405949406249999534, 9.363379034771803333, -73.09375000204838102 ) ) ;
#13409=CARTESIAN_POINT ( 'NONE',  ( -10.81189881249999907, -6.242252689847864744, -41.15625000204836681 ) ) ;
#13411=CARTESIAN_POINT ( 'NONE',  ( 7.070501591499376803E-16, 11.54700538379251284, -57.12499999999997868 ) ) ;
#13413=CARTESIAN_POINT ( 'NONE',  ( 9.999999999999998224, 0.000000000000000000, -126.5000000000000000 ) ) ;
#13414=CARTESIAN_POINT ( 'NONE',  ( -5.405949406250003975, -9.363379034771801557, -137.0312500020484094 ) ) ;
#13415=CARTESIAN_POINT ( 'NONE',  ( 10.00000000000051159, -5.773502691895965988, -150.6250000000000000 ) ) ;
#13416=CARTESIAN_POINT ( 'NONE',  ( -5.000000000000003553, -8.660254037844383745, -115.3750000040967905 ) ) ;
#13421=CARTESIAN_POINT ( 'NONE',  ( 5.405949406249992428, -9.363379034771808662, -162.2812500020484094 ) ) ;
#13422=CARTESIAN_POINT ( 'NONE',  ( -10.00000000000000000, -5.773502691896251982, -43.50000000409675494 ) ) ;
#13425=CARTESIAN_POINT ( 'NONE',  ( -9.999999999999998224, 1.224646799147353059E-15, -73.24999999999998579 ) ) ;
#13426=CARTESIAN_POINT ( 'NONE',  ( -10.81189881249999729, 1.324075727343319199E-15, -161.2812500020484094 ) ) ;
#13427=CARTESIAN_POINT ( 'NONE',  ( 10.81189881249999551, -6.242252689847874514, -134.9687500020483810 ) ) ;
#13428=CARTESIAN_POINT ( 'NONE',  ( 9.999999999999998224, 0.000000000000000000, -31.99999999999997158 ) ) ;
#13430=VERTEX_POINT ( 'NONE', #34645 ) ;
#13431=CARTESIAN_POINT ( 'NONE',  ( -2.121150477449813534E-15, -11.54700538379251284, -30.87499999999995381 ) ) ;
#13432=CARTESIAN_POINT ( 'NONE',  ( 10.81189881249999907, 6.242252689847868297, -73.40625000204836681 ) ) ;
#13435=CARTESIAN_POINT ( 'NONE',  ( -10.81189881249999729, 1.324075727343319199E-15, -120.5937500020483952 ) ) ;
#13437=ORIENTED_EDGE ( 'NONE', *, *, #41440, .F. ) ;
#13438=VECTOR ( 'NONE', #23100, 1000.000000000000000 ) ;
#13439=CARTESIAN_POINT ( 'NONE',  ( 10.81189881249999729, 0.000000000000000000, -17.84375000204835260 ) ) ;
#13440=CARTESIAN_POINT ( 'NONE',  ( 7.644554776091147741E-16, 12.48450537969573659, -195.9687500020484094 ) ) ;
#13441=CARTESIAN_POINT ( 'NONE',  ( 5.405949406249999534, 9.363379034771803333, -44.59375000204837391 ) ) ;
#13442=CARTESIAN_POINT ( 'NONE',  ( 10.00000000000051159, -5.773502691895965988, -71.50000000409676204 ) ) ;
#13444=CARTESIAN_POINT ( 'NONE',  ( 10.81189881249999729, 6.242252689847867408, -178.2187500020484094 ) ) ;
#13445=AXIS2_PLACEMENT_3D ( 'NONE', #11056, #17315, #3962 ) ;
#13446=CARTESIAN_POINT ( 'NONE',  ( 5.405949406249992428, -9.363379034771808662, -168.0937500020484094 ) ) ;
#13449=CARTESIAN_POINT ( 'NONE',  ( 10.00000000000051159, -5.773502691895965988, -118.0000000040967763 ) ) ;
#13452=CARTESIAN_POINT ( 'NONE',  ( 5.405949406249999534, 9.363379034771803333, -95.59375000204838102 ) ) ;
#13453=DIRECTION ( 'NONE',  ( -0.000000000000000000, -0.000000000000000000, 1.000000000000000000 ) ) ;
#13454=CARTESIAN_POINT ( 'NONE',  ( -10.81189881249999729, 1.324075727343319199E-15, -69.78125000204838102 ) ) ;
#13456=ADVANCED_FACE ( 'NONE', ( #40871 ), #1411, .T. ) ;
#13458=CARTESIAN_POINT ( 'NONE',  ( -2.293366432827344421E-15, -12.48450537969573659, -124.9062500020483810 ) ) ;
#13459=CARTESIAN_POINT ( 'NONE',  ( 5.405949406249992428, -9.363379034771808662, -160.7812500020484094 ) ) ;
#13462=CARTESIAN_POINT ( 'NONE',  ( -2.121150477449813534E-15, -11.54700538379251284, -139.2500000040967905 ) ) ;
#13468=CARTESIAN_POINT ( 'NONE',  ( -10.81189881249999729, 6.242252689847871849, -188.4062500020484094 ) ) ;
#13472=CARTESIAN_POINT ( 'NONE',  ( 9.999999999999998224, 0.000000000000000000, -60.49999999999997158 ) ) ;
#13474=CARTESIAN_POINT ( 'NONE',  ( 7.070501591499377789E-16, 11.54700538379251284, -65.00000000409677625 ) ) ;
#13476=( BOUNDED_CURVE ( )  B_SPLINE_CURVE ( 2, ( #30035, #34715, #3915, #479, #13595, #688, #33695 ),
 .UNSPECIFIED., .F., .F. ) 
 B_SPLINE_CURVE_WITH_KNOTS ( ( 3, 2, 2, 3 ),
 ( 0.7014925373134330844, 0.7027363184079604697, 0.7039800995024877439, 0.7052238805970151292 ),
 .UNSPECIFIED. ) 
 CURVE ( )  GEOMETRIC_REPRESENTATION_ITEM ( )  RATIONAL_B_SPLINE_CURVE ( ( 0.9999999999999761302, 0.8660254037844625774, 1.000000000000000000, 0.8660254037844387076, 1.000000000000000000, 0.8660254037844148378, 1.000000000000023981 ) ) 
 REPRESENTATION_ITEM ( '' )  );
#13479=AXIS2_PLACEMENT_3D ( 'NONE', #21434, #40627, #8070 ) ;
#13480=CARTESIAN_POINT ( 'NONE',  ( -10.81189881249999729, 6.242252689847871849, -56.40625000204837391 ) ) ;
#13484=DIRECTION ( 'NONE',  ( 1.000000000000000000, 0.000000000000000000, 0.000000000000000000 ) ) ;
#13485=CARTESIAN_POINT ( 'NONE',  ( -2.293366432827344421E-15, -12.48450537969573659, -187.9062500020484094 ) ) ;
#13487=CARTESIAN_POINT ( 'NONE',  ( -9.999999999999998224, 1.224646799147353059E-15, -172.6250000040968189 ) ) ;
#13492=CARTESIAN_POINT ( 'NONE',  ( -4.999999999999996447, 8.660254037844387298, -169.5000000000000000 ) ) ;
#13493=DIRECTION ( 'NONE',  ( -0.000000000000000000, -0.000000000000000000, 1.000000000000000000 ) ) ;
#13494=CARTESIAN_POINT ( 'NONE',  ( -10.81189881249999729, 6.242252689847871849, -96.90625000204838102 ) ) ;
#13495=VERTEX_POINT ( 'NONE', #24726 ) ;
#13496=CARTESIAN_POINT ( 'NONE',  ( -9.999999999999998224, 1.224646799147353059E-15, -181.6250000040967905 ) ) ;
#13498=VERTEX_POINT ( 'NONE', #8097 ) ;
#13500=CARTESIAN_POINT ( 'NONE',  ( -10.81189881249999729, 1.324075727343319199E-15, -36.59375000204836681 ) ) ;
#13501=CARTESIAN_POINT ( 'NONE',  ( 10.81189881249999907, 6.242252689847868297, -19.40625000204837747 ) ) ;
#13502=CARTESIAN_POINT ( 'NONE',  ( 10.81189881249999729, 0.000000000000000000, -74.84375000204838102 ) ) ;
#13503=CARTESIAN_POINT ( 'NONE',  ( -4.999999999999996447, 8.660254037844387298, -104.9999999999999858 ) ) ;
#13504=CARTESIAN_POINT ( 'NONE',  ( 10.81189881249999729, 0.000000000000000000, -196.3437500020484094 ) ) ;
#13505=CARTESIAN_POINT ( 'NONE',  ( -10.81189881249999907, -6.242252689847864744, -148.9687500020484094 ) ) ;
#13506=VECTOR ( 'NONE', #7961, 1000.000000000000000 ) ;
#13509=CARTESIAN_POINT ( 'NONE',  ( -9.999999999999998224, 5.773502691896259087, -0.2500000040967449433 ) ) ;
#13510=CARTESIAN_POINT ( 'NONE',  ( -11.54700538379251817, 15.00000000000010836, 49.99999999999998579 ) ) ;
#13511=CARTESIAN_POINT ( 'NONE',  ( 5.405949406249992428, -9.363379034771808662, -120.0937500020483952 ) ) ;
#13513=CARTESIAN_POINT ( 'NONE',  ( 10.81189881249999729, 0.000000000000000000, -91.53125000204838102 ) ) ;
#13515=CARTESIAN_POINT ( 'NONE',  ( 5.405949406249999534, 9.363379034771803333, -109.0937500020483810 ) ) ;
#13518=CARTESIAN_POINT ( 'NONE',  ( 5.000000000000000000, 8.660254037844385522, -159.6250000040967905 ) ) ;
#13519=EDGE_CURVE ( 'NONE', #22340, #11539, #24298, .T. ) ;
#13520=( BOUNDED_CURVE ( )  B_SPLINE_CURVE ( 2, ( #27885, #33725, #37805, #7600, #34583, #5013, #30277 ),
 .UNSPECIFIED., .F., .F. ) 
 B_SPLINE_CURVE_WITH_KNOTS ( ( 3, 2, 2, 3 ),
 ( 0.4067164179104478250, 0.4079601990049751548, 0.4092039800995025400, 0.4104477611940299253 ),
 .UNSPECIFIED. ) 
 CURVE ( )  GEOMETRIC_REPRESENTATION_ITEM ( )  RATIONAL_B_SPLINE_CURVE ( ( 0.9999999999999940048, 0.8660254037844447028, 1.000000000000000000, 0.8660254037844387076, 1.000000000000000000, 0.8660254037844327124, 1.000000000000005995 ) ) 
 REPRESENTATION_ITEM ( '' )  );
#13524=CARTESIAN_POINT ( 'NONE',  ( -5.000000000000003553, -8.660254037844383745, -190.0000000000000000 ) ) ;
#13527=CARTESIAN_POINT ( 'NONE',  ( -9.999999999999998224, 5.773502691896259087, -82.37499999999998579 ) ) ;
#13529=CARTESIAN_POINT ( 'NONE',  ( -9.999999999999998224, 1.224646799147353059E-15, -87.12500000409677625 ) ) ;
#13530=CARTESIAN_POINT ( 'NONE',  ( 11.54700538379253416, -19.99999999999999289, 49.99999999999998579 ) ) ;
#13533=CARTESIAN_POINT ( 'NONE',  ( -10.81189881249999729, -6.242252689847864744, -81.65625000204839523 ) ) ;
#13534=VERTEX_POINT ( 'NONE', #4639 ) ;
#13537=CARTESIAN_POINT ( 'NONE',  ( -10.00000000000051337, 5.773502691895962435, -47.87499999999995737 ) ) ;
#13540=CARTESIAN_POINT ( 'NONE',  ( -4.999999999999996447, 8.660254037844387298, -5.999999999999977796 ) ) ;
#13541=CARTESIAN_POINT ( 'NONE',  ( 9.999999999999998224, 0.000000000000000000, -147.5000000000000000 ) ) ;
#13542=CARTESIAN_POINT ( 'NONE',  ( -10.00000000000051337, 5.773502691895962435, -45.25000000409674783 ) ) ;
#13546=CARTESIAN_POINT ( 'NONE',  ( -9.999999999999998224, 5.773502691896259087, -193.3750000000000000 ) ) ;
#13548=CARTESIAN_POINT ( 'NONE',  ( 7.644554776091147741E-16, 12.48450537969573659, -116.6562500020483952 ) ) ;
#13550=CARTESIAN_POINT ( 'NONE',  ( 10.00000000000051159, -5.773502691895965988, -74.50000000409676204 ) ) ;
#13552=CARTESIAN_POINT ( 'NONE',  ( -10.81189881249999907, -6.242252689847864744, -45.65625000204837391 ) ) ;
#13554=CARTESIAN_POINT ( 'NONE',  ( 7.644554776091147741E-16, 12.48450537969573659, -98.46875000204839523 ) ) ;
#13555=CARTESIAN_POINT ( 'NONE',  ( 7.644554776091147741E-16, 12.48450537969573659, -125.6562500020483810 ) ) ;
#13556=ORIENTED_EDGE ( 'NONE', *, *, #11329, .T. ) ;
#13557=LINE ( 'NONE', #3444, #28028 ) ;
#13560=CARTESIAN_POINT ( 'NONE',  ( 5.405949406249992428, -9.363379034771808662, -135.0937500020483810 ) ) ;
#13564=CARTESIAN_POINT ( 'NONE',  ( 10.00000000000000000, 5.773502691896255534, -183.7500000040968189 ) ) ;
#13566=CARTESIAN_POINT ( 'NONE',  ( -5.405949406250003975, -9.363379034771801557, -174.5312500020484094 ) ) ;
#13567=CARTESIAN_POINT ( 'NONE',  ( 7.070501591499376803E-16, 11.54700538379251284, -3.124999999999950262 ) ) ;
#13568=CARTESIAN_POINT ( 'NONE',  ( 9.999999999999548805, 5.773502691896515771, -181.8749999999999716 ) ) ;
#13570=CARTESIAN_POINT ( 'NONE',  ( -10.81189881249999729, 6.242252689847871849, -59.21875000204836681 ) ) ;
#13571=CARTESIAN_POINT ( 'NONE',  ( -5.405949406249996869, 9.363379034771805109, -39.84375000204837391 ) ) ;
#13573=CARTESIAN_POINT ( 'NONE',  ( -10.81189881249999729, 1.324075727343319199E-15, -18.78125000204835970 ) ) ;
#13577=CARTESIAN_POINT ( 'NONE',  ( 5.000000000000000000, 8.660254037844385522, -103.7500000000000000 ) ) ;
#13579=CARTESIAN_POINT ( 'NONE',  ( 9.999999999999479527, 5.773502691896553074, -119.2500000040967620 ) ) ;
#13582=CARTESIAN_POINT ( 'NONE',  ( 10.81189881249999729, 6.242252689847867408, -110.9062500020483952 ) ) ;
#13584=CYLINDRICAL_SURFACE ( 'NONE', #27923, 9.999999999999998224 ) ;
#13588=EDGE_LOOP ( 'NONE', ( #24252, #15623, #16044, #38313 ) ) ;
#13589=CARTESIAN_POINT ( 'NONE',  ( 9.999999999999998224, 0.000000000000000000, -36.49999999999997868 ) ) ;
#13591=CARTESIAN_POINT ( 'NONE',  ( 4.999999999999992006, -8.660254037844389075, -20.62500000409675494 ) ) ;
#13592=CARTESIAN_POINT ( 'NONE',  ( -5.405949406250003975, -9.363379034771801557, -32.03125000204837391 ) ) ;
#13593=CARTESIAN_POINT ( 'NONE',  ( -9.999999999999998224, 1.224646799147353059E-15, -34.62500000409676915 ) ) ;
#13595=CARTESIAN_POINT ( 'NONE',  ( -4.999999999999996447, 8.660254037844387298, -57.37500000409676204 ) ) ;
#13596=CARTESIAN_POINT ( 'NONE',  ( 10.81189881249999907, 6.242252689847868297, -139.4062500020484094 ) ) ;
#13597=( BOUNDED_CURVE ( )  B_SPLINE_CURVE ( 2, ( #17963, #31163, #1594, #27266, #28137, #34397, #40621 ),
 .UNSPECIFIED., .F., .F. ) 
 B_SPLINE_CURVE_WITH_KNOTS ( ( 3, 2, 2, 3 ),
 ( 0.05223880597014930738, 0.05348258706467667184, 0.05472636815920402936, 0.05597014925373139382 ),
 .UNSPECIFIED. ) 
 CURVE ( )  GEOMETRIC_REPRESENTATION_ITEM ( )  RATIONAL_B_SPLINE_CURVE ( ( 0.9999999999999940048, 0.8660254037844447028, 1.000000000000000000, 0.8660254037844387076, 1.000000000000000000, 0.8660254037844334896, 1.000000000000005329 ) ) 
 REPRESENTATION_ITEM ( '' )  );
#13599=ORIENTED_EDGE ( 'NONE', *, *, #25277, .F. ) ;
#13601=CARTESIAN_POINT ( 'NONE',  ( 9.999999999999998224, 0.000000000000000000, -162.5000000000000000 ) ) ;
#13602=CARTESIAN_POINT ( 'NONE',  ( 7.644554776091147741E-16, 12.48450537969573659, -176.4687500020483810 ) ) ;
#13604=CARTESIAN_POINT ( 'NONE',  ( -10.81189881249999729, 6.242252689847871849, -21.71875000204837036 ) ) ;
#13605=CARTESIAN_POINT ( 'NONE',  ( 9.999999999999998224, 0.000000000000000000, -123.5000000000000000 ) ) ;
#13607=AXIS2_PLACEMENT_3D ( 'NONE', #4457, #17600, #10921 ) ;
#13608=CARTESIAN_POINT ( 'NONE',  ( -2.293366432827344421E-15, -12.48450537969573659, -157.7187500020483810 ) ) ;
#13610=CARTESIAN_POINT ( 'NONE',  ( -2.293366432827344421E-15, -12.48450537969573659, -133.7187500020483810 ) ) ;
#13615=CARTESIAN_POINT ( 'NONE',  ( 5.405949406249992428, -9.363379034771808662, -10.59375000204834727 ) ) ;
#13618=CARTESIAN_POINT ( 'NONE',  ( 9.999999999999998224, 0.000000000000000000, -177.8750000040967905 ) ) ;
#13621=CARTESIAN_POINT ( 'NONE',  ( -10.81189881249999729, -6.242252689847864744, -81.46875000204838102 ) ) ;
#13622=CARTESIAN_POINT ( 'NONE',  ( -10.81189881249999729, 6.242252689847871849, -71.21875000204839523 ) ) ;
#13623=CARTESIAN_POINT ( 'NONE',  ( 7.644554776091147741E-16, 12.48450537969573659, -43.15625000204838102 ) ) ;
#13626=CARTESIAN_POINT ( 'NONE',  ( 4.999999999999992006, -8.660254037844389075, -129.7499999999999716 ) ) ;
#13627=CARTESIAN_POINT ( 'NONE',  ( -10.81189881249999729, 6.242252689847871849, -140.4062500020484094 ) ) ;
#13628=LINE ( 'NONE', #39335, #37178 ) ;
#13630=CARTESIAN_POINT ( 'NONE',  ( 7.644554776091147741E-16, 12.48450537969573659, -17.65625000204836681 ) ) ;
#13635=CARTESIAN_POINT ( 'NONE',  ( 9.999999999999998224, 0.000000000000000000, -45.87500000409677625 ) ) ;
#13636=DIRECTION ( 'NONE',  ( 1.000000000000000000, 0.000000000000000000, 0.000000000000000000 ) ) ;
#13638=( BOUNDED_CURVE ( )  B_SPLINE_CURVE ( 2, ( #9720, #19642, #12727, #25924, #32826, #6701, #19853 ),
 .UNSPECIFIED., .F., .F. ) 
 B_SPLINE_CURVE_WITH_KNOTS ( ( 3, 2, 2, 3 ),
 ( 0.8507462686567166532, 0.8519900497512440385, 0.8532338308457714238, 0.8544776119402988090 ),
 .UNSPECIFIED. ) 
 CURVE ( )  GEOMETRIC_REPRESENTATION_ITEM ( )  RATIONAL_B_SPLINE_CURVE ( ( 0.9999999999999761302, 0.8660254037844625774, 1.000000000000000000, 0.8660254037844387076, 1.000000000000000000, 0.8660254037844028474, 1.000000000000035971 ) ) 
 REPRESENTATION_ITEM ( '' )  );
#13639=CARTESIAN_POINT ( 'NONE',  ( -9.999999999999998224, 1.224646799147353059E-15, -194.7500000000000000 ) ) ;
#13640=CARTESIAN_POINT ( 'NONE',  ( 7.644554776091147741E-16, 12.48450537969573659, -160.1562500020484094 ) ) ;
#13641=CARTESIAN_POINT ( 'NONE',  ( 5.405949406249992428, -9.363379034771808662, -135.0937500020483810 ) ) ;
#13643=CARTESIAN_POINT ( 'NONE',  ( 9.999999999999479527, 5.773502691896553074, -151.8749999999999716 ) ) ;
#13647=EDGE_CURVE ( 'NONE', #3490, #6420, #13597, .T. ) ;
#13648=CARTESIAN_POINT ( 'NONE',  ( -5.405949406250003975, -9.363379034771801557, -62.03125000204837391 ) ) ;
#13649=ORIENTED_EDGE ( 'NONE', *, *, #17359, .T. ) ;
#13651=CARTESIAN_POINT ( 'NONE',  ( 5.405949406249999534, 9.363379034771803333, -118.0937500020483810 ) ) ;
#13653=CARTESIAN_POINT ( 'NONE',  ( -10.81189881249999729, 1.324075727343319199E-15, -24.59375000204835970 ) ) ;
#13654=CARTESIAN_POINT ( 'NONE',  ( -2.293366432827344421E-15, -12.48450537969573659, -198.2187500020484379 ) ) ;
#13655=CARTESIAN_POINT ( 'NONE',  ( 5.405949406249999534, 9.363379034771803333, -49.09375000204838102 ) ) ;
#13657=CARTESIAN_POINT ( 'NONE',  ( -10.00000000000025580, 5.773502691896109873, -151.7500000040967336 ) ) ;
#13658=CARTESIAN_POINT ( 'NONE',  ( 7.644554776091147741E-16, 12.48450537969573659, -180.9687500020484094 ) ) ;
#13659=CARTESIAN_POINT ( 'NONE',  ( -10.81189881249999907, -6.242252689847864744, -160.9687500020484094 ) ) ;
#13662=CARTESIAN_POINT ( 'NONE',  ( -9.999999999999998224, 1.224646799147353059E-15, -200.0000000000000000 ) ) ;
#13664=CARTESIAN_POINT ( 'NONE',  ( -10.81189881249999729, 6.242252689847871849, -98.21875000204838102 ) ) ;
#13665=EDGE_CURVE ( 'NONE', #10245, #39524, #5944, .T. ) ;
#13666=CARTESIAN_POINT ( 'NONE',  ( 5.000000000000000000, 8.660254037844385522, -34.74999999999997868 ) ) ;
#13667=CARTESIAN_POINT ( 'NONE',  ( -5.405949406250003975, -9.363379034771801557, -69.53125000204838102 ) ) ;
#13668=CARTESIAN_POINT ( 'NONE',  ( -9.999999999999998224, 1.224646799147353059E-15, -81.12500000409677625 ) ) ;
#13670=CARTESIAN_POINT ( 'NONE',  ( 5.405949406249992428, -9.363379034771808662, -120.2812500020483952 ) ) ;
#13672=CARTESIAN_POINT ( 'NONE',  ( 5.405949406249992428, -9.363379034771808662, -159.2812500020484094 ) ) ;
#13674=CARTESIAN_POINT ( 'NONE',  ( 10.00000000000000000, 5.773502691896255534, -138.7500000040967905 ) ) ;
#13680=CARTESIAN_POINT ( 'NONE',  ( 10.81189881249999907, 6.242252689847868297, -187.4062500020484379 ) ) ;
#13683=CARTESIAN_POINT ( 'NONE',  ( -5.000000000000003553, -8.660254037844383745, -54.99999999999996447 ) ) ;
#13685=CARTESIAN_POINT ( 'NONE',  ( -4.999999999999996447, 8.660254037844387298, -67.87500000409677625 ) ) ;
#13688=CARTESIAN_POINT ( 'NONE',  ( 10.81189881249999729, 0.000000000000000000, -60.03125000204836681 ) ) ;
#13691=CARTESIAN_POINT ( 'NONE',  ( -8.675003188131697129, -4.974413003141673784, -0.0003472602639886801512 ) ) ;
#13692=CARTESIAN_POINT ( 'NONE',  ( -2.293366432827344421E-15, -12.48450537969573659, -181.9062500020483810 ) ) ;
#13694=LINE ( 'NONE', #23230, #37308 ) ;
#13696=CARTESIAN_POINT ( 'NONE',  ( -10.00000000000038547, 5.773502691896036154, -154.3749999999999716 ) ) ;
#13697=FACE_OUTER_BOUND ( 'NONE', #14935, .T. ) ;
#13698=LINE ( 'NONE', #10475, #29645 ) ;
#13699=CARTESIAN_POINT ( 'NONE',  ( 10.81189881249999907, 6.242252689847868297, -91.40625000204836681 ) ) ;
#13701=CARTESIAN_POINT ( 'NONE',  ( 0.000000000000000000, 0.000000000000000000, -200.0000000000000000 ) ) ;
#13702=EDGE_CURVE ( 'NONE', #26311, #3284, #21427, .T. ) ;
#13703=CYLINDRICAL_SURFACE ( 'NONE', #24797, 9.999999999999998224 ) ;
#13704=VERTEX_POINT ( 'NONE', #20783 ) ;
#13705=VERTEX_POINT ( 'NONE', #14071 ) ;
#13706=CARTESIAN_POINT ( 'NONE',  ( -5.405949406250003975, -9.363379034771801557, -22.84375000204835615 ) ) ;
#13707=CARTESIAN_POINT ( 'NONE',  ( -10.81189881249999729, 6.242252689847871849, -20.40625000204837747 ) ) ;
#13709=AXIS2_PLACEMENT_3D ( 'NONE', #16523, #793, #36182 ) ;
#13710=CARTESIAN_POINT ( 'NONE',  ( -5.405949406249996869, 9.363379034771805109, -69.84375000204836681 ) ) ;
#13711=CARTESIAN_POINT ( 'NONE',  ( -9.999999999999998224, 1.224646799147353059E-15, -104.7499999999999858 ) ) ;
#13713=CARTESIAN_POINT ( 'NONE',  ( 7.644554776091147741E-16, 12.48450537969573659, -192.9687500020483810 ) ) ;
#13714=CARTESIAN_POINT ( 'NONE',  ( -5.405949406249996869, 9.363379034771805109, -147.8437500020483810 ) ) ;
#13715=VECTOR ( 'NONE', #21338, 1000.000000000000000 ) ;
#13717=CARTESIAN_POINT ( 'NONE',  ( 7.070501591499377789E-16, 11.54700538379251284, -6.500000004096742501 ) ) ;
#13719=CARTESIAN_POINT ( 'NONE',  ( -5.405949406249996869, 9.363379034771805109, -123.8437500020483952 ) ) ;
#13720=DIRECTION ( 'NONE',  ( -0.000000000000000000, -0.000000000000000000, 1.000000000000000000 ) ) ;
#13721=CARTESIAN_POINT ( 'NONE',  ( -2.293366432827344421E-15, -12.48450537969573659, -91.90625000204838102 ) ) ;
#13722=CARTESIAN_POINT ( 'NONE',  ( -10.81189881249999729, -6.242252689847864744, -96.46875000204839523 ) ) ;
#13723=( BOUNDED_CURVE ( )  B_SPLINE_CURVE ( 2, ( #6553, #3111, #30084, #26622, #19282, #19918, #22535 ),
 .UNSPECIFIED., .F., .F. ) 
 B_SPLINE_CURVE_WITH_KNOTS ( ( 3, 2, 2, 3 ),
 ( 0.7686567164179105571, 0.7699004975124379424, 0.7711442786069654387, 0.7723880597014927130 ),
 .UNSPECIFIED. ) 
 CURVE ( )  GEOMETRIC_REPRESENTATION_ITEM ( )  RATIONAL_B_SPLINE_CURVE ( ( 0.9999999999999880096, 0.8660254037844506980, 1.000000000000000000, 0.8660254037844387076, 1.000000000000000000, 0.8660254037844148378, 1.000000000000023981 ) ) 
 REPRESENTATION_ITEM ( '' )  );
#13726=CARTESIAN_POINT ( 'NONE',  ( -5.000000000000003553, -8.660254037844383745, -164.8750000040967905 ) ) ;
#13729=CARTESIAN_POINT ( 'NONE',  ( -10.00000000000031797, 5.773502691896072569, -184.3750000000000568 ) ) ;
#13730=DIRECTION ( 'NONE',  ( -0.000000000000000000, -0.000000000000000000, 1.000000000000000000 ) ) ;
#13731=CARTESIAN_POINT ( 'NONE',  ( 4.999999999999992006, -8.660254037844389075, -108.7499999999999858 ) ) ;
#13733=CARTESIAN_POINT ( 'NONE',  ( -9.999999999999998224, 1.224646799147353059E-15, -79.24999999999998579 ) ) ;
#13735=CARTESIAN_POINT ( 'NONE',  ( 9.999999999999998224, 0.000000000000000000, -92.37500000409677625 ) ) ;
#13736=CARTESIAN_POINT ( 'NONE',  ( 5.000000000000000000, 8.660254037844385522, -168.6250000040967905 ) ) ;
#13738=CARTESIAN_POINT ( 'NONE',  ( 10.81189881249999729, 6.242252689847867408, -85.40625000204836681 ) ) ;
#13742=EDGE_LOOP ( 'NONE', ( #2129, #3961, #13391, #2182 ) ) ;
#13743=CARTESIAN_POINT ( 'NONE',  ( -10.00000000000000000, -5.773502691896251982, -10.12499999999998401 ) ) ;
#13746=CARTESIAN_POINT ( 'NONE',  ( 4.999999999999992006, -8.660254037844389075, -147.7500000000000000 ) ) ;
#13747=CARTESIAN_POINT ( 'NONE',  ( 9.999999999999998224, 0.000000000000000000, -132.5000000000000000 ) ) ;
#13749=CARTESIAN_POINT ( 'NONE',  ( -4.999999999999996447, 8.660254037844387298, -192.0000000000000000 ) ) ;
#13750=EDGE_CURVE ( 'NONE', #26724, #6996, #28253, .T. ) ;
#13751=CARTESIAN_POINT ( 'NONE',  ( -10.00000000000051337, 5.773502691895962435, -95.87499999999998579 ) ) ;
#13752=CARTESIAN_POINT ( 'NONE',  ( -10.81189881249999729, 1.324075727343319199E-15, -117.7812500020483952 ) ) ;
#13753=ORIENTED_EDGE ( 'NONE', *, *, #6261, .F. ) ;
#13754=CARTESIAN_POINT ( 'NONE',  ( 9.999999999998969713, 5.773502691896851502, -36.75000000409674072 ) ) ;
#13755=EDGE_CURVE ( 'NONE', #23881, #15716, #4178, .T. ) ;
#13758=ORIENTED_EDGE ( 'NONE', *, *, #8291, .F. ) ;
#13759=( BOUNDED_CURVE ( )  B_SPLINE_CURVE ( 2, ( #15518, #2601, #39047, #6044, #6468, #12496, #32383 ),
 .UNSPECIFIED., .F., .F. ) 
 B_SPLINE_CURVE_WITH_KNOTS ( ( 3, 2, 2, 3 ),
 ( 0.9291044776119405935, 0.9303482587064679787, 0.9315920398009952530, 0.9328358208955226383 ),
 .UNSPECIFIED. ) 
 CURVE ( )  GEOMETRIC_REPRESENTATION_ITEM ( )  RATIONAL_B_SPLINE_CURVE ( ( 0.9999999999999641398, 0.8660254037844745678, 1.000000000000000000, 0.8660254037844387076, 1.000000000000000000, 0.8660254037844148378, 1.000000000000023981 ) ) 
 REPRESENTATION_ITEM ( '' )  );
#13760=CARTESIAN_POINT ( 'NONE',  ( -5.405949406249996869, 9.363379034771805109, -43.03125000204838102 ) ) ;
#13762=CARTESIAN_POINT ( 'NONE',  ( 10.81189881249999551, -6.242252689847874514, -94.46875000204838102 ) ) ;
#13763=CARTESIAN_POINT ( 'NONE',  ( 10.81189881249999729, 0.000000000000000000, -124.5312500020483952 ) ) ;
#13764=ORIENTED_EDGE ( 'NONE', *, *, #34132, .T. ) ;
#13766=CARTESIAN_POINT ( 'NONE',  ( 0.000000000000000000, 0.000000000000000000, -200.0000000000000000 ) ) ;
#13767=( BOUNDED_CURVE ( )  B_SPLINE_CURVE ( 2, ( #15642, #39171, #8979, #12615, #25389, #22563, #42397 ),
 .UNSPECIFIED., .F., .F. ) 
 B_SPLINE_CURVE_WITH_KNOTS ( ( 3, 2, 2, 3 ),
 ( 0.7500000000000001110, 0.7512437810945274963, 0.7524875621890549926, 0.7537313432835822669 ),
 .UNSPECIFIED. ) 
 CURVE ( )  GEOMETRIC_REPRESENTATION_ITEM ( )  RATIONAL_B_SPLINE_CURVE ( ( 0.9999999999999880096, 0.8660254037844506980, 1.000000000000000000, 0.8660254037844387076, 1.000000000000000000, 0.8660254037844148378, 1.000000000000023981 ) ) 
 REPRESENTATION_ITEM ( '' )  );
#13769=DIRECTION ( 'NONE',  ( -0.000000000000000000, -0.000000000000000000, 1.000000000000000000 ) ) ;
#13770=AXIS2_PLACEMENT_3D ( 'NONE', #15200, #18231, #8330 ) ;
#13771=EDGE_CURVE ( 'NONE', #3969, #26141, #32669, .T. ) ;
#13772=CARTESIAN_POINT ( 'NONE',  ( 10.81189881249999551, -6.242252689847874514, -134.9687500020483810 ) ) ;
#13774=FACE_OUTER_BOUND ( 'NONE', #42682, .T. ) ;
#13776=CARTESIAN_POINT ( 'NONE',  ( -9.999999999999998224, 1.224646799147353059E-15, -184.6250000040967905 ) ) ;
#13778=CARTESIAN_POINT ( 'NONE',  ( -5.405949406249996869, 9.363379034771805109, -181.0312500020483810 ) ) ;
#13779=( BOUNDED_CURVE ( )  B_SPLINE_CURVE ( 2, ( #3237, #29994, #16363, #32602, #440, #3445, #26327 ),
 .UNSPECIFIED., .F., .F. ) 
 B_SPLINE_CURVE_WITH_KNOTS ( ( 3, 2, 2, 3 ),
 ( 0.3619402985074628432, 0.3631840796019901729, 0.3644278606965175027, 0.3656716417910448325 ),
 .UNSPECIFIED. ) 
 CURVE ( )  GEOMETRIC_REPRESENTATION_ITEM ( )  RATIONAL_B_SPLINE_CURVE ( ( 0.9999999999999820144, 0.8660254037844566932, 1.000000000000000000, 0.8660254037844387076, 1.000000000000000000, 0.8660254037844327124, 1.000000000000005995 ) ) 
 REPRESENTATION_ITEM ( '' )  );
#13780=CARTESIAN_POINT ( 'NONE',  ( 9.999999999999998224, 0.000000000000000000, -3.499999999999975131 ) ) ;
#13783=CARTESIAN_POINT ( 'NONE',  ( 5.405949406249992428, -9.363379034771808662, -61.59375000204836681 ) ) ;
#13784=CARTESIAN_POINT ( 'NONE',  ( 10.81189881249999907, 6.242252689847868297, -41.71875000204835260 ) ) ;
#13786=CARTESIAN_POINT ( 'NONE',  ( -10.81189881249999729, 6.242252689847871849, -20.40625000204837747 ) ) ;
#13790=CARTESIAN_POINT ( 'NONE',  ( 9.999999999999996447, -5.773502691896262640, -105.6249999999999858 ) ) ;
#13792=EDGE_CURVE ( 'NONE', #12497, #6518, #30942, .T. ) ;
#13793=CARTESIAN_POINT ( 'NONE',  ( -2.121150477449813534E-15, -11.54700538379251284, -168.8750000000000000 ) ) ;
#13796=CARTESIAN_POINT ( 'NONE',  ( -10.81189881249999729, 6.242252689847871849, -110.4062500020483810 ) ) ;
#13799=CARTESIAN_POINT ( 'NONE',  ( -2.121150477449813534E-15, -11.54700538379251284, -194.7500000040967905 ) ) ;
#13802=CARTESIAN_POINT ( 'NONE',  ( 7.070501591499377789E-16, 11.54700538379251284, -34.62499999999995737 ) ) ;
#13803=CARTESIAN_POINT ( 'NONE',  ( -5.405949406249996869, 9.363379034771805109, -34.03125000204837391 ) ) ;
#13804=CARTESIAN_POINT ( 'NONE',  ( 9.999999999999998224, 0.000000000000000000, -200.0000000000000000 ) ) ;
#13806=CARTESIAN_POINT ( 'NONE',  ( 5.000000000000000000, 8.660254037844385522, -161.1250000040967905 ) ) ;
#13808=CARTESIAN_POINT ( 'NONE',  ( -10.81189881249999729, 6.242252689847871849, -143.4062500020484094 ) ) ;
#13809=CARTESIAN_POINT ( 'NONE',  ( 4.999999999999992006, -8.660254037844389075, -119.6250000040967905 ) ) ;
#13810=EDGE_LOOP ( 'NONE', ( #1431, #16491, #12027, #23516 ) ) ;
#13811=ADVANCED_FACE ( 'NONE', ( #11277 ), #32017, .T. ) ;
#13812=EDGE_CURVE ( 'NONE', #23552, #22272, #29292, .T. ) ;
#13814=CARTESIAN_POINT ( 'NONE',  ( 7.070501591499376803E-16, 11.54700538379251284, -114.1249999999999858 ) ) ;
#13815=DIRECTION ( 'NONE',  ( 1.000000000000000000, 1.502314598737160017E-16, 0.000000000000000000 ) ) ;
#13816=CARTESIAN_POINT ( 'NONE',  ( -10.81189881249999907, -6.242252689847864744, -165.4687500020484094 ) ) ;
#13818=CARTESIAN_POINT ( 'NONE',  ( -2.293366432827344421E-15, -12.48450537969573659, -15.21875000204835615 ) ) ;
#13819=DIRECTION ( 'NONE',  ( -0.000000000000000000, -0.000000000000000000, 1.000000000000000000 ) ) ;
#13820=CARTESIAN_POINT ( 'NONE',  ( 5.405949406249992428, -9.363379034771808662, -156.0937500020483810 ) ) ;
#13821=CARTESIAN_POINT ( 'NONE',  ( 10.81189881249999551, -6.242252689847874514, -139.4687500020483810 ) ) ;
#13826=CARTESIAN_POINT ( 'NONE',  ( -10.81189881249999907, -6.242252689847864744, -7.968750002048352599 ) ) ;
#13829=CARTESIAN_POINT ( 'NONE',  ( -10.00000000000102496, 5.773502691895664007, -63.25000000409674783 ) ) ;
#13833=CARTESIAN_POINT ( 'NONE',  ( 5.405949406249992428, -9.363379034771808662, -87.09375000204836681 ) ) ;
#13834=CARTESIAN_POINT ( 'NONE',  ( -2.293366432827344421E-15, -12.48450537969573659, -63.21875000204839523 ) ) ;
#13836=CARTESIAN_POINT ( 'NONE',  ( -5.405949406250003975, -9.363379034771801557, -42.53125000204838102 ) ) ;
#13838=CARTESIAN_POINT ( 'NONE',  ( -9.999999999999998224, 1.224646799147353059E-15, -200.0000000000000000 ) ) ;
#13840=CARTESIAN_POINT ( 'NONE',  ( -9.999999999999998224, 1.224646799147353059E-15, -128.7499999999999716 ) ) ;
#13841=CARTESIAN_POINT ( 'NONE',  ( 10.81189881249999729, 0.000000000000000000, -129.0312500020484094 ) ) ;
#13842=CARTESIAN_POINT ( 'NONE',  ( 0.000000000000000000, 0.000000000000000000, -200.0000000000000000 ) ) ;
#13844=CARTESIAN_POINT ( 'NONE',  ( -10.81189881249999729, 6.242252689847871849, -17.40625000204838457 ) ) ;
#13845=ORIENTED_EDGE ( 'NONE', *, *, #3429, .T. ) ;
#13848=DIRECTION ( 'NONE',  ( -0.000000000000000000, -0.000000000000000000, 1.000000000000000000 ) ) ;
#13849=CARTESIAN_POINT ( 'NONE',  ( -5.000000000000003553, -8.660254037844383745, -41.87500000409677625 ) ) ;
#13850=( BOUNDED_CURVE ( )  B_SPLINE_CURVE ( 2, ( #545, #26226, #33133, #9601, #22988, #2929, #40010 ),
 .UNSPECIFIED., .F., .F. ) 
 B_SPLINE_CURVE_WITH_KNOTS ( ( 3, 2, 2, 3 ),
 ( 0.05223880597014930738, 0.05348258706467667184, 0.05472636815920402936, 0.05597014925373139382 ),
 .UNSPECIFIED. ) 
 CURVE ( )  GEOMETRIC_REPRESENTATION_ITEM ( )  RATIONAL_B_SPLINE_CURVE ( ( 0.9999999999999940048, 0.8660254037844447028, 1.000000000000000000, 0.8660254037844387076, 1.000000000000000000, 0.8660254037844334896, 1.000000000000005329 ) ) 
 REPRESENTATION_ITEM ( '' )  );
#13851=CARTESIAN_POINT ( 'NONE',  ( -9.999999999999998224, 1.224646799147353059E-15, -58.62500000409676204 ) ) ;
#13853=CARTESIAN_POINT ( 'NONE',  ( 9.999999999999998224, 0.000000000000000000, -24.49999999999996447 ) ) ;
#13854=CARTESIAN_POINT ( 'NONE',  ( -10.81189881249999729, 6.242252689847871849, -156.9062500020483810 ) ) ;
#13855=CARTESIAN_POINT ( 'NONE',  ( -10.81189881249999907, -6.242252689847864744, -132.4687500020483810 ) ) ;
#13856=DIRECTION ( 'NONE',  ( -0.000000000000000000, -0.000000000000000000, 1.000000000000000000 ) ) ;
#13857=ORIENTED_EDGE ( 'NONE', *, *, #5970, .F. ) ;
#13861=CARTESIAN_POINT ( 'NONE',  ( 7.644554776091147741E-16, 12.48450537969573659, -62.65625000204838813 ) ) ;
#13862=ORIENTED_EDGE ( 'NONE', *, *, #36084, .T. ) ;
#13864=CARTESIAN_POINT ( 'NONE',  ( -10.81189881249999907, -6.242252689847864744, -111.4687500020483810 ) ) ;
#13865=VERTEX_POINT ( 'NONE', #35674 ) ;
#13866=CARTESIAN_POINT ( 'NONE',  ( -5.405949406249996869, 9.363379034771805109, -18.84375000204835260 ) ) ;
#13867=CARTESIAN_POINT ( 'NONE',  ( -2.293366432827344421E-15, -12.48450537969573659, -189.2187500020484094 ) ) ;
#13868=CARTESIAN_POINT ( 'NONE',  ( 7.644554776091147741E-16, 12.48450537969573659, -45.96875000204837391 ) ) ;
#13869=ADVANCED_FACE ( 'NONE', ( #22079 ), #28984, .T. ) ;
#13870=CARTESIAN_POINT ( 'NONE',  ( -6.596080831067816064, -7.719381798922900551, 5.985441654281310823E-15 ) ) ;
#13872=CARTESIAN_POINT ( 'NONE',  ( 10.81189881249999729, 6.242252689847867408, -179.7187500020484094 ) ) ;
#13873=CARTESIAN_POINT ( 'NONE',  ( 10.81189881249999907, 6.242252689847868297, -163.2187500020483810 ) ) ;
#13876=CARTESIAN_POINT ( 'NONE',  ( -9.999999999999998224, 1.224646799147353059E-15, -94.24999999999998579 ) ) ;
#13878=CARTESIAN_POINT ( 'NONE',  ( 5.405949406249992428, -9.363379034771808662, -93.09375000204838102 ) ) ;
#13880=CARTESIAN_POINT ( 'NONE',  ( -5.405949406250003975, -9.363379034771801557, -66.53125000204838102 ) ) ;
#13881=LINE ( 'NONE', #17125, #14351 ) ;
#13883=CARTESIAN_POINT ( 'NONE',  ( 10.81189881249999729, 0.000000000000000000, -126.0312500020483952 ) ) ;
#13884=CARTESIAN_POINT ( 'NONE',  ( 10.81189881249999729, 0.000000000000000000, -162.0312500020484094 ) ) ;
#13886=CARTESIAN_POINT ( 'NONE',  ( -5.000000000000003553, -8.660254037844383745, -136.3750000040967905 ) ) ;
#13888=EDGE_CURVE ( 'NONE', #7309, #5998, #25237, .T. ) ;
#13890=( BOUNDED_CURVE ( )  B_SPLINE_CURVE ( 2, ( #39800, #13249, #10232, #6583, #38966, #7014, #36150 ),
 .UNSPECIFIED., .F., .F. ) 
 B_SPLINE_CURVE_WITH_KNOTS ( ( 3, 2, 2, 3 ),
 ( 0.9664179104477613746, 0.9676616915422887599, 0.9689054726368161452, 0.9701492537313435305 ),
 .UNSPECIFIED. ) 
 CURVE ( )  GEOMETRIC_REPRESENTATION_ITEM ( )  RATIONAL_B_SPLINE_CURVE ( ( 0.9999999999999761302, 0.8660254037844625774, 1.000000000000000000, 0.8660254037844387076, 1.000000000000000000, 0.8660254037844148378, 1.000000000000023981 ) ) 
 REPRESENTATION_ITEM ( '' )  );
#13891=EDGE_LOOP ( 'NONE', ( #16572, #5713, #22697, #41266 ) ) ;
#13894=CARTESIAN_POINT ( 'NONE',  ( -5.405949406250003975, -9.363379034771801557, -186.5312500020484094 ) ) ;
#13896=ORIENTED_EDGE ( 'NONE', *, *, #41795, .T. ) ;
#13897=CARTESIAN_POINT ( 'NONE',  ( 4.999999999999992006, -8.660254037844389075, -53.24999999999996447 ) ) ;
#13899=CARTESIAN_POINT ( 'NONE',  ( 5.000000000000000000, 8.660254037844385522, -65.12500000409676204 ) ) ;
#13900=CARTESIAN_POINT ( 'NONE',  ( -9.999999999999998224, 1.224646799147353059E-15, -200.0000000000000000 ) ) ;
#13901=LINE ( 'NONE', #4427, #22927 ) ;
#13903=CARTESIAN_POINT ( 'NONE',  ( 5.405949406249992428, -9.363379034771808662, -55.78125000204836681 ) ) ;
#13906=DIRECTION ( 'NONE',  ( -0.000000000000000000, -0.000000000000000000, 1.000000000000000000 ) ) ;
#13907=CARTESIAN_POINT ( 'NONE',  ( 5.405949406249992428, -9.363379034771808662, -174.2812500020484094 ) ) ;
#13909=CARTESIAN_POINT ( 'NONE',  ( 9.999999999999998224, 0.000000000000000000, -87.49999999999998579 ) ) ;
#13912=DIRECTION ( 'NONE',  ( -0.000000000000000000, -0.000000000000000000, 1.000000000000000000 ) ) ;
#13913=CARTESIAN_POINT ( 'NONE',  ( 10.81189881249999729, 0.000000000000000000, -85.53125000204838102 ) ) ;
#13914=ORIENTED_EDGE ( 'NONE', *, *, #25430, .F. ) ;
#13917=ORIENTED_EDGE ( 'NONE', *, *, #30576, .T. ) ;
#13918=AXIS2_PLACEMENT_3D ( 'NONE', #1058, #40519, #28033 ) ;
#13919=EDGE_CURVE ( 'NONE', #26513, #3816, #6104, .T. ) ;
#13920=CARTESIAN_POINT ( 'NONE',  ( -5.405949406250003975, -9.363379034771801557, -30.34375000204836326 ) ) ;
#13921=CARTESIAN_POINT ( 'NONE',  ( 10.81189881249999729, 0.000000000000000000, -10.53125000204835260 ) ) ;
#13923=CARTESIAN_POINT ( 'NONE',  ( -2.293366432827344421E-15, -12.48450537969573659, -67.71875000204838102 ) ) ;
#13924=CARTESIAN_POINT ( 'NONE',  ( -9.999999999999998224, 1.224646799147353059E-15, -92.74999999999998579 ) ) ;
#13926=CARTESIAN_POINT ( 'NONE',  ( -10.81189881249999907, -6.242252689847864744, -184.9687500020484094 ) ) ;
#13927=CARTESIAN_POINT ( 'NONE',  ( 5.405949406249992428, -9.363379034771808662, -0.09375000204836503315 ) ) ;
#13931=CARTESIAN_POINT ( 'NONE',  ( -9.999999999999998224, 1.224646799147353059E-15, -200.0000000000000000 ) ) ;
#13932=CARTESIAN_POINT ( 'NONE',  ( -10.81189881249999729, 1.324075727343319199E-15, -123.5937500020483952 ) ) ;
#13934=CARTESIAN_POINT ( 'NONE',  ( 10.81189881249999907, 6.242252689847868297, -94.40625000204836681 ) ) ;
#13935=CARTESIAN_POINT ( 'NONE',  ( -10.81189881249999729, 1.324075727343319199E-15, -96.59375000204838102 ) ) ;
#13936=EDGE_CURVE ( 'NONE', #4873, #21320, #42122, .T. ) ;
#13939=CARTESIAN_POINT ( 'NONE',  ( -5.000000000000003553, -8.660254037844383745, -158.8750000040967905 ) ) ;
#13945=DIRECTION ( 'NONE',  ( 1.000000000000000000, 0.000000000000000000, 0.000000000000000000 ) ) ;
#13946=CARTESIAN_POINT ( 'NONE',  ( 10.00000000000000000, 5.773502691896255534, -75.37499999999998579 ) ) ;
#13948=CARTESIAN_POINT ( 'NONE',  ( -2.121150477449813534E-15, -11.54700538379251284, -92.75000000409677625 ) ) ;
#13949=CARTESIAN_POINT ( 'NONE',  ( -4.999999999999996447, 8.660254037844387298, -168.3750000040967905 ) ) ;
#13951=CARTESIAN_POINT ( 'NONE',  ( -5.405949406249996869, 9.363379034771805109, -86.53125000204838102 ) ) ;
#13953=CARTESIAN_POINT ( 'NONE',  ( 5.000000000000000000, 8.660254037844385522, -19.74999999999996092 ) ) ;
#13956=CARTESIAN_POINT ( 'NONE',  ( -9.999999999999998224, 1.224646799147353059E-15, -7.249999999999978684 ) ) ;
#13958=CARTESIAN_POINT ( 'NONE',  ( -10.81189881249999729, 6.242252689847871849, -9.718750002048361480 ) ) ;
#13959=CARTESIAN_POINT ( 'NONE',  ( 9.999999999999998224, 0.000000000000000000, -45.87500000409677625 ) ) ;
#13961=CARTESIAN_POINT ( 'NONE',  ( -10.81189881249999729, 1.324075727343319199E-15, -134.2812500020483810 ) ) ;
#13962=CARTESIAN_POINT ( 'NONE',  ( -9.999999999999998224, 5.773502691896259087, -187.3750000000000000 ) ) ;
#13963=CARTESIAN_POINT ( 'NONE',  ( 10.00000000000031619, -5.773502691896077010, -184.0000000040967905 ) ) ;
#13964=CARTESIAN_POINT ( 'NONE',  ( 5.405949406249999534, 9.363379034771803333, -107.7812500020483810 ) ) ;
#13965=ORIENTED_EDGE ( 'NONE', *, *, #15257, .T. ) ;
#13966=CYLINDRICAL_SURFACE ( 'NONE', #29669, 9.999999999999998224 ) ;
#13968=ORIENTED_EDGE ( 'NONE', *, *, #109, .T. ) ;
#13969=CARTESIAN_POINT ( 'NONE',  ( -10.81189881249999729, 1.324075727343319199E-15, -48.78125000204838813 ) ) ;
#13971=CARTESIAN_POINT ( 'NONE',  ( -10.81189881249999729, 1.324075727343319199E-15, -92.09375000204838102 ) ) ;
#13972=CARTESIAN_POINT ( 'NONE',  ( 5.405949406249999534, 9.363379034771803333, -122.7812500020483952 ) ) ;
#13974=CARTESIAN_POINT ( 'NONE',  ( 7.644554776091147741E-16, 12.48450537969573659, -192.9687500020484094 ) ) ;
#13976=CARTESIAN_POINT ( 'NONE',  ( -10.81189881249999729, -6.242252689847864744, -126.4687500020483810 ) ) ;
#13978=CARTESIAN_POINT ( 'NONE',  ( 0.000000000000000000, 0.000000000000000000, -200.0000000000000000 ) ) ;
#13980=CARTESIAN_POINT ( 'NONE',  ( -9.999999999999998224, 5.773502691896259087, -186.2500000040967905 ) ) ;
#13982=CARTESIAN_POINT ( 'NONE',  ( 10.81189881249999551, -6.242252689847874514, -177.1562500020484094 ) ) ;
#13983=CARTESIAN_POINT ( 'NONE',  ( 9.999999999999998224, 0.000000000000000000, -171.5000000000000000 ) ) ;
#13986=CARTESIAN_POINT ( 'NONE',  ( -10.81189881249999729, -6.242252689847864744, -49.96875000204835970 ) ) ;
#13987=CARTESIAN_POINT ( 'NONE',  ( 10.81189881249999907, 6.242252689847868297, -40.21875000204835970 ) ) ;
#13989=CARTESIAN_POINT ( 'NONE',  ( 5.405949406249992428, -9.363379034771808662, -10.78125000204835438 ) ) ;
#13993=ADVANCED_FACE ( 'NONE', ( #12554 ), #22499, .T. ) ;
#13994=CARTESIAN_POINT ( 'NONE',  ( -9.999999999999998224, 5.773502691896259087, -107.8749999999999858 ) ) ;
#14000=CARTESIAN_POINT ( 'NONE',  ( -10.81189881249999729, 1.324075727343319199E-15, -105.7812500020483810 ) ) ;
#14002=CARTESIAN_POINT ( 'NONE',  ( -10.00000000000025580, 5.773502691896109873, -160.3750000000000000 ) ) ;
#14004=DIRECTION ( 'NONE',  ( 1.000000000000000000, 0.000000000000000000, 0.000000000000000000 ) ) ;
#14006=VERTEX_POINT ( 'NONE', #42331 ) ;
#14007=CARTESIAN_POINT ( 'NONE',  ( 9.999999999999998224, 0.000000000000000000, -34.99999999999997868 ) ) ;
#14008=CARTESIAN_POINT ( 'NONE',  ( -10.81189881249999729, 1.324075727343319199E-15, -36.78125000204837391 ) ) ;
#14009=LINE ( 'NONE', #9945, #39354 ) ;
#14011=( BOUNDED_CURVE ( )  B_SPLINE_CURVE ( 2, ( #10745, #23508, #9030, #20252, #638, #13550, #3437 ),
 .UNSPECIFIED., .F., .F. ) 
 B_SPLINE_CURVE_WITH_KNOTS ( ( 3, 2, 2, 3 ),
 ( 0.6156716417910449435, 0.6169154228855723288, 0.6181592039800996030, 0.6194029850746269883 ),
 .UNSPECIFIED. ) 
 CURVE ( )  GEOMETRIC_REPRESENTATION_ITEM ( )  RATIONAL_B_SPLINE_CURVE ( ( 0.9999999999999761302, 0.8660254037844625774, 1.000000000000000000, 0.8660254037844387076, 1.000000000000000000, 0.8660254037844267172, 1.000000000000011990 ) ) 
 REPRESENTATION_ITEM ( '' )  );
#14012=CARTESIAN_POINT ( 'NONE',  ( -9.999999999999998224, 1.224646799147353059E-15, -160.6250000040967905 ) ) ;
#14013=CARTESIAN_POINT ( 'NONE',  ( 10.81189881249999551, -6.242252689847874514, -141.1562500020484094 ) ) ;
#14015=VERTEX_POINT ( 'NONE', #12761 ) ;
#14016=( BOUNDED_CURVE ( )  B_SPLINE_CURVE ( 2, ( #14404, #37088, #34729, #40739, #17864, #30840, #4295 ),
 .UNSPECIFIED., .F., .F. ) 
 B_SPLINE_CURVE_WITH_KNOTS ( ( 3, 2, 2, 3 ),
 ( 0.1268656716417910224, 0.1281094527363183799, 0.1293532338308457652, 0.1305970149253731227 ),
 .UNSPECIFIED. ) 
 CURVE ( )  GEOMETRIC_REPRESENTATION_ITEM ( )  RATIONAL_B_SPLINE_CURVE ( ( 1.000000000000003109, 0.8660254037844358210, 1.000000000000000000, 0.8660254037844387076, 1.000000000000000000, 0.8660254037844387076, 1.000000000000000000 ) ) 
 REPRESENTATION_ITEM ( '' )  );
#14017=VERTEX_POINT ( 'NONE', #8707 ) ;
#14019=DIRECTION ( 'NONE',  ( -0.000000000000000000, -0.000000000000000000, 1.000000000000000000 ) ) ;
#14020=CARTESIAN_POINT ( 'NONE',  ( -10.81189881249999729, 1.324075727343319199E-15, -165.5937500020484094 ) ) ;
#14022=CARTESIAN_POINT ( 'NONE',  ( -5.405949406249996869, 9.363379034771805109, -14.34375000204834905 ) ) ;
#14024=CARTESIAN_POINT ( 'NONE',  ( 10.81189881249999551, -6.242252689847874514, -145.4687500020484094 ) ) ;
#14025=CARTESIAN_POINT ( 'NONE',  ( -5.405949406249996869, 9.363379034771805109, -134.3437500020484094 ) ) ;
#14026=CARTESIAN_POINT ( 'NONE',  ( -10.81189881249999907, -6.242252689847864744, -102.6562500020483952 ) ) ;
#14030=CARTESIAN_POINT ( 'NONE',  ( 10.81189881249999729, 0.000000000000000000, -11.84375000204834727 ) ) ;
#14032=CARTESIAN_POINT ( 'NONE',  ( -2.121150477449813534E-15, -11.54700538379251284, -54.87499999999997158 ) ) ;
#14033=CARTESIAN_POINT ( 'NONE',  ( 7.070501591499376803E-16, 11.54700538379251284, -5.000000004096767370 ) ) ;
#14036=CARTESIAN_POINT ( 'NONE',  ( -10.81189881249999729, 6.242252689847871849, -83.21875000204836681 ) ) ;
#14037=CARTESIAN_POINT ( 'NONE',  ( 10.81189881249999551, -6.242252689847874514, -62.96875000204838813 ) ) ;
#14039=CARTESIAN_POINT ( 'NONE',  ( 5.405949406249999534, 9.363379034771803333, -35.78125000204837391 ) ) ;
#14041=CARTESIAN_POINT ( 'NONE',  ( 9.999999999999998224, 0.000000000000000000, -186.5000000000000000 ) ) ;
#14043=EDGE_CURVE ( 'NONE', #42118, #37834, #38052, .T. ) ;
#14044=CARTESIAN_POINT ( 'NONE',  ( 4.999999999999992006, -8.660254037844389075, -131.2499999999999716 ) ) ;
#14045=CARTESIAN_POINT ( 'NONE',  ( -5.405949406250003975, -9.363379034771801557, -131.0312500020484094 ) ) ;
#14048=CARTESIAN_POINT ( 'NONE',  ( -2.293366432827344421E-15, -12.48450537969573659, -19.90625000204837747 ) ) ;
#14049=EDGE_CURVE ( 'NONE', #7881, #41377, #4549, .T. ) ;
#14055=CARTESIAN_POINT ( 'NONE',  ( -9.999999999999998224, 5.773502691896259087, -30.25000000409675849 ) ) ;
#14056=CARTESIAN_POINT ( 'NONE',  ( -9.999999999998456346, -5.773502691897145489, -58.50000000409673362 ) ) ;
#14059=FACE_OUTER_BOUND ( 'NONE', #29173, .T. ) ;
#14060=CARTESIAN_POINT ( 'NONE',  ( 10.81189881249999729, 0.000000000000000000, -151.5312500020484094 ) ) ;
#14061=CARTESIAN_POINT ( 'NONE',  ( 10.81189881249999729, 0.000000000000000000, -134.8437500020484094 ) ) ;
#14062=CARTESIAN_POINT ( 'NONE',  ( -9.999999999999998224, 1.224646799147353059E-15, -103.6250000040967763 ) ) ;
#14063=ORIENTED_EDGE ( 'NONE', *, *, #24260, .F. ) ;
#14065=ORIENTED_EDGE ( 'NONE', *, *, #6580, .T. ) ;
#14066=EDGE_CURVE ( 'NONE', #22153, #15045, #42544, .T. ) ;
#14067=ORIENTED_EDGE ( 'NONE', *, *, #18568, .F. ) ;
#14069=CARTESIAN_POINT ( 'NONE',  ( 10.81189881249999907, 6.242252689847868297, -109.2187500020483810 ) ) ;
#14071=CARTESIAN_POINT ( 'NONE',  ( -9.999999999999998224, 1.224646799147353059E-15, -131.7499999999999716 ) ) ;
#14072=CARTESIAN_POINT ( 'NONE',  ( -10.81189881249999907, -6.242252689847864744, -192.4687500020484094 ) ) ;
#14073=CARTESIAN_POINT ( 'NONE',  ( 7.644554776091147741E-16, 12.48450537969573659, -35.46875000204835260 ) ) ;
#14075=CYLINDRICAL_SURFACE ( 'NONE', #10052, 9.999999999999998224 ) ;
#14076=CARTESIAN_POINT ( 'NONE',  ( 5.405949406249992428, -9.363379034771808662, -178.5937500020484094 ) ) ;
#14077=CARTESIAN_POINT ( 'NONE',  ( 10.81189881249999729, 0.000000000000000000, -158.8437500020483810 ) ) ;
#14078=CARTESIAN_POINT ( 'NONE',  ( -9.999999999999804601, 5.773502691896371886, -178.3750000000000284 ) ) ;
#14081=CARTESIAN_POINT ( 'NONE',  ( 9.999999999999998224, 0.000000000000000000, -126.8750000040967905 ) ) ;
#14084=CARTESIAN_POINT ( 'NONE',  ( 10.81189881249999729, 0.000000000000000000, -92.84375000204838102 ) ) ;
#14085=CARTESIAN_POINT ( 'NONE',  ( -5.405949406249996869, 9.363379034771805109, -70.03125000204838102 ) ) ;
#14088=CARTESIAN_POINT ( 'NONE',  ( -5.405949406249996869, 9.363379034771805109, -121.0312500020483952 ) ) ;
#14089=CARTESIAN_POINT ( 'NONE',  ( 5.405949406249999534, 9.363379034771803333, -155.7812500020484094 ) ) ;
#14090=( BOUNDED_CURVE ( )  B_SPLINE_CURVE ( 2, ( #5050, #21873, #31602, #11934, #18196, #31387, #14948 ),
 .UNSPECIFIED., .F., .F. ) 
 B_SPLINE_CURVE_WITH_KNOTS ( ( 3, 2, 2, 3 ),
 ( 0.1492537313432835966, 0.1504975124378109819, 0.1517412935323383116, 0.1529850746268656692 ),
 .UNSPECIFIED. ) 
 CURVE ( )  GEOMETRIC_REPRESENTATION_ITEM ( )  RATIONAL_B_SPLINE_CURVE ( ( 0.9999999999999970024, 0.8660254037844417052, 1.000000000000000000, 0.8660254037844387076, 1.000000000000000000, 0.8660254037844387076, 1.000000000000000000 ) ) 
 REPRESENTATION_ITEM ( '' )  );
#14092=CARTESIAN_POINT ( 'NONE',  ( -5.000000000000003553, -8.660254037844383745, -131.8750000040967905 ) ) ;
#14094=EDGE_LOOP ( 'NONE', ( #2187, #21914, #19775, #30239 ) ) ;
#14098=CARTESIAN_POINT ( 'NONE',  ( 5.405949406249992428, -9.363379034771808662, -184.7812500020484094 ) ) ;
#14099=EDGE_LOOP ( 'NONE', ( #32225, #19559, #20891, #25578 ) ) ;
#14100=CARTESIAN_POINT ( 'NONE',  ( 9.999999999999996447, -5.773502691896262640, -47.12499999999996447 ) ) ;
#14102=AXIS2_PLACEMENT_3D ( 'NONE', #25416, #9423, #12224 ) ;
#14103=CARTESIAN_POINT ( 'NONE',  ( 7.070501591499377789E-16, 11.54700538379251284, -56.00000000409676915 ) ) ;
#14104=CARTESIAN_POINT ( 'NONE',  ( -9.999999999999998224, 1.224646799147353059E-15, -109.6250000040967763 ) ) ;
#14107=CARTESIAN_POINT ( 'NONE',  ( -10.81189881249999729, -6.242252689847864744, -63.65625000204837391 ) ) ;
#14110=CARTESIAN_POINT ( 'NONE',  ( -4.999999999999996447, 8.660254037844387298, -88.49999999999998579 ) ) ;
#14111=CARTESIAN_POINT ( 'NONE',  ( 7.644554776091147741E-16, 12.48450537969573659, -179.6562500020484094 ) ) ;
#14112=EDGE_CURVE ( 'NONE', #32436, #35302, #22931, .T. ) ;
#14115=CARTESIAN_POINT ( 'NONE',  ( 7.070501591499376803E-16, 11.54700538379251284, -198.1250000000000284 ) ) ;
#14117=CARTESIAN_POINT ( 'NONE',  ( -5.000000000000003553, -8.660254037844383745, -154.0000000000000000 ) ) ;
#14118=CARTESIAN_POINT ( 'NONE',  ( 11.54700538379250396, 20.00000000000000711, 0.000000000000000000 ) ) ;
#14119=CARTESIAN_POINT ( 'NONE',  ( -5.405949406249996869, 9.363379034771805109, -85.03125000204838102 ) ) ;
#14120=EDGE_LOOP ( 'NONE', ( #41156, #36022, #3283, #29879 ) ) ;
#14123=ORIENTED_EDGE ( 'NONE', *, *, #11142, .F. ) ;
#14124=ORIENTED_EDGE ( 'NONE', *, *, #29172, .F. ) ;
#14125=CARTESIAN_POINT ( 'NONE',  ( 5.405949406249992428, -9.363379034771808662, -40.59375000204837391 ) ) ;
#14126=CARTESIAN_POINT ( 'NONE',  ( 5.405949406249992428, -9.363379034771808662, -30.09375000204836326 ) ) ;
#14128=CARTESIAN_POINT ( 'NONE',  ( 7.644554776091147741E-16, 12.48450537969573659, -10.15625000204837924 ) ) ;
#14129=CARTESIAN_POINT ( 'NONE',  ( 7.644554776091147741E-16, 12.48450537969573659, -66.96875000204838102 ) ) ;
#14130=CARTESIAN_POINT ( 'NONE',  ( -10.00000000000012434, 5.773502691896184480, -163.7500000040967905 ) ) ;
#14132=CARTESIAN_POINT ( 'NONE',  ( 7.644554776091147741E-16, 12.48450537969573659, -182.4687500020484094 ) ) ;
#14135=CARTESIAN_POINT ( 'NONE',  ( 5.405949406249992428, -9.363379034771808662, -1.593750002048366365 ) ) ;
#14136=DIRECTION ( 'NONE',  ( -0.000000000000000000, -0.000000000000000000, 1.000000000000000000 ) ) ;
#14137=CARTESIAN_POINT ( 'NONE',  ( 10.00000000000154010, -5.773502691895370020, -20.50000000409673007 ) ) ;
#14138=FACE_OUTER_BOUND ( 'NONE', #9566, .T. ) ;
#14139=CARTESIAN_POINT ( 'NONE',  ( -5.405949406249996869, 9.363379034771805109, -116.3437500020483810 ) ) ;
#14140=DIRECTION ( 'NONE',  ( -0.000000000000000000, -0.000000000000000000, 1.000000000000000000 ) ) ;
#14141=CARTESIAN_POINT ( 'NONE',  ( -5.405949406249996869, 9.363379034771805109, -88.03125000204838102 ) ) ;
#14142=CARTESIAN_POINT ( 'NONE',  ( -10.81189881249999729, -6.242252689847864744, -99.46875000204838102 ) ) ;
#14146=CARTESIAN_POINT ( 'NONE',  ( -9.999999999999998224, 5.773502691896259087, -157.7500000040967905 ) ) ;
#14148=CIRCLE ( 'NONE', #6604, 9.999999999999998224 ) ;
#14154=CARTESIAN_POINT ( 'NONE',  ( -9.999999999999998224, 1.224646799147353059E-15, -184.6250000040967905 ) ) ;
#14155=CARTESIAN_POINT ( 'NONE',  ( 5.000000000000000000, 8.660254037844385522, -73.74999999999998579 ) ) ;
#14157=CARTESIAN_POINT ( 'NONE',  ( 7.070501591499377789E-16, 11.54700538379251284, -93.50000000409677625 ) ) ;
#14159=CARTESIAN_POINT ( 'NONE',  ( -5.000000000000003553, -8.660254037844383745, -172.0000000000000000 ) ) ;
#14161=CARTESIAN_POINT ( 'NONE',  ( -5.405949406250003975, -9.363379034771801557, -86.03125000204838102 ) ) ;
#14163=CARTESIAN_POINT ( 'NONE',  ( 10.00000000000000000, 5.773502691896255534, -168.3750000000000000 ) ) ;
#14166=CARTESIAN_POINT ( 'NONE',  ( -9.999999999999998224, 5.773502691896259087, -2.874999999999949374 ) ) ;
#14168=CARTESIAN_POINT ( 'NONE',  ( -10.81189881249999729, -6.242252689847864744, -12.46875000204837391 ) ) ;
#14169=DIRECTION ( 'NONE',  ( 1.000000000000000000, 0.000000000000000000, 0.000000000000000000 ) ) ;
#14171=CARTESIAN_POINT ( 'NONE',  ( -2.293366432827344421E-15, -12.48450537969573659, -127.9062500020483952 ) ) ;
#14172=CARTESIAN_POINT ( 'NONE',  ( -5.000000000000003553, -8.660254037844383745, -181.0000000000000000 ) ) ;
#14174=CARTESIAN_POINT ( 'NONE',  ( 5.405949406249999534, 9.363379034771803333, -109.2812500020483810 ) ) ;
#14175=ORIENTED_EDGE ( 'NONE', *, *, #15377, .F. ) ;
#14176=CARTESIAN_POINT ( 'NONE',  ( 9.999999999999998224, 0.000000000000000000, -39.87500000409676915 ) ) ;
#14178=AXIS2_PLACEMENT_3D ( 'NONE', #32601, #35413, #22447 ) ;
#14179=ORIENTED_EDGE ( 'NONE', *, *, #5896, .T. ) ;
#14181=CARTESIAN_POINT ( 'NONE',  ( -5.405949406250003975, -9.363379034771801557, -39.53125000204838102 ) ) ;
#14183=CARTESIAN_POINT ( 'NONE',  ( -2.293366432827344421E-15, -12.48450537969573659, -97.71875000204838102 ) ) ;
#14184=CARTESIAN_POINT ( 'NONE',  ( 0.000000000000000000, 0.000000000000000000, -200.0000000000000000 ) ) ;
#14186=CARTESIAN_POINT ( 'NONE',  ( -10.81189881249999729, 1.324075727343319199E-15, -195.5937500020484094 ) ) ;
#14189=CARTESIAN_POINT ( 'NONE',  ( 5.405949406249992428, -9.363379034771808662, -124.5937500020483952 ) ) ;
#14191=CARTESIAN_POINT ( 'NONE',  ( 5.405949406249999534, 9.363379034771803333, -5.781250002048377468 ) ) ;
#14194=CARTESIAN_POINT ( 'NONE',  ( -9.999999999999998224, 1.224646799147353059E-15, -186.1250000040967905 ) ) ;
#14196=CARTESIAN_POINT ( 'NONE',  ( 5.405949406249992428, -9.363379034771808662, -181.7812500020483810 ) ) ;
#14197=CARTESIAN_POINT ( 'NONE',  ( 4.999999999999992006, -8.660254037844389075, -107.2499999999999858 ) ) ;
#14200=CARTESIAN_POINT ( 'NONE',  ( -2.293366432827344421E-15, -12.48450537969573659, -54.21875000204838102 ) ) ;
#14201=CARTESIAN_POINT ( 'NONE',  ( -5.405949406249996869, 9.363379034771805109, -42.84375000204837391 ) ) ;
#14204=CARTESIAN_POINT ( 'NONE',  ( -10.81189881249999729, 6.242252689847871849, -8.406250002048372139 ) ) ;
#14206=CARTESIAN_POINT ( 'NONE',  ( -2.121150477449813534E-15, -11.54700538379251284, -124.2500000040967763 ) ) ;
#14208=CARTESIAN_POINT ( 'NONE',  ( -5.000000000000003553, -8.660254037844383745, -95.49999999999998579 ) ) ;
#14210=CARTESIAN_POINT ( 'NONE',  ( -10.00000000000000000, -5.773502691896251982, -117.0000000040967905 ) ) ;
#14214=CARTESIAN_POINT ( 'NONE',  ( 5.405949406249992428, -9.363379034771808662, -106.7812500020483810 ) ) ;
#14215=EDGE_LOOP ( 'NONE', ( #9487, #24639, #22003, #11533 ) ) ;
#14216=CARTESIAN_POINT ( 'NONE',  ( 5.000000000000000000, 8.660254037844385522, -8.125000004096744277 ) ) ;
#14219=CARTESIAN_POINT ( 'NONE',  ( 5.405949406249992428, -9.363379034771808662, -166.7812500020484094 ) ) ;
#14221=ORIENTED_EDGE ( 'NONE', *, *, #13665, .F. ) ;
#14222=CARTESIAN_POINT ( 'NONE',  ( 5.000000000000000000, 8.660254037844385522, -22.74999999999996447 ) ) ;
#14223=CARTESIAN_POINT ( 'NONE',  ( -2.293366432827344421E-15, -12.48450537969573659, -37.90625000204837391 ) ) ;
#14224=CARTESIAN_POINT ( 'NONE',  ( -10.00000000000000000, -5.773502691896251982, -164.6249999999999716 ) ) ;
#14225=CARTESIAN_POINT ( 'NONE',  ( 9.999999999999998224, 0.000000000000000000, -200.0000000000000000 ) ) ;
#14227=CARTESIAN_POINT ( 'NONE',  ( 5.405949406249992428, -9.363379034771808662, -132.2812500020483810 ) ) ;
#14228=CARTESIAN_POINT ( 'NONE',  ( 7.070501591499376803E-16, 11.54700538379251284, -75.50000000409677625 ) ) ;
#14229=CARTESIAN_POINT ( 'NONE',  ( 9.999999999999998224, 0.000000000000000000, -51.87500000409675494 ) ) ;
#14230=ORIENTED_EDGE ( 'NONE', *, *, #15090, .F. ) ;
#14231=ADVANCED_FACE ( 'NONE', ( #3713 ), #487, .T. ) ;
#14232=VERTEX_POINT ( 'NONE', #19883 ) ;
#14236=CARTESIAN_POINT ( 'NONE',  ( 5.405949406249999534, 9.363379034771803333, -163.0937500020484094 ) ) ;
#14238=CARTESIAN_POINT ( 'NONE',  ( -5.405949406249996869, 9.363379034771805109, -15.84375000204835082 ) ) ;
#14239=DIRECTION ( 'NONE',  ( -0.000000000000000000, -0.000000000000000000, 1.000000000000000000 ) ) ;
#14240=CARTESIAN_POINT ( 'NONE',  ( -10.81189881249999729, -6.242252689847864744, -148.9687500020484094 ) ) ;
#14241=CARTESIAN_POINT ( 'NONE',  ( -2.293366432827344421E-15, -12.48450537969573659, -139.7187500020483810 ) ) ;
#14242=CARTESIAN_POINT ( 'NONE',  ( -2.293366432827344421E-15, -12.48450537969573659, -106.9062500020483952 ) ) ;
#14246=CARTESIAN_POINT ( 'NONE',  ( 5.405949406249999534, 9.363379034771803333, -7.093750002048371250 ) ) ;
#14248=CARTESIAN_POINT ( 'NONE',  ( -10.81189881249999729, 1.324075727343319199E-15, -198.7812500020484094 ) ) ;
#14249=CARTESIAN_POINT ( 'NONE',  ( -2.121150477449813534E-15, -11.54700538379251284, -196.2500000040967905 ) ) ;
#14252=CARTESIAN_POINT ( 'NONE',  ( 10.81189881249999551, -6.242252689847874514, -76.46875000204838102 ) ) ;
#14253=CARTESIAN_POINT ( 'NONE',  ( 5.405949406249992428, -9.363379034771808662, -61.59375000204836681 ) ) ;
#14254=CARTESIAN_POINT ( 'NONE',  ( -9.999999999999998224, 1.224646799147353059E-15, -19.62500000409675494 ) ) ;
#14255=CARTESIAN_POINT ( 'NONE',  ( -5.405949406250003975, -9.363379034771801557, -36.53125000204837391 ) ) ;
#14257=FACE_OUTER_BOUND ( 'NONE', #8491, .T. ) ;
#14259=CARTESIAN_POINT ( 'NONE',  ( 5.000000000000000000, 8.660254037844385522, -120.2500000000000000 ) ) ;
#14260=CARTESIAN_POINT ( 'NONE',  ( -5.405949406249996869, 9.363379034771805109, -131.5312500020484094 ) ) ;
#14263=CARTESIAN_POINT ( 'NONE',  ( 10.81189881249999551, -6.242252689847874514, -15.15625000204837214 ) ) ;
#14264=( BOUNDED_CURVE ( )  B_SPLINE_CURVE ( 2, ( #7732, #17848, #31471, #38148, #37285, #1476, #14611 ),
 .UNSPECIFIED., .F., .F. ) 
 B_SPLINE_CURVE_WITH_KNOTS ( ( 3, 2, 2, 3 ),
 ( 0.2835820895522389029, 0.2848258706467662882, 0.2860696517412936180, 0.2873134328358210032 ),
 .UNSPECIFIED. ) 
 CURVE ( )  GEOMETRIC_REPRESENTATION_ITEM ( )  RATIONAL_B_SPLINE_CURVE ( ( 0.9999999999999880096, 0.8660254037844506980, 1.000000000000000000, 0.8660254037844387076, 1.000000000000000000, 0.8660254037844267172, 1.000000000000011990 ) ) 
 REPRESENTATION_ITEM ( '' )  );
#14265=ORIENTED_EDGE ( 'NONE', *, *, #4286, .F. ) ;
#14268=CARTESIAN_POINT ( 'NONE',  ( -5.000000000000003553, -8.660254037844383745, -56.87500000409676204 ) ) ;
#14269=CARTESIAN_POINT ( 'NONE',  ( -9.999999999999998224, 5.773502691896259087, -34.75000000409674783 ) ) ;
#14270=FACE_OUTER_BOUND ( 'NONE', #26058, .T. ) ;
#14273=CARTESIAN_POINT ( 'NONE',  ( 5.405949406249992428, -9.363379034771808662, -151.7812500020484094 ) ) ;
#14274=CARTESIAN_POINT ( 'NONE',  ( 10.81189881249999729, 0.000000000000000000, -125.8437500020483952 ) ) ;
#14276=ORIENTED_EDGE ( 'NONE', *, *, #9830, .T. ) ;
#14277=CARTESIAN_POINT ( 'NONE',  ( 5.000000000000000000, 8.660254037844385522, -31.74999999999997158 ) ) ;
#14278=EDGE_LOOP ( 'NONE', ( #35544, #34332, #10216, #37555 ) ) ;
#14279=ORIENTED_EDGE ( 'NONE', *, *, #35208, .T. ) ;
#14280=VECTOR ( 'NONE', #36831, 1000.000000000000000 ) ;
#14281=EDGE_CURVE ( 'NONE', #6102, #16786, #11017, .T. ) ;
#14282=CARTESIAN_POINT ( 'NONE',  ( -10.81189881249999729, 1.324075727343319199E-15, -114.5937500020483810 ) ) ;
#14284=AXIS2_PLACEMENT_3D ( 'NONE', #7698, #14136, #15003 ) ;
#14285=EDGE_CURVE ( 'NONE', #18018, #23066, #23566, .T. ) ;
#14286=EDGE_CURVE ( 'NONE', #25687, #14871, #3922, .T. ) ;
#14287=CARTESIAN_POINT ( 'NONE',  ( 5.405949406249999534, 9.363379034771803333, -187.0937500020483810 ) ) ;
#14288=CARTESIAN_POINT ( 'NONE',  ( -2.293366432827344421E-15, -12.48450537969573659, -42.21875000204835970 ) ) ;
#14289=CARTESIAN_POINT ( 'NONE',  ( 4.999999999999992006, -8.660254037844389075, -155.6250000040967905 ) ) ;
#14290=CARTESIAN_POINT ( 'NONE',  ( 4.999999999999992006, -8.660254037844389075, -31.12500000409676559 ) ) ;
#14291=CARTESIAN_POINT ( 'NONE',  ( -5.405949406249996869, 9.363379034771805109, -168.8437500020484094 ) ) ;
#14292=CARTESIAN_POINT ( 'NONE',  ( 10.81189881249999729, 0.000000000000000000, -157.3437500020483810 ) ) ;
#14294=CARTESIAN_POINT ( 'NONE',  ( -5.000000000000003553, -8.660254037844383745, -76.37500000409677625 ) ) ;
#14297=CARTESIAN_POINT ( 'NONE',  ( 9.999999999999998224, 0.000000000000000000, -53.37500000409675494 ) ) ;
#14299=CARTESIAN_POINT ( 'NONE',  ( -2.293366432827344421E-15, -12.48450537969573659, -87.21875000204838102 ) ) ;
#14301=CARTESIAN_POINT ( 'NONE',  ( 10.81189881249999551, -6.242252689847874514, -57.15625000204837391 ) ) ;
#14302=CARTESIAN_POINT ( 'NONE',  ( -8.659811548901195977, -5.000849327365069819, 0.000000000000000000 ) ) ;
#14304=EDGE_CURVE ( 'NONE', #18939, #24456, #15180, .T. ) ;
#14305=CARTESIAN_POINT ( 'NONE',  ( 5.405949406249992428, -9.363379034771808662, -114.2812500020483952 ) ) ;
#14306=CARTESIAN_POINT ( 'NONE',  ( 10.81189881249999551, -6.242252689847874514, -151.6562500020484094 ) ) ;
#14309=CARTESIAN_POINT ( 'NONE',  ( 9.999999999999996447, -5.773502691896262640, -133.0000000040967905 ) ) ;
#14311=ORIENTED_EDGE ( 'NONE', *, *, #31628, .F. ) ;
#14315=EDGE_CURVE ( 'NONE', #31960, #29666, #3075, .T. ) ;
#14316=CARTESIAN_POINT ( 'NONE',  ( -2.293366432827344421E-15, -12.48450537969573659, -187.9062500020484094 ) ) ;
#14317=AXIS2_PLACEMENT_3D ( 'NONE', #23038, #26488, #23681 ) ;
#14318=EDGE_LOOP ( 'NONE', ( #586, #2021, #1592, #2555 ) ) ;
#14319=CARTESIAN_POINT ( 'NONE',  ( -5.000000000000003553, -8.660254037844383745, -45.99999999999998579 ) ) ;
#14321=CARTESIAN_POINT ( 'NONE',  ( -4.999999999999996447, 8.660254037844387298, -61.87500000409676204 ) ) ;
#14323=AXIS2_PLACEMENT_3D ( 'NONE', #32452, #9968, #26176 ) ;
#14324=CARTESIAN_POINT ( 'NONE',  ( 5.000000000000000000, 8.660254037844385522, -21.62500000409675494 ) ) ;
#14325=CARTESIAN_POINT ( 'NONE',  ( 0.000000000000000000, 0.000000000000000000, -200.0000000000000000 ) ) ;
#14327=CARTESIAN_POINT ( 'NONE',  ( -2.293366432827344421E-15, -12.48450537969573659, -54.40625000204838102 ) ) ;
#14330=CARTESIAN_POINT ( 'NONE',  ( 9.999999999999998224, 0.000000000000000000, -200.0000000000000000 ) ) ;
#14331=CARTESIAN_POINT ( 'NONE',  ( -10.81189881249999729, 6.242252689847871849, -173.4062500020483810 ) ) ;
#14334=FACE_OUTER_BOUND ( 'NONE', #28722, .T. ) ;
#14335=ADVANCED_FACE ( 'NONE', ( #39734 ), #6943, .T. ) ;
#14337=CARTESIAN_POINT ( 'NONE',  ( 5.000000000000000000, 8.660254037844385522, -177.2500000000000284 ) ) ;
#14338=CARTESIAN_POINT ( 'NONE',  ( 0.000000000000000000, 0.000000000000000000, -200.0000000000000000 ) ) ;
#14339=CARTESIAN_POINT ( 'NONE',  ( 5.405949406249999534, 9.363379034771803333, -82.28125000204838102 ) ) ;
#14340=ORIENTED_EDGE ( 'NONE', *, *, #27221, .T. ) ;
#14342=CARTESIAN_POINT ( 'NONE',  ( 9.999999999999998224, 0.000000000000000000, -173.3750000040968189 ) ) ;
#14343=VERTEX_POINT ( 'NONE', #23354 ) ;
#14344=VERTEX_POINT ( 'NONE', #13601 ) ;
#14345=CARTESIAN_POINT ( 'NONE',  ( -5.405949406250003975, -9.363379034771801557, -34.84375000204836681 ) ) ;
#14346=CARTESIAN_POINT ( 'NONE',  ( -2.293366432827344421E-15, -12.48450537969573659, -27.21875000204838102 ) ) ;
#14347=CARTESIAN_POINT ( 'NONE',  ( -10.81189881249999729, 6.242252689847871849, -14.40625000204836859 ) ) ;
#14348=CARTESIAN_POINT ( 'NONE',  ( -2.293366432827344421E-15, -12.48450537969573659, -61.71875000204838102 ) ) ;
#14349=CARTESIAN_POINT ( 'NONE',  ( 9.999999999998969713, 5.773502691896851502, -28.87499999999995381 ) ) ;
#14351=VECTOR ( 'NONE', #23846, 1000.000000000000000 ) ;
#14352=CARTESIAN_POINT ( 'NONE',  ( -10.81189881249999729, 6.242252689847871849, -182.2187500020484379 ) ) ;
#14353=( BOUNDED_CURVE ( )  B_SPLINE_CURVE ( 2, ( #28894, #25651, #2141, #21552, #34733, #15054, #35369 ),
 .UNSPECIFIED., .F., .F. ) 
 B_SPLINE_CURVE_WITH_KNOTS ( ( 3, 2, 2, 3 ),
 ( 0.6082089552238807428, 0.6094527363184080171, 0.6106965174129354024, 0.6119402985074627876 ),
 .UNSPECIFIED. ) 
 CURVE ( )  GEOMETRIC_REPRESENTATION_ITEM ( )  RATIONAL_B_SPLINE_CURVE ( ( 0.9999999999999880096, 0.8660254037844506980, 1.000000000000000000, 0.8660254037844387076, 1.000000000000000000, 0.8660254037844267172, 1.000000000000011990 ) ) 
 REPRESENTATION_ITEM ( '' )  );
#14356=CARTESIAN_POINT ( 'NONE',  ( 9.999999999999998224, 0.000000000000000000, -104.3750000040967763 ) ) ;
#14358=CYLINDRICAL_SURFACE ( 'NONE', #1922, 9.999999999999998224 ) ;
#14359=CARTESIAN_POINT ( 'NONE',  ( -5.405949406250003975, -9.363379034771801557, -115.8437500020483810 ) ) ;
#14361=CARTESIAN_POINT ( 'NONE',  ( 7.644554776091147741E-16, 12.48450537969573659, -79.15625000204838102 ) ) ;
#14362=CARTESIAN_POINT ( 'NONE',  ( -2.293366432827344421E-15, -12.48450537969573659, -100.7187500020483952 ) ) ;
#14365=CARTESIAN_POINT ( 'NONE',  ( 7.070501591499377789E-16, 11.54700538379251284, -153.5000000040967905 ) ) ;
#14367=ADVANCED_FACE ( 'NONE', ( #39945 ), #695, .T. ) ;
#14374=CARTESIAN_POINT ( 'NONE',  ( 10.00000000000000000, 5.773502691896255534, -76.87499999999997158 ) ) ;
#14376=CARTESIAN_POINT ( 'NONE',  ( -10.00000000000000000, -5.773502691896251982, -81.00000000409677625 ) ) ;
#14377=DIRECTION ( 'NONE',  ( 1.000000000000000000, 0.000000000000000000, 0.000000000000000000 ) ) ;
#14379=CARTESIAN_POINT ( 'NONE',  ( -5.405949406250003975, -9.363379034771801557, -72.53125000204838102 ) ) ;
#14381=CARTESIAN_POINT ( 'NONE',  ( 9.999999999999998224, 0.000000000000000000, -198.8750000040967905 ) ) ;
#14383=ORIENTED_EDGE ( 'NONE', *, *, #37564, .F. ) ;
#14384=CARTESIAN_POINT ( 'NONE',  ( -5.000000000000003553, -8.660254037844383745, -3.999999999999976019 ) ) ;
#14386=CARTESIAN_POINT ( 'NONE',  ( 7.644554776091147741E-16, 12.48450537969573659, -11.46875000204836859 ) ) ;
#14387=CARTESIAN_POINT ( 'NONE',  ( -9.999999999998969713, -5.773502691896847949, -64.50000000409674783 ) ) ;
#14389=CARTESIAN_POINT ( 'NONE',  ( -10.81189881249999729, 1.324075727343319199E-15, -129.7812500020483810 ) ) ;
#14390=CARTESIAN_POINT ( 'NONE',  ( -5.000000000000003553, -8.660254037844383745, -185.5000000000000000 ) ) ;
#14391=CARTESIAN_POINT ( 'NONE',  ( -9.999999999999868550, 5.773502691896333694, -175.7500000040967905 ) ) ;
#14393=CARTESIAN_POINT ( 'NONE',  ( -2.293366432827344421E-15, -12.48450537969573659, -112.9062500020483952 ) ) ;
#14395=CARTESIAN_POINT ( 'NONE',  ( -9.999999999999998224, 1.224646799147353059E-15, -200.0000000000000000 ) ) ;
#14399=VECTOR ( 'NONE', #9668, 1000.000000000000000 ) ;
#14400=CARTESIAN_POINT ( 'NONE',  ( -2.293366432827344421E-15, -12.48450537969573659, -36.40625000204835970 ) ) ;
#14402=CARTESIAN_POINT ( 'NONE',  ( -5.405949406249996869, 9.363379034771805109, -86.34375000204836681 ) ) ;
#14403=DIRECTION ( 'NONE',  ( -1.000000000000000000, 0.000000000000000000, -0.000000000000000000 ) ) ;
#14404=CARTESIAN_POINT ( 'NONE',  ( 9.999999999999998224, 0.000000000000000000, -174.5000000000000284 ) ) ;
#14405=( BOUNDED_CURVE ( )  B_SPLINE_CURVE ( 2, ( #37357, #34562, #11014, #4554, #41215, #11873, #31329 ),
 .UNSPECIFIED., .F., .F. ) 
 B_SPLINE_CURVE_WITH_KNOTS ( ( 3, 2, 2, 3 ),
 ( 0.08208955223880604057, 0.08333333333333339810, 0.08457711442786078337, 0.08582089552238814090 ),
 .UNSPECIFIED. ) 
 CURVE ( )  GEOMETRIC_REPRESENTATION_ITEM ( )  RATIONAL_B_SPLINE_CURVE ( ( 0.9999999999999924505, 0.8660254037844461461, 1.000000000000000000, 0.8660254037844387076, 1.000000000000000000, 0.8660254037844297148, 1.000000000000008882 ) ) 
 REPRESENTATION_ITEM ( '' )  );
#14406=CARTESIAN_POINT ( 'NONE',  ( 9.999999999999998224, 0.000000000000000000, -200.0000000000000000 ) ) ;
#14408=CARTESIAN_POINT ( 'NONE',  ( -10.00000000000102496, 5.773502691895664007, -58.37499999999997158 ) ) ;
#14409=EDGE_CURVE ( 'NONE', #18779, #17639, #34246, .T. ) ;
#14410=CARTESIAN_POINT ( 'NONE',  ( -2.293366432827344421E-15, -12.48450537969573659, -121.7187500020483952 ) ) ;
#14412=DIRECTION ( 'NONE',  ( -0.000000000000000000, -0.000000000000000000, 1.000000000000000000 ) ) ;
#14415=CARTESIAN_POINT ( 'NONE',  ( 7.070501591499377789E-16, 11.54700538379251284, -182.0000000040968189 ) ) ;
#14417=CARTESIAN_POINT ( 'NONE',  ( 10.81189881249999551, -6.242252689847874514, -175.6562500020484094 ) ) ;
#14418=CARTESIAN_POINT ( 'NONE',  ( -2.121150477449813534E-15, -11.54700538379251284, -107.3749999999999858 ) ) ;
#14419=CARTESIAN_POINT ( 'NONE',  ( 9.999999999999998224, 0.000000000000000000, -164.3750000040967905 ) ) ;
#14421=CARTESIAN_POINT ( 'NONE',  ( 10.81189881249999729, 0.000000000000000000, -53.84375000204835970 ) ) ;
#14422=VECTOR ( 'NONE', #3864, 1000.000000000000000 ) ;
#14424=CARTESIAN_POINT ( 'NONE',  ( 5.405949406249992428, -9.363379034771808662, -12.28125000204835438 ) ) ;
#14426=CARTESIAN_POINT ( 'NONE',  ( 10.00000000000025402, -5.773502691896113426, -158.5000000040968473 ) ) ;
#14428=CARTESIAN_POINT ( 'NONE',  ( 4.999999999999992006, -8.660254037844389075, -95.24999999999998579 ) ) ;
#14430=CARTESIAN_POINT ( 'NONE',  ( -2.121150477449813534E-15, -11.54700538379251284, -103.2500000040967763 ) ) ;
#14434=CARTESIAN_POINT ( 'NONE',  ( -10.81189881249999729, -6.242252689847864744, -111.6562500020483952 ) ) ;
#14436=VERTEX_POINT ( 'NONE', #21380 ) ;
#14437=CARTESIAN_POINT ( 'NONE',  ( 0.000000000000000000, 0.000000000000000000, -200.0000000000000000 ) ) ;
#14439=CARTESIAN_POINT ( 'NONE',  ( 7.070501591499376803E-16, 11.54700538379251284, -91.62500000000000000 ) ) ;
#14440=CARTESIAN_POINT ( 'NONE',  ( -10.81189881249999729, 1.324075727343319199E-15, -164.2812500020484094 ) ) ;
#14442=ORIENTED_EDGE ( 'NONE', *, *, #35792, .F. ) ;
#14443=CARTESIAN_POINT ( 'NONE',  ( 7.070501591499377789E-16, 11.54700538379251284, -27.12499999999998224 ) ) ;
#14444=CARTESIAN_POINT ( 'NONE',  ( 10.81189881249999729, 0.000000000000000000, -36.03125000204837391 ) ) ;
#14445=CARTESIAN_POINT ( 'NONE',  ( 10.00000000000000000, 5.773502691896255534, -163.8750000000000000 ) ) ;
#14446=CARTESIAN_POINT ( 'NONE',  ( 0.000000000000000000, 0.000000000000000000, -200.0000000000000000 ) ) ;
#14449=CARTESIAN_POINT ( 'NONE',  ( -2.293366432827344421E-15, -12.48450537969573659, -130.9062500020483810 ) ) ;
#14450=CARTESIAN_POINT ( 'NONE',  ( -4.999999999999996447, 8.660254037844387298, -110.9999999999999858 ) ) ;
#14451=DIRECTION ( 'NONE',  ( -0.000000000000000000, -0.000000000000000000, 1.000000000000000000 ) ) ;
#14453=VECTOR ( 'NONE', #10901, 1000.000000000000000 ) ;
#14454=ORIENTED_EDGE ( 'NONE', *, *, #22828, .T. ) ;
#14457=CARTESIAN_POINT ( 'NONE',  ( -5.000000000000003553, -8.660254037844383745, -146.8750000040967905 ) ) ;
#14458=CARTESIAN_POINT ( 'NONE',  ( 5.405949406249992428, -9.363379034771808662, -162.0937500020484094 ) ) ;
#14459=ADVANCED_FACE ( 'NONE', ( #17915 ), #37133, .T. ) ;
#14461=CARTESIAN_POINT ( 'NONE',  ( -10.81189881249999729, 6.242252689847871849, -12.71875000204837747 ) ) ;
#14462=DIRECTION ( 'NONE',  ( 1.000000000000000000, 0.000000000000000000, 0.000000000000000000 ) ) ;
#14463=CARTESIAN_POINT ( 'NONE',  ( 10.81189881249999729, 0.000000000000000000, -145.3437500020483810 ) ) ;
#14464=CARTESIAN_POINT ( 'NONE',  ( -10.81189881249999729, 6.242252689847871849, -134.2187500020483810 ) ) ;
#14465=CARTESIAN_POINT ( 'NONE',  ( 7.644554776091147741E-16, 12.48450537969573659, -109.1562500020483810 ) ) ;
#14469=CARTESIAN_POINT ( 'NONE',  ( 7.644554776091147741E-16, 12.48450537969573659, 0.5312499979516547288 ) ) ;
#14474=CARTESIAN_POINT ( 'NONE',  ( -5.405949406250003975, -9.363379034771801557, -78.34375000204838102 ) ) ;
#14475=CARTESIAN_POINT ( 'NONE',  ( -2.293366432827344421E-15, -12.48450537969573659, -67.71875000204838102 ) ) ;
#14477=CARTESIAN_POINT ( 'NONE',  ( 5.405949406249999534, 9.363379034771803333, -31.28125000204837036 ) ) ;
#14479=CARTESIAN_POINT ( 'NONE',  ( -9.999999999999998224, 1.224646799147353059E-15, -114.1250000040967763 ) ) ;
#14481=CARTESIAN_POINT ( 'NONE',  ( 10.00000000000000000, 5.773502691896255534, -118.8749999999999858 ) ) ;
#14482=CARTESIAN_POINT ( 'NONE',  ( -10.81189881249999729, 6.242252689847871849, -129.9062500020483810 ) ) ;
#14485=CARTESIAN_POINT ( 'NONE',  ( -2.293366432827344421E-15, -12.48450537969573659, -21.40625000204837036 ) ) ;
#14486=EDGE_LOOP ( 'NONE', ( #13845, #38765, #18452, #33651 ) ) ;
#14490=AXIS2_PLACEMENT_3D ( 'NONE', #8797, #9428, #25420 ) ;
#14491=CARTESIAN_POINT ( 'NONE',  ( -4.999999999999996447, 8.660254037844387298, -34.87500000409676915 ) ) ;
#14492=EDGE_CURVE ( 'NONE', #36795, #32436, #41653, .T. ) ;
#14493=CARTESIAN_POINT ( 'NONE',  ( 9.999999999998969713, 5.773502691896851502, -61.87499999999997158 ) ) ;
#14495=CARTESIAN_POINT ( 'NONE',  ( -2.121150477449813534E-15, -11.54700538379251284, -40.25000000409676204 ) ) ;
#14496=CARTESIAN_POINT ( 'NONE',  ( 10.81189881249999551, -6.242252689847874514, -156.1562500020484094 ) ) ;
#14497=CARTESIAN_POINT ( 'NONE',  ( 10.81189881249999729, 0.000000000000000000, -128.8437500020484094 ) ) ;
#14498=CARTESIAN_POINT ( 'NONE',  ( -9.999999999999998224, 1.224646799147353059E-15, -181.6250000040967905 ) ) ;
#14499=VERTEX_POINT ( 'NONE', #20734 ) ;
#14500=LINE ( 'NONE', #8275, #19694 ) ;
#14503=CARTESIAN_POINT ( 'NONE',  ( -10.81189881249999729, 1.324075727343319199E-15, -108.5937500020483810 ) ) ;
#14504=ORIENTED_EDGE ( 'NONE', *, *, #37512, .T. ) ;
#14506=CARTESIAN_POINT ( 'NONE',  ( -2.293366432827344421E-15, -12.48450537969573659, -187.7187500020484094 ) ) ;
#14508=CARTESIAN_POINT ( 'NONE',  ( 7.644554776091147741E-16, 12.48450537969573659, -42.96875000204835970 ) ) ;
#14509=CARTESIAN_POINT ( 'NONE',  ( -7.481659653677922073, -6.786049171891036735, 9.002545116942492289E-15 ) ) ;
#14510=CARTESIAN_POINT ( 'NONE',  ( -2.121150477449813534E-15, -11.54700538379251284, -74.37499999999997158 ) ) ;
#14511=CARTESIAN_POINT ( 'NONE',  ( -5.405949406250003975, -9.363379034771801557, -168.3437500020484094 ) ) ;
#14512=CARTESIAN_POINT ( 'NONE',  ( -2.293366432827344421E-15, -12.48450537969573659, -163.7187500020483810 ) ) ;
#14513=CARTESIAN_POINT ( 'NONE',  ( 7.070501591499376803E-16, 11.54700538379251284, -178.6250000000000000 ) ) ;
#14516=( BOUNDED_CURVE ( )  B_SPLINE_CURVE ( 2, ( #3656, #26731, #27158, #425, #20033, #13751, #39885 ),
 .UNSPECIFIED., .F., .F. ) 
 B_SPLINE_CURVE_WITH_KNOTS ( ( 3, 2, 2, 3 ),
 ( 0.5149253731343285123, 0.5161691542288557866, 0.5174129353233831718, 0.5186567164179105571 ),
 .UNSPECIFIED. ) 
 CURVE ( )  GEOMETRIC_REPRESENTATION_ITEM ( )  RATIONAL_B_SPLINE_CURVE ( ( 0.9999999999999880096, 0.8660254037844506980, 1.000000000000000000, 0.8660254037844387076, 1.000000000000000000, 0.8660254037844267172, 1.000000000000011990 ) ) 
 REPRESENTATION_ITEM ( '' )  );
#14518=CARTESIAN_POINT ( 'NONE',  ( 4.999999999999992006, -8.660254037844389075, -93.74999999999998579 ) ) ;
#14519=CARTESIAN_POINT ( 'NONE',  ( 9.999999999999998224, 0.000000000000000000, -200.0000000000000000 ) ) ;
#14521=CARTESIAN_POINT ( 'NONE',  ( -10.81189881249999729, 6.242252689847871849, -92.21875000204838102 ) ) ;
#14523=CARTESIAN_POINT ( 'NONE',  ( -2.293366432827344421E-15, -12.48450537969573659, -57.40625000204838102 ) ) ;
#14524=CARTESIAN_POINT ( 'NONE',  ( -9.999999999999998224, 1.224646799147353059E-15, -145.6250000040967905 ) ) ;
#14526=CARTESIAN_POINT ( 'NONE',  ( -10.81189881249999729, 6.242252689847871849, -114.9062500020483952 ) ) ;
#14527=CARTESIAN_POINT ( 'NONE',  ( -10.81189881249999729, -6.242252689847864744, -153.6562500020484094 ) ) ;
#14530=CARTESIAN_POINT ( 'NONE',  ( 4.999999999999992006, -8.660254037844389075, -131.6250000040967620 ) ) ;
#14536=CARTESIAN_POINT ( 'NONE',  ( -10.81189881249999907, -6.242252689847864744, -182.1562500020483810 ) ) ;
#14538=CARTESIAN_POINT ( 'NONE',  ( 4.999999999999992006, -8.660254037844389075, -50.24999999999998579 ) ) ;
#14540=CARTESIAN_POINT ( 'NONE',  ( 9.999999999999998224, 0.000000000000000000, -60.87500000409676204 ) ) ;
#14543=FACE_OUTER_BOUND ( 'NONE', #17105, .T. ) ;
#14544=ADVANCED_FACE ( 'NONE', ( #21161 ), #34347, .T. ) ;
#14546=CARTESIAN_POINT ( 'NONE',  ( -10.81189881249999729, 1.324075727343319199E-15, -51.78125000204835970 ) ) ;
#14547=AXIS2_PLACEMENT_3D ( 'NONE', #29437, #35500, #29224 ) ;
#14551=CARTESIAN_POINT ( 'NONE',  ( -10.81189881249999729, 6.242252689847871849, -179.4062500020484094 ) ) ;
#14553=CARTESIAN_POINT ( 'NONE',  ( -2.121150477449813534E-15, -11.54700538379251284, -73.25000000409676204 ) ) ;
#14557=FACE_OUTER_BOUND ( 'NONE', #9436, .T. ) ;
#14558=VECTOR ( 'NONE', #18836, 1000.000000000000000 ) ;
#14559=CARTESIAN_POINT ( 'NONE',  ( -5.405949406249996869, 9.363379034771805109, -86.53125000204838102 ) ) ;
#14561=CARTESIAN_POINT ( 'NONE',  ( 9.999999999999998224, 0.000000000000000000, -200.0000000000000000 ) ) ;
#14562=VERTEX_POINT ( 'NONE', #8230 ) ;
#14564=VERTEX_POINT ( 'NONE', #20516 ) ;
#14565=CARTESIAN_POINT ( 'NONE',  ( 7.644554776091147741E-16, 12.48450537969573659, -33.96875000204834549 ) ) ;
#14566=CARTESIAN_POINT ( 'NONE',  ( 5.405949406249992428, -9.363379034771808662, -28.59375000204836326 ) ) ;
#14567=CARTESIAN_POINT ( 'NONE',  ( -5.405949406250003975, -9.363379034771801557, -17.03125000204835970 ) ) ;
#14568=CARTESIAN_POINT ( 'NONE',  ( -10.81189881249999729, 6.242252689847871849, -63.71875000204838102 ) ) ;
#14569=CARTESIAN_POINT ( 'NONE',  ( -2.121150477449813534E-15, -11.54700538379251284, -17.75000000409676204 ) ) ;
#14571=ADVANCED_FACE ( 'NONE', ( #4129 ), #27865, .T. ) ;
#14572=CARTESIAN_POINT ( 'NONE',  ( 5.405949406249992428, -9.363379034771808662, -186.0937500020483810 ) ) ;
#14574=VECTOR ( 'NONE', #6481, 1000.000000000000000 ) ;
#14576=CARTESIAN_POINT ( 'NONE',  ( 7.070501591499376803E-16, 11.54700538379251284, -132.1250000000000000 ) ) ;
#14577=CARTESIAN_POINT ( 'NONE',  ( -9.999999999999998224, 1.224646799147353059E-15, -140.7500000000000000 ) ) ;
#14579=CARTESIAN_POINT ( 'NONE',  ( 9.999999999999998224, 0.000000000000000000, -186.5000000000000000 ) ) ;
#14581=CARTESIAN_POINT ( 'NONE',  ( -10.81189881249999729, 1.324075727343319199E-15, -110.0937500020483810 ) ) ;
#14582=DIRECTION ( 'NONE',  ( -0.000000000000000000, -0.000000000000000000, 1.000000000000000000 ) ) ;
#14583=CARTESIAN_POINT ( 'NONE',  ( -5.405949406250003975, -9.363379034771801557, -86.03125000204838102 ) ) ;
#14584=CARTESIAN_POINT ( 'NONE',  ( -2.293366432827344421E-15, -12.48450537969573659, -102.2187500020483668 ) ) ;
#14587=CARTESIAN_POINT ( 'NONE',  ( 9.999999999999996447, -5.773502691896262640, -155.5000000040968189 ) ) ;
#14594=CARTESIAN_POINT ( 'NONE',  ( 9.999999999999742428, 5.773502691896404748, -120.7500000040967905 ) ) ;
#14595=CARTESIAN_POINT ( 'NONE',  ( -10.00000000000000000, -5.773502691896251982, -73.12499999999995737 ) ) ;
#14597=CARTESIAN_POINT ( 'NONE',  ( 4.999999999999992006, -8.660254037844389075, -82.12500000409676204 ) ) ;
#14598=EDGE_CURVE ( 'NONE', #28673, #22153, #20988, .T. ) ;
#14599=CARTESIAN_POINT ( 'NONE',  ( -4.999999999999996447, 8.660254037844387298, -25.87500000409675849 ) ) ;
#14601=CARTESIAN_POINT ( 'NONE',  ( -10.81189881249999729, -6.242252689847864744, -77.15625000204836681 ) ) ;
#14602=ADVANCED_FACE ( 'NONE', ( #23772 ), #18135, .T. ) ;
#14604=CARTESIAN_POINT ( 'NONE',  ( -4.999999999999996447, 8.660254037844387298, -112.8750000040967763 ) ) ;
#14606=ORIENTED_EDGE ( 'NONE', *, *, #9588, .T. ) ;
#14607=CARTESIAN_POINT ( 'NONE',  ( 10.81189881249999729, 0.000000000000000000, -198.0312500020484094 ) ) ;
#14608=EDGE_CURVE ( 'NONE', #4966, #12865, #10584, .T. ) ;
#14610=CARTESIAN_POINT ( 'NONE',  ( 7.644554776091147741E-16, 12.48450537969573659, -9.968750002048363257 ) ) ;
#14611=CARTESIAN_POINT ( 'NONE',  ( -9.999999999999998224, 1.224646799147353059E-15, -142.2500000000000000 ) ) ;
#14613=CARTESIAN_POINT ( 'NONE',  ( -10.81189881249999729, 6.242252689847871849, -131.4062500020484094 ) ) ;
#14615=CARTESIAN_POINT ( 'NONE',  ( 4.999999999999992006, -8.660254037844389075, -183.7500000000000000 ) ) ;
#14616=FACE_OUTER_BOUND ( 'NONE', #26190, .T. ) ;
#14617=CARTESIAN_POINT ( 'NONE',  ( -10.81189881249999729, 6.242252689847871849, -107.4062500020483810 ) ) ;
#14618=ORIENTED_EDGE ( 'NONE', *, *, #15617, .T. ) ;
#14619=CARTESIAN_POINT ( 'NONE',  ( 9.999999999999998224, 0.000000000000000000, -40.99999999999997868 ) ) ;
#14621=( BOUNDED_CURVE ( )  B_SPLINE_CURVE ( 2, ( #36984, #11066, #23625, #30314, #26639, #13657, #20359 ),
 .UNSPECIFIED., .F., .F. ) 
 B_SPLINE_CURVE_WITH_KNOTS ( ( 3, 2, 2, 3 ),
 ( 0.2313432835820896372, 0.2325870646766169947, 0.2338308457711443245, 0.2350746268656717097 ),
 .UNSPECIFIED. ) 
 CURVE ( )  GEOMETRIC_REPRESENTATION_ITEM ( )  RATIONAL_B_SPLINE_CURVE ( ( 0.9999999999999910072, 0.8660254037844477004, 1.000000000000000000, 0.8660254037844387076, 1.000000000000000000, 0.8660254037844327124, 1.000000000000005995 ) ) 
 REPRESENTATION_ITEM ( '' )  );
#14622=EDGE_LOOP ( 'NONE', ( #29136, #22710, #40357, #4111 ) ) ;
#14624=CARTESIAN_POINT ( 'NONE',  ( -5.405949406249996869, 9.363379034771805109, -35.53125000204837391 ) ) ;
#14626=VECTOR ( 'NONE', #10199, 1000.000000000000000 ) ;
#14627=CARTESIAN_POINT ( 'NONE',  ( 10.81189881249999907, 6.242252689847868297, -91.21875000204838102 ) ) ;
#14629=CARTESIAN_POINT ( 'NONE',  ( 5.000000000000000000, 8.660254037844385522, -170.1250000040968189 ) ) ;
#14631=CARTESIAN_POINT ( 'NONE',  ( -9.999999999999998224, 1.224646799147353059E-15, -173.7500000000000284 ) ) ;
#14632=CARTESIAN_POINT ( 'NONE',  ( -10.81189881249999729, 1.324075727343319199E-15, -123.5937500020483952 ) ) ;
#14634=CARTESIAN_POINT ( 'NONE',  ( -10.81189881249999729, 6.242252689847871849, -2.406250002048375247 ) ) ;
#14637=CARTESIAN_POINT ( 'NONE',  ( -9.999999999999998224, 1.224646799147353059E-15, -177.1250000040968189 ) ) ;
#14639=CARTESIAN_POINT ( 'NONE',  ( -5.405949406250003975, -9.363379034771801557, -167.0312500020484094 ) ) ;
#14640=CARTESIAN_POINT ( 'NONE',  ( -9.999999999999998224, 1.224646799147353059E-15, -28.62500000409676204 ) ) ;
#14643=CARTESIAN_POINT ( 'NONE',  ( 7.644554776091147741E-16, 12.48450537969573659, -51.96875000204836681 ) ) ;
#14645=CARTESIAN_POINT ( 'NONE',  ( 10.81189881249999551, -6.242252689847874514, -12.15625000204835793 ) ) ;
#14647=CARTESIAN_POINT ( 'NONE',  ( -9.999999999999998224, 1.224646799147353059E-15, -153.1250000040967905 ) ) ;
#14649=CARTESIAN_POINT ( 'NONE',  ( 9.999999999999996447, -5.773502691896262640, -96.62500000000000000 ) ) ;
#14651=CARTESIAN_POINT ( 'NONE',  ( 5.000000000000000000, 8.660254037844385522, -108.6250000040967763 ) ) ;
#14652=CARTESIAN_POINT ( 'NONE',  ( -5.000000000000003553, -8.660254037844383745, -190.3750000040967905 ) ) ;
#14655=CARTESIAN_POINT ( 'NONE',  ( -10.81189881249999729, 1.324075727343319199E-15, -99.78125000204839523 ) ) ;
#14658=CARTESIAN_POINT ( 'NONE',  ( -5.000000000000003553, -8.660254037844383745, -166.3750000040967905 ) ) ;
#14659=CARTESIAN_POINT ( 'NONE',  ( 10.81189881249999907, 6.242252689847868297, -166.4062500020483810 ) ) ;
#14662=CARTESIAN_POINT ( 'NONE',  ( -10.00000000000000000, -5.773502691896251982, -28.12499999999998934 ) ) ;
#14663=CARTESIAN_POINT ( 'NONE',  ( 10.81189881249999729, 0.000000000000000000, -24.03125000204836681 ) ) ;
#14664=CARTESIAN_POINT ( 'NONE',  ( 9.999999999999998224, 0.000000000000000000, -159.5000000000000000 ) ) ;
#14665=DIRECTION ( 'NONE',  ( 1.000000000000000000, 0.000000000000000000, 0.000000000000000000 ) ) ;
#14668=CARTESIAN_POINT ( 'NONE',  ( 9.999999999999998224, 0.000000000000000000, -22.99999999999996447 ) ) ;
#14669=EDGE_CURVE ( 'NONE', #11871, #18780, #35627, .T. ) ;
#14670=CARTESIAN_POINT ( 'NONE',  ( 10.81189881249999551, -6.242252689847874514, -130.6562500020484094 ) ) ;
#14671=CARTESIAN_POINT ( 'NONE',  ( 1.490774595143464776, 10.17940913545393578, 1.249419088690773332E-14 ) ) ;
#14672=CARTESIAN_POINT ( 'NONE',  ( 9.999999999999998224, 0.000000000000000000, -200.0000000000000000 ) ) ;
#14673=VERTEX_POINT ( 'NONE', #8869 ) ;
#14674=( BOUNDED_CURVE ( )  B_SPLINE_CURVE ( 2, ( #26953, #39898, #3878, #4083, #12916, #439, #23086 ),
 .UNSPECIFIED., .F., .F. ) 
 B_SPLINE_CURVE_WITH_KNOTS ( ( 3, 2, 2, 3 ),
 ( 0.7313432835820897759, 0.7325870646766171612, 0.7338308457711446575, 0.7350746268656719318 ),
 .UNSPECIFIED. ) 
 CURVE ( )  GEOMETRIC_REPRESENTATION_ITEM ( )  RATIONAL_B_SPLINE_CURVE ( ( 0.9999999999999761302, 0.8660254037844625774, 1.000000000000000000, 0.8660254037844387076, 1.000000000000000000, 0.8660254037844028474, 1.000000000000035971 ) ) 
 REPRESENTATION_ITEM ( '' )  );
#14675=CARTESIAN_POINT ( 'NONE',  ( 10.81189881249999729, 0.000000000000000000, -60.03125000204836681 ) ) ;
#14676=VERTEX_POINT ( 'NONE', #22031 ) ;
#14677=VERTEX_POINT ( 'NONE', #25700 ) ;
#14679=CARTESIAN_POINT ( 'NONE',  ( 10.81189881249999729, 0.000000000000000000, -157.3437500020483810 ) ) ;
#14681=CARTESIAN_POINT ( 'NONE',  ( -10.81189881249999907, -6.242252689847864744, -12.46875000204837391 ) ) ;
#14682=DIRECTION ( 'NONE',  ( -0.000000000000000000, -0.000000000000000000, 1.000000000000000000 ) ) ;
#14683=CARTESIAN_POINT ( 'NONE',  ( 10.81189881249999551, -6.242252689847874514, -151.4687500020484094 ) ) ;
#14684=CARTESIAN_POINT ( 'NONE',  ( 10.81189881249999551, -6.242252689847874514, -131.9687500020483810 ) ) ;
#14685=CARTESIAN_POINT ( 'NONE',  ( -10.81189881249999729, 6.242252689847871849, -110.4062500020483810 ) ) ;
#14688=CARTESIAN_POINT ( 'NONE',  ( 7.644554776091147741E-16, 12.48450537969573659, -3.968750002048366810 ) ) ;
#14690=CARTESIAN_POINT ( 'NONE',  ( 4.999999999999992006, -8.660254037844389075, -54.74999999999996447 ) ) ;
#14694=CARTESIAN_POINT ( 'NONE',  ( -10.81189881249999729, 6.242252689847871849, -72.71875000204836681 ) ) ;
#14695=CARTESIAN_POINT ( 'NONE',  ( -5.405949406250003975, -9.363379034771801557, -66.34375000204836681 ) ) ;
#14696=CARTESIAN_POINT ( 'NONE',  ( -9.999999999999998224, 1.224646799147353059E-15, -136.2499999999999716 ) ) ;
#14697=CARTESIAN_POINT ( 'NONE',  ( 10.81189881249999551, -6.242252689847874514, -31.65625000204834905 ) ) ;
#14701=CARTESIAN_POINT ( 'NONE',  ( 5.000000000000000000, 8.660254037844385522, -123.2500000000000000 ) ) ;
#14702=CARTESIAN_POINT ( 'NONE',  ( -10.81189881249999729, 1.324075727343319199E-15, -129.7812500020483810 ) ) ;
#14704=CARTESIAN_POINT ( 'NONE',  ( 5.405949406249999534, 9.363379034771803333, -10.28125000204835260 ) ) ;
#14705=ORIENTED_EDGE ( 'NONE', *, *, #20946, .F. ) ;
#14708=DIRECTION ( 'NONE',  ( -0.000000000000000000, -0.000000000000000000, 1.000000000000000000 ) ) ;
#14710=CARTESIAN_POINT ( 'NONE',  ( 9.999999999999998224, 0.000000000000000000, -36.87500000409676915 ) ) ;
#14711=CARTESIAN_POINT ( 'NONE',  ( 9.999999999999479527, 5.773502691896553074, -75.37499999999998579 ) ) ;
#14713=DIRECTION ( 'NONE',  ( 1.000000000000000000, 0.000000000000000000, 0.000000000000000000 ) ) ;
#14714=CARTESIAN_POINT ( 'NONE',  ( 5.405949406249999534, 9.363379034771803333, -155.7812500020484094 ) ) ;
#14715=CARTESIAN_POINT ( 'NONE',  ( -2.293366432827344421E-15, -12.48450537969573659, -130.7187500020483810 ) ) ;
#14716=CARTESIAN_POINT ( 'NONE',  ( 9.999999999999998224, 0.000000000000000000, -95.37500000409677625 ) ) ;
#14717=EDGE_LOOP ( 'NONE', ( #26203, #12443, #20383, #7049 ) ) ;
#14720=ORIENTED_EDGE ( 'NONE', *, *, #38855, .F. ) ;
#14721=EDGE_LOOP ( 'NONE', ( #40551, #10567, #18398, #25327 ) ) ;
#14722=CARTESIAN_POINT ( 'NONE',  ( -9.999999999999998224, 1.224646799147353059E-15, -200.0000000000000000 ) ) ;
#14723=CARTESIAN_POINT ( 'NONE',  ( -10.81189881249999729, 6.242252689847871849, -189.7187500020484379 ) ) ;
#14724=CARTESIAN_POINT ( 'NONE',  ( -10.81189881249999729, 1.324075727343319199E-15, -36.59375000204836681 ) ) ;
#14725=CARTESIAN_POINT ( 'NONE',  ( -5.599846275199223733, -8.529742854289207088, 2.111525036386693496E-16 ) ) ;
#14726=DIRECTION ( 'NONE',  ( -0.000000000000000000, -0.000000000000000000, 1.000000000000000000 ) ) ;
#14727=CARTESIAN_POINT ( 'NONE',  ( 5.405949406249999534, 9.363379034771803333, -175.0937500020484094 ) ) ;
#14728=CARTESIAN_POINT ( 'NONE',  ( 7.644554776091147741E-16, 12.48450537969573659, -156.9687500020484094 ) ) ;
#14729=( BOUNDED_CURVE ( )  B_SPLINE_CURVE ( 2, ( #38136, #31460, #25205, #17838, #8152, #34703, #38346 ),
 .UNSPECIFIED., .F., .F. ) 
 B_SPLINE_CURVE_WITH_KNOTS ( ( 3, 2, 2, 3 ),
 ( 0.2798507462686568026, 0.2810945273631841879, 0.2823383084577115731, 0.2835820895522389029 ),
 .UNSPECIFIED. ) 
 CURVE ( )  GEOMETRIC_REPRESENTATION_ITEM ( )  RATIONAL_B_SPLINE_CURVE ( ( 0.9999999999999880096, 0.8660254037844506980, 1.000000000000000000, 0.8660254037844387076, 1.000000000000000000, 0.8660254037844267172, 1.000000000000011990 ) ) 
 REPRESENTATION_ITEM ( '' )  );
#14730=CARTESIAN_POINT ( 'NONE',  ( -9.999999999999998224, 1.224646799147353059E-15, -33.12500000409676915 ) ) ;
#14734=CARTESIAN_POINT ( 'NONE',  ( 5.000000000000000000, 8.660254037844385522, -126.6250000040967620 ) ) ;
#14735=CYLINDRICAL_SURFACE ( 'NONE', #27525, 9.999999999999998224 ) ;
#14737=CARTESIAN_POINT ( 'NONE',  ( 5.405949406249999534, 9.363379034771803333, -92.59375000204838102 ) ) ;
#14738=CARTESIAN_POINT ( 'NONE',  ( 9.999999999999548805, 5.773502691896515771, -180.7500000040967905 ) ) ;
#14739=CARTESIAN_POINT ( 'NONE',  ( -5.405949406249996869, 9.363379034771805109, -58.03125000204836681 ) ) ;
#14740=DIRECTION ( 'NONE',  ( 1.000000000000000000, 0.000000000000000000, 0.000000000000000000 ) ) ;
#14742=CARTESIAN_POINT ( 'NONE',  ( -2.293366432827344421E-15, -12.48450537969573659, -111.4062500020483952 ) ) ;
#14743=CARTESIAN_POINT ( 'NONE',  ( -5.405949406249996869, 9.363379034771805109, -152.5312500020484094 ) ) ;
#14746=CARTESIAN_POINT ( 'NONE',  ( -9.999999999999998224, 1.224646799147353059E-15, -132.1250000040967620 ) ) ;
#14752=CARTESIAN_POINT ( 'NONE',  ( 10.81189881249999551, -6.242252689847874514, -181.6562500020484379 ) ) ;
#14753=EDGE_LOOP ( 'NONE', ( #18977, #16892, #103, #21378 ) ) ;
#14755=CARTESIAN_POINT ( 'NONE',  ( -9.999999999999998224, 5.773502691896259087, -54.25000000409677625 ) ) ;
#14756=DIRECTION ( 'NONE',  ( -0.000000000000000000, -0.000000000000000000, 1.000000000000000000 ) ) ;
#14757=CARTESIAN_POINT ( 'NONE',  ( -10.00000000000076916, 5.773502691895813221, -135.2500000040967905 ) ) ;
#14759=CARTESIAN_POINT ( 'NONE',  ( -5.405949406249996869, 9.363379034771805109, -50.53125000204835970 ) ) ;
#14762=CARTESIAN_POINT ( 'NONE',  ( 5.405949406249999534, 9.363379034771803333, -175.2812500020484094 ) ) ;
#14763=CARTESIAN_POINT ( 'NONE',  ( -9.999999999999998224, 1.224646799147353059E-15, -200.0000000000000000 ) ) ;
#14766=CARTESIAN_POINT ( 'NONE',  ( -10.00000000000154188, 5.773502691895366468, -16.75000000409671586 ) ) ;
#14768=CARTESIAN_POINT ( 'NONE',  ( 0.000000000000000000, 0.000000000000000000, -200.0000000000000000 ) ) ;
#14769=CARTESIAN_POINT ( 'NONE',  ( -10.81189881249999729, 1.324075727343319199E-15, -83.28125000204838102 ) ) ;
#14770=ORIENTED_EDGE ( 'NONE', *, *, #8798, .F. ) ;
#14771=LINE ( 'NONE', #31424, #31062 ) ;
#14772=LINE ( 'NONE', #34240, #29609 ) ;
#14773=ORIENTED_EDGE ( 'NONE', *, *, #10123, .F. ) ;
#14774=ORIENTED_EDGE ( 'NONE', *, *, #32403, .T. ) ;
#14775=( BOUNDED_CURVE ( )  B_SPLINE_CURVE ( 2, ( #2486, #41949, #5291, #18444, #15614, #12381, #12802 ),
 .UNSPECIFIED., .F., .F. ) 
 B_SPLINE_CURVE_WITH_KNOTS ( ( 3, 2, 2, 3 ),
 ( 0.1082089552238805485, 0.1094527363184079616, 0.1106965174129353746, 0.1119402985074627876 ),
 .UNSPECIFIED. ) 
 CURVE ( )  GEOMETRIC_REPRESENTATION_ITEM ( )  RATIONAL_B_SPLINE_CURVE ( ( 1.000000000000004441, 0.8660254037844343777, 1.000000000000000000, 0.8660254037844387076, 1.000000000000000000, 0.8660254037844282715, 1.000000000000010436 ) ) 
 REPRESENTATION_ITEM ( '' )  );
#14776=CARTESIAN_POINT ( 'NONE',  ( 5.405949406249999534, 9.363379034771803333, -40.09375000204837391 ) ) ;
#14778=CARTESIAN_POINT ( 'NONE',  ( 5.405949406249999534, 9.363379034771803333, -13.28125000204835615 ) ) ;
#14779=CARTESIAN_POINT ( 'NONE',  ( -10.81189881249999907, -6.242252689847864744, -66.46875000204838102 ) ) ;
#14783=CARTESIAN_POINT ( 'NONE',  ( 10.81189881249999907, 6.242252689847868297, -187.2187500020484094 ) ) ;
#14786=CARTESIAN_POINT ( 'NONE',  ( -9.999999999999998224, 1.224646799147353059E-15, -131.7499999999999716 ) ) ;
#14787=VECTOR ( 'NONE', #38554, 1000.000000000000000 ) ;
#14788=DIRECTION ( 'NONE',  ( -0.000000000000000000, -0.000000000000000000, 1.000000000000000000 ) ) ;
#14789=DIRECTION ( 'NONE',  ( 1.000000000000000000, 0.000000000000000000, 0.000000000000000000 ) ) ;
#14791=CARTESIAN_POINT ( 'NONE',  ( 10.81189881249999907, 6.242252689847868297, -112.2187500020483810 ) ) ;
#14793=CARTESIAN_POINT ( 'NONE',  ( -2.293366432827344421E-15, -12.48450537969573659, -79.90625000204839523 ) ) ;
#14794=CARTESIAN_POINT ( 'NONE',  ( 10.81189881249999729, 6.242252689847867408, -88.21875000204838102 ) ) ;
#14797=CARTESIAN_POINT ( 'NONE',  ( 7.070501591499377789E-16, 11.54700538379251284, -150.5000000040968189 ) ) ;
#14801=CARTESIAN_POINT ( 'NONE',  ( -10.00000000000051337, 5.773502691895962435, -97.75000000409676204 ) ) ;
#14802=CYLINDRICAL_SURFACE ( 'NONE', #10275, 9.999999999999998224 ) ;
#14804=CARTESIAN_POINT ( 'NONE',  ( 9.999999999999998224, 0.000000000000000000, -10.99999999999995381 ) ) ;
#14805=CARTESIAN_POINT ( 'NONE',  ( 9.999999999999998224, 0.000000000000000000, -72.49999999999998579 ) ) ;
#14807=CARTESIAN_POINT ( 'NONE',  ( 7.070501591499377789E-16, 11.54700538379251284, -78.50000000409677625 ) ) ;
#14811=CARTESIAN_POINT ( 'NONE',  ( 5.405949406249992428, -9.363379034771808662, -75.28125000204838102 ) ) ;
#14815=ORIENTED_EDGE ( 'NONE', *, *, #36380, .F. ) ;
#14816=CARTESIAN_POINT ( 'NONE',  ( -9.999999999999998224, 5.773502691896259087, -1.374999999999974465 ) ) ;
#14818=CARTESIAN_POINT ( 'NONE',  ( -5.405949406249996869, 9.363379034771805109, -12.84375000204834905 ) ) ;
#14821=CARTESIAN_POINT ( 'NONE',  ( 5.405949406249992428, -9.363379034771808662, -129.2812500020483810 ) ) ;
#14822=CARTESIAN_POINT ( 'NONE',  ( -9.999999999999998224, 1.224646799147353059E-15, -184.2500000000000000 ) ) ;
#14823=DIRECTION ( 'NONE',  ( 1.000000000000000000, 0.000000000000000000, 0.000000000000000000 ) ) ;
#14824=CARTESIAN_POINT ( 'NONE',  ( 5.405949406249999534, 9.363379034771803333, -112.2812500020483952 ) ) ;
#14825=ORIENTED_EDGE ( 'NONE', *, *, #12742, .F. ) ;
#14828=ORIENTED_EDGE ( 'NONE', *, *, #5361, .T. ) ;
#14829=CARTESIAN_POINT ( 'NONE',  ( 10.81189881249999729, 0.000000000000000000, -34.53125000204837391 ) ) ;
#14831=CARTESIAN_POINT ( 'NONE',  ( -2.293366432827344421E-15, -12.48450537969573659, -87.21875000204838102 ) ) ;
#14832=CARTESIAN_POINT ( 'NONE',  ( 9.999999999999998224, 0.000000000000000000, -90.87500000409677625 ) ) ;
#14835=EDGE_CURVE ( 'NONE', #38736, #13374, #35414, .T. ) ;
#14837=ADVANCED_FACE ( 'NONE', ( #2190 ), #38850, .T. ) ;
#14840=CARTESIAN_POINT ( 'NONE',  ( 4.999999999999992006, -8.660254037844389075, -68.24999999999997158 ) ) ;
#14841=CARTESIAN_POINT ( 'NONE',  ( -10.81189881249999729, 1.324075727343319199E-15, -126.5937500020483668 ) ) ;
#14842=AXIS2_PLACEMENT_3D ( 'NONE', #8748, #41314, #38095 ) ;
#14845=CARTESIAN_POINT ( 'NONE',  ( 10.81189881249999729, 6.242252689847867408, -4.406250002048352599 ) ) ;
#14848=CARTESIAN_POINT ( 'NONE',  ( 9.999999999999998224, 0.000000000000000000, -180.8750000040967905 ) ) ;
#14849=CARTESIAN_POINT ( 'NONE',  ( 10.81189881249999551, -6.242252689847874514, -166.6562500020484094 ) ) ;
#14850=CARTESIAN_POINT ( 'NONE',  ( 5.000000000000000000, 8.660254037844385522, -103.7500000000000000 ) ) ;
#14853=CARTESIAN_POINT ( 'NONE',  ( -5.405949406249996869, 9.363379034771805109, -51.84375000204835260 ) ) ;
#14855=CARTESIAN_POINT ( 'NONE',  ( 7.644554776091147741E-16, 12.48450537969573659, -8.656250002048372139 ) ) ;
#14857=CARTESIAN_POINT ( 'NONE',  ( -5.000000000000003553, -8.660254037844383745, -152.8750000040967905 ) ) ;
#14859=CARTESIAN_POINT ( 'NONE',  ( -10.00000000000000000, -5.773502691896251982, -98.62499999999998579 ) ) ;
#14861=CARTESIAN_POINT ( 'NONE',  ( -4.999999999999996447, 8.660254037844387298, -103.8750000040967763 ) ) ;
#14865=CARTESIAN_POINT ( 'NONE',  ( 10.81189881249999729, 0.000000000000000000, -96.03125000204838102 ) ) ;
#14866=EDGE_LOOP ( 'NONE', ( #1912, #18831 ) ) ;
#14869=CARTESIAN_POINT ( 'NONE',  ( -10.81189881249999907, -6.242252689847864744, -159.6562500020484094 ) ) ;
#14871=VERTEX_POINT ( 'NONE', #34780 ) ;
#14872=EDGE_CURVE ( 'NONE', #22602, #23620, #12088, .T. ) ;
#14873=CARTESIAN_POINT ( 'NONE',  ( -9.999999999999998224, 1.224646799147353059E-15, -28.24999999999996803 ) ) ;
#14874=CARTESIAN_POINT ( 'NONE',  ( -2.293366432827344421E-15, -12.48450537969573659, -24.40625000204838457 ) ) ;
#14875=CARTESIAN_POINT ( 'NONE',  ( -9.999999999999998224, 1.224646799147353059E-15, -163.2500000000000000 ) ) ;
#14876=CARTESIAN_POINT ( 'NONE',  ( 9.999999999999998224, 0.000000000000000000, -19.99999999999996092 ) ) ;
#14881=CARTESIAN_POINT ( 'NONE',  ( 10.81189881249999907, 6.242252689847868297, -136.4062500020484094 ) ) ;
#14882=CARTESIAN_POINT ( 'NONE',  ( 10.31059247562686210, 3.150086566999095616, 3.656666817559539767E-15 ) ) ;
#14883=EDGE_CURVE ( 'NONE', #22659, #23066, #19598, .T. ) ;
#14884=CARTESIAN_POINT ( 'NONE',  ( -2.121150477449813534E-15, -11.54700538379251284, -68.75000000409679046 ) ) ;
#14886=CARTESIAN_POINT ( 'NONE',  ( -10.81189881249999729, 1.324075727343319199E-15, -62.28125000204837391 ) ) ;
#14888=ORIENTED_EDGE ( 'NONE', *, *, #34117, .F. ) ;
#14889=VERTEX_POINT ( 'NONE', #42075 ) ;
#14890=CARTESIAN_POINT ( 'NONE',  ( 10.00000000000051159, -5.773502691895965988, -120.6250000000000000 ) ) ;
#14891=CARTESIAN_POINT ( 'NONE',  ( -9.999999999999998224, 1.224646799147353059E-15, -144.1250000040967905 ) ) ;
#14892=CARTESIAN_POINT ( 'NONE',  ( 10.81189881249999907, 6.242252689847868297, -160.2187500020483810 ) ) ;
#14894=CARTESIAN_POINT ( 'NONE',  ( 10.81189881249999907, 6.242252689847868297, -7.218750002048349934 ) ) ;
#14895=CARTESIAN_POINT ( 'NONE',  ( -17.32050807568889539, 1.110223024625133663E-15, 49.99999999999998579 ) ) ;
#14896=CARTESIAN_POINT ( 'NONE',  ( 7.644554776091147741E-16, 12.48450537969573659, -150.9687500020484094 ) ) ;
#14897=CARTESIAN_POINT ( 'NONE',  ( 10.81189881249999551, -6.242252689847874514, -103.6562500020483668 ) ) ;
#14899=CARTESIAN_POINT ( 'NONE',  ( 9.999999999999998224, 0.000000000000000000, -129.8750000040967905 ) ) ;
#14901=CARTESIAN_POINT ( 'NONE',  ( 7.644554776091147741E-16, 12.48450537969573659, -0.9687500020483524876 ) ) ;
#14903=CARTESIAN_POINT ( 'NONE',  ( 7.644554776091147741E-16, 12.48450537969573659, -193.1562500020484094 ) ) ;
#14906=EDGE_CURVE ( 'NONE', #39524, #9909, #28457, .T. ) ;
#14907=CARTESIAN_POINT ( 'NONE',  ( 10.81189881249999551, -6.242252689847874514, -79.46875000204836681 ) ) ;
#14908=CARTESIAN_POINT ( 'NONE',  ( 10.81189881249999551, -6.242252689847874514, -59.96875000204837391 ) ) ;
#14910=CARTESIAN_POINT ( 'NONE',  ( -5.405949406249996869, 9.363379034771805109, -32.53125000204837391 ) ) ;
#14912=CARTESIAN_POINT ( 'NONE',  ( 0.000000000000000000, 0.000000000000000000, -200.0000000000000000 ) ) ;
#14914=CARTESIAN_POINT ( 'NONE',  ( 5.000000000000000000, 8.660254037844385522, -124.7500000000000000 ) ) ;
#14917=CARTESIAN_POINT ( 'NONE',  ( -2.293366432827344421E-15, -12.48450537969573659, -13.90625000204836503 ) ) ;
#14918=ORIENTED_EDGE ( 'NONE', *, *, #40401, .T. ) ;
#14919=( BOUNDED_CURVE ( )  B_SPLINE_CURVE ( 2, ( #32812, #35840, #39484, #23307, #13352, #16161, #35633 ),
 .UNSPECIFIED., .F., .F. ) 
 B_SPLINE_CURVE_WITH_KNOTS ( ( 3, 2, 2, 3 ),
 ( 0.4104477611940299253, 0.4116915422885572551, 0.4129353233830846959, 0.4141791044776120256 ),
 .UNSPECIFIED. ) 
 CURVE ( )  GEOMETRIC_REPRESENTATION_ITEM ( )  RATIONAL_B_SPLINE_CURVE ( ( 0.9999999999999940048, 0.8660254037844447028, 1.000000000000000000, 0.8660254037844387076, 1.000000000000000000, 0.8660254037844267172, 1.000000000000011990 ) ) 
 REPRESENTATION_ITEM ( '' )  );
#14922=CARTESIAN_POINT ( 'NONE',  ( 10.00000000000102318, -5.773502691895667560, -56.50000000409674783 ) ) ;
#14924=CARTESIAN_POINT ( 'NONE',  ( 10.00000000000000000, 5.773502691896255534, -36.75000000409675494 ) ) ;
#14925=CARTESIAN_POINT ( 'NONE',  ( 0.000000000000000000, 0.000000000000000000, -200.0000000000000000 ) ) ;
#14927=( BOUNDED_CURVE ( )  B_SPLINE_CURVE ( 2, ( #224, #13346, #23299, #36457, #6891, #16793, #29993 ),
 .UNSPECIFIED., .F., .F. ) 
 B_SPLINE_CURVE_WITH_KNOTS ( ( 3, 2, 2, 3 ),
 ( 0.4365671641791046276, 0.4378109452736320129, 0.4390547263681593981, 0.4402985074626867279 ),
 .UNSPECIFIED. ) 
 CURVE ( )  GEOMETRIC_REPRESENTATION_ITEM ( )  RATIONAL_B_SPLINE_CURVE ( ( 0.9999999999999820144, 0.8660254037844566932, 1.000000000000000000, 0.8660254037844387076, 1.000000000000000000, 0.8660254037844207220, 1.000000000000017986 ) ) 
 REPRESENTATION_ITEM ( '' )  );
#14928=CARTESIAN_POINT ( 'NONE',  ( 10.00000000000051159, -5.773502691895965988, -99.62499999999997158 ) ) ;
#14929=CARTESIAN_POINT ( 'NONE',  ( -5.405949406250003975, -9.363379034771801557, -149.0312500020483810 ) ) ;
#14930=CARTESIAN_POINT ( 'NONE',  ( -10.81189881249999729, 6.242252689847871849, -129.7187500020483810 ) ) ;
#14931=CARTESIAN_POINT ( 'NONE',  ( -9.999999999999998224, 1.224646799147353059E-15, -3.125000004096767370 ) ) ;
#14935=EDGE_LOOP ( 'NONE', ( #23547, #29452, #16609, #37237 ) ) ;
#14937=CARTESIAN_POINT ( 'NONE',  ( -9.999999999999998224, 1.224646799147353059E-15, -145.6250000040967905 ) ) ;
#14938=CARTESIAN_POINT ( 'NONE',  ( -10.81189881249999729, 6.242252689847871849, -182.2187500020484379 ) ) ;
#14939=CARTESIAN_POINT ( 'NONE',  ( -5.405949406249996869, 9.363379034771805109, -39.84375000204837391 ) ) ;
#14940=CARTESIAN_POINT ( 'NONE',  ( 9.999999999999998224, 0.000000000000000000, -108.4999999999999858 ) ) ;
#14941=CARTESIAN_POINT ( 'NONE',  ( -10.81189881249999729, -6.242252689847864744, -172.9687500020483526 ) ) ;
#14942=CARTESIAN_POINT ( 'NONE',  ( -10.81189881249999729, 1.324075727343319199E-15, -156.5937500020483810 ) ) ;
#14943=CARTESIAN_POINT ( 'NONE',  ( 4.999999999999992006, -8.660254037844389075, -122.6250000040967905 ) ) ;
#14947=CARTESIAN_POINT ( 'NONE',  ( -2.121150477449813534E-15, -11.54700538379251284, -152.3749999999999716 ) ) ;
#14948=CARTESIAN_POINT ( 'NONE',  ( -9.999999999999998224, 1.224646799147353059E-15, -169.2500000000000000 ) ) ;
#14951=CARTESIAN_POINT ( 'NONE',  ( -5.405949406250003975, -9.363379034771801557, -84.34375000204836681 ) ) ;
#14952=CARTESIAN_POINT ( 'NONE',  ( -9.999999999999998224, 1.224646799147353059E-15, -136.2499999999999716 ) ) ;
#14953=CARTESIAN_POINT ( 'NONE',  ( -10.81189881249999729, 1.324075727343319199E-15, -62.28125000204837391 ) ) ;
#14954=DIRECTION ( 'NONE',  ( -0.000000000000000000, -0.000000000000000000, 1.000000000000000000 ) ) ;
#14956=CARTESIAN_POINT ( 'NONE',  ( -5.405949406249996869, 9.363379034771805109, -110.5312500020483810 ) ) ;
#14957=CARTESIAN_POINT ( 'NONE',  ( 10.81189881249999729, 0.000000000000000000, -156.0312500020484094 ) ) ;
#14958=DIRECTION ( 'NONE',  ( 0.5000000000000007772, -0.8660254037844381525, -0.000000000000000000 ) ) ;
#14960=CARTESIAN_POINT ( 'NONE',  ( 9.999999999999996447, -5.773502691896262640, -131.5000000040967905 ) ) ;
#14962=ORIENTED_EDGE ( 'NONE', *, *, #8533, .T. ) ;
#14965=CYLINDRICAL_SURFACE ( 'NONE', #3622, 9.999999999999998224 ) ;
#14966=CARTESIAN_POINT ( 'NONE',  ( -10.81189881249999729, 1.324075727343319199E-15, -177.7812500020484094 ) ) ;
#14969=CARTESIAN_POINT ( 'NONE',  ( -4.999999999999996447, 8.660254037844387298, -58.87500000409676204 ) ) ;
#14970=CARTESIAN_POINT ( 'NONE',  ( 0.000000000000000000, 0.000000000000000000, -200.0000000000000000 ) ) ;
#14971=CARTESIAN_POINT ( 'NONE',  ( -4.999999999999996447, 8.660254037844387298, -130.5000000000000000 ) ) ;
#14973=EDGE_CURVE ( 'NONE', #15207, #28849, #37506, .T. ) ;
#14977=CARTESIAN_POINT ( 'NONE',  ( -2.293366432827344421E-15, -12.48450537969573659, -165.4062500020483810 ) ) ;
#14978=VECTOR ( 'NONE', #30062, 1000.000000000000000 ) ;
#14979=FACE_OUTER_BOUND ( 'NONE', #38107, .T. ) ;
#14980=CARTESIAN_POINT ( 'NONE',  ( -9.999999999999479527, -5.773502691896549521, -82.12499999999997158 ) ) ;
#14981=VERTEX_POINT ( 'NONE', #29784 ) ;
#14982=LINE ( 'NONE', #31211, #5645 ) ;
#14983=CARTESIAN_POINT ( 'NONE',  ( 4.999999999999992006, -8.660254037844389075, -153.7500000000000000 ) ) ;
#14984=CARTESIAN_POINT ( 'NONE',  ( 5.000000000000000000, 8.660254037844385522, -195.6250000040967905 ) ) ;
#14985=CARTESIAN_POINT ( 'NONE',  ( -5.405949406249996869, 9.363379034771805109, -77.53125000204838102 ) ) ;
#14988=CARTESIAN_POINT ( 'NONE',  ( 4.999999999999992006, -8.660254037844389075, -69.74999999999997158 ) ) ;
#14992=CARTESIAN_POINT ( 'NONE',  ( -5.405949406250003975, -9.363379034771801557, -37.84375000204837391 ) ) ;
#14993=CARTESIAN_POINT ( 'NONE',  ( -10.81189881249999907, -6.242252689847864744, -3.656250002048349046 ) ) ;
#14994=CARTESIAN_POINT ( 'NONE',  ( 7.644554776091147741E-16, 12.48450537969573659, -59.46875000204837391 ) ) ;
#14995=ORIENTED_EDGE ( 'NONE', *, *, #20645, .F. ) ;
#14997=ADVANCED_FACE ( 'NONE', ( #39687 ), #20045, .T. ) ;
#14999=CARTESIAN_POINT ( 'NONE',  ( -2.293366432827344421E-15, -12.48450537969573659, -178.7187500020484094 ) ) ;
#15001=CARTESIAN_POINT ( 'NONE',  ( 9.999999999999998224, 0.000000000000000000, -200.0000000000000000 ) ) ;
#15002=EDGE_CURVE ( 'NONE', #30921, #20035, #13779, .T. ) ;
#15003=DIRECTION ( 'NONE',  ( 1.000000000000000000, 0.000000000000000000, 0.000000000000000000 ) ) ;
#15004=CARTESIAN_POINT ( 'NONE',  ( -5.000000000000003553, -8.660254037844383745, -191.8750000040967905 ) ) ;
#15006=CARTESIAN_POINT ( 'NONE',  ( -10.81189881249999729, 1.324075727343319199E-15, -104.0937500020483810 ) ) ;
#15008=CARTESIAN_POINT ( 'NONE',  ( 10.81189881249999551, -6.242252689847874514, -85.65625000204838102 ) ) ;
#15009=CARTESIAN_POINT ( 'NONE',  ( -2.293366432827344421E-15, -12.48450537969573659, -91.71875000204838102 ) ) ;
#15010=VECTOR ( 'NONE', #8400, 1000.000000000000000 ) ;
#15012=CARTESIAN_POINT ( 'NONE',  ( 9.999999999999998224, 0.000000000000000000, -153.8750000040967905 ) ) ;
#15016=DIRECTION ( 'NONE',  ( -1.000000000000000000, -4.506943796211477094E-16, 0.000000000000000000 ) ) ;
#15017=CARTESIAN_POINT ( 'NONE',  ( -9.999999999999612754, -5.773502691896474914, -182.6249999999999716 ) ) ;
#15019=ORIENTED_EDGE ( 'NONE', *, *, #37085, .F. ) ;
#15020=CARTESIAN_POINT ( 'NONE',  ( 9.999999999999996447, -5.773502691896262640, -66.62499999999998579 ) ) ;
#15022=CARTESIAN_POINT ( 'NONE',  ( -4.999999999999996447, 8.660254037844387298, -85.87500000409677625 ) ) ;
#15025=CARTESIAN_POINT ( 'NONE',  ( 5.405949406249999534, 9.363379034771803333, -73.28125000204838102 ) ) ;
#15027=LINE ( 'NONE', #38142, #5723 ) ;
#15030=CARTESIAN_POINT ( 'NONE',  ( -9.999999999999998224, 5.773502691896259087, -4.374999999999956479 ) ) ;
#15032=ADVANCED_FACE ( 'NONE', ( #13130 ), #33016, .T. ) ;
#15033=CARTESIAN_POINT ( 'NONE',  ( -10.81189881249999729, 6.242252689847871849, -2.218750002048358372 ) ) ;
#15035=CARTESIAN_POINT ( 'NONE',  ( 5.405949406249992428, -9.363379034771808662, -142.5937500020483810 ) ) ;
#15036=CARTESIAN_POINT ( 'NONE',  ( 9.999999999999998224, 0.000000000000000000, -107.3750000040967763 ) ) ;
#15038=( BOUNDED_CURVE ( )  B_SPLINE_CURVE ( 2, ( #36727, #7166, #10813, #33512, #17073, #13829, #7594 ),
 .UNSPECIFIED., .F., .F. ) 
 B_SPLINE_CURVE_WITH_KNOTS ( ( 3, 2, 2, 3 ),
 ( 0.6716417910447763928, 0.6728855721393036671, 0.6741293532338310523, 0.6753731343283584376 ),
 .UNSPECIFIED. ) 
 CURVE ( )  GEOMETRIC_REPRESENTATION_ITEM ( )  RATIONAL_B_SPLINE_CURVE ( ( 0.9999999999999761302, 0.8660254037844625774, 1.000000000000000000, 0.8660254037844387076, 1.000000000000000000, 0.8660254037844148378, 1.000000000000023981 ) ) 
 REPRESENTATION_ITEM ( '' )  );
#15039=CARTESIAN_POINT ( 'NONE',  ( -9.999999999999998224, 5.773502691896259087, -182.8750000000000000 ) ) ;
#15041=CARTESIAN_POINT ( 'NONE',  ( -10.81189881249999907, -6.242252689847864744, -98.15625000204839523 ) ) ;
#15042=VERTEX_POINT ( 'NONE', #36667 ) ;
#15043=DIRECTION ( 'NONE',  ( -0.000000000000000000, -0.000000000000000000, 1.000000000000000000 ) ) ;
#15045=VERTEX_POINT ( 'NONE', #12917 ) ;
#15047=CARTESIAN_POINT ( 'NONE',  ( -10.81189881249999729, 6.242252689847871849, -41.40625000204836681 ) ) ;
#15049=CARTESIAN_POINT ( 'NONE',  ( 5.405949406249999534, 9.363379034771803333, -83.59375000204836681 ) ) ;
#15050=CARTESIAN_POINT ( 'NONE',  ( 0.000000000000000000, 0.000000000000000000, -200.0000000000000000 ) ) ;
#15054=CARTESIAN_POINT ( 'NONE',  ( 10.00000000000051159, -5.773502691895965988, -77.12499999999997158 ) ) ;
#15055=CARTESIAN_POINT ( 'NONE',  ( 10.81189881249999551, -6.242252689847874514, -115.4687500020483810 ) ) ;
#15057=CARTESIAN_POINT ( 'NONE',  ( 5.405949406249999534, 9.363379034771803333, -1.281250002048373027 ) ) ;
#15060=CARTESIAN_POINT ( 'NONE',  ( 10.00000000000000000, 5.773502691896255534, -174.7500000040968189 ) ) ;
#15061=CARTESIAN_POINT ( 'NONE',  ( 5.405949406249992428, -9.363379034771808662, -166.7812500020484094 ) ) ;
#15064=CARTESIAN_POINT ( 'NONE',  ( 5.405949406249999534, 9.363379034771803333, -44.59375000204837391 ) ) ;
#15066=CARTESIAN_POINT ( 'NONE',  ( 7.644554776091147741E-16, 12.48450537969573659, -5.656250002048358816 ) ) ;
#15069=CARTESIAN_POINT ( 'NONE',  ( -4.999999999999996447, 8.660254037844387298, -88.49999999999998579 ) ) ;
#15071=CARTESIAN_POINT ( 'NONE',  ( -9.999999999999998224, 1.224646799147353059E-15, -102.1250000040967905 ) ) ;
#15072=AXIS2_PLACEMENT_3D ( 'NONE', #12677, #35384, #18962 ) ;
#15073=CARTESIAN_POINT ( 'NONE',  ( -10.00000000000051337, 5.773502691895962435, -82.37499999999997158 ) ) ;
#15076=CARTESIAN_POINT ( 'NONE',  ( 5.405949406249999534, 9.363379034771803333, -103.2812500020483952 ) ) ;
#15077=VERTEX_POINT ( 'NONE', #10330 ) ;
#15079=DIRECTION ( 'NONE',  ( -0.000000000000000000, -0.000000000000000000, 1.000000000000000000 ) ) ;
#15080=CARTESIAN_POINT ( 'NONE',  ( -5.405949406250003975, -9.363379034771801557, -159.5312500020484094 ) ) ;
#15083=CARTESIAN_POINT ( 'NONE',  ( -4.999999999999996447, 8.660254037844387298, -23.99999999999996447 ) ) ;
#15084=EDGE_CURVE ( 'NONE', #3910, #34292, #41906, .T. ) ;
#15087=CARTESIAN_POINT ( 'NONE',  ( 7.644554776091147741E-16, 12.48450537969573659, -29.65625000204835970 ) ) ;
#15088=CARTESIAN_POINT ( 'NONE',  ( 10.00000000000000000, 5.773502691896255534, -159.3750000000000000 ) ) ;
#15090=EDGE_CURVE ( 'NONE', #30784, #15995, #19413, .T. ) ;
#15091=DIRECTION ( 'NONE',  ( 1.000000000000000000, 0.000000000000000000, 0.000000000000000000 ) ) ;
#15092=CARTESIAN_POINT ( 'NONE',  ( 10.81189881249999551, -6.242252689847874514, -132.1562500020484094 ) ) ;
#15093=CARTESIAN_POINT ( 'NONE',  ( -10.00000000000051337, 5.773502691895962435, -46.37499999999995026 ) ) ;
#15094=CARTESIAN_POINT ( 'NONE',  ( 9.999999999999998224, 0.000000000000000000, -135.5000000000000000 ) ) ;
#15095=VERTEX_POINT ( 'NONE', #19619 ) ;
#15096=CARTESIAN_POINT ( 'NONE',  ( 10.81189881249999907, 6.242252689847868297, -62.90625000204838813 ) ) ;
#15103=CARTESIAN_POINT ( 'NONE',  ( 5.405949406249992428, -9.363379034771808662, -154.5937500020483810 ) ) ;
#15105=CARTESIAN_POINT ( 'NONE',  ( -2.293366432827344421E-15, -12.48450537969573659, -9.218750002048359704 ) ) ;
#15106=AXIS2_PLACEMENT_3D ( 'NONE', #8955, #22118, #35293 ) ;
#15107=EDGE_CURVE ( 'NONE', #10156, #36017, #22385, .T. ) ;
#15108=CARTESIAN_POINT ( 'NONE',  ( 10.81189881249999729, 0.000000000000000000, -137.8437500020484094 ) ) ;
#15109=CARTESIAN_POINT ( 'NONE',  ( 5.405949406249999534, 9.363379034771803333, -98.78125000204839523 ) ) ;
#15111=CARTESIAN_POINT ( 'NONE',  ( 9.999999999999742428, 5.773502691896404748, -187.8750000000000000 ) ) ;
#15113=CARTESIAN_POINT ( 'NONE',  ( -10.81189881249999729, 6.242252689847871849, -0.7187500020483512664 ) ) ;
#15115=CARTESIAN_POINT ( 'NONE',  ( -2.293366432827344421E-15, -12.48450537969573659, -190.9062500020484094 ) ) ;
#15119=CARTESIAN_POINT ( 'NONE',  ( -10.81189881249999729, -6.242252689847864744, -76.96875000204838102 ) ) ;
#15120=CARTESIAN_POINT ( 'NONE',  ( -10.81189881249999907, -6.242252689847864744, -55.96875000204836681 ) ) ;
#15122=CARTESIAN_POINT ( 'NONE',  ( 10.81189881249999551, -6.242252689847874514, -22.65625000204837391 ) ) ;
#15124=CARTESIAN_POINT ( 'NONE',  ( 7.070501591499376803E-16, 11.54700538379251284, -136.6250000000000000 ) ) ;
#15126=CARTESIAN_POINT ( 'NONE',  ( -5.000000000000003553, -8.660254037844383745, -124.0000000000000000 ) ) ;
#15127=( BOUNDED_CURVE ( )  B_SPLINE_CURVE ( 2, ( #12176, #31637, #11751, #38514, #2070, #9163, #5934 ),
 .UNSPECIFIED., .F., .F. ) 
 B_SPLINE_CURVE_WITH_KNOTS ( ( 3, 2, 2, 3 ),
 ( 0.3731343283582090331, 0.3743781094527363629, 0.3756218905472638037, 0.3768656716417911334 ),
 .UNSPECIFIED. ) 
 CURVE ( )  GEOMETRIC_REPRESENTATION_ITEM ( )  RATIONAL_B_SPLINE_CURVE ( ( 0.9999999999999940048, 0.8660254037844447028, 1.000000000000000000, 0.8660254037844387076, 1.000000000000000000, 0.8660254037844267172, 1.000000000000011990 ) ) 
 REPRESENTATION_ITEM ( '' )  );
#15131=CARTESIAN_POINT ( 'NONE',  ( -10.81189881249999729, 6.242252689847871849, -11.40625000204835438 ) ) ;
#15132=ORIENTED_EDGE ( 'NONE', *, *, #32636, .T. ) ;
#15135=DIRECTION ( 'NONE',  ( -0.000000000000000000, -0.000000000000000000, 1.000000000000000000 ) ) ;
#15137=CARTESIAN_POINT ( 'NONE',  ( -4.999999999999996447, 8.660254037844387298, -27.37500000409676204 ) ) ;
#15139=CARTESIAN_POINT ( 'NONE',  ( 7.070501591499376803E-16, 11.54700538379251284, -75.12499999999997158 ) ) ;
#15141=ADVANCED_FACE ( 'NONE', ( #1061 ), #34887, .T. ) ;
#15143=CARTESIAN_POINT ( 'NONE',  ( 5.405949406249999534, 9.363379034771803333, -142.2812500020483810 ) ) ;
#15145=EDGE_CURVE ( 'NONE', #34431, #18400, #3612, .T. ) ;
#15146=CARTESIAN_POINT ( 'NONE',  ( 10.81189881249999729, 0.000000000000000000, -127.3437500020483952 ) ) ;
#15147=CARTESIAN_POINT ( 'NONE',  ( 5.000000000000000000, 8.660254037844385522, -78.62500000409677625 ) ) ;
#15149=ORIENTED_EDGE ( 'NONE', *, *, #42029, .F. ) ;
#15150=ORIENTED_EDGE ( 'NONE', *, *, #42537, .T. ) ;
#15151=ORIENTED_EDGE ( 'NONE', *, *, #23539, .T. ) ;
#15152=EDGE_CURVE ( 'NONE', #33065, #34698, #40009, .T. ) ;
#15153=DIRECTION ( 'NONE',  ( -0.000000000000000000, -0.000000000000000000, 1.000000000000000000 ) ) ;
#15154=CARTESIAN_POINT ( 'NONE',  ( -2.293366432827344421E-15, -12.48450537969573659, -180.2187500020484094 ) ) ;
#15155=CARTESIAN_POINT ( 'NONE',  ( -5.405949406249996869, 9.363379034771805109, -30.84375000204836326 ) ) ;
#15156=CARTESIAN_POINT ( 'NONE',  ( -9.999999999999998224, 1.224646799147353059E-15, -60.12500000409676204 ) ) ;
#15157=CARTESIAN_POINT ( 'NONE',  ( 5.405949406249992428, -9.363379034771808662, -160.5937500020484094 ) ) ;
#15158=CARTESIAN_POINT ( 'NONE',  ( -2.293366432827344421E-15, -12.48450537969573659, -150.2187500020483810 ) ) ;
#15159=FACE_OUTER_BOUND ( 'NONE', #34611, .T. ) ;
#15163=DIRECTION ( 'NONE',  ( -0.000000000000000000, -0.000000000000000000, 1.000000000000000000 ) ) ;
#15165=CARTESIAN_POINT ( 'NONE',  ( 9.999999999999676703, 5.773502691896441164, -183.3749999999999432 ) ) ;
#15167=AXIS2_PLACEMENT_3D ( 'NONE', #15729, #9065, #36031 ) ;
#15168=CARTESIAN_POINT ( 'NONE',  ( 10.81189881249999729, 0.000000000000000000, -79.34375000204838102 ) ) ;
#15170=CARTESIAN_POINT ( 'NONE',  ( 10.81189881249999729, 0.000000000000000000, -58.53125000204836681 ) ) ;
#15173=CARTESIAN_POINT ( 'NONE',  ( 10.81189881249999551, -6.242252689847874514, -114.1562500020483952 ) ) ;
#15174=CARTESIAN_POINT ( 'NONE',  ( 7.644554776091147741E-16, 12.48450537969573659, -149.6562500020484094 ) ) ;
#15175=CARTESIAN_POINT ( 'NONE',  ( 4.999999999999992006, -8.660254037844389075, -29.24999999999997158 ) ) ;
#15177=CARTESIAN_POINT ( 'NONE',  ( -9.999999999999998224, 1.224646799147353059E-15, -118.6250000040967905 ) ) ;
#15179=EDGE_LOOP ( 'NONE', ( #6031, #4929 ) ) ;
#15180=( BOUNDED_CURVE ( )  B_SPLINE_CURVE ( 2, ( #36712, #13181, #26164, #33289, #29612, #26374, #16631 ),
 .UNSPECIFIED., .F., .F. ) 
 B_SPLINE_CURVE_WITH_KNOTS ( ( 3, 2, 2, 3 ),
 ( 0.3843283582089552786, 0.3855721393034826638, 0.3868159203980099936, 0.3880597014925373789 ),
 .UNSPECIFIED. ) 
 CURVE ( )  GEOMETRIC_REPRESENTATION_ITEM ( )  RATIONAL_B_SPLINE_CURVE ( ( 0.9999999999999940048, 0.8660254037844447028, 1.000000000000000000, 0.8660254037844387076, 1.000000000000000000, 0.8660254037844327124, 1.000000000000005995 ) ) 
 REPRESENTATION_ITEM ( '' )  );
#15183=CARTESIAN_POINT ( 'NONE',  ( -10.00000000000102496, 5.773502691895664007, -67.75000000409676204 ) ) ;
#15184=CARTESIAN_POINT ( 'NONE',  ( 10.81189881249999907, 6.242252689847868297, -179.9062500020484094 ) ) ;
#15185=ORIENTED_EDGE ( 'NONE', *, *, #37263, .T. ) ;
#15187=CARTESIAN_POINT ( 'NONE',  ( 9.999999999999998224, 0.000000000000000000, -47.37500000409677625 ) ) ;
#15188=CARTESIAN_POINT ( 'NONE',  ( -9.999999999999998224, 1.224646799147353059E-15, -10.24999999999995381 ) ) ;
#15189=CYLINDRICAL_SURFACE ( 'NONE', #20074, 9.999999999999998224 ) ;
#15193=CARTESIAN_POINT ( 'NONE',  ( 0.000000000000000000, 0.000000000000000000, -200.0000000000000000 ) ) ;
#15194=CARTESIAN_POINT ( 'NONE',  ( -10.81189881249999729, 1.324075727343319199E-15, -171.7812500020484094 ) ) ;
#15195=DIRECTION ( 'NONE',  ( 1.000000000000000000, 0.000000000000000000, 0.000000000000000000 ) ) ;
#15196=CARTESIAN_POINT ( 'NONE',  ( 9.999999999999998224, 0.000000000000000000, -200.0000000000000000 ) ) ;
#15199=CARTESIAN_POINT ( 'NONE',  ( -5.000000000000003553, -8.660254037844383745, -194.5000000000000000 ) ) ;
#15200=CARTESIAN_POINT ( 'NONE',  ( 0.000000000000000000, 0.000000000000000000, -200.0000000000000000 ) ) ;
#15202=EDGE_CURVE ( 'NONE', #35906, #38687, #16561, .T. ) ;
#15203=CARTESIAN_POINT ( 'NONE',  ( 10.81189881249999551, -6.242252689847874514, -78.15625000204838102 ) ) ;
#15206=ORIENTED_EDGE ( 'NONE', *, *, #27256, .F. ) ;
#15207=VERTEX_POINT ( 'NONE', #26465 ) ;
#15208=CARTESIAN_POINT ( 'NONE',  ( 5.405949406249992428, -9.363379034771808662, -25.59375000204835970 ) ) ;
#15209=CARTESIAN_POINT ( 'NONE',  ( 9.999999999999998224, 0.000000000000000000, -144.5000000000000000 ) ) ;
#15210=CARTESIAN_POINT ( 'NONE',  ( 10.81189881249999729, 0.000000000000000000, -4.531250002048375691 ) ) ;
#15211=CARTESIAN_POINT ( 'NONE',  ( 10.81189881249999907, 6.242252689847868297, -58.21875000204836681 ) ) ;
#15212=EDGE_LOOP ( 'NONE', ( #10323, #19537, #4497, #36709 ) ) ;
#15213=DIRECTION ( 'NONE',  ( -0.000000000000000000, -0.000000000000000000, 1.000000000000000000 ) ) ;
#15215=CARTESIAN_POINT ( 'NONE',  ( 10.81189881249999729, 6.242252689847867408, -194.7187500020484094 ) ) ;
#15216=CARTESIAN_POINT ( 'NONE',  ( -10.81189881249999729, 6.242252689847871849, -176.2187500020483810 ) ) ;
#15218=EDGE_CURVE ( 'NONE', #3659, #15095, #37242, .T. ) ;
#15220=CARTESIAN_POINT ( 'NONE',  ( 9.999999999999998224, 0.000000000000000000, -41.37500000409677625 ) ) ;
#15221=CARTESIAN_POINT ( 'NONE',  ( 9.999999999999998224, 0.000000000000000000, -24.49999999999996447 ) ) ;
#15223=CARTESIAN_POINT ( 'NONE',  ( 10.81189881249999551, -6.242252689847874514, -106.4687500020483810 ) ) ;
#15224=CARTESIAN_POINT ( 'NONE',  ( 9.999999999999998224, 0.000000000000000000, -200.0000000000000000 ) ) ;
#15225=CARTESIAN_POINT ( 'NONE',  ( -5.405949406250003975, -9.363379034771801557, -80.03125000204838102 ) ) ;
#15226=CARTESIAN_POINT ( 'NONE',  ( -5.405949406249996869, 9.363379034771805109, -89.34375000204838102 ) ) ;
#15228=CARTESIAN_POINT ( 'NONE',  ( -5.000000000000003553, -8.660254037844383745, -148.3750000040967905 ) ) ;
#15230=AXIS2_PLACEMENT_3D ( 'NONE', #33321, #30081, #3746 ) ;
#15239=CARTESIAN_POINT ( 'NONE',  ( 10.00000000000000000, 5.773502691896255534, -66.37499999999998579 ) ) ;
#15241=CARTESIAN_POINT ( 'NONE',  ( -10.00000000000000000, -5.773502691896251982, -82.50000000409677625 ) ) ;
#15244=CARTESIAN_POINT ( 'NONE',  ( -10.81189881249999729, 1.324075727343319199E-15, -78.78125000204838102 ) ) ;
#15246=LINE ( 'NONE', #15458, #36238 ) ;
#15248=ORIENTED_EDGE ( 'NONE', *, *, #21754, .T. ) ;
#15249=CARTESIAN_POINT ( 'NONE',  ( 7.644554776091147741E-16, 12.48450537969573659, -193.1562500020484094 ) ) ;
#15251=CARTESIAN_POINT ( 'NONE',  ( 7.644554776091147741E-16, 12.48450537969573659, -8.468750002048356151 ) ) ;
#15253=CARTESIAN_POINT ( 'NONE',  ( 7.644554776091147741E-16, 12.48450537969573659, -143.4687500020483810 ) ) ;
#15254=( BOUNDED_CURVE ( )  B_SPLINE_CURVE ( 2, ( #35051, #12354, #21439, #11719, #38272, #25551, #38702 ),
 .UNSPECIFIED., .F., .F. ) 
 B_SPLINE_CURVE_WITH_KNOTS ( ( 3, 2, 2, 3 ),
 ( 0.9328358208955226383, 0.9340796019900500236, 0.9353233830845774088, 0.9365671641791047941 ),
 .UNSPECIFIED. ) 
 CURVE ( )  GEOMETRIC_REPRESENTATION_ITEM ( )  RATIONAL_B_SPLINE_CURVE ( ( 0.9999999999999761302, 0.8660254037844625774, 1.000000000000000000, 0.8660254037844387076, 1.000000000000000000, 0.8660254037844028474, 1.000000000000035971 ) ) 
 REPRESENTATION_ITEM ( '' )  );
#15255=CARTESIAN_POINT ( 'NONE',  ( 5.000000000000000000, 8.660254037844385522, -192.2500000000000000 ) ) ;
#15256=DIRECTION ( 'NONE',  ( 0.5000000000000007772, -0.8660254037844381525, 0.000000000000000000 ) ) ;
#15257=EDGE_CURVE ( 'NONE', #11871, #16838, #10050, .T. ) ;
#15258=CARTESIAN_POINT ( 'NONE',  ( -9.999999999999998224, 5.773502691896259087, -172.3750000000000000 ) ) ;
#15260=CARTESIAN_POINT ( 'NONE',  ( -10.81189881249999907, -6.242252689847864744, -101.1562500020483952 ) ) ;
#15262=CARTESIAN_POINT ( 'NONE',  ( -5.000000000000003553, -8.660254037844383745, -161.8750000040967905 ) ) ;
#15263=ORIENTED_EDGE ( 'NONE', *, *, #39587, .F. ) ;
#15264=EDGE_LOOP ( 'NONE', ( #15887, #26633, #13180, #5732 ) ) ;
#15266=CARTESIAN_POINT ( 'NONE',  ( -10.81189881249999907, -6.242252689847864744, -33.65625000204836681 ) ) ;
#15269=CARTESIAN_POINT ( 'NONE',  ( 10.81189881249999551, -6.242252689847874514, -85.46875000204836681 ) ) ;
#15270=CARTESIAN_POINT ( 'NONE',  ( 9.999999999999998224, 0.000000000000000000, -3.875000004096768258 ) ) ;
#15271=EDGE_CURVE ( 'NONE', #5984, #24638, #13694, .T. ) ;
#15273=CARTESIAN_POINT ( 'NONE',  ( -9.999999999998969713, -5.773502691896847949, -130.5000000040967905 ) ) ;
#15275=CARTESIAN_POINT ( 'NONE',  ( -4.999999999999996447, 8.660254037844387298, -13.87500000409674961 ) ) ;
#15276=AXIS2_PLACEMENT_3D ( 'NONE', #31330, #17270, #13815 ) ;
#15278=CARTESIAN_POINT ( 'NONE',  ( 7.644554776091147741E-16, 12.48450537969573659, -117.9687500020483668 ) ) ;
#15282=CARTESIAN_POINT ( 'NONE',  ( 7.070501591499377789E-16, 11.54700538379251284, -168.5000000040967905 ) ) ;
#15283=CARTESIAN_POINT ( 'NONE',  ( 10.81189881249999729, 6.242252689847867408, -170.9062500020484094 ) ) ;
#15284=CARTESIAN_POINT ( 'NONE',  ( 7.070501591499376803E-16, 11.54700538379251284, -69.12499999999998579 ) ) ;
#15287=CARTESIAN_POINT ( 'NONE',  ( 7.644554776091147741E-16, 12.48450537969573659, -47.46875000204836681 ) ) ;
#15289=CARTESIAN_POINT ( 'NONE',  ( 5.405949406249999534, 9.363379034771803333, -4.281250002048375691 ) ) ;
#15291=CARTESIAN_POINT ( 'NONE',  ( 0.000000000000000000, 0.000000000000000000, -200.0000000000000000 ) ) ;
#15293=CARTESIAN_POINT ( 'NONE',  ( 9.999999999999996447, -5.773502691896262640, -89.12499999999997158 ) ) ;
#15295=CARTESIAN_POINT ( 'NONE',  ( -10.00000000000000000, -5.773502691896251982, -109.5000000040967905 ) ) ;
#15299=CARTESIAN_POINT ( 'NONE',  ( -10.81189881249999729, 6.242252689847871849, -98.40625000204838102 ) ) ;
#15300=ORIENTED_EDGE ( 'NONE', *, *, #10422, .F. ) ;
#15301=( BOUNDED_CURVE ( )  B_SPLINE_CURVE ( 2, ( #28488, #31299, #21782, #38182, #41180, #7980, #1942 ),
 .UNSPECIFIED., .F., .F. ) 
 B_SPLINE_CURVE_WITH_KNOTS ( ( 3, 2, 2, 3 ),
 ( 0.7238805970149256863, 0.7251243781094530716, 0.7263681592039803459, 0.7276119402985077311 ),
 .UNSPECIFIED. ) 
 CURVE ( )  GEOMETRIC_REPRESENTATION_ITEM ( )  RATIONAL_B_SPLINE_CURVE ( ( 0.9999999999999641398, 0.8660254037844745678, 1.000000000000000000, 0.8660254037844387076, 1.000000000000000000, 0.8660254037844148378, 1.000000000000023981 ) ) 
 REPRESENTATION_ITEM ( '' )  );
#15303=CARTESIAN_POINT ( 'NONE',  ( -10.00000000000051337, 5.773502691895962435, -71.87499999999998579 ) ) ;
#15304=CARTESIAN_POINT ( 'NONE',  ( 10.81189881249999551, -6.242252689847874514, -154.6562500020484379 ) ) ;
#15307=CARTESIAN_POINT ( 'NONE',  ( 9.999999999999998224, 0.000000000000000000, -18.49999999999996092 ) ) ;
#15308=CARTESIAN_POINT ( 'NONE',  ( -10.81189881249999729, 1.324075727343319199E-15, -27.78125000204837036 ) ) ;
#15309=CARTESIAN_POINT ( 'NONE',  ( 7.070501591499377789E-16, 11.54700538379251284, -153.1250000000000000 ) ) ;
#15311=AXIS2_PLACEMENT_3D ( 'NONE', #37776, #20940, #21590 ) ;
#15312=CARTESIAN_POINT ( 'NONE',  ( 5.000000000000000000, 8.660254037844385522, -199.7500000000000000 ) ) ;
#15313=CARTESIAN_POINT ( 'NONE',  ( 10.81189881249999729, 0.000000000000000000, -127.5312500020483952 ) ) ;
#15314=CARTESIAN_POINT ( 'NONE',  ( -9.999999999999998224, 1.224646799147353059E-15, -22.24999999999996447 ) ) ;
#15315=CARTESIAN_POINT ( 'NONE',  ( -9.999999999999776179, -5.773502691896382544, -188.6250000000000568 ) ) ;
#15316=ORIENTED_EDGE ( 'NONE', *, *, #22547, .F. ) ;
#15317=CARTESIAN_POINT ( 'NONE',  ( -10.81189881249999729, 6.242252689847871849, -57.90625000204838813 ) ) ;
#15319=CARTESIAN_POINT ( 'NONE',  ( -5.405949406249996869, 9.363379034771805109, -114.8437500020483810 ) ) ;
#15322=CYLINDRICAL_SURFACE ( 'NONE', #25930, 9.999999999999998224 ) ;
#15324=CARTESIAN_POINT ( 'NONE',  ( 10.81189881249999729, 0.000000000000000000, -161.8437500020484094 ) ) ;
#15326=CARTESIAN_POINT ( 'NONE',  ( -5.405949406250003975, -9.363379034771801557, -7.843750002048343717 ) ) ;
#15327=EDGE_CURVE ( 'NONE', #42072, #14017, #18211, .T. ) ;
#15328=CARTESIAN_POINT ( 'NONE',  ( 10.81189881249999729, 6.242252689847867408, -140.7187500020483810 ) ) ;
#15330=CARTESIAN_POINT ( 'NONE',  ( 0.000000000000000000, 0.000000000000000000, -200.0000000000000000 ) ) ;
#15332=CARTESIAN_POINT ( 'NONE',  ( -10.81189881249999729, 6.242252689847871849, -2.218750002048357928 ) ) ;
#15334=CARTESIAN_POINT ( 'NONE',  ( 10.81189881249999729, 6.242252689847867408, -197.9062500020484379 ) ) ;
#15338=CARTESIAN_POINT ( 'NONE',  ( 5.405949406249999534, 9.363379034771803333, -68.59375000204836681 ) ) ;
#15339=CARTESIAN_POINT ( 'NONE',  ( 5.405949406249999534, 9.363379034771803333, -61.09375000204836681 ) ) ;
#15341=CARTESIAN_POINT ( 'NONE',  ( -5.405949406250003975, -9.363379034771801557, -27.53125000204836681 ) ) ;
#15344=CARTESIAN_POINT ( 'NONE',  ( -9.999999999999998224, 5.773502691896259087, -113.8750000000000000 ) ) ;
#15348=CARTESIAN_POINT ( 'NONE',  ( 5.405949406249992428, -9.363379034771808662, -12.28125000204835438 ) ) ;
#15349=ORIENTED_EDGE ( 'NONE', *, *, #20048, .T. ) ;
#15354=CARTESIAN_POINT ( 'NONE',  ( -9.999999999999998224, 5.773502691896259087, -50.87499999999998579 ) ) ;
#15355=CARTESIAN_POINT ( 'NONE',  ( 5.000000000000000000, 8.660254037844385522, -23.12500000409675849 ) ) ;
#15356=CARTESIAN_POINT ( 'NONE',  ( 9.999999999999998224, 0.000000000000000000, -13.99999999999995737 ) ) ;
#15358=CYLINDRICAL_SURFACE ( 'NONE', #17265, 9.999999999999998224 ) ;
#15359=CARTESIAN_POINT ( 'NONE',  ( 10.81189881249999551, -6.242252689847874514, -145.6562500020484094 ) ) ;
#15360=CARTESIAN_POINT ( 'NONE',  ( -10.81189881249999729, 1.324075727343319199E-15, -152.2812500020484094 ) ) ;
#15362=CARTESIAN_POINT ( 'NONE',  ( 10.00000000000051159, -5.773502691895965988, -127.0000000040967763 ) ) ;
#15363=VERTEX_POINT ( 'NONE', #16941 ) ;
#15364=EDGE_LOOP ( 'NONE', ( #18758, #38403, #38520, #18242 ) ) ;
#15366=CARTESIAN_POINT ( 'NONE',  ( 4.999999999999992006, -8.660254037844389075, -100.1250000040967905 ) ) ;
#15367=CARTESIAN_POINT ( 'NONE',  ( -5.405949406249996869, 9.363379034771805109, -179.3437500020483810 ) ) ;
#15368=CARTESIAN_POINT ( 'NONE',  ( -5.405949406250003975, -9.363379034771801557, -33.34375000204836681 ) ) ;
#15369=CARTESIAN_POINT ( 'NONE',  ( 9.999999999999479527, 5.773502691896553074, -118.8749999999999858 ) ) ;
#15371=CARTESIAN_POINT ( 'NONE',  ( 7.644554776091147741E-16, 12.48450537969573659, -164.4687500020483810 ) ) ;
#15372=CARTESIAN_POINT ( 'NONE',  ( -10.81189881249999729, 6.242252689847871849, -149.2187500020484379 ) ) ;
#15373=CARTESIAN_POINT ( 'NONE',  ( -9.999999999999998224, 1.224646799147353059E-15, -88.62500000409677625 ) ) ;
#15377=EDGE_CURVE ( 'NONE', #32801, #14436, #5627, .T. ) ;
#15378=CARTESIAN_POINT ( 'NONE',  ( -9.999999999999998224, 1.224646799147353059E-15, -128.7499999999999716 ) ) ;
#15379=CARTESIAN_POINT ( 'NONE',  ( 5.000000000000000000, 8.660254037844385522, -183.2500000000000000 ) ) ;
#15382=CARTESIAN_POINT ( 'NONE',  ( 10.81189881249999907, 6.242252689847868297, -83.71875000204836681 ) ) ;
#15383=DIRECTION ( 'NONE',  ( -0.000000000000000000, -0.000000000000000000, 1.000000000000000000 ) ) ;
#15384=CARTESIAN_POINT ( 'NONE',  ( 7.644554776091147741E-16, 12.48450537969573659, -53.65625000204838102 ) ) ;
#15387=CARTESIAN_POINT ( 'NONE',  ( -10.00000000000000000, -5.773502691896251982, -136.1250000000000000 ) ) ;
#15388=CARTESIAN_POINT ( 'NONE',  ( -2.293366432827344421E-15, -12.48450537969573659, -144.4062500020484094 ) ) ;
#15390=CARTESIAN_POINT ( 'NONE',  ( 9.999999999999998224, 0.000000000000000000, -69.49999999999997158 ) ) ;
#15392=CARTESIAN_POINT ( 'NONE',  ( 4.999999999999992006, -8.660254037844389075, -124.1250000040967905 ) ) ;
#15394=VERTEX_POINT ( 'NONE', #21257 ) ;
#15397=CARTESIAN_POINT ( 'NONE',  ( -9.999999999999998224, 1.224646799147353059E-15, -154.6250000040967905 ) ) ;
#15398=CARTESIAN_POINT ( 'NONE',  ( 10.81189881249999907, 6.242252689847868297, -182.9062500020484094 ) ) ;
#15399=ORIENTED_EDGE ( 'NONE', *, *, #33696, .F. ) ;
#15400=CARTESIAN_POINT ( 'NONE',  ( 10.00000000000000000, 5.773502691896255534, -47.25000000409676915 ) ) ;
#15401=DIRECTION ( 'NONE',  ( 1.000000000000000000, 0.000000000000000000, 0.000000000000000000 ) ) ;
#15403=FACE_BOUND ( 'NONE', #12757, .T. ) ;
#15404=CARTESIAN_POINT ( 'NONE',  ( -2.293366432827344421E-15, -12.48450537969573659, -171.4062500020484379 ) ) ;
#15405=EDGE_CURVE ( 'NONE', #3969, #8277, #1635, .T. ) ;
#15406=PLANE ( 'NONE',  #24264 ) ;
#15407=FACE_OUTER_BOUND ( 'NONE', #30364, .T. ) ;
#15409=DIRECTION ( 'NONE',  ( -0.000000000000000000, -0.000000000000000000, 1.000000000000000000 ) ) ;
#15412=CARTESIAN_POINT ( 'NONE',  ( 9.999999999998969713, 5.773502691896851502, -27.37499999999996092 ) ) ;
#15413=CARTESIAN_POINT ( 'NONE',  ( 10.81189881249999729, 0.000000000000000000, -75.03125000204838102 ) ) ;
#15414=ORIENTED_EDGE ( 'NONE', *, *, #11683, .T. ) ;
#15416=CARTESIAN_POINT ( 'NONE',  ( -2.121150477449813534E-15, -11.54700538379251284, -143.3750000000000000 ) ) ;
#15417=ORIENTED_EDGE ( 'NONE', *, *, #41370, .T. ) ;
#15418=ORIENTED_EDGE ( 'NONE', *, *, #41781, .T. ) ;
#15419=CARTESIAN_POINT ( 'NONE',  ( -5.405949406250003975, -9.363379034771801557, -30.34375000204836326 ) ) ;
#15422=CARTESIAN_POINT ( 'NONE',  ( -10.81189881249999907, -6.242252689847864744, -9.656250002048379244 ) ) ;
#15423=CARTESIAN_POINT ( 'NONE',  ( 5.405949406249999534, 9.363379034771803333, -56.59375000204835970 ) ) ;
#15427=CARTESIAN_POINT ( 'NONE',  ( 7.644554776091147741E-16, 12.48450537969573659, -189.9687500020484094 ) ) ;
#15428=CARTESIAN_POINT ( 'NONE',  ( 5.405949406249999534, 9.363379034771803333, -181.0937500020483810 ) ) ;
#15431=CARTESIAN_POINT ( 'NONE',  ( 9.999999999999998224, 0.000000000000000000, -165.5000000000000000 ) ) ;
#15432=( BOUNDED_CURVE ( )  B_SPLINE_CURVE ( 2, ( #18443, #8325, #34653, #11962, #25152, #38300, #8745 ),
 .UNSPECIFIED., .F., .F. ) 
 B_SPLINE_CURVE_WITH_KNOTS ( ( 3, 2, 2, 3 ),
 ( 0.9776119402985076201, 0.9788557213930348944, 0.9800995024875623907, 0.9813432835820897759 ),
 .UNSPECIFIED. ) 
 CURVE ( )  GEOMETRIC_REPRESENTATION_ITEM ( )  RATIONAL_B_SPLINE_CURVE ( ( 0.9999999999999880096, 0.8660254037844506980, 1.000000000000000000, 0.8660254037844387076, 1.000000000000000000, 0.8660254037844148378, 1.000000000000023981 ) ) 
 REPRESENTATION_ITEM ( '' )  );
#15433=DIRECTION ( 'NONE',  ( -0.000000000000000000, -0.000000000000000000, 1.000000000000000000 ) ) ;
#15435=CARTESIAN_POINT ( 'NONE',  ( 7.644554776091147741E-16, 12.48450537969573659, -101.4687500020483668 ) ) ;
#15436=CARTESIAN_POINT ( 'NONE',  ( -9.999999999999998224, 1.224646799147353059E-15, -73.24999999999998579 ) ) ;
#15437=CARTESIAN_POINT ( 'NONE',  ( 10.81189881249999551, -6.242252689847874514, -70.65625000204839523 ) ) ;
#15438=CARTESIAN_POINT ( 'NONE',  ( 5.405949406249999534, 9.363379034771803333, -94.09375000204838102 ) ) ;
#15440=CARTESIAN_POINT ( 'NONE',  ( -10.00000000000000000, -5.773502691896251982, -145.5000000040967905 ) ) ;
#15445=EDGE_CURVE ( 'NONE', #8390, #35567, #33107, .T. ) ;
#15446=CARTESIAN_POINT ( 'NONE',  ( -10.00000000000012790, -5.773502691896178263, -175.1250000000000284 ) ) ;
#15447=CARTESIAN_POINT ( 'NONE',  ( -9.999999999999998224, 1.224646799147353059E-15, -148.2500000000000000 ) ) ;
#15449=ORIENTED_EDGE ( 'NONE', *, *, #30112, .T. ) ;
#15450=CARTESIAN_POINT ( 'NONE',  ( -10.00000000000000000, -5.773502691896251982, -65.62499999999998579 ) ) ;
#15452=CARTESIAN_POINT ( 'NONE',  ( 4.999999999999992006, -8.660254037844389075, -77.62500000409677625 ) ) ;
#15456=CARTESIAN_POINT ( 'NONE',  ( -10.81189881249999729, 6.242252689847871849, -71.40625000204838102 ) ) ;
#15458=CARTESIAN_POINT ( 'NONE',  ( 9.999999999999998224, 0.000000000000000000, -200.0000000000000000 ) ) ;
#15461=CARTESIAN_POINT ( 'NONE',  ( 10.81189881249999729, 0.000000000000000000, -190.5312500020484094 ) ) ;
#15463=CARTESIAN_POINT ( 'NONE',  ( 10.81189881249999729, 0.000000000000000000, -2.843750002048367698 ) ) ;
#15464=CARTESIAN_POINT ( 'NONE',  ( -9.999999999999998224, 1.224646799147353059E-15, -63.12500000409676204 ) ) ;
#15465=CARTESIAN_POINT ( 'NONE',  ( -9.999999999999479527, -5.773502691896549521, -112.5000000040967478 ) ) ;
#15466=CARTESIAN_POINT ( 'NONE',  ( -9.999999999999998224, 1.224646799147353059E-15, -175.2500000000000284 ) ) ;
#15467=CARTESIAN_POINT ( 'NONE',  ( -9.999999999999998224, 1.224646799147353059E-15, -1.249999999999973355 ) ) ;
#15468=CARTESIAN_POINT ( 'NONE',  ( -10.81189881249999729, 6.242252689847871849, -102.9062500020483810 ) ) ;
#15469=ORIENTED_EDGE ( 'NONE', *, *, #2974, .F. ) ;
#15470=CARTESIAN_POINT ( 'NONE',  ( -9.999999999999998224, 1.224646799147353059E-15, -162.1250000040967905 ) ) ;
#15472=ORIENTED_EDGE ( 'NONE', *, *, #3823, .F. ) ;
#15473=CARTESIAN_POINT ( 'NONE',  ( 10.81189881249999551, -6.242252689847874514, -33.15625000204835970 ) ) ;
#15475=CARTESIAN_POINT ( 'NONE',  ( 10.81189881249999551, -6.242252689847874514, -77.96875000204838102 ) ) ;
#15477=CARTESIAN_POINT ( 'NONE',  ( -10.81189881249999907, -6.242252689847864744, -198.4687500020484379 ) ) ;
#15480=CARTESIAN_POINT ( 'NONE',  ( 7.070501591499377789E-16, 11.54700538379251284, -12.50000000409677092 ) ) ;
#15481=CARTESIAN_POINT ( 'NONE',  ( -5.000000000000003553, -8.660254037844383745, -86.49999999999998579 ) ) ;
#15482=CARTESIAN_POINT ( 'NONE',  ( -10.81189881249999729, 1.324075727343319199E-15, -132.5937500020483810 ) ) ;
#15483=CARTESIAN_POINT ( 'NONE',  ( -10.81189881249999729, 6.242252689847871849, -113.2187500020483810 ) ) ;
#15486=CARTESIAN_POINT ( 'NONE',  ( -4.999999999999996447, 8.660254037844387298, -168.3750000040967905 ) ) ;
#15487=CARTESIAN_POINT ( 'NONE',  ( 5.405949406249992428, -9.363379034771808662, -174.2812500020484094 ) ) ;
#15488=CARTESIAN_POINT ( 'NONE',  ( 9.999999999999998224, 0.000000000000000000, -200.0000000000000000 ) ) ;
#15491=CARTESIAN_POINT ( 'NONE',  ( 10.81189881249999551, -6.242252689847874514, -43.46875000204835970 ) ) ;
#15493=CARTESIAN_POINT ( 'NONE',  ( 5.000000000000000000, 8.660254037844385522, -86.12500000409677625 ) ) ;
#15496=CARTESIAN_POINT ( 'NONE',  ( 10.00000000000000000, 5.773502691896255534, -85.87499999999997158 ) ) ;
#15498=CARTESIAN_POINT ( 'NONE',  ( 7.070501591499377789E-16, 11.54700538379251284, -98.00000000409677625 ) ) ;
#15499=( BOUNDED_CURVE ( )  B_SPLINE_CURVE ( 2, ( #38018, #34577, #5434, #41451, #22044, #27880, #5007 ),
 .UNSPECIFIED., .F., .F. ) 
 B_SPLINE_CURVE_WITH_KNOTS ( ( 3, 2, 2, 3 ),
 ( 0.1641791044776119424, 0.1654228855721392999, 0.1666666666666666574, 0.1679104477611940427 ),
 .UNSPECIFIED. ) 
 CURVE ( )  GEOMETRIC_REPRESENTATION_ITEM ( )  RATIONAL_B_SPLINE_CURVE ( ( 1.000000000000000000, 0.8660254037844387076, 1.000000000000000000, 0.8660254037844387076, 1.000000000000000000, 0.8660254037844387076, 1.000000000000000000 ) ) 
 REPRESENTATION_ITEM ( '' )  );
#15502=CARTESIAN_POINT ( 'NONE',  ( -10.81189881249999729, -6.242252689847864744, -99.65625000204839523 ) ) ;
#15504=AXIS2_PLACEMENT_3D ( 'NONE', #29324, #3212, #16339 ) ;
#15506=CARTESIAN_POINT ( 'NONE',  ( 5.000000000000000000, 8.660254037844385522, -72.24999999999998579 ) ) ;
#15507=CARTESIAN_POINT ( 'NONE',  ( 5.405949406249999534, 9.363379034771803333, -160.2812500020484094 ) ) ;
#15510=CARTESIAN_POINT ( 'NONE',  ( 9.999999999999998224, 0.000000000000000000, -13.99999999999995737 ) ) ;
#15511=CARTESIAN_POINT ( 'NONE',  ( -5.405949406249996869, 9.363379034771805109, -25.03125000204836681 ) ) ;
#15512=CARTESIAN_POINT ( 'NONE',  ( 5.000000000000000000, 8.660254037844385522, -151.7500000000000000 ) ) ;
#15514=EDGE_CURVE ( 'NONE', #18936, #6937, #3347, .T. ) ;
#15515=CARTESIAN_POINT ( 'NONE',  ( 10.00000000000000000, 5.773502691896255534, -198.3750000000000000 ) ) ;
#15516=CARTESIAN_POINT ( 'NONE',  ( -5.405949406250003975, -9.363379034771801557, -129.5312500020484094 ) ) ;
#15518=CARTESIAN_POINT ( 'NONE',  ( -9.999999999999998224, 1.224646799147353059E-15, -13.24999999999995559 ) ) ;
#15521=CARTESIAN_POINT ( 'NONE',  ( 5.405949406249992428, -9.363379034771808662, -52.78125000204836681 ) ) ;
#15523=CARTESIAN_POINT ( 'NONE',  ( -2.293366432827344421E-15, -12.48450537969573659, -102.2187500020483952 ) ) ;
#15524=EDGE_LOOP ( 'NONE', ( #30524, #35778, #18460, #8759 ) ) ;
#15527=FACE_OUTER_BOUND ( 'NONE', #22541, .T. ) ;
#15529=CARTESIAN_POINT ( 'NONE',  ( -10.81189881249999729, 1.324075727343319199E-15, -158.0937500020483810 ) ) ;
#15531=CARTESIAN_POINT ( 'NONE',  ( -5.405949406250003975, -9.363379034771801557, -9.343750002048345493 ) ) ;
#15533=EDGE_CURVE ( 'NONE', #8915, #10633, #17365, .T. ) ;
#15534=CARTESIAN_POINT ( 'NONE',  ( -5.405949406250003975, -9.363379034771801557, -139.8437500020484094 ) ) ;
#15536=CARTESIAN_POINT ( 'NONE',  ( 5.321294541346989426, -5.321294541346989426, -220.0000000000000000 ) ) ;
#15538=CARTESIAN_POINT ( 'NONE',  ( -2.121150477449813534E-15, -11.54700538379251284, -191.7500000040967905 ) ) ;
#15540=CARTESIAN_POINT ( 'NONE',  ( -10.81189881249999729, 1.324075727343319199E-15, -192.7812500020484094 ) ) ;
#15541=( BOUNDED_CURVE ( )  B_SPLINE_CURVE ( 2, ( #35050, #38913, #2258, #18627, #8928, #34837, #15378 ),
 .UNSPECIFIED., .F., .F. ) 
 B_SPLINE_CURVE_WITH_KNOTS ( ( 3, 2, 2, 3 ),
 ( 0.3507462686567164867, 0.3519900497512438720, 0.3532338308457712572, 0.3544776119402986980 ),
 .UNSPECIFIED. ) 
 CURVE ( )  GEOMETRIC_REPRESENTATION_ITEM ( )  RATIONAL_B_SPLINE_CURVE ( ( 0.9999999999999940048, 0.8660254037844447028, 1.000000000000000000, 0.8660254037844387076, 1.000000000000000000, 0.8660254037844207220, 1.000000000000017986 ) ) 
 REPRESENTATION_ITEM ( '' )  );
#15545=CARTESIAN_POINT ( 'NONE',  ( 5.405949406249999534, 9.363379034771803333, -70.09375000204836681 ) ) ;
#15546=CARTESIAN_POINT ( 'NONE',  ( -10.81189881249999729, 1.324075727343319199E-15, -54.59375000204835970 ) ) ;
#15548=CARTESIAN_POINT ( 'NONE',  ( 5.405949406249999534, 9.363379034771803333, -23.78125000204836681 ) ) ;
#15552=CARTESIAN_POINT ( 'NONE',  ( 5.000000000000000000, 8.660254037844385522, -112.7499999999999858 ) ) ;
#15553=LINE ( 'NONE', #12531, #34852 ) ;
#15557=CARTESIAN_POINT ( 'NONE',  ( 10.81189881249999729, 0.000000000000000000, -10.53125000204835260 ) ) ;
#15558=ORIENTED_EDGE ( 'NONE', *, *, #26514, .F. ) ;
#15559=VECTOR ( 'NONE', #27747, 1000.000000000000114 ) ;
#15560=CARTESIAN_POINT ( 'NONE',  ( -9.999999999999998224, 1.224646799147353059E-15, -121.2500000000000000 ) ) ;
#15562=CARTESIAN_POINT ( 'NONE',  ( 9.999999999999998224, 0.000000000000000000, -86.37500000409677625 ) ) ;
#15564=CARTESIAN_POINT ( 'NONE',  ( 10.00000000000000000, 5.773502691896255534, -37.87499999999995737 ) ) ;
#15565=CARTESIAN_POINT ( 'NONE',  ( -9.999999999999998224, 5.773502691896259087, -28.75000000409675138 ) ) ;
#15566=CARTESIAN_POINT ( 'NONE',  ( 10.81189881249999729, 6.242252689847867408, -53.90625000204838102 ) ) ;
#15569=DIRECTION ( 'NONE',  ( 1.000000000000000000, 0.000000000000000000, 0.000000000000000000 ) ) ;
#15570=CARTESIAN_POINT ( 'NONE',  ( 5.405949406249999534, 9.363379034771803333, -143.7812500020483810 ) ) ;
#15571=CARTESIAN_POINT ( 'NONE',  ( 5.405949406249999534, 9.363379034771803333, -149.7812500020483810 ) ) ;
#15573=DIRECTION ( 'NONE',  ( -0.000000000000000000, -0.000000000000000000, 1.000000000000000000 ) ) ;
#15574=ORIENTED_EDGE ( 'NONE', *, *, #35571, .F. ) ;
#15575=EDGE_LOOP ( 'NONE', ( #5352, #24526, #31969, #9580 ) ) ;
#15576=VERTEX_POINT ( 'NONE', #24088 ) ;
#15577=VECTOR ( 'NONE', #4936, 1000.000000000000000 ) ;
#15578=DIRECTION ( 'NONE',  ( 1.000000000000000000, 0.000000000000000000, 0.000000000000000000 ) ) ;
#15579=CARTESIAN_POINT ( 'NONE',  ( 10.81189881249999907, 6.242252689847868297, -184.2187500020483810 ) ) ;
#15580=CARTESIAN_POINT ( 'NONE',  ( -5.405949406249996869, 9.363379034771805109, -33.84375000204836681 ) ) ;
#15581=CARTESIAN_POINT ( 'NONE',  ( 9.999999999999998224, 0.000000000000000000, -109.9999999999999858 ) ) ;
#15582=CARTESIAN_POINT ( 'NONE',  ( -5.405949406250003975, -9.363379034771801557, -162.3437500020484094 ) ) ;
#15583=CARTESIAN_POINT ( 'NONE',  ( -5.405949406249996869, 9.363379034771805109, -153.8437500020483810 ) ) ;
#15584=CARTESIAN_POINT ( 'NONE',  ( -9.999999999999998224, 1.224646799147353059E-15, -200.0000000000000000 ) ) ;
#15587=CARTESIAN_POINT ( 'NONE',  ( 7.644554776091147741E-16, 12.48450537969573659, -17.46875000204836681 ) ) ;
#15589=DIRECTION ( 'NONE',  ( -0.000000000000000000, -0.000000000000000000, 1.000000000000000000 ) ) ;
#15590=CARTESIAN_POINT ( 'NONE',  ( -9.999999999999998224, 1.224646799147353059E-15, -157.2500000000000000 ) ) ;
#15592=CARTESIAN_POINT ( 'NONE',  ( 5.405949406249999534, 9.363379034771803333, -85.09375000204836681 ) ) ;
#15593=CARTESIAN_POINT ( 'NONE',  ( -10.81189881249999729, 1.324075727343319199E-15, -51.78125000204835970 ) ) ;
#15597=CARTESIAN_POINT ( 'NONE',  ( 10.00000000000000000, 5.773502691896255534, -136.8750000000000000 ) ) ;
#15598=CARTESIAN_POINT ( 'NONE',  ( -10.81189881249999729, -6.242252689847864744, -143.1562500020484094 ) ) ;
#15599=CARTESIAN_POINT ( 'NONE',  ( 9.999999999999998224, 0.000000000000000000, -111.8750000040967763 ) ) ;
#15601=CARTESIAN_POINT ( 'NONE',  ( 10.00000000000000000, 5.773502691896255534, -120.7500000040967905 ) ) ;
#15603=ORIENTED_EDGE ( 'NONE', *, *, #8320, .F. ) ;
#15606=CARTESIAN_POINT ( 'NONE',  ( 5.000000000000000000, 8.660254037844385522, -52.74999999999996447 ) ) ;
#15607=CARTESIAN_POINT ( 'NONE',  ( -5.405949406250003975, -9.363379034771801557, -170.0312500020484094 ) ) ;
#15608=CARTESIAN_POINT ( 'NONE',  ( -5.000000000000003553, -8.660254037844383745, -46.37500000409677625 ) ) ;
#15609=CARTESIAN_POINT ( 'NONE',  ( 10.00000000000051159, -5.773502691895965988, -98.12499999999998579 ) ) ;
#15612=CARTESIAN_POINT ( 'NONE',  ( 10.81189881249999729, 0.000000000000000000, -171.0312500020484094 ) ) ;
#15614=CARTESIAN_POINT ( 'NONE',  ( 4.999999999999992006, -8.660254037844389075, -177.7500000000000284 ) ) ;
#15615=EDGE_CURVE ( 'NONE', #16149, #26720, #4010, .T. ) ;
#15617=EDGE_CURVE ( 'NONE', #35866, #13495, #40664, .T. ) ;
#15618=FACE_OUTER_BOUND ( 'NONE', #37402, .T. ) ;
#15619=EDGE_CURVE ( 'NONE', #24959, #14677, #995, .T. ) ;
#15620=CARTESIAN_POINT ( 'NONE',  ( -10.81189881249999907, -6.242252689847864744, -75.65625000204839523 ) ) ;
#15621=ORIENTED_EDGE ( 'NONE', *, *, #41083, .F. ) ;
#15622=CARTESIAN_POINT ( 'NONE',  ( 9.999999999999998224, 0.000000000000000000, -30.49999999999997158 ) ) ;
#15623=ORIENTED_EDGE ( 'NONE', *, *, #20097, .T. ) ;
#15626=CARTESIAN_POINT ( 'NONE',  ( -10.81189881249999729, 1.324075727343319199E-15, -27.59375000204836326 ) ) ;
#15627=CARTESIAN_POINT ( 'NONE',  ( -10.81189881249999907, -6.242252689847864744, -2.156250002048373915 ) ) ;
#15628=CARTESIAN_POINT ( 'NONE',  ( 10.81189881249999729, 0.000000000000000000, -55.34375000204835970 ) ) ;
#15632=EDGE_CURVE ( 'NONE', #21702, #36795, #7765, .T. ) ;
#15633=CARTESIAN_POINT ( 'NONE',  ( 10.81189881249999551, -6.242252689847874514, -187.4687500020484094 ) ) ;
#15634=CARTESIAN_POINT ( 'NONE',  ( 7.644554776091147741E-16, 12.48450537969573659, -174.9687500020484094 ) ) ;
#15637=LINE ( 'NONE', #9394, #38449 ) ;
#15638=DIRECTION ( 'NONE',  ( -0.000000000000000000, -0.000000000000000000, 1.000000000000000000 ) ) ;
#15641=CARTESIAN_POINT ( 'NONE',  ( -10.81189881249999729, 1.324075727343319199E-15, -102.5937500020483810 ) ) ;
#15642=CARTESIAN_POINT ( 'NONE',  ( -9.999999999999998224, 1.224646799147353059E-15, -48.12500000409677625 ) ) ;
#15643=CARTESIAN_POINT ( 'NONE',  ( 5.405949406249992428, -9.363379034771808662, -78.28125000204838102 ) ) ;
#15644=CARTESIAN_POINT ( 'NONE',  ( -10.81189881249999729, 6.242252689847871849, -95.21875000204838102 ) ) ;
#15647=CARTESIAN_POINT ( 'NONE',  ( 10.00000000000000000, 5.773502691896255534, -143.2500000040967905 ) ) ;
#15649=ORIENTED_EDGE ( 'NONE', *, *, #31800, .F. ) ;
#15652=CARTESIAN_POINT ( 'NONE',  ( -5.405949406249996869, 9.363379034771805109, -197.5312500020484094 ) ) ;
#15653=CARTESIAN_POINT ( 'NONE',  ( -9.999999999999998224, 1.224646799147353059E-15, -200.0000000000000000 ) ) ;
#15655=ORIENTED_EDGE ( 'NONE', *, *, #18991, .F. ) ;
#15656=CARTESIAN_POINT ( 'NONE',  ( -9.999999999999998224, 5.773502691896259087, -67.37500000000001421 ) ) ;
#15658=CARTESIAN_POINT ( 'NONE',  ( -9.999999999999998224, 1.224646799147353059E-15, -76.62500000409677625 ) ) ;
#15659=CARTESIAN_POINT ( 'NONE',  ( -10.00000000000025580, 5.773502691896109873, -101.8750000000000000 ) ) ;
#15660=CARTESIAN_POINT ( 'NONE',  ( 10.00000000000012257, -5.773502691896187144, -160.0000000040968189 ) ) ;
#15662=CARTESIAN_POINT ( 'NONE',  ( 10.81189881249999551, -6.242252689847874514, -70.65625000204839523 ) ) ;
#15663=( BOUNDED_CURVE ( )  B_SPLINE_CURVE ( 2, ( #34929, #41372, #1697, #28021, #41151, #24796, #18290 ),
 .UNSPECIFIED., .F., .F. ) 
 B_SPLINE_CURVE_WITH_KNOTS ( ( 3, 2, 2, 3 ),
 ( 0.8097014925373136052, 0.8109452736318409904, 0.8121890547263682647, 0.8134328358208956500 ),
 .UNSPECIFIED. ) 
 CURVE ( )  GEOMETRIC_REPRESENTATION_ITEM ( )  RATIONAL_B_SPLINE_CURVE ( ( 0.9999999999999761302, 0.8660254037844625774, 1.000000000000000000, 0.8660254037844387076, 1.000000000000000000, 0.8660254037844267172, 1.000000000000011990 ) ) 
 REPRESENTATION_ITEM ( '' )  );
#15665=CARTESIAN_POINT ( 'NONE',  ( 9.999999999999998224, 0.000000000000000000, -93.87500000409677625 ) ) ;
#15667=CARTESIAN_POINT ( 'NONE',  ( 5.000000000000000000, 8.660254037844385522, -47.12500000409677625 ) ) ;
#15668=CARTESIAN_POINT ( 'NONE',  ( -5.405949406250003975, -9.363379034771801557, -197.0312500020484094 ) ) ;
#15670=CARTESIAN_POINT ( 'NONE',  ( -5.405949406250003975, -9.363379034771801557, -6.343750002048370362 ) ) ;
#15673=CARTESIAN_POINT ( 'NONE',  ( -9.999999999999998224, 1.224646799147353059E-15, -112.6250000040967763 ) ) ;
#15675=CARTESIAN_POINT ( 'NONE',  ( -2.121150477449813534E-15, -11.54700538379251284, -171.8750000000000284 ) ) ;
#15676=CARTESIAN_POINT ( 'NONE',  ( -2.121150477449813534E-15, -11.54700538379251284, -36.87499999999996447 ) ) ;
#15677=CARTESIAN_POINT ( 'NONE',  ( 10.81189881249999907, 6.242252689847868297, -101.9062500020484094 ) ) ;
#15678=VERTEX_POINT ( 'NONE', #40879 ) ;
#15682=CARTESIAN_POINT ( 'NONE',  ( 5.405949406249999534, 9.363379034771803333, -26.78125000204836681 ) ) ;
#15684=CARTESIAN_POINT ( 'NONE',  ( -2.293366432827344421E-15, -12.48450537969573659, -79.71875000204838102 ) ) ;
#15685=CARTESIAN_POINT ( 'NONE',  ( 0.000000000000000000, 0.000000000000000000, -200.0000000000000000 ) ) ;
#15688=AXIS2_PLACEMENT_3D ( 'NONE', #12036, #19364, #25231 ) ;
#15689=CARTESIAN_POINT ( 'NONE',  ( -9.999999999999998224, 1.224646799147353059E-15, -19.62500000409675494 ) ) ;
#15690=ADVANCED_FACE ( 'NONE', ( #24734 ), #15406, .T. ) ;
#15691=CARTESIAN_POINT ( 'NONE',  ( -9.999999999999998224, 1.224646799147353059E-15, -200.0000000000000000 ) ) ;
#15692=CARTESIAN_POINT ( 'NONE',  ( 5.000000000000000000, 8.660254037844385522, -49.74999999999998579 ) ) ;
#15694=CARTESIAN_POINT ( 'NONE',  ( 9.999999999999996447, -5.773502691896262640, -14.50000000409676382 ) ) ;
#15696=CARTESIAN_POINT ( 'NONE',  ( -5.405949406250003975, -9.363379034771801557, -132.3437500020484094 ) ) ;
#15697=CARTESIAN_POINT ( 'NONE',  ( -10.81189881249999729, 6.242252689847871849, -114.7187500020483810 ) ) ;
#15700=CARTESIAN_POINT ( 'NONE',  ( -5.000000000000003553, -8.660254037844383745, -173.8750000040968189 ) ) ;
#15701=CARTESIAN_POINT ( 'NONE',  ( 9.999999999999998224, 0.000000000000000000, -140.3750000040967905 ) ) ;
#15704=CARTESIAN_POINT ( 'NONE',  ( -10.81189881249999729, 6.242252689847871849, -45.71875000204837391 ) ) ;
#15706=CARTESIAN_POINT ( 'NONE',  ( 5.405949406249992428, -9.363379034771808662, -1.781250002048373471 ) ) ;
#15708=FACE_OUTER_BOUND ( 'NONE', #3710, .T. ) ;
#15710=CARTESIAN_POINT ( 'NONE',  ( -5.000000000000003553, -8.660254037844383745, -92.49999999999998579 ) ) ;
#15712=CARTESIAN_POINT ( 'NONE',  ( 10.00000000000000000, 5.773502691896255534, -96.75000000409679046 ) ) ;
#15713=DIRECTION ( 'NONE',  ( -0.000000000000000000, -0.000000000000000000, 1.000000000000000000 ) ) ;
#15715=CARTESIAN_POINT ( 'NONE',  ( 5.405949406249992428, -9.363379034771808662, -93.28125000204838102 ) ) ;
#15716=VERTEX_POINT ( 'NONE', #25575 ) ;
#15719=CARTESIAN_POINT ( 'NONE',  ( 5.405949406249992428, -9.363379034771808662, -156.2812500020484094 ) ) ;
#15721=ORIENTED_EDGE ( 'NONE', *, *, #9304, .T. ) ;
#15722=CARTESIAN_POINT ( 'NONE',  ( -4.999999999999996447, 8.660254037844387298, -17.99999999999996092 ) ) ;
#15723=CARTESIAN_POINT ( 'NONE',  ( 10.81189881249999729, 0.000000000000000000, -22.53125000204836326 ) ) ;
#15724=CARTESIAN_POINT ( 'NONE',  ( -4.999999999999996447, 8.660254037844387298, -151.5000000000000000 ) ) ;
#15727=CARTESIAN_POINT ( 'NONE',  ( -5.405949406250003975, -9.363379034771801557, -128.0312500020484094 ) ) ;
#15729=CARTESIAN_POINT ( 'NONE',  ( 0.000000000000000000, 0.000000000000000000, 49.99999999999998579 ) ) ;
#15730=ORIENTED_EDGE ( 'NONE', *, *, #14906, .F. ) ;
#15731=CARTESIAN_POINT ( 'NONE',  ( -10.81189881249999729, 6.242252689847871849, -53.40625000204837391 ) ) ;
#15734=CARTESIAN_POINT ( 'NONE',  ( 10.81189881249999907, 6.242252689847868297, -104.7187500020483810 ) ) ;
#15735=ORIENTED_EDGE ( 'NONE', *, *, #27427, .T. ) ;
#15736=ORIENTED_EDGE ( 'NONE', *, *, #39587, .T. ) ;
#15738=CARTESIAN_POINT ( 'NONE',  ( -9.999999999999998224, 1.224646799147353059E-15, -184.2500000000000000 ) ) ;
#15739=CARTESIAN_POINT ( 'NONE',  ( -10.81189881249999907, -6.242252689847864744, -151.9687500020484094 ) ) ;
#15741=CARTESIAN_POINT ( 'NONE',  ( 10.81189881249999729, 0.000000000000000000, -4.343750002048368586 ) ) ;
#15742=CARTESIAN_POINT ( 'NONE',  ( -10.00000000000076916, 5.773502691895813221, -139.3750000000000000 ) ) ;
#15743=CARTESIAN_POINT ( 'NONE',  ( -10.81189881249999729, 6.242252689847871849, -141.7187500020483810 ) ) ;
#15746=CARTESIAN_POINT ( 'NONE',  ( 0.000000000000000000, 0.000000000000000000, -200.0000000000000000 ) ) ;
#15748=CARTESIAN_POINT ( 'NONE',  ( -9.999999999999998224, 1.224646799147353059E-15, -192.1250000040967905 ) ) ;
#15750=ADVANCED_FACE ( 'NONE', ( #31415 ), #41733, .T. ) ;
#15751=CARTESIAN_POINT ( 'NONE',  ( 10.81189881249999551, -6.242252689847874514, -193.6562500020484094 ) ) ;
#15752=CARTESIAN_POINT ( 'NONE',  ( 7.070501591499376803E-16, 11.54700538379251284, -149.0000000040967905 ) ) ;
#15755=CARTESIAN_POINT ( 'NONE',  ( -10.81189881249999729, 6.242252689847871849, -65.21875000204838102 ) ) ;
#15756=CARTESIAN_POINT ( 'NONE',  ( -10.81189881249999729, 1.324075727343319199E-15, -45.59375000204838102 ) ) ;
#15758=CARTESIAN_POINT ( 'NONE',  ( -10.81189881249999729, 1.324075727343319199E-15, -23.28125000204836326 ) ) ;
#15760=CARTESIAN_POINT ( 'NONE',  ( 10.00000000000205347, -5.773502691895071592, -8.124999999999923617 ) ) ;
#15762=CARTESIAN_POINT ( 'NONE',  ( 5.000000000000000000, 8.660254037844385522, -115.7499999999999858 ) ) ;
#15763=DIRECTION ( 'NONE',  ( -0.000000000000000000, -0.000000000000000000, 1.000000000000000000 ) ) ;
#15766=CARTESIAN_POINT ( 'NONE',  ( -2.293366432827344421E-15, -12.48450537969573659, -115.9062500020483952 ) ) ;
#15767=ORIENTED_EDGE ( 'NONE', *, *, #15983, .T. ) ;
#15768=CARTESIAN_POINT ( 'NONE',  ( 5.000000000000000000, 8.660254037844385522, -121.7500000000000000 ) ) ;
#15772=CARTESIAN_POINT ( 'NONE',  ( -4.999999999999996447, 8.660254037844387298, -40.49999999999997868 ) ) ;
#15773=CARTESIAN_POINT ( 'NONE',  ( -2.121150477449813534E-15, -11.54700538379251284, -28.25000000409675138 ) ) ;
#15774=CARTESIAN_POINT ( 'NONE',  ( 5.405949406249992428, -9.363379034771808662, -54.28125000204836681 ) ) ;
#15778=CARTESIAN_POINT ( 'NONE',  ( -5.405949406249996869, 9.363379034771805109, -143.5312500020483810 ) ) ;
#15779=CARTESIAN_POINT ( 'NONE',  ( -10.81189881249999729, 6.242252689847871849, -149.4062500020484094 ) ) ;
#15781=EDGE_LOOP ( 'NONE', ( #7135, #20598, #29289, #7101 ) ) ;
#15782=EDGE_CURVE ( 'NONE', #23886, #36957, #25424, .T. ) ;
#15787=( BOUNDED_CURVE ( )  B_SPLINE_CURVE ( 2, ( #34829, #22297, #21431, #31594, #18620, #41491, #32020 ),
 .UNSPECIFIED., .F., .F. ) 
 B_SPLINE_CURVE_WITH_KNOTS ( ( 3, 2, 2, 3 ),
 ( 0.7873134328358211143, 0.7885572139303484995, 0.7898009950248758848, 0.7910447761194031591 ),
 .UNSPECIFIED. ) 
 CURVE ( )  GEOMETRIC_REPRESENTATION_ITEM ( )  RATIONAL_B_SPLINE_CURVE ( ( 0.9999999999999761302, 0.8660254037844625774, 1.000000000000000000, 0.8660254037844387076, 1.000000000000000000, 0.8660254037844148378, 1.000000000000023981 ) ) 
 REPRESENTATION_ITEM ( '' )  );
#15788=CARTESIAN_POINT ( 'NONE',  ( 7.644554776091147741E-16, 12.48450537969573659, -185.4687500020483810 ) ) ;
#15790=CARTESIAN_POINT ( 'NONE',  ( -5.405949406249996869, 9.363379034771805109, -27.84375000204836326 ) ) ;
#15792=CARTESIAN_POINT ( 'NONE',  ( 7.644554776091147741E-16, 12.48450537969573659, -162.9687500020483810 ) ) ;
#15793=CARTESIAN_POINT ( 'NONE',  ( -10.81189881249999729, 1.324075727343319199E-15, -141.5937500020483810 ) ) ;
#15794=DIRECTION ( 'NONE',  ( 1.000000000000000000, 0.000000000000000000, 0.000000000000000000 ) ) ;
#15797=CARTESIAN_POINT ( 'NONE',  ( 10.81189881249999907, 6.242252689847868297, -19.21875000204837747 ) ) ;
#15799=DIRECTION ( 'NONE',  ( 1.000000000000000000, 0.000000000000000000, 0.000000000000000000 ) ) ;
#15800=CARTESIAN_POINT ( 'NONE',  ( -10.00000000000102496, 5.773502691895664007, -33.25000000409673362 ) ) ;
#15802=CARTESIAN_POINT ( 'NONE',  ( -5.405949406250003975, -9.363379034771801557, -79.84375000204838102 ) ) ;
#15803=CARTESIAN_POINT ( 'NONE',  ( -10.81189881249999907, -6.242252689847864744, -51.65625000204838102 ) ) ;
#15805=CARTESIAN_POINT ( 'NONE',  ( 5.000000000000000000, 8.660254037844385522, -57.24999999999996447 ) ) ;
#15806=ADVANCED_FACE ( 'NONE', ( #14979 ), #8954, .T. ) ;
#15808=CARTESIAN_POINT ( 'NONE',  ( -5.000000000000003553, -8.660254037844383745, -134.5000000000000000 ) ) ;
#15809=CARTESIAN_POINT ( 'NONE',  ( -2.293366432827344421E-15, -12.48450537969573659, -145.9062500020484094 ) ) ;
#15810=DIRECTION ( 'NONE',  ( 1.000000000000000000, 0.000000000000000000, 0.000000000000000000 ) ) ;
#15811=CARTESIAN_POINT ( 'NONE',  ( 10.00000000000000000, 5.773502691896255534, -119.2500000040967905 ) ) ;
#15813=ORIENTED_EDGE ( 'NONE', *, *, #39940, .T. ) ;
#15816=CARTESIAN_POINT ( 'NONE',  ( -9.999999999999998224, 1.224646799147353059E-15, -193.6250000040967905 ) ) ;
#15817=VECTOR ( 'NONE', #8701, 1000.000000000000000 ) ;
#15818=CARTESIAN_POINT ( 'NONE',  ( -2.293366432827344421E-15, -12.48450537969573659, -171.4062500020484379 ) ) ;
#15819=CARTESIAN_POINT ( 'NONE',  ( -4.999999999999996447, 8.660254037844387298, -49.87500000409675494 ) ) ;
#15822=CARTESIAN_POINT ( 'NONE',  ( -10.00000000000154188, 5.773502691895366468, -83.87499999999992895 ) ) ;
#15823=CARTESIAN_POINT ( 'NONE',  ( -5.405949406249996869, 9.363379034771805109, -172.0312500020484094 ) ) ;
#15824=CARTESIAN_POINT ( 'NONE',  ( 9.999999999999998224, 0.000000000000000000, -134.3750000040967905 ) ) ;
#15825=CYLINDRICAL_SURFACE ( 'NONE', #4806, 9.999999999999998224 ) ;
#15826=ORIENTED_EDGE ( 'NONE', *, *, #42633, .F. ) ;
#15828=CARTESIAN_POINT ( 'NONE',  ( 9.999999999999998224, 0.000000000000000000, -70.99999999999998579 ) ) ;
#15829=CARTESIAN_POINT ( 'NONE',  ( -10.81189881249999729, 6.242252689847871849, -77.40625000204838102 ) ) ;
#15830=VERTEX_POINT ( 'NONE', #15824 ) ;
#15833=CARTESIAN_POINT ( 'NONE',  ( 10.81189881249999551, -6.242252689847874514, -28.46875000204837036 ) ) ;
#15835=CARTESIAN_POINT ( 'NONE',  ( -10.81189881249999729, 6.242252689847871849, -9.906250002048379244 ) ) ;
#15837=CARTESIAN_POINT ( 'NONE',  ( -2.293366432827344421E-15, -12.48450537969573659, -58.71875000204836681 ) ) ;
#15841=CARTESIAN_POINT ( 'NONE',  ( -5.405949406249996869, 9.363379034771805109, -186.8437500020483810 ) ) ;
#15842=CARTESIAN_POINT ( 'NONE',  ( 5.405949406249992428, -9.363379034771808662, -178.5937500020484094 ) ) ;
#15845=CARTESIAN_POINT ( 'NONE',  ( 9.999999999999742428, 5.773502691896404748, -124.8749999999999858 ) ) ;
#15848=CARTESIAN_POINT ( 'NONE',  ( 10.81189881249999729, 0.000000000000000000, -107.8437500020483810 ) ) ;
#15850=CARTESIAN_POINT ( 'NONE',  ( 5.405949406249992428, -9.363379034771808662, -75.28125000204838102 ) ) ;
#15851=CARTESIAN_POINT ( 'NONE',  ( 4.999999999999992006, -8.660254037844389075, -159.7500000000000000 ) ) ;
#15852=EDGE_CURVE ( 'NONE', #14676, #19099, #28176, .T. ) ;
#15853=CARTESIAN_POINT ( 'NONE',  ( -5.405949406249996869, 9.363379034771805109, -84.84375000204836681 ) ) ;
#15856=CARTESIAN_POINT ( 'NONE',  ( 9.999999999999998224, 0.000000000000000000, -144.8750000040967905 ) ) ;
#15861=CARTESIAN_POINT ( 'NONE',  ( -5.405949406249996869, 9.363379034771805109, -193.0312500020484094 ) ) ;
#15863=ORIENTED_EDGE ( 'NONE', *, *, #19093, .T. ) ;
#15864=CARTESIAN_POINT ( 'NONE',  ( -9.999999999999998224, 5.773502691896259087, -64.37499999999998579 ) ) ;
#15866=CARTESIAN_POINT ( 'NONE',  ( 7.070501591499377789E-16, 11.54700538379251284, -72.50000000409676204 ) ) ;
#15869=CARTESIAN_POINT ( 'NONE',  ( -10.81189881249999729, 6.242252689847871849, -63.90625000204837391 ) ) ;
#15872=VERTEX_POINT ( 'NONE', #5080 ) ;
#15873=CARTESIAN_POINT ( 'NONE',  ( 7.644554776091147741E-16, 12.48450537969573659, -194.6562500020484094 ) ) ;
#15874=( GEOMETRIC_REPRESENTATION_CONTEXT ( 3 ) GLOBAL_UNCERTAINTY_ASSIGNED_CONTEXT ( ( #23403 ) ) GLOBAL_UNIT_ASSIGNED_CONTEXT ( ( #11537, #34664, #18234 ) ) REPRESENTATION_CONTEXT ( 'NONE', 'WORKASPACE' ) );
#15876=CARTESIAN_POINT ( 'NONE',  ( 10.81189881249999729, 6.242252689847867408, -7.218750002048349934 ) ) ;
#15878=CARTESIAN_POINT ( 'NONE',  ( 9.999999999999998224, 0.000000000000000000, -45.49999999999998579 ) ) ;
#15879=DIRECTION ( 'NONE',  ( -0.000000000000000000, -0.000000000000000000, 1.000000000000000000 ) ) ;
#15880=CARTESIAN_POINT ( 'NONE',  ( 9.999999999999996447, -5.773502691896262640, -177.6250000000000000 ) ) ;
#15881=CARTESIAN_POINT ( 'NONE',  ( -9.999999999999998224, 1.224646799147353059E-15, -166.2500000000000000 ) ) ;
#15882=CARTESIAN_POINT ( 'NONE',  ( 5.405949406249992428, -9.363379034771808662, -100.7812500020483952 ) ) ;
#15884=CARTESIAN_POINT ( 'NONE',  ( -4.999999999999996447, 8.660254037844387298, -37.49999999999997868 ) ) ;
#15885=EDGE_CURVE ( 'NONE', #18018, #42167, #35878, .T. ) ;
#15886=ORIENTED_EDGE ( 'NONE', *, *, #23177, .F. ) ;
#15887=ORIENTED_EDGE ( 'NONE', *, *, #7580, .T. ) ;
#15888=CARTESIAN_POINT ( 'NONE',  ( 10.81189881249999907, 6.242252689847868297, -31.40625000204834905 ) ) ;
#15890=CARTESIAN_POINT ( 'NONE',  ( 5.405949406249992428, -9.363379034771808662, -76.59375000204838102 ) ) ;
#15891=CARTESIAN_POINT ( 'NONE',  ( 9.999999999999998224, 0.000000000000000000, -180.5000000000000000 ) ) ;
#15893=CARTESIAN_POINT ( 'NONE',  ( 10.00000000000025402, -5.773502691896113426, -130.0000000040967905 ) ) ;
#15894=LINE ( 'NONE', #11447, #30876 ) ;
#15896=CARTESIAN_POINT ( 'NONE',  ( -9.999999999999998224, 5.773502691896259087, -15.25000000409676737 ) ) ;
#15899=CARTESIAN_POINT ( 'NONE',  ( -10.81189881249999729, 6.242252689847871849, -126.7187500020483952 ) ) ;
#15900=CARTESIAN_POINT ( 'NONE',  ( 10.81189881249999729, 0.000000000000000000, -100.5312500020483952 ) ) ;
#15901=EDGE_CURVE ( 'NONE', #6715, #13020, #42160, .T. ) ;
#15902=CARTESIAN_POINT ( 'NONE',  ( 10.81189881249999551, -6.242252689847874514, -104.9687500020483810 ) ) ;
#15905=CARTESIAN_POINT ( 'NONE',  ( -2.121150477449813534E-15, -11.54700538379251284, -166.2500000040968189 ) ) ;
#15906=( BOUNDED_CURVE ( )  B_SPLINE_CURVE ( 2, ( #18264, #8780, #27781, #21937, #40916, #14801, #35117 ),
 .UNSPECIFIED., .F., .F. ) 
 B_SPLINE_CURVE_WITH_KNOTS ( ( 3, 2, 2, 3 ),
 ( 0.5000000000000001110, 0.5012437810945274963, 0.5024875621890548816, 0.5037313432835821558 ),
 .UNSPECIFIED. ) 
 CURVE ( )  GEOMETRIC_REPRESENTATION_ITEM ( )  RATIONAL_B_SPLINE_CURVE ( ( 0.9999999999999880096, 0.8660254037844506980, 1.000000000000000000, 0.8660254037844387076, 1.000000000000000000, 0.8660254037844267172, 1.000000000000011990 ) ) 
 REPRESENTATION_ITEM ( '' )  );
#15907=EDGE_CURVE ( 'NONE', #26894, #9613, #15432, .T. ) ;
#15908=CARTESIAN_POINT ( 'NONE',  ( 0.000000000000000000, 0.000000000000000000, -200.0000000000000000 ) ) ;
#15911=EDGE_CURVE ( 'NONE', #19609, #37214, #36335, .T. ) ;
#15913=CARTESIAN_POINT ( 'NONE',  ( -5.405949406249996869, 9.363379034771805109, 0.4687499979516285276 ) ) ;
#15917=CARTESIAN_POINT ( 'NONE',  ( -4.999999999999996447, 8.660254037844387298, -92.99999999999998579 ) ) ;
#15919=CARTESIAN_POINT ( 'NONE',  ( 7.070501591499377789E-16, 11.54700538379251284, -96.50000000409679046 ) ) ;
#15923=CARTESIAN_POINT ( 'NONE',  ( 10.81189881249999551, -6.242252689847874514, -93.15625000204838102 ) ) ;
#15929=CARTESIAN_POINT ( 'NONE',  ( 10.00000000000000000, 5.773502691896255534, -19.87499999999996803 ) ) ;
#15930=CARTESIAN_POINT ( 'NONE',  ( 9.999999999999996447, -5.773502691896262640, -155.1250000000000000 ) ) ;
#15931=EDGE_CURVE ( 'NONE', #32336, #5197, #16884, .T. ) ;
#15933=EDGE_CURVE ( 'NONE', #22272, #23552, #16647, .T. ) ;
#15934=AXIS2_PLACEMENT_3D ( 'NONE', #38085, #40872, #5499 ) ;
#15936=CARTESIAN_POINT ( 'NONE',  ( -9.999999999999998224, 1.224646799147353059E-15, -194.7500000000000000 ) ) ;
#15937=CARTESIAN_POINT ( 'NONE',  ( -5.405949406249996869, 9.363379034771805109, -122.5312500020483952 ) ) ;
#15938=ORIENTED_EDGE ( 'NONE', *, *, #4445, .F. ) ;
#15939=CARTESIAN_POINT ( 'NONE',  ( -4.999999999999996447, 8.660254037844387298, -64.87500000409676204 ) ) ;
#15940=ORIENTED_EDGE ( 'NONE', *, *, #39110, .F. ) ;
#15941=CARTESIAN_POINT ( 'NONE',  ( -2.293366432827344421E-15, -12.48450537969573659, -52.90625000204837391 ) ) ;
#15943=VECTOR ( 'NONE', #37227, 1000.000000000000000 ) ;
#15944=CARTESIAN_POINT ( 'NONE',  ( -10.81189881249999907, -6.242252689847864744, -102.4687500020483810 ) ) ;
#15947=CARTESIAN_POINT ( 'NONE',  ( 10.00000000000051159, -5.773502691895965988, -175.0000000040968189 ) ) ;
#15948=CARTESIAN_POINT ( 'NONE',  ( -4.999999999999996447, 8.660254037844387298, -32.99999999999997158 ) ) ;
#15950=CARTESIAN_POINT ( 'NONE',  ( -10.81189881249999729, 6.242252689847871849, -2.218750002048357928 ) ) ;
#15952=CARTESIAN_POINT ( 'NONE',  ( 7.644554776091147741E-16, 12.48450537969573659, -141.9687500020483810 ) ) ;
#15953=B_SPLINE_CURVE_WITH_KNOTS ( 'NONE', 3,
 ( #23023, #16515, #32534, #42637, #22810, #26051 ),
 .UNSPECIFIED., .F., .F.,
 ( 4, 2, 4 ),
 ( 0.9171367075385271628, 0.9585683537692635259, 1.000000000000000000 ),
 .UNSPECIFIED. ) ;
#15955=CARTESIAN_POINT ( 'NONE',  ( 9.999999999999998224, 0.000000000000000000, -147.5000000000000000 ) ) ;
#15957=CARTESIAN_POINT ( 'NONE',  ( 9.999999999999996447, -5.773502691896262640, -194.5000000040968189 ) ) ;
#15959=VECTOR ( 'NONE', #38648, 1000.000000000000114 ) ;
#15960=CARTESIAN_POINT ( 'NONE',  ( -5.405949406250003975, -9.363379034771801557, -188.0312500020484094 ) ) ;
#15961=CARTESIAN_POINT ( 'NONE',  ( -2.121150477449813534E-15, -11.54700538379251284, -95.37500000000000000 ) ) ;
#15964=CARTESIAN_POINT ( 'NONE',  ( -10.81189881249999729, 6.242252689847871849, -66.71875000204838102 ) ) ;
#15965=CARTESIAN_POINT ( 'NONE',  ( -5.405949406249996869, 9.363379034771805109, -48.84375000204838102 ) ) ;
#15967=CARTESIAN_POINT ( 'NONE',  ( 5.405949406249992428, -9.363379034771808662, -27.28125000204836681 ) ) ;
#15971=CARTESIAN_POINT ( 'NONE',  ( -5.000000000000003553, -8.660254037844383745, -114.9999999999999858 ) ) ;
#15972=CYLINDRICAL_SURFACE ( 'NONE', #20342, 9.999999999999998224 ) ;
#15975=CARTESIAN_POINT ( 'NONE',  ( -10.81189881249999729, -6.242252689847864744, -117.6562500020483952 ) ) ;
#15976=ORIENTED_EDGE ( 'NONE', *, *, #28450, .T. ) ;
#15977=CARTESIAN_POINT ( 'NONE',  ( 9.999999999999998224, 0.000000000000000000, -197.3750000040967905 ) ) ;
#15979=CARTESIAN_POINT ( 'NONE',  ( 4.999999999999992006, -8.660254037844389075, -128.2499999999999716 ) ) ;
#15981=CARTESIAN_POINT ( 'NONE',  ( -9.999999999999998224, 5.773502691896259087, -44.87499999999997868 ) ) ;
#15982=AXIS2_PLACEMENT_3D ( 'NONE', #22969, #96, #15091 ) ;
#15983=EDGE_CURVE ( 'NONE', #437, #22331, #35712, .T. ) ;
#15984=CARTESIAN_POINT ( 'NONE',  ( -4.999999999999996447, 8.660254037844387298, -25.87500000409675849 ) ) ;
#15985=CARTESIAN_POINT ( 'NONE',  ( 7.644554776091147741E-16, 12.48450537969573659, -40.15625000204835260 ) ) ;
#15989=CARTESIAN_POINT ( 'NONE',  ( 5.405949406249999534, 9.363379034771803333, -133.2812500020483810 ) ) ;
#15990=CARTESIAN_POINT ( 'NONE',  ( 5.405949406249992428, -9.363379034771808662, -148.7812500020483810 ) ) ;
#15991=CARTESIAN_POINT ( 'NONE',  ( -2.121150477449813534E-15, -11.54700538379251284, -65.37499999999998579 ) ) ;
#15992=CARTESIAN_POINT ( 'NONE',  ( -5.000000000000003553, -8.660254037844383745, -124.0000000000000000 ) ) ;
#15995=VERTEX_POINT ( 'NONE', #36125 ) ;
#15996=( BOUNDED_CURVE ( )  B_SPLINE_CURVE ( 2, ( #34083, #36880, #31283, #30633, #27171, #37739, #40523 ),
 .UNSPECIFIED., .F., .F. ) 
 B_SPLINE_CURVE_WITH_KNOTS ( ( 3, 2, 2, 3 ),
 ( 0.3022388059701494045, 0.3034825870646767343, 0.3047263681592040085, 0.3059701492537313383 ),
 .UNSPECIFIED. ) 
 CURVE ( )  GEOMETRIC_REPRESENTATION_ITEM ( )  RATIONAL_B_SPLINE_CURVE ( ( 0.9999999999999820144, 0.8660254037844566932, 1.000000000000000000, 0.8660254037844387076, 1.000000000000000000, 0.8660254037844387076, 1.000000000000000000 ) ) 
 REPRESENTATION_ITEM ( '' )  );
#15998=CARTESIAN_POINT ( 'NONE',  ( 5.405949406249999534, 9.363379034771803333, -172.0937500020484094 ) ) ;
#15999=CARTESIAN_POINT ( 'NONE',  ( 7.644554776091147741E-16, 12.48450537969573659, -29.46875000204835970 ) ) ;
#16000=CARTESIAN_POINT ( 'NONE',  ( -2.121150477449813534E-15, -11.54700538379251284, -128.7500000040967905 ) ) ;
#16001=CARTESIAN_POINT ( 'NONE',  ( 5.405949406249999534, 9.363379034771803333, -161.5937500020484094 ) ) ;
#16002=CARTESIAN_POINT ( 'NONE',  ( -10.81189881249999729, 1.324075727343319199E-15, -149.0937500020483810 ) ) ;
#16006=CARTESIAN_POINT ( 'NONE',  ( 5.405949406249999534, 9.363379034771803333, -17.59375000204835260 ) ) ;
#16008=CARTESIAN_POINT ( 'NONE',  ( 0.000000000000000000, 0.000000000000000000, -200.0000000000000000 ) ) ;
#16009=CARTESIAN_POINT ( 'NONE',  ( 9.999999999999479527, 5.773502691896553074, -44.25000000409674783 ) ) ;
#16012=CARTESIAN_POINT ( 'NONE',  ( 10.81189881249999551, -6.242252689847874514, -71.96875000204838102 ) ) ;
#16013=CARTESIAN_POINT ( 'NONE',  ( 7.644554776091147741E-16, 12.48450537969573659, -49.15625000204837391 ) ) ;
#16017=CARTESIAN_POINT ( 'NONE',  ( -5.000000000000003553, -8.660254037844383745, -140.5000000000000000 ) ) ;
#16018=CARTESIAN_POINT ( 'NONE',  ( -2.293366432827344421E-15, -12.48450537969573659, -150.4062500020484379 ) ) ;
#16020=CARTESIAN_POINT ( 'NONE',  ( -2.121150477449813534E-15, -11.54700538379251284, -115.2500000040967763 ) ) ;
#16022=ORIENTED_EDGE ( 'NONE', *, *, #15002, .F. ) ;
#16025=FACE_OUTER_BOUND ( 'NONE', #21810, .T. ) ;
#16026=CARTESIAN_POINT ( 'NONE',  ( 7.644554776091147741E-16, 12.48450537969573659, -172.1562500020484094 ) ) ;
#16027=CARTESIAN_POINT ( 'NONE',  ( -9.999999999999998224, 5.773502691896259087, -51.25000000409676915 ) ) ;
#16029=DIRECTION ( 'NONE',  ( 0.4999999999999997224, 0.8660254037844388186, 0.000000000000000000 ) ) ;
#16031=CARTESIAN_POINT ( 'NONE',  ( 9.999999999999998224, 0.000000000000000000, -156.5000000000000000 ) ) ;
#16032=CARTESIAN_POINT ( 'NONE',  ( -10.81189881249999729, 6.242252689847871849, -164.4062500020484094 ) ) ;
#16033=CARTESIAN_POINT ( 'NONE',  ( 10.81189881249999907, 6.242252689847868297, -140.7187500020483810 ) ) ;
#16034=CARTESIAN_POINT ( 'NONE',  ( 0.000000000000000000, 0.000000000000000000, -200.0000000000000000 ) ) ;
#16035=CARTESIAN_POINT ( 'NONE',  ( 9.999999999999998224, 0.000000000000000000, -55.99999999999996447 ) ) ;
#16036=VERTEX_POINT ( 'NONE', #3535 ) ;
#16037=FACE_OUTER_BOUND ( 'NONE', #6657, .T. ) ;
#16038=EDGE_CURVE ( 'NONE', #6564, #5725, #38643, .T. ) ;
#16040=CARTESIAN_POINT ( 'NONE',  ( 10.81189881249999729, 0.000000000000000000, -66.03125000204838102 ) ) ;
#16043=CARTESIAN_POINT ( 'NONE',  ( -10.81189881249999729, 6.242252689847871849, -119.2187500020483810 ) ) ;
#16044=ORIENTED_EDGE ( 'NONE', *, *, #17790, .T. ) ;
#16045=VERTEX_POINT ( 'NONE', #13428 ) ;
#16046=CARTESIAN_POINT ( 'NONE',  ( -10.81189881249999729, -6.242252689847864744, -27.46875000204838102 ) ) ;
#16048=CARTESIAN_POINT ( 'NONE',  ( -10.81189881249999907, -6.242252689847864744, -196.9687500020484379 ) ) ;
#16049=( BOUNDED_CURVE ( )  B_SPLINE_CURVE ( 2, ( #41138, #8156, #20874, #21304, #34060, #37929, #17624 ),
 .UNSPECIFIED., .F., .F. ) 
 B_SPLINE_CURVE_WITH_KNOTS ( ( 3, 2, 2, 3 ),
 ( 0.6977611940298510396, 0.6990049751243784248, 0.7002487562189056991, 0.7014925373134330844 ),
 .UNSPECIFIED. ) 
 CURVE ( )  GEOMETRIC_REPRESENTATION_ITEM ( )  RATIONAL_B_SPLINE_CURVE ( ( 0.9999999999999641398, 0.8660254037844745678, 1.000000000000000000, 0.8660254037844387076, 1.000000000000000000, 0.8660254037844148378, 1.000000000000023981 ) ) 
 REPRESENTATION_ITEM ( '' )  );
#16050=CARTESIAN_POINT ( 'NONE',  ( 5.405949406249999534, 9.363379034771803333, -58.09375000204835970 ) ) ;
#16053=CARTESIAN_POINT ( 'NONE',  ( -10.81189881249999729, 6.242252689847871849, -188.2187500020484379 ) ) ;
#16054=CARTESIAN_POINT ( 'NONE',  ( -10.81189881249999729, 1.324075727343319199E-15, -173.0937500020484094 ) ) ;
#16057=CARTESIAN_POINT ( 'NONE',  ( -2.121150477449813534E-15, -11.54700538379251284, -75.87500000000000000 ) ) ;
#16058=CARTESIAN_POINT ( 'NONE',  ( 9.999999999999998224, 0.000000000000000000, -176.3750000040967905 ) ) ;
#16060=CARTESIAN_POINT ( 'NONE',  ( -5.405949406250003975, -9.363379034771801557, -94.84375000204838102 ) ) ;
#16061=CARTESIAN_POINT ( 'NONE',  ( 9.999999999999998224, 0.000000000000000000, -18.49999999999996092 ) ) ;
#16062=CARTESIAN_POINT ( 'NONE',  ( -5.405949406249996869, 9.363379034771805109, -73.03125000204838102 ) ) ;
#16063=CARTESIAN_POINT ( 'NONE',  ( 9.999999999999998224, 0.000000000000000000, -159.5000000000000000 ) ) ;
#16065=CARTESIAN_POINT ( 'NONE',  ( -10.81189881249999729, 1.324075727343319199E-15, -87.59375000204836681 ) ) ;
#16067=CARTESIAN_POINT ( 'NONE',  ( -4.999999999999996447, 8.660254037844387298, -142.8750000040967905 ) ) ;
#16069=ORIENTED_EDGE ( 'NONE', *, *, #6218, .T. ) ;
#16072=CARTESIAN_POINT ( 'NONE',  ( -10.81189881249999729, 6.242252689847871849, -197.4062500020484379 ) ) ;
#16073=CYLINDRICAL_SURFACE ( 'NONE', #13006, 9.999999999999998224 ) ;
#16075=ORIENTED_EDGE ( 'NONE', *, *, #26995, .F. ) ;
#16076=CARTESIAN_POINT ( 'NONE',  ( -5.000000000000003553, -8.660254037844383745, -59.49999999999997158 ) ) ;
#16078=CARTESIAN_POINT ( 'NONE',  ( 4.999999999999992006, -8.660254037844389075, -76.12500000409677625 ) ) ;
#16079=CYLINDRICAL_SURFACE ( 'NONE', #39457, 9.999999999999998224 ) ;
#16081=CARTESIAN_POINT ( 'NONE',  ( -5.405949406249996869, 9.363379034771805109, -65.53125000204838102 ) ) ;
#16084=CARTESIAN_POINT ( 'NONE',  ( -9.999999999999998224, 1.224646799147353059E-15, -156.1250000040967905 ) ) ;
#16085=CARTESIAN_POINT ( 'NONE',  ( 10.81189881249999551, -6.242252689847874514, -190.6562500020484094 ) ) ;
#16088=FACE_OUTER_BOUND ( 'NONE', #19393, .T. ) ;
#16089=CARTESIAN_POINT ( 'NONE',  ( 7.071067811865472841, -7.071067811865472841, -200.0000000000000000 ) ) ;
#16090=DIRECTION ( 'NONE',  ( -0.000000000000000000, -0.000000000000000000, 1.000000000000000000 ) ) ;
#16091=CARTESIAN_POINT ( 'NONE',  ( 4.999999999999992006, -8.660254037844389075, -173.2500000000000284 ) ) ;
#16092=CARTESIAN_POINT ( 'NONE',  ( -4.999999999999996447, 8.660254037844387298, -97.49999999999998579 ) ) ;
#16093=CARTESIAN_POINT ( 'NONE',  ( 7.644554776091147741E-16, 12.48450537969573659, -97.15625000204839523 ) ) ;
#16095=CARTESIAN_POINT ( 'NONE',  ( -2.121150477449813534E-15, -11.54700538379251284, -164.3749999999999716 ) ) ;
#16096=ADVANCED_FACE ( 'NONE', ( #26625 ), #16457, .T. ) ;
#16098=VERTEX_POINT ( 'NONE', #39773 ) ;
#16099=CARTESIAN_POINT ( 'NONE',  ( -2.293366432827344421E-15, -12.48450537969573659, -37.71875000204836681 ) ) ;
#16100=CARTESIAN_POINT ( 'NONE',  ( 5.405949406249992428, -9.363379034771808662, -31.78125000204837391 ) ) ;
#16102=CARTESIAN_POINT ( 'NONE',  ( -5.405949406249996869, 9.363379034771805109, -81.84375000204838102 ) ) ;
#16103=CARTESIAN_POINT ( 'NONE',  ( -2.293366432827344421E-15, -12.48450537969573659, -190.7187500020484094 ) ) ;
#16104=CARTESIAN_POINT ( 'NONE',  ( -9.999999999999998224, 1.224646799147353059E-15, -130.6250000040967620 ) ) ;
#16105=CARTESIAN_POINT ( 'NONE',  ( 9.999999999999998224, 0.000000000000000000, -30.87500000409676559 ) ) ;
#16107=CARTESIAN_POINT ( 'NONE',  ( -5.000000000000003553, -8.660254037844383745, -8.875000004096744277 ) ) ;
#16108=CARTESIAN_POINT ( 'NONE',  ( 10.00000000000025402, -5.773502691896113426, -125.1249999999999574 ) ) ;
#16109=CARTESIAN_POINT ( 'NONE',  ( -5.405949406249996869, 9.363379034771805109, -132.8437500020484094 ) ) ;
#16110=CARTESIAN_POINT ( 'NONE',  ( 10.81189881249999551, -6.242252689847874514, -100.6562500020483952 ) ) ;
#16111=CARTESIAN_POINT ( 'NONE',  ( 5.405949406249992428, -9.363379034771808662, -106.5937500020483810 ) ) ;
#16112=( BOUNDED_CURVE ( )  B_SPLINE_CURVE ( 2, ( #32041, #12577, #38923, #28156, #9563, #10404, #29856 ),
 .UNSPECIFIED., .F., .F. ) 
 B_SPLINE_CURVE_WITH_KNOTS ( ( 3, 2, 2, 3 ),
 ( 0.8694029850746272103, 0.8706467661691545956, 0.8718905472636818699, 0.8731343283582092551 ),
 .UNSPECIFIED. ) 
 CURVE ( )  GEOMETRIC_REPRESENTATION_ITEM ( )  RATIONAL_B_SPLINE_CURVE ( ( 0.9999999999999641398, 0.8660254037844745678, 1.000000000000000000, 0.8660254037844387076, 1.000000000000000000, 0.8660254037844028474, 1.000000000000035971 ) ) 
 REPRESENTATION_ITEM ( '' )  );
#16115=CARTESIAN_POINT ( 'NONE',  ( -4.999999999999996447, 8.660254037844387298, -171.3750000040968189 ) ) ;
#16116=DIRECTION ( 'NONE',  ( -0.000000000000000000, -0.000000000000000000, 1.000000000000000000 ) ) ;
#16122=CARTESIAN_POINT ( 'NONE',  ( 5.000000000000000000, 8.660254037844385522, -127.7499999999999716 ) ) ;
#16124=CARTESIAN_POINT ( 'NONE',  ( 4.999999999999992006, -8.660254037844389075, -78.74999999999998579 ) ) ;
#16126=CARTESIAN_POINT ( 'NONE',  ( -9.999999999999998224, 1.224646799147353059E-15, -99.12500000409677625 ) ) ;
#16127=FACE_OUTER_BOUND ( 'NONE', #34666, .T. ) ;
#16129=CARTESIAN_POINT ( 'NONE',  ( 10.81189881249999551, -6.242252689847874514, -90.15625000204836681 ) ) ;
#16135=CARTESIAN_POINT ( 'NONE',  ( 9.999999999999996447, -5.773502691896262640, -15.62499999999997691 ) ) ;
#16136=CARTESIAN_POINT ( 'NONE',  ( -2.121150477449813534E-15, -11.54700538379251284, -152.3750000000000000 ) ) ;
#16138=CARTESIAN_POINT ( 'NONE',  ( -10.00000000000000000, -5.773502691896251982, -199.1250000000000284 ) ) ;
#16139=CARTESIAN_POINT ( 'NONE',  ( -10.81189881249999729, 6.242252689847871849, -123.9062500020483952 ) ) ;
#16140=ORIENTED_EDGE ( 'NONE', *, *, #31434, .T. ) ;
#16142=EDGE_CURVE ( 'NONE', #40023, #5178, #31222, .T. ) ;
#16143=EDGE_CURVE ( 'NONE', #12803, #15095, #36543, .T. ) ;
#16144=ORIENTED_EDGE ( 'NONE', *, *, #15632, .F. ) ;
#16146=CARTESIAN_POINT ( 'NONE',  ( 7.644554776091147741E-16, 12.48450537969573659, -56.65625000204838102 ) ) ;
#16148=CARTESIAN_POINT ( 'NONE',  ( 5.405949406249999534, 9.363379034771803333, -100.0937500020483810 ) ) ;
#16149=VERTEX_POINT ( 'NONE', #38938 ) ;
#16150=ORIENTED_EDGE ( 'NONE', *, *, #28811, .T. ) ;
#16151=CYLINDRICAL_SURFACE ( 'NONE', #16962, 9.999999999999998224 ) ;
#16153=CARTESIAN_POINT ( 'NONE',  ( -9.999999999999998224, 1.224646799147353059E-15, -200.0000000000000000 ) ) ;
#16154=( BOUNDED_CURVE ( )  B_SPLINE_CURVE ( 2, ( #28200, #34890, #21708, #41334, #8128, #30794, #1228 ),
 .UNSPECIFIED., .F., .F. ) 
 B_SPLINE_CURVE_WITH_KNOTS ( ( 3, 2, 2, 3 ),
 ( 0.7761194029850747578, 0.7773631840796021431, 0.7786069651741295283, 0.7798507462686569136 ),
 .UNSPECIFIED. ) 
 CURVE ( )  GEOMETRIC_REPRESENTATION_ITEM ( )  RATIONAL_B_SPLINE_CURVE ( ( 0.9999999999999880096, 0.8660254037844506980, 1.000000000000000000, 0.8660254037844387076, 1.000000000000000000, 0.8660254037844148378, 1.000000000000023981 ) ) 
 REPRESENTATION_ITEM ( '' )  );
#16156=CARTESIAN_POINT ( 'NONE',  ( -10.81189881249999729, 1.324075727343319199E-15, -0.5937500020483654772 ) ) ;
#16158=ADVANCED_FACE ( 'NONE', ( #9369 ), #39148, .T. ) ;
#16159=CARTESIAN_POINT ( 'NONE',  ( -10.81189881249999729, -6.242252689847864744, -133.9687500020483810 ) ) ;
#16161=CARTESIAN_POINT ( 'NONE',  ( -10.00000000000051337, 5.773502691895962435, -115.7500000040967905 ) ) ;
#16163=CARTESIAN_POINT ( 'NONE',  ( -10.00000000000000000, -5.773502691896251982, -193.5000000040967905 ) ) ;
#16165=CARTESIAN_POINT ( 'NONE',  ( -2.293366432827344421E-15, -12.48450537969573659, -187.9062500020484094 ) ) ;
#16166=CARTESIAN_POINT ( 'NONE',  ( 4.999999999999992006, -8.660254037844389075, -185.6250000040967905 ) ) ;
#16170=CARTESIAN_POINT ( 'NONE',  ( -10.81189881249999729, -6.242252689847864744, -64.96875000204838102 ) ) ;
#16171=CARTESIAN_POINT ( 'NONE',  ( 5.405949406249992428, -9.363379034771808662, -49.59375000204838102 ) ) ;
#16173=CARTESIAN_POINT ( 'NONE',  ( 10.81189881249999907, 6.242252689847868297, -19.40625000204837747 ) ) ;
#16175=CARTESIAN_POINT ( 'NONE',  ( 9.999999999999998224, 0.000000000000000000, -7.999999999999952038 ) ) ;
#16177=CARTESIAN_POINT ( 'NONE',  ( 9.999999999999996447, -5.773502691896262640, -116.1250000000000000 ) ) ;
#16180=CARTESIAN_POINT ( 'NONE',  ( 7.644554776091147741E-16, 12.48450537969573659, -115.1562500020483952 ) ) ;
#16181=ORIENTED_EDGE ( 'NONE', *, *, #11440, .T. ) ;
#16182=CYLINDRICAL_SURFACE ( 'NONE', #8651, 9.999999999999998224 ) ;
#16184=CARTESIAN_POINT ( 'NONE',  ( 4.999999999999992006, -8.660254037844389075, -86.62500000409677625 ) ) ;
#16186=ORIENTED_EDGE ( 'NONE', *, *, #17764, .F. ) ;
#16187=CARTESIAN_POINT ( 'NONE',  ( 7.070501591499377789E-16, 11.54700538379251284, -45.12499999999997158 ) ) ;
#16188=CARTESIAN_POINT ( 'NONE',  ( 9.999999999999996447, -5.773502691896262640, -17.50000000409676204 ) ) ;
#16189=CARTESIAN_POINT ( 'NONE',  ( -2.293366432827344421E-15, -12.48450537969573659, -40.90625000204836681 ) ) ;
#16190=ADVANCED_FACE ( 'NONE', ( #26201 ), #9790, .T. ) ;
#16191=CARTESIAN_POINT ( 'NONE',  ( 5.000000000000000000, 8.660254037844385522, -16.74999999999996092 ) ) ;
#16194=CARTESIAN_POINT ( 'NONE',  ( -9.999999999999998224, 1.224646799147353059E-15, -200.0000000000000000 ) ) ;
#16195=CARTESIAN_POINT ( 'NONE',  ( 10.81189881249999729, 0.000000000000000000, -139.5312500020484094 ) ) ;
#16196=CARTESIAN_POINT ( 'NONE',  ( 5.405949406249992428, -9.363379034771808662, -147.2812500020483810 ) ) ;
#16199=VERTEX_POINT ( 'NONE', #11222 ) ;
#16202=CARTESIAN_POINT ( 'NONE',  ( 5.405949406249999534, 9.363379034771803333, -176.5937500020484094 ) ) ;
#16203=CARTESIAN_POINT ( 'NONE',  ( 5.405949406249999534, 9.363379034771803333, -26.59375000204835970 ) ) ;
#16204=EDGE_CURVE ( 'NONE', #38561, #6885, #18468, .T. ) ;
#16206=CARTESIAN_POINT ( 'NONE',  ( 10.81189881249999729, 0.000000000000000000, -154.3437500020483810 ) ) ;
#16207=CARTESIAN_POINT ( 'NONE',  ( -10.81189881249999729, 1.324075727343319199E-15, -146.0937500020483810 ) ) ;
#16208=CARTESIAN_POINT ( 'NONE',  ( 10.00000000000012790, 5.773502691896179151, -173.2500000040967905 ) ) ;
#16212=CARTESIAN_POINT ( 'NONE',  ( 7.644554776091147741E-16, 12.48450537969573659, -14.46875000204836859 ) ) ;
#16214=DIRECTION ( 'NONE',  ( -0.000000000000000000, -0.000000000000000000, 1.000000000000000000 ) ) ;
#16218=CARTESIAN_POINT ( 'NONE',  ( -5.000000000000003553, -8.660254037844383745, -167.8750000040967905 ) ) ;
#16219=CARTESIAN_POINT ( 'NONE',  ( -5.405949406250003975, -9.363379034771801557, -72.34375000204836681 ) ) ;
#16220=CARTESIAN_POINT ( 'NONE',  ( -5.405949406250003975, -9.363379034771801557, -47.03125000204838813 ) ) ;
#16222=LINE ( 'NONE', #29422, #19882 ) ;
#16224=CARTESIAN_POINT ( 'NONE',  ( -2.121150477449813534E-15, -11.54700538379251284, -137.3750000000000000 ) ) ;
#16226=CARTESIAN_POINT ( 'NONE',  ( -5.405949406250003975, -9.363379034771801557, -135.5312500020484094 ) ) ;
#16228=CARTESIAN_POINT ( 'NONE',  ( 9.999999999999998224, 0.000000000000000000, -117.8750000040967905 ) ) ;
#16230=ORIENTED_EDGE ( 'NONE', *, *, #37696, .F. ) ;
#16234=CARTESIAN_POINT ( 'NONE',  ( 7.644554776091147741E-16, 12.48450537969573659, -175.1562500020484094 ) ) ;
#16235=CARTESIAN_POINT ( 'NONE',  ( -2.121150477449813534E-15, -11.54700538379251284, -43.25000000409675494 ) ) ;
#16236=CARTESIAN_POINT ( 'NONE',  ( -9.999999999999998224, 1.224646799147353059E-15, -48.12500000409677625 ) ) ;
#16238=DIRECTION ( 'NONE',  ( 1.000000000000000000, 1.502314598737160017E-16, 0.000000000000000000 ) ) ;
#16239=CARTESIAN_POINT ( 'NONE',  ( -10.81189881249999729, 1.324075727343319199E-15, -162.7812500020484094 ) ) ;
#16240=CARTESIAN_POINT ( 'NONE',  ( 7.644554776091147741E-16, 12.48450537969573659, -146.4687500020484094 ) ) ;
#16243=ORIENTED_EDGE ( 'NONE', *, *, #38620, .T. ) ;
#16244=( BOUNDED_CURVE ( )  B_SPLINE_CURVE ( 2, ( #17571, #20394, #4220, #33586, #17150, #21039, #18003 ),
 .UNSPECIFIED., .F., .F. ) 
 B_SPLINE_CURVE_WITH_KNOTS ( ( 3, 2, 2, 3 ),
 ( 0.8171641791044778058, 0.8184079601990051911, 0.8196517412935324653, 0.8208955223880598506 ),
 .UNSPECIFIED. ) 
 CURVE ( )  GEOMETRIC_REPRESENTATION_ITEM ( )  RATIONAL_B_SPLINE_CURVE ( ( 0.9999999999999761302, 0.8660254037844625774, 1.000000000000000000, 0.8660254037844387076, 1.000000000000000000, 0.8660254037844267172, 1.000000000000011990 ) ) 
 REPRESENTATION_ITEM ( '' )  );
#16245=CARTESIAN_POINT ( 'NONE',  ( 7.070501591499376803E-16, 11.54700538379251284, -114.5000000040967905 ) ) ;
#16246=AXIS2_PLACEMENT_3D ( 'NONE', #3025, #9074, #34993 ) ;
#16247=CARTESIAN_POINT ( 'NONE',  ( -2.293366432827344421E-15, -12.48450537969573659, -70.90625000204839523 ) ) ;
#16248=ORIENTED_EDGE ( 'NONE', *, *, #2566, .F. ) ;
#16250=CARTESIAN_POINT ( 'NONE',  ( 7.644554776091147741E-16, 12.48450537969573659, -117.9687500020483668 ) ) ;
#16251=ORIENTED_EDGE ( 'NONE', *, *, #35465, .T. ) ;
#16252=EDGE_LOOP ( 'NONE', ( #2700, #7411, #32420, #770 ) ) ;
#16253=CARTESIAN_POINT ( 'NONE',  ( 10.81189881249999729, 0.000000000000000000, -25.34375000204835970 ) ) ;
#16254=CARTESIAN_POINT ( 'NONE',  ( -2.293366432827344421E-15, -12.48450537969573659, -196.7187500020484094 ) ) ;
#16255=CARTESIAN_POINT ( 'NONE',  ( 10.81189881249999729, 0.000000000000000000, -47.84375000204838102 ) ) ;
#16259=CARTESIAN_POINT ( 'NONE',  ( -10.81189881249999729, 6.242252689847871849, -186.7187500020484379 ) ) ;
#16260=CARTESIAN_POINT ( 'NONE',  ( -10.81189881249999729, 6.242252689847871849, -165.7187500020483810 ) ) ;
#16263=CYLINDRICAL_SURFACE ( 'NONE', #8172, 9.999999999999998224 ) ;
#16266=CARTESIAN_POINT ( 'NONE',  ( -5.405949406249996869, 9.363379034771805109, -96.84375000204838102 ) ) ;
#16267=CARTESIAN_POINT ( 'NONE',  ( 7.070501591499376803E-16, 11.54700538379251284, -18.12499999999997513 ) ) ;
#16268=CARTESIAN_POINT ( 'NONE',  ( -5.405949406249996869, 9.363379034771805109, -77.53125000204838102 ) ) ;
#16269=CARTESIAN_POINT ( 'NONE',  ( 9.999999999999479527, 5.773502691896553074, -96.75000000409676204 ) ) ;
#16271=CARTESIAN_POINT ( 'NONE',  ( -10.81189881249999729, 6.242252689847871849, -159.9062500020483810 ) ) ;
#16273=CARTESIAN_POINT ( 'NONE',  ( -5.000000000000003553, -8.660254037844383745, -139.3750000040968189 ) ) ;
#16276=ORIENTED_EDGE ( 'NONE', *, *, #17483, .T. ) ;
#16280=CARTESIAN_POINT ( 'NONE',  ( -5.405949406250003975, -9.363379034771801557, -198.5312500020484094 ) ) ;
#16283=ORIENTED_EDGE ( 'NONE', *, *, #12451, .F. ) ;
#16284=CARTESIAN_POINT ( 'NONE',  ( 9.999999999999996447, -5.773502691896262640, -56.12499999999997868 ) ) ;
#16286=CARTESIAN_POINT ( 'NONE',  ( -9.999999999999998224, 1.224646799147353059E-15, -75.12500000409677625 ) ) ;
#16288=CARTESIAN_POINT ( 'NONE',  ( -9.999999999999742428, -5.773502691896402084, -160.5000000040968189 ) ) ;
#16290=CARTESIAN_POINT ( 'NONE',  ( 7.644554776091147741E-16, 12.48450537969573659, -71.65625000204836681 ) ) ;
#16291=( BOUNDED_CURVE ( )  B_SPLINE_CURVE ( 2, ( #23343, #19872, #39516, #33057, #39725, #3483, #40348 ),
 .UNSPECIFIED., .F., .F. ) 
 B_SPLINE_CURVE_WITH_KNOTS ( ( 3, 2, 2, 3 ),
 ( 0.9813432835820897759, 0.9825870646766171612, 0.9838308457711445465, 0.9850746268656718208 ),
 .UNSPECIFIED. ) 
 CURVE ( )  GEOMETRIC_REPRESENTATION_ITEM ( )  RATIONAL_B_SPLINE_CURVE ( ( 0.9999999999999761302, 0.8660254037844625774, 1.000000000000000000, 0.8660254037844387076, 1.000000000000000000, 0.8660254037844148378, 1.000000000000023981 ) ) 
 REPRESENTATION_ITEM ( '' )  );
#16294=DIRECTION ( 'NONE',  ( 1.000000000000000000, 0.000000000000000000, 0.000000000000000000 ) ) ;
#16295=CARTESIAN_POINT ( 'NONE',  ( -5.405949406250003975, -9.363379034771801557, -186.5312500020484094 ) ) ;
#16297=CARTESIAN_POINT ( 'NONE',  ( 10.81189881249999729, 6.242252689847867408, -1.218750002048353709 ) ) ;
#16299=CARTESIAN_POINT ( 'NONE',  ( 4.999999999999992006, -8.660254037844389075, -62.62500000409676204 ) ) ;
#16300=CARTESIAN_POINT ( 'NONE',  ( -9.999999999999998224, 0.8726646254783168022, 0.000000000000000000 ) ) ;
#16301=( BOUNDED_CURVE ( )  B_SPLINE_CURVE ( 2, ( #15373, #20312, #3500, #496, #6323, #10176, #36513 ),
 .UNSPECIFIED., .F., .F. ) 
 B_SPLINE_CURVE_WITH_KNOTS ( ( 3, 2, 2, 3 ),
 ( 0.5485074626865672487, 0.5497512437810946340, 0.5509950248756221303, 0.5522388059701495155 ),
 .UNSPECIFIED. ) 
 CURVE ( )  GEOMETRIC_REPRESENTATION_ITEM ( )  RATIONAL_B_SPLINE_CURVE ( ( 0.9999999999999880096, 0.8660254037844506980, 1.000000000000000000, 0.8660254037844387076, 1.000000000000000000, 0.8660254037844148378, 1.000000000000023981 ) ) 
 REPRESENTATION_ITEM ( '' )  );
#16302=CARTESIAN_POINT ( 'NONE',  ( 10.00000000000000000, 5.773502691896255534, -169.8750000000000000 ) ) ;
#16303=CARTESIAN_POINT ( 'NONE',  ( -9.999999999999998224, 1.224646799147353059E-15, -200.0000000000000000 ) ) ;
#16304=CARTESIAN_POINT ( 'NONE',  ( 10.81189881249999907, 6.242252689847868297, -95.90625000204839523 ) ) ;
#16306=CARTESIAN_POINT ( 'NONE',  ( 10.00000000000044764, -5.773502691896004180, -181.0000000040967620 ) ) ;
#16308=ORIENTED_EDGE ( 'NONE', *, *, #15377, .T. ) ;
#16310=EDGE_CURVE ( 'NONE', #28672, #30453, #37561, .T. ) ;
#16311=CARTESIAN_POINT ( 'NONE',  ( -10.81189881249999729, 1.324075727343319199E-15, -33.59375000204836681 ) ) ;
#16312=CARTESIAN_POINT ( 'NONE',  ( -5.405949406250003975, -9.363379034771801557, -21.53125000204836326 ) ) ;
#16313=CARTESIAN_POINT ( 'NONE',  ( 10.81189881249999551, -6.242252689847874514, -82.46875000204836681 ) ) ;
#16315=CARTESIAN_POINT ( 'NONE',  ( -10.81189881249999729, 1.324075727343319199E-15, -194.0937500020484094 ) ) ;
#16316=CARTESIAN_POINT ( 'NONE',  ( 0.000000000000000000, 0.000000000000000000, -200.0000000000000000 ) ) ;
#16319=CARTESIAN_POINT ( 'NONE',  ( -5.000000000000003553, -8.660254037844383745, -1.375000004096765815 ) ) ;
#16320=DIRECTION ( 'NONE',  ( -1.000000000000000000, -1.502314598737160017E-16, 0.000000000000000000 ) ) ;
#16321=CARTESIAN_POINT ( 'NONE',  ( -5.405949406250003975, -9.363379034771801557, -121.8437500020483952 ) ) ;
#16322=CARTESIAN_POINT ( 'NONE',  ( 5.405949406249999534, 9.363379034771803333, -101.7812500020483952 ) ) ;
#16323=CARTESIAN_POINT ( 'NONE',  ( -10.81189881249999729, -6.242252689847864744, -106.9687500020483810 ) ) ;
#16326=CARTESIAN_POINT ( 'NONE',  ( 9.999999999999996447, -5.773502691896262640, -164.5000000040967905 ) ) ;
#16327=CARTESIAN_POINT ( 'NONE',  ( -9.999999999999998224, 1.224646799147353059E-15, -81.12500000409677625 ) ) ;
#16331=DIRECTION ( 'NONE',  ( 1.000000000000000000, 0.000000000000000000, 0.000000000000000000 ) ) ;
#16333=CARTESIAN_POINT ( 'NONE',  ( 9.999999999999998224, 0.000000000000000000, -126.5000000000000000 ) ) ;
#16336=CARTESIAN_POINT ( 'NONE',  ( -4.999999999999996447, 8.660254037844387298, -82.49999999999998579 ) ) ;
#16338=CARTESIAN_POINT ( 'NONE',  ( -9.999999999999998224, 1.224646799147353059E-15, -94.62500000409677625 ) ) ;
#16339=DIRECTION ( 'NONE',  ( 1.000000000000000000, 0.000000000000000000, 0.000000000000000000 ) ) ;
#16341=CARTESIAN_POINT ( 'NONE',  ( 5.405949406249999534, 9.363379034771803333, -88.28125000204838102 ) ) ;
#16345=ORIENTED_EDGE ( 'NONE', *, *, #8806, .F. ) ;
#16346=CARTESIAN_POINT ( 'NONE',  ( -5.000000000000003553, -8.660254037844383745, -11.49999999999995381 ) ) ;
#16347=CARTESIAN_POINT ( 'NONE',  ( -4.999999999999996447, 8.660254037844387298, -148.5000000000000000 ) ) ;
#16349=CARTESIAN_POINT ( 'NONE',  ( -10.00000000000000000, -5.773502691896251982, -191.6250000000000284 ) ) ;
#16350=CARTESIAN_POINT ( 'NONE',  ( 5.405949406249992428, -9.363379034771808662, -114.2812500020483952 ) ) ;
#16353=CARTESIAN_POINT ( 'NONE',  ( -10.00000000000102496, 5.773502691895664007, -36.25000000409672651 ) ) ;
#16355=ORIENTED_EDGE ( 'NONE', *, *, #40022, .F. ) ;
#16356=CARTESIAN_POINT ( 'NONE',  ( 5.405949406249992428, -9.363379034771808662, -42.28125000204838102 ) ) ;
#16358=CARTESIAN_POINT ( 'NONE',  ( -5.405949406250003975, -9.363379034771801557, -99.34375000204838102 ) ) ;
#16359=CARTESIAN_POINT ( 'NONE',  ( -2.293366432827344421E-15, -12.48450537969573659, -123.4062500020483952 ) ) ;
#16360=ORIENTED_EDGE ( 'NONE', *, *, #2495, .F. ) ;
#16362=CARTESIAN_POINT ( 'NONE',  ( -8.659811548901195977, -5.000849327365069819, 0.000000000000000000 ) ) ;
#16363=CARTESIAN_POINT ( 'NONE',  ( -5.000000000000003553, -8.660254037844383745, -125.8750000040967905 ) ) ;
#16365=LINE ( 'NONE', #33820, #34429 ) ;
#16367=CARTESIAN_POINT ( 'NONE',  ( -10.81189881249999729, 6.242252689847871849, -131.2187500020483810 ) ) ;
#16369=LINE ( 'NONE', #22456, #35947 ) ;
#16371=CARTESIAN_POINT ( 'NONE',  ( 7.070501591499377789E-16, 11.54700538379251284, -194.0000000040967905 ) ) ;
#16373=CARTESIAN_POINT ( 'NONE',  ( -2.293366432827344421E-15, -12.48450537969573659, -184.9062500020484094 ) ) ;
#16374=CARTESIAN_POINT ( 'NONE',  ( -9.999999999999742428, -5.773502691896402084, -186.0000000040967905 ) ) ;
#16375=DIRECTION ( 'NONE',  ( -0.000000000000000000, -0.000000000000000000, 1.000000000000000000 ) ) ;
#16378=CARTESIAN_POINT ( 'NONE',  ( -10.81189881249999729, -6.242252689847864744, -60.46875000204836681 ) ) ;
#16379=CARTESIAN_POINT ( 'NONE',  ( -5.405949406250003975, -9.363379034771801557, -52.84375000204835970 ) ) ;
#16381=CARTESIAN_POINT ( 'NONE',  ( 5.405949406249992428, -9.363379034771808662, -18.28125000204835970 ) ) ;
#16382=VECTOR ( 'NONE', #19783, 1000.000000000000000 ) ;
#16386=ADVANCED_FACE ( 'NONE', ( #7191 ), #34125, .T. ) ;
#16387=CARTESIAN_POINT ( 'NONE',  ( -5.000000000000003553, -8.660254037844383745, -103.0000000000000000 ) ) ;
#16390=EDGE_CURVE ( 'NONE', #5036, #10156, #26791, .T. ) ;
#16393=CARTESIAN_POINT ( 'NONE',  ( -10.81189881249999729, 6.242252689847871849, -116.4062500020483952 ) ) ;
#16394=ORIENTED_EDGE ( 'NONE', *, *, #18829, .F. ) ;
#16395=CARTESIAN_POINT ( 'NONE',  ( 5.000000000000000000, 8.660254037844385522, -160.7500000000000000 ) ) ;
#16399=ORIENTED_EDGE ( 'NONE', *, *, #24629, .T. ) ;
#16400=CARTESIAN_POINT ( 'NONE',  ( 5.000000000000000000, 8.660254037844385522, -33.24999999999997158 ) ) ;
#16401=CARTESIAN_POINT ( 'NONE',  ( -9.999999999999998224, 1.224646799147353059E-15, -19.62500000409675494 ) ) ;
#16402=CARTESIAN_POINT ( 'NONE',  ( -10.81189881249999729, 6.242252689847871849, -41.40625000204836681 ) ) ;
#16403=LINE ( 'NONE', #23761, #37298 ) ;
#16405=CYLINDRICAL_SURFACE ( 'NONE', #23148, 9.999999999999998224 ) ;
#16406=CARTESIAN_POINT ( 'NONE',  ( 10.81189881249999907, 6.242252689847868297, -136.4062500020484094 ) ) ;
#16407=CARTESIAN_POINT ( 'NONE',  ( -5.405949406249996869, 9.363379034771805109, -142.0312500020483810 ) ) ;
#16408=ADVANCED_FACE ( 'NONE', ( #17686 ), #34769, .F. ) ;
#16410=ORIENTED_EDGE ( 'NONE', *, *, #1916, .F. ) ;
#16411=( BOUNDED_CURVE ( )  B_SPLINE_CURVE ( 2, ( #14479, #39754, #10189, #36524, #26817, #10399, #23589 ),
 .UNSPECIFIED., .F., .F. ) 
 B_SPLINE_CURVE_WITH_KNOTS ( ( 3, 2, 2, 3 ),
 ( 0.4216417910447762818, 0.4228855721393036671, 0.4241293532338309413, 0.4253731343283583266 ),
 .UNSPECIFIED. ) 
 CURVE ( )  GEOMETRIC_REPRESENTATION_ITEM ( )  RATIONAL_B_SPLINE_CURVE ( ( 0.9999999999999820144, 0.8660254037844566932, 1.000000000000000000, 0.8660254037844387076, 1.000000000000000000, 0.8660254037844267172, 1.000000000000011990 ) ) 
 REPRESENTATION_ITEM ( '' )  );
#16414=ORIENTED_EDGE ( 'NONE', *, *, #35988, .T. ) ;
#16415=EDGE_CURVE ( 'NONE', #33809, #1539, #8017, .T. ) ;
#16416=VECTOR ( 'NONE', #3142, 1000.000000000000000 ) ;
#16417=CARTESIAN_POINT ( 'NONE',  ( 7.644554776091147741E-16, 12.48450537969573659, -171.9687500020483810 ) ) ;
#16418=CARTESIAN_POINT ( 'NONE',  ( 10.81189881249999729, 0.000000000000000000, -26.84375000204835970 ) ) ;
#16419=DIRECTION ( 'NONE',  ( -0.000000000000000000, -0.000000000000000000, 1.000000000000000000 ) ) ;
#16420=CARTESIAN_POINT ( 'NONE',  ( -2.293366432827344421E-15, -12.48450537969573659, -153.2187500020483810 ) ) ;
#16421=CARTESIAN_POINT ( 'NONE',  ( 7.644554776091147741E-16, 12.48450537969573659, -147.9687500020484094 ) ) ;
#16425=CARTESIAN_POINT ( 'NONE',  ( -2.293366432827344421E-15, -12.48450537969573659, -19.71875000204837747 ) ) ;
#16431=CARTESIAN_POINT ( 'NONE',  ( 10.81189881249999907, 6.242252689847868297, -74.71875000204838102 ) ) ;
#16432=CARTESIAN_POINT ( 'NONE',  ( -10.81189881249999729, 6.242252689847871849, -44.40625000204836681 ) ) ;
#16434=CARTESIAN_POINT ( 'NONE',  ( -9.999999999999998224, 1.224646799147353059E-15, -200.0000000000000000 ) ) ;
#16437=CARTESIAN_POINT ( 'NONE',  ( 7.070501591499377789E-16, 11.54700538379251284, -132.1250000000000000 ) ) ;
#16438=CARTESIAN_POINT ( 'NONE',  ( 5.405949406249999534, 9.363379034771803333, -142.2812500020483810 ) ) ;
#16439=DIRECTION ( 'NONE',  ( -0.000000000000000000, -0.000000000000000000, 1.000000000000000000 ) ) ;
#16440=CARTESIAN_POINT ( 'NONE',  ( 7.070501591499377789E-16, 11.54700538379251284, -114.5000000040967905 ) ) ;
#16446=CARTESIAN_POINT ( 'NONE',  ( 9.999999999998969713, 5.773502691896851502, -39.37499999999995026 ) ) ;
#16448=CARTESIAN_POINT ( 'NONE',  ( -10.81189881249999729, 1.324075727343319199E-15, -170.2812500020484094 ) ) ;
#16449=CARTESIAN_POINT ( 'NONE',  ( -9.999999999999998224, 5.773502691896259087, -40.75000000409676204 ) ) ;
#16451=CARTESIAN_POINT ( 'NONE',  ( 9.999999999999998224, 0.000000000000000000, -48.87500000409678336 ) ) ;
#16454=CARTESIAN_POINT ( 'NONE',  ( -5.405949406250003975, -9.363379034771801557, -161.0312500020484094 ) ) ;
#16455=VECTOR ( 'NONE', #34680, 1000.000000000000000 ) ;
#16456=CARTESIAN_POINT ( 'NONE',  ( 5.405949406249992428, -9.363379034771808662, -147.0937500020483810 ) ) ;
#16457=CYLINDRICAL_SURFACE ( 'NONE', #4979, 9.999999999999998224 ) ;
#16459=ORIENTED_EDGE ( 'NONE', *, *, #26285, .F. ) ;
#16460=CARTESIAN_POINT ( 'NONE',  ( 9.999999999999998224, 0.000000000000000000, -28.99999999999997158 ) ) ;
#16463=CARTESIAN_POINT ( 'NONE',  ( 10.81189881249999907, 6.242252689847868297, -67.40625000204839523 ) ) ;
#16464=VERTEX_POINT ( 'NONE', #25890 ) ;
#16466=CARTESIAN_POINT ( 'NONE',  ( -10.81189881249999729, 1.324075727343319199E-15, -119.0937500020483810 ) ) ;
#16468=ORIENTED_EDGE ( 'NONE', *, *, #37813, .F. ) ;
#16469=CARTESIAN_POINT ( 'NONE',  ( 7.644554776091147741E-16, 12.48450537969573659, -23.46875000204836326 ) ) ;
#16470=CARTESIAN_POINT ( 'NONE',  ( 5.405949406249992428, -9.363379034771808662, -0.2812500020483721386 ) ) ;
#16471=CARTESIAN_POINT ( 'NONE',  ( 10.81189881249999729, 0.000000000000000000, -46.34375000204838102 ) ) ;
#16472=DIRECTION ( 'NONE',  ( -0.000000000000000000, -0.000000000000000000, 1.000000000000000000 ) ) ;
#16474=CARTESIAN_POINT ( 'NONE',  ( 10.81189881249999729, 6.242252689847867408, -182.7187500020484094 ) ) ;
#16475=CARTESIAN_POINT ( 'NONE',  ( 5.405949406249999534, 9.363379034771803333, -169.0937500020484094 ) ) ;
#16479=CARTESIAN_POINT ( 'NONE',  ( -9.999999999999998224, 1.224646799147353059E-15, -193.6250000040967905 ) ) ;
#16481=VECTOR ( 'NONE', #23505, 1000.000000000000000 ) ;
#16482=CARTESIAN_POINT ( 'NONE',  ( -10.81189881249999729, 6.242252689847871849, -93.71875000204838102 ) ) ;
#16483=CARTESIAN_POINT ( 'NONE',  ( 7.070501591499376803E-16, 11.54700538379251284, -198.5000000040968189 ) ) ;
#16484=CARTESIAN_POINT ( 'NONE',  ( 10.81189881249999907, 6.242252689847868297, -65.90625000204839523 ) ) ;
#16487=CARTESIAN_POINT ( 'NONE',  ( -5.405949406249996869, 9.363379034771805109, -166.0312500020484094 ) ) ;
#16489=CARTESIAN_POINT ( 'NONE',  ( 9.999999999999996447, -5.773502691896262640, -137.5000000040967905 ) ) ;
#16491=ORIENTED_EDGE ( 'NONE', *, *, #29746, .F. ) ;
#16495=CARTESIAN_POINT ( 'NONE',  ( 10.81189881249999729, 0.000000000000000000, -196.5312500020484094 ) ) ;
#16498=VERTEX_POINT ( 'NONE', #35188 ) ;
#16499=CARTESIAN_POINT ( 'NONE',  ( 10.00000000000000000, 5.773502691896255534, -58.87499999999998579 ) ) ;
#16501=CARTESIAN_POINT ( 'NONE',  ( 9.999999999999998224, 0.000000000000000000, -69.87500000409677625 ) ) ;
#16503=( BOUNDED_CURVE ( )  B_SPLINE_CURVE ( 2, ( #5928, #21896, #11746, #38508, #32260, #28174, #21468 ),
 .UNSPECIFIED., .F., .F. ) 
 B_SPLINE_CURVE_WITH_KNOTS ( ( 3, 2, 2, 3 ),
 ( 0.9402985074626868389, 0.9415422885572141132, 0.9427860696517416095, 0.9440298507462689948 ),
 .UNSPECIFIED. ) 
 CURVE ( )  GEOMETRIC_REPRESENTATION_ITEM ( )  RATIONAL_B_SPLINE_CURVE ( ( 0.9999999999999761302, 0.8660254037844625774, 1.000000000000000000, 0.8660254037844387076, 1.000000000000000000, 0.8660254037844028474, 1.000000000000035971 ) ) 
 REPRESENTATION_ITEM ( '' )  );
#16506=CARTESIAN_POINT ( 'NONE',  ( 10.81189881249999551, -6.242252689847874514, -61.65625000204838813 ) ) ;
#16509=FACE_OUTER_BOUND ( 'NONE', #32855, .T. ) ;
#16510=CARTESIAN_POINT ( 'NONE',  ( -10.81189881249999729, 1.324075727343319199E-15, -183.7812500020484094 ) ) ;
#16513=CARTESIAN_POINT ( 'NONE',  ( 0.000000000000000000, 0.000000000000000000, -200.0000000000000000 ) ) ;
#16514=CARTESIAN_POINT ( 'NONE',  ( 10.00000000000025402, -5.773502691896113426, -117.6250000000000142 ) ) ;
#16515=CARTESIAN_POINT ( 'NONE',  ( -9.106632906167126507, -4.221636404539722776, 0.000000000000000000 ) ) ;
#16516=CARTESIAN_POINT ( 'NONE',  ( -7.688134889256605042, 6.454000733898044295, 0.000000000000000000 ) ) ;
#16517=CARTESIAN_POINT ( 'NONE',  ( 10.00000000000000000, 5.773502691896255534, -168.3750000000000000 ) ) ;
#16520=CARTESIAN_POINT ( 'NONE',  ( 10.81189881249999907, 6.242252689847868297, -92.90625000204839523 ) ) ;
#16521=ORIENTED_EDGE ( 'NONE', *, *, #25421, .T. ) ;
#16522=CARTESIAN_POINT ( 'NONE',  ( 4.999999999999992006, -8.660254037844389075, -162.7500000000000000 ) ) ;
#16523=CARTESIAN_POINT ( 'NONE',  ( 0.000000000000000000, 0.000000000000000000, -200.0000000000000000 ) ) ;
#16525=ORIENTED_EDGE ( 'NONE', *, *, #31200, .T. ) ;
#16526=CARTESIAN_POINT ( 'NONE',  ( -10.81189881249999729, 1.324075727343319199E-15, -30.59375000204836326 ) ) ;
#16527=CARTESIAN_POINT ( 'NONE',  ( -5.405949406249996869, 9.363379034771805109, -25.03125000204836681 ) ) ;
#16529=CARTESIAN_POINT ( 'NONE',  ( -10.81189881249999907, -6.242252689847864744, -73.96875000204836681 ) ) ;
#16530=CARTESIAN_POINT ( 'NONE',  ( 7.070501591499376803E-16, 11.54700538379251284, -105.1249999999999858 ) ) ;
#16531=CARTESIAN_POINT ( 'NONE',  ( 10.81189881249999907, 6.242252689847868297, -196.2187500020484094 ) ) ;
#16532=CARTESIAN_POINT ( 'NONE',  ( -5.405949406250003975, -9.363379034771801557, -147.3437500020483810 ) ) ;
#16533=LINE ( 'NONE', #6426, #5407 ) ;
#16536=CARTESIAN_POINT ( 'NONE',  ( 7.070501591499377789E-16, 11.54700538379251284, -0.5000000040967461645 ) ) ;
#16538=CARTESIAN_POINT ( 'NONE',  ( -10.81189881249999729, 6.242252689847871849, -117.7187500020483952 ) ) ;
#16539=CARTESIAN_POINT ( 'NONE',  ( -10.81189881249999729, 6.242252689847871849, -95.40625000204838102 ) ) ;
#16540=CARTESIAN_POINT ( 'NONE',  ( 5.405949406249992428, -9.363379034771808662, -105.0937500020483810 ) ) ;
#16543=CARTESIAN_POINT ( 'NONE',  ( 9.999999999999998224, 0.000000000000000000, -162.8750000040967905 ) ) ;
#16544=( BOUNDED_CURVE ( )  B_SPLINE_CURVE ( 2, ( #16061, #38538, #28842, #16267, #31879, #26019, #22146 ),
 .UNSPECIFIED., .F., .F. ) 
 B_SPLINE_CURVE_WITH_KNOTS ( ( 3, 2, 2, 3 ),
 ( 0.9029850746268659467, 0.9042288557213932210, 0.9054726368159207173, 0.9067164179104481025 ),
 .UNSPECIFIED. ) 
 CURVE ( )  GEOMETRIC_REPRESENTATION_ITEM ( )  RATIONAL_B_SPLINE_CURVE ( ( 0.9999999999999761302, 0.8660254037844625774, 1.000000000000000000, 0.8660254037844387076, 1.000000000000000000, 0.8660254037844028474, 1.000000000000035971 ) ) 
 REPRESENTATION_ITEM ( '' )  );
#16545=CARTESIAN_POINT ( 'NONE',  ( 0.000000000000000000, 0.000000000000000000, -200.0000000000000000 ) ) ;
#16548=AXIS2_PLACEMENT_3D ( 'NONE', #33008, #6884, #33230 ) ;
#16550=CARTESIAN_POINT ( 'NONE',  ( -2.121150477449813534E-15, -11.54700538379251284, -189.8750000000000284 ) ) ;
#16552=CARTESIAN_POINT ( 'NONE',  ( -2.121150477449813534E-15, -11.54700538379251284, -108.8749999999999858 ) ) ;
#16554=CARTESIAN_POINT ( 'NONE',  ( 4.999999999999992006, -8.660254037844389075, -81.74999999999998579 ) ) ;
#16556=CARTESIAN_POINT ( 'NONE',  ( 4.999999999999992006, -8.660254037844389075, -86.62500000409677625 ) ) ;
#16559=CARTESIAN_POINT ( 'NONE',  ( -5.405949406249996869, 9.363379034771805109, -88.03125000204838102 ) ) ;
#16561=( BOUNDED_CURVE ( )  B_SPLINE_CURVE ( 2, ( #19764, #26049, #22807, #39827, #29282, #7247, #10260 ),
 .UNSPECIFIED., .F., .F. ) 
 B_SPLINE_CURVE_WITH_KNOTS ( ( 3, 2, 2, 3 ),
 ( 0.5970149253731344974, 0.5982587064676618827, 0.5995024875621891569, 0.6007462686567165422 ),
 .UNSPECIFIED. ) 
 CURVE ( )  GEOMETRIC_REPRESENTATION_ITEM ( )  RATIONAL_B_SPLINE_CURVE ( ( 0.9999999999999761302, 0.8660254037844625774, 1.000000000000000000, 0.8660254037844387076, 1.000000000000000000, 0.8660254037844267172, 1.000000000000011990 ) ) 
 REPRESENTATION_ITEM ( '' )  );
#16566=CARTESIAN_POINT ( 'NONE',  ( -2.121150477449813534E-15, -11.54700538379251284, -9.874999999999982236 ) ) ;
#16567=CARTESIAN_POINT ( 'NONE',  ( -9.999999999999998224, 1.224646799147353059E-15, -142.2500000000000000 ) ) ;
#16568=DIRECTION ( 'NONE',  ( -0.000000000000000000, -0.000000000000000000, 1.000000000000000000 ) ) ;
#16570=CARTESIAN_POINT ( 'NONE',  ( 5.000000000000000000, 8.660254037844385522, -189.2500000000000000 ) ) ;
#16571=CARTESIAN_POINT ( 'NONE',  ( -10.81189881249999907, -6.242252689847864744, -116.1562500020483952 ) ) ;
#16572=ORIENTED_EDGE ( 'NONE', *, *, #20226, .T. ) ;
#16573=CARTESIAN_POINT ( 'NONE',  ( -4.999999999999996447, 8.660254037844387298, -13.49999999999995737 ) ) ;
#16574=ADVANCED_FACE ( 'NONE', ( #12284 ), #22641, .F. ) ;
#16576=CARTESIAN_POINT ( 'NONE',  ( -10.81189881249999729, 6.242252689847871849, -48.90625000204836681 ) ) ;
#16578=CARTESIAN_POINT ( 'NONE',  ( -10.81189881249999907, -6.242252689847864744, -96.46875000204838102 ) ) ;
#16579=CARTESIAN_POINT ( 'NONE',  ( -2.293366432827344421E-15, -12.48450537969573659, -120.4062500020483952 ) ) ;
#16580=ORIENTED_EDGE ( 'NONE', *, *, #38580, .F. ) ;
#16581=DIRECTION ( 'NONE',  ( -0.000000000000000000, -0.000000000000000000, 1.000000000000000000 ) ) ;
#16584=CYLINDRICAL_SURFACE ( 'NONE', #39018, 9.999999999999998224 ) ;
#16585=CARTESIAN_POINT ( 'NONE',  ( -10.81189881249999729, -6.242252689847864744, -132.4687500020483810 ) ) ;
#16587=CARTESIAN_POINT ( 'NONE',  ( 4.999999999999992006, -8.660254037844389075, -158.2500000000000000 ) ) ;
#16589=CARTESIAN_POINT ( 'NONE',  ( 7.070501591499377789E-16, 11.54700538379251284, -186.5000000040967905 ) ) ;
#16591=CARTESIAN_POINT ( 'NONE',  ( -10.81189881249999729, 1.324075727343319199E-15, -186.7812500020484094 ) ) ;
#16592=CARTESIAN_POINT ( 'NONE',  ( -9.999999999999998224, 1.224646799147353059E-15, -6.125000004096770034 ) ) ;
#16593=DIRECTION ( 'NONE',  ( 1.000000000000000000, 0.000000000000000000, 0.000000000000000000 ) ) ;
#16596=CARTESIAN_POINT ( 'NONE',  ( -10.81189881249999729, -6.242252689847864744, -63.46875000204838102 ) ) ;
#16597=CARTESIAN_POINT ( 'NONE',  ( 7.644554776091147741E-16, 12.48450537969573659, -45.96875000204837391 ) ) ;
#16599=CARTESIAN_POINT ( 'NONE',  ( -5.405949406249996869, 9.363379034771805109, -19.03125000204835970 ) ) ;
#16601=CARTESIAN_POINT ( 'NONE',  ( 9.999999999999998224, 0.000000000000000000, -92.37500000409677625 ) ) ;
#16603=CARTESIAN_POINT ( 'NONE',  ( -9.999999999999998224, 1.224646799147353059E-15, -109.2499999999999858 ) ) ;
#16605=CARTESIAN_POINT ( 'NONE',  ( 5.000000000000000000, 8.660254037844385522, -163.7500000000000000 ) ) ;
#16608=CARTESIAN_POINT ( 'NONE',  ( -10.81189881249999729, -6.242252689847864744, -119.1562500020484237 ) ) ;
#16609=ORIENTED_EDGE ( 'NONE', *, *, #2895, .T. ) ;
#16611=CARTESIAN_POINT ( 'NONE',  ( 10.00000000000102318, -5.773502691895667560, -6.624999999999941380 ) ) ;
#16615=CARTESIAN_POINT ( 'NONE',  ( 9.999999999999996447, -5.773502691896262640, -35.12499999999996447 ) ) ;
#16617=CARTESIAN_POINT ( 'NONE',  ( 9.999999999999996447, -5.773502691896262640, -20.50000000409677625 ) ) ;
#16618=CARTESIAN_POINT ( 'NONE',  ( 5.405949406249992428, -9.363379034771808662, -43.78125000204838102 ) ) ;
#16619=DIRECTION ( 'NONE',  ( -0.000000000000000000, -0.000000000000000000, 1.000000000000000000 ) ) ;
#16621=CARTESIAN_POINT ( 'NONE',  ( 9.999999999999998224, 0.000000000000000000, -156.8750000040967905 ) ) ;
#16622=VECTOR ( 'NONE', #34014, 1000.000000000000000 ) ;
#16623=CARTESIAN_POINT ( 'NONE',  ( 10.81189881249999729, 0.000000000000000000, -145.5312500020483810 ) ) ;
#16624=( BOUNDED_CURVE ( )  B_SPLINE_CURVE ( 2, ( #5905, #42136, #2035, #24704, #37850, #8293, #12146 ),
 .UNSPECIFIED., .F., .F. ) 
 B_SPLINE_CURVE_WITH_KNOTS ( ( 3, 2, 2, 3 ),
 ( 0.6417910447761195902, 0.6430348258706469755, 0.6442786069651742498, 0.6455223880597016350 ),
 .UNSPECIFIED. ) 
 CURVE ( )  GEOMETRIC_REPRESENTATION_ITEM ( )  RATIONAL_B_SPLINE_CURVE ( ( 0.9999999999999761302, 0.8660254037844625774, 1.000000000000000000, 0.8660254037844387076, 1.000000000000000000, 0.8660254037844267172, 1.000000000000011990 ) ) 
 REPRESENTATION_ITEM ( '' )  );
#16625=CARTESIAN_POINT ( 'NONE',  ( -9.999999999998969713, -5.773502691896847949, -16.12499999999995737 ) ) ;
#16626=ORIENTED_EDGE ( 'NONE', *, *, #631, .T. ) ;
#16627=EDGE_LOOP ( 'NONE', ( #39522, #16992, #19829, #15938 ) ) ;
#16628=EDGE_CURVE ( 'NONE', #6595, #12803, #19842, .T. ) ;
#16629=VERTEX_POINT ( 'NONE', #32769 ) ;
#16631=CARTESIAN_POINT ( 'NONE',  ( 9.999999999999998224, 0.000000000000000000, -120.8750000040967905 ) ) ;
#16632=CARTESIAN_POINT ( 'NONE',  ( 5.405949406249992428, -9.363379034771808662, -175.5937500020484094 ) ) ;
#16634=CARTESIAN_POINT ( 'NONE',  ( -10.81189881249999729, 1.324075727343319199E-15, -21.59375000204835615 ) ) ;
#16636=CARTESIAN_POINT ( 'NONE',  ( -10.81189881249999729, -6.242252689847864744, -156.4687500020484094 ) ) ;
#16637=CARTESIAN_POINT ( 'NONE',  ( -2.293366432827344421E-15, -12.48450537969573659, -145.7187500020484094 ) ) ;
#16638=CARTESIAN_POINT ( 'NONE',  ( 7.070501591499376803E-16, 11.54700538379251284, -67.62500000000000000 ) ) ;
#16641=CARTESIAN_POINT ( 'NONE',  ( 7.644554776091147741E-16, 12.48450537969573659, -6.968750002048349046 ) ) ;
#16643=CYLINDRICAL_SURFACE ( 'NONE', #2653, 9.999999999999998224 ) ;
#16644=DIRECTION ( 'NONE',  ( -0.000000000000000000, -0.000000000000000000, 1.000000000000000000 ) ) ;
#16646=CARTESIAN_POINT ( 'NONE',  ( 9.999999999999998224, 0.000000000000000000, -100.9999999999999858 ) ) ;
#16647=CIRCLE ( 'NONE', #12542, 10.00000000000000178 ) ;
#16648=CARTESIAN_POINT ( 'NONE',  ( -2.293366432827344421E-15, -12.48450537969573659, -73.71875000204835260 ) ) ;
#16649=CARTESIAN_POINT ( 'NONE',  ( 7.644554776091147741E-16, 12.48450537969573659, -46.15625000204837391 ) ) ;
#16651=CARTESIAN_POINT ( 'NONE',  ( 9.999999999999998224, 0.000000000000000000, -57.49999999999996447 ) ) ;
#16653=CARTESIAN_POINT ( 'NONE',  ( -10.00000000000000000, -5.773502691896251982, -127.1249999999999858 ) ) ;
#16654=CARTESIAN_POINT ( 'NONE',  ( 7.644554776091147741E-16, 12.48450537969573659, -136.1562500020484094 ) ) ;
#16655=CARTESIAN_POINT ( 'NONE',  ( -9.999999999999479527, -5.773502691896549521, -151.1250000000000000 ) ) ;
#16656=CARTESIAN_POINT ( 'NONE',  ( -9.999999999999998224, 5.773502691896259087, -117.2500000040967763 ) ) ;
#16661=CARTESIAN_POINT ( 'NONE',  ( 9.999999999999998224, 0.000000000000000000, -200.0000000000000000 ) ) ;
#16662=CARTESIAN_POINT ( 'NONE',  ( 10.81189881249999907, 6.242252689847868297, -167.9062500020484094 ) ) ;
#16663=CARTESIAN_POINT ( 'NONE',  ( -2.121150477449813534E-15, -11.54700538379251284, -41.75000000409675494 ) ) ;
#16664=DIRECTION ( 'NONE',  ( 1.000000000000000000, 0.000000000000000000, 0.000000000000000000 ) ) ;
#16666=AXIS2_PLACEMENT_3D ( 'NONE', #10487, #23676, #32751 ) ;
#16667=( BOUNDED_CURVE ( )  B_SPLINE_CURVE ( 2, ( #14041, #1134, #6964, #7174, #11038, #27237, #20326 ),
 .UNSPECIFIED., .F., .F. ) 
 B_SPLINE_CURVE_WITH_KNOTS ( ( 3, 2, 2, 3 ),
 ( 0.06716417910447768091, 0.06840796019900503844, 0.06965174129353240984, 0.07089552238805976736 ),
 .UNSPECIFIED. ) 
 CURVE ( )  GEOMETRIC_REPRESENTATION_ITEM ( )  RATIONAL_B_SPLINE_CURVE ( ( 0.9999999999999924505, 0.8660254037844461461, 1.000000000000000000, 0.8660254037844387076, 1.000000000000000000, 0.8660254037844312691, 1.000000000000007550 ) ) 
 REPRESENTATION_ITEM ( '' )  );
#16668=CARTESIAN_POINT ( 'NONE',  ( 10.40594940624999865, 0.000000000000000000, -199.7656250010242047 ) ) ;
#16669=CARTESIAN_POINT ( 'NONE',  ( 5.405949406249999534, 9.363379034771803333, -161.7812500020484094 ) ) ;
#16670=CARTESIAN_POINT ( 'NONE',  ( -10.81189881249999729, 1.324075727343319199E-15, -138.5937500020483810 ) ) ;
#16671=CARTESIAN_POINT ( 'NONE',  ( 9.999999999999998224, 0.000000000000000000, -200.0000000000000000 ) ) ;
#16672=CARTESIAN_POINT ( 'NONE',  ( -9.999999999999998224, 1.224646799147353059E-15, -149.7500000000000000 ) ) ;
#16673=ORIENTED_EDGE ( 'NONE', *, *, #40653, .F. ) ;
#16674=CARTESIAN_POINT ( 'NONE',  ( -4.999999999999996447, 8.660254037844387298, -189.3750000040967905 ) ) ;
#16675=AXIS2_PLACEMENT_3D ( 'NONE', #17729, #15135, #1792 ) ;
#16676=CARTESIAN_POINT ( 'NONE',  ( -2.293366432827344421E-15, -12.48450537969573659, -72.40625000204836681 ) ) ;
#16677=ORIENTED_EDGE ( 'NONE', *, *, #15933, .F. ) ;
#16680=CARTESIAN_POINT ( 'NONE',  ( -5.405949406250003975, -9.363379034771801557, -120.3437500020483952 ) ) ;
#16681=ORIENTED_EDGE ( 'NONE', *, *, #6386, .T. ) ;
#16682=ORIENTED_EDGE ( 'NONE', *, *, #11456, .T. ) ;
#16684=CARTESIAN_POINT ( 'NONE',  ( 10.81189881249999729, 0.000000000000000000, -19.34375000204835260 ) ) ;
#16685=CARTESIAN_POINT ( 'NONE',  ( 10.81189881249999907, 6.242252689847868297, -196.2187500020484094 ) ) ;
#16686=CARTESIAN_POINT ( 'NONE',  ( -2.293366432827344421E-15, -12.48450537969573659, -43.71875000204835970 ) ) ;
#16687=CARTESIAN_POINT ( 'NONE',  ( 0.000000000000000000, 0.000000000000000000, -200.0000000000000000 ) ) ;
#16688=CARTESIAN_POINT ( 'NONE',  ( 0.000000000000000000, 0.000000000000000000, -200.0000000000000000 ) ) ;
#16689=CARTESIAN_POINT ( 'NONE',  ( 10.81189881249999551, -6.242252689847874514, -179.9687500020484094 ) ) ;
#16690=CARTESIAN_POINT ( 'NONE',  ( 5.405949406249992428, -9.363379034771808662, -172.5937500020484094 ) ) ;
#16694=DIRECTION ( 'NONE',  ( -0.000000000000000000, -0.000000000000000000, 1.000000000000000000 ) ) ;
#16695=CARTESIAN_POINT ( 'NONE',  ( 0.000000000000000000, 0.000000000000000000, -200.0000000000000000 ) ) ;
#16697=CARTESIAN_POINT ( 'NONE',  ( -10.81189881249999907, -6.242252689847864744, -100.9687500020483810 ) ) ;
#16698=LINE ( 'NONE', #36994, #23800 ) ;
#16699=CARTESIAN_POINT ( 'NONE',  ( -5.405949406249996869, 9.363379034771805109, -65.53125000204838102 ) ) ;
#16702=CARTESIAN_POINT ( 'NONE',  ( 10.81189881249999907, 6.242252689847868297, -119.9062500020483810 ) ) ;
#16703=CARTESIAN_POINT ( 'NONE',  ( 7.644554776091147741E-16, 12.48450537969573659, -166.1562500020483810 ) ) ;
#16705=CARTESIAN_POINT ( 'NONE',  ( -10.00000000000000000, -5.773502691896251982, -139.5000000040967905 ) ) ;
#16707=ORIENTED_EDGE ( 'NONE', *, *, #21426, .F. ) ;
#16712=CARTESIAN_POINT ( 'NONE',  ( 5.405949406249992428, -9.363379034771808662, -190.7812500020484094 ) ) ;
#16713=CARTESIAN_POINT ( 'NONE',  ( -10.00000000000102496, 5.773502691895664007, -130.7500000040967620 ) ) ;
#16716=CARTESIAN_POINT ( 'NONE',  ( -10.00000000000000000, -5.773502691896251982, -61.12499999999998579 ) ) ;
#16718=CARTESIAN_POINT ( 'NONE',  ( -10.00000000000000000, -5.773502691896251982, -69.00000000409677625 ) ) ;
#16719=CARTESIAN_POINT ( 'NONE',  ( 0.000000000000000000, 0.000000000000000000, -200.0000000000000000 ) ) ;
#16722=CARTESIAN_POINT ( 'NONE',  ( -5.405949406249996869, 9.363379034771805109, -58.03125000204836681 ) ) ;
#16726=CARTESIAN_POINT ( 'NONE',  ( 10.81189881249999551, -6.242252689847874514, -187.6562500020484379 ) ) ;
#16728=DIRECTION ( 'NONE',  ( -1.000000000000000000, 0.000000000000000000, 0.000000000000000000 ) ) ;
#16729=DIRECTION ( 'NONE',  ( 1.000000000000000000, 0.000000000000000000, 0.000000000000000000 ) ) ;
#16730=CARTESIAN_POINT ( 'NONE',  ( -9.096586351904823786, 4.244250262519885020, 0.000000000000000000 ) ) ;
#16731=CARTESIAN_POINT ( 'NONE',  ( 5.000000000000000000, 8.660254037844385522, -168.2500000000000000 ) ) ;
#16732=CARTESIAN_POINT ( 'NONE',  ( -2.121150477449813534E-15, -11.54700538379251284, -169.2500000040968189 ) ) ;
#16733=CARTESIAN_POINT ( 'NONE',  ( -10.81189881249999907, -6.242252689847864744, -93.65625000204840944 ) ) ;
#16735=CARTESIAN_POINT ( 'NONE',  ( -9.999999999999998224, 1.224646799147353059E-15, -163.2500000000000000 ) ) ;
#16736=CARTESIAN_POINT ( 'NONE',  ( 0.000000000000000000, 0.000000000000000000, -200.0000000000000000 ) ) ;
#16737=ORIENTED_EDGE ( 'NONE', *, *, #3279, .T. ) ;
#16739=CARTESIAN_POINT ( 'NONE',  ( 5.405949406249992428, -9.363379034771808662, -33.09375000204836681 ) ) ;
#16740=CARTESIAN_POINT ( 'NONE',  ( -10.81189881249999907, -6.242252689847864744, -18.65625000204837036 ) ) ;
#16742=CARTESIAN_POINT ( 'NONE',  ( -5.405949406249996869, 9.363379034771805109, -72.84375000204838102 ) ) ;
#16743=CARTESIAN_POINT ( 'NONE',  ( -5.405949406250003975, -9.363379034771801557, -193.8437500020484094 ) ) ;
#16744=CARTESIAN_POINT ( 'NONE',  ( 5.405949406249992428, -9.363379034771808662, -151.5937500020483810 ) ) ;
#16745=CARTESIAN_POINT ( 'NONE',  ( -9.999999999999998224, 1.224646799147353059E-15, -98.74999999999998579 ) ) ;
#16748=CARTESIAN_POINT ( 'NONE',  ( -5.000000000000003553, -8.660254037844383745, -4.375000004096768258 ) ) ;
#16749=CARTESIAN_POINT ( 'NONE',  ( -9.999999999999227285, -5.773502691896698735, -103.5000000040967336 ) ) ;
#16751=CARTESIAN_POINT ( 'NONE',  ( -10.81189881249999907, -6.242252689847864744, -121.9687500020483952 ) ) ;
#16753=CARTESIAN_POINT ( 'NONE',  ( 7.644554776091147741E-16, 12.48450537969573659, -91.15625000204838102 ) ) ;
#16754=CARTESIAN_POINT ( 'NONE',  ( 7.644554776091147741E-16, 12.48450537969573659, -107.4687500020483668 ) ) ;
#16755=( BOUNDED_CURVE ( )  B_SPLINE_CURVE ( 2, ( #20343, #31152, #7841, #14495, #20989, #27050, #34176 ),
 .UNSPECIFIED., .F., .F. ) 
 B_SPLINE_CURVE_WITH_KNOTS ( ( 3, 2, 2, 3 ),
 ( 0.7873134328358211143, 0.7885572139303484995, 0.7898009950248758848, 0.7910447761194031591 ),
 .UNSPECIFIED. ) 
 CURVE ( )  GEOMETRIC_REPRESENTATION_ITEM ( )  RATIONAL_B_SPLINE_CURVE ( ( 0.9999999999999761302, 0.8660254037844625774, 1.000000000000000000, 0.8660254037844387076, 1.000000000000000000, 0.8660254037844148378, 1.000000000000023981 ) ) 
 REPRESENTATION_ITEM ( '' )  );
#16758=CARTESIAN_POINT ( 'NONE',  ( 4.999999999999992006, -8.660254037844389075, -164.6250000040967905 ) ) ;
#16759=CARTESIAN_POINT ( 'NONE',  ( -9.999999999999998224, 1.224646799147353059E-15, -200.0000000000000000 ) ) ;
#16766=CARTESIAN_POINT ( 'NONE',  ( 5.000000000000000000, 8.660254037844385522, -78.24999999999998579 ) ) ;
#16768=CARTESIAN_POINT ( 'NONE',  ( 4.999999999999992006, -8.660254037844389075, -89.62500000409677625 ) ) ;
#16771=CARTESIAN_POINT ( 'NONE',  ( -5.405949406250003975, -9.363379034771801557, -84.53125000204838102 ) ) ;
#16774=CARTESIAN_POINT ( 'NONE',  ( 9.999999999998969713, 5.773502691896851502, -48.37499999999995026 ) ) ;
#16777=CARTESIAN_POINT ( 'NONE',  ( -4.999999999999996447, 8.660254037844387298, -7.499999999999978684 ) ) ;
#16778=CARTESIAN_POINT ( 'NONE',  ( -10.00000000000000000, -5.773502691896251982, -143.6250000000000000 ) ) ;
#16779=LINE ( 'NONE', #838, #31723 ) ;
#16781=CARTESIAN_POINT ( 'NONE',  ( -10.00000000000000000, -5.773502691896251982, -194.6250000000000284 ) ) ;
#16783=CARTESIAN_POINT ( 'NONE',  ( 10.81189881249999907, 6.242252689847868297, -119.9062500020483810 ) ) ;
#16784=ORIENTED_EDGE ( 'NONE', *, *, #8063, .T. ) ;
#16785=CARTESIAN_POINT ( 'NONE',  ( 5.000000000000000000, 8.660254037844385522, -23.12500000409675849 ) ) ;
#16786=VERTEX_POINT ( 'NONE', #29962 ) ;
#16787=( BOUNDED_CURVE ( )  B_SPLINE_CURVE ( 2, ( #6829, #30361, #29934, #10269, #26684, #26057, #30145 ),
 .UNSPECIFIED., .F., .F. ) 
 B_SPLINE_CURVE_WITH_KNOTS ( ( 3, 2, 2, 3 ),
 ( 0.4552238805970150737, 0.4564676616915424590, 0.4577114427860698442, 0.4589552238805971740 ),
 .UNSPECIFIED. ) 
 CURVE ( )  GEOMETRIC_REPRESENTATION_ITEM ( )  RATIONAL_B_SPLINE_CURVE ( ( 0.9999999999999820144, 0.8660254037844566932, 1.000000000000000000, 0.8660254037844387076, 1.000000000000000000, 0.8660254037844207220, 1.000000000000017986 ) ) 
 REPRESENTATION_ITEM ( '' )  );
#16788=CARTESIAN_POINT ( 'NONE',  ( 10.81189881249999551, -6.242252689847874514, -46.65625000204835970 ) ) ;
#16790=CARTESIAN_POINT ( 'NONE',  ( -10.81189881249999729, 1.324075727343319199E-15, -98.09375000204838102 ) ) ;
#16791=CARTESIAN_POINT ( 'NONE',  ( 10.81189881249999551, -6.242252689847874514, -126.1562500020483810 ) ) ;
#16792=ORIENTED_EDGE ( 'NONE', *, *, #6099, .F. ) ;
#16793=CARTESIAN_POINT ( 'NONE',  ( 10.00000000000076916, -5.773502691895816774, -111.6249999999999716 ) ) ;
#16798=CARTESIAN_POINT ( 'NONE',  ( -5.405949406250003975, -9.363379034771801557, -129.3437500020484094 ) ) ;
#16802=CARTESIAN_POINT ( 'NONE',  ( 5.000000000000000000, 8.660254037844385522, -185.1250000040967905 ) ) ;
#16804=CARTESIAN_POINT ( 'NONE',  ( -5.405949406249996869, 9.363379034771805109, -182.5312500020484094 ) ) ;
#16805=( BOUNDED_CURVE ( )  B_SPLINE_CURVE ( 2, ( #27946, #35068, #5495, #18645, #31839, #13729, #40076 ),
 .UNSPECIFIED., .F., .F. ) 
 B_SPLINE_CURVE_WITH_KNOTS ( ( 3, 2, 2, 3 ),
 ( 0.07462686567164185381, 0.07587064676616922521, 0.07711442786069658273, 0.07835820895522395413 ),
 .UNSPECIFIED. ) 
 CURVE ( )  GEOMETRIC_REPRESENTATION_ITEM ( )  RATIONAL_B_SPLINE_CURVE ( ( 0.9999999999999925615, 0.8660254037844461461, 1.000000000000000000, 0.8660254037844387076, 1.000000000000000000, 0.8660254037844312691, 1.000000000000007550 ) ) 
 REPRESENTATION_ITEM ( '' )  );
#16806=DIRECTION ( 'NONE',  ( 1.000000000000000000, 0.000000000000000000, 0.000000000000000000 ) ) ;
#16809=CARTESIAN_POINT ( 'NONE',  ( -5.405949406249996869, 9.363379034771805109, -56.34375000204835970 ) ) ;
#16810=CARTESIAN_POINT ( 'NONE',  ( -5.405949406250003975, -9.363379034771801557, -40.84375000204837391 ) ) ;
#16812=CARTESIAN_POINT ( 'NONE',  ( 5.405949406249999534, 9.363379034771803333, -22.28125000204836326 ) ) ;
#16814=CARTESIAN_POINT ( 'NONE',  ( 9.999999999999998224, 0.000000000000000000, -182.3750000040967905 ) ) ;
#16816=CARTESIAN_POINT ( 'NONE',  ( 9.999999999999996447, -5.773502691896262640, -108.6249999999999858 ) ) ;
#16818=CARTESIAN_POINT ( 'NONE',  ( 9.999999999999998224, 0.000000000000000000, -191.0000000000000000 ) ) ;
#16821=CARTESIAN_POINT ( 'NONE',  ( 5.405949406249992428, -9.363379034771808662, -105.2812500020483810 ) ) ;
#16822=EDGE_CURVE ( 'NONE', #3816, #3490, #40507, .T. ) ;
#16823=ORIENTED_EDGE ( 'NONE', *, *, #34660, .F. ) ;
#16824=LINE ( 'NONE', #6502, #32762 ) ;
#16828=EDGE_LOOP ( 'NONE', ( #25784, #9309, #24496, #13862, #19722, #21642, #19437, #30424, #5886, #9382, #12552, #9358, #24802, #4018, #3443, #26686, #20410, #6309, #10688, #33218, #8635, #25951, #31090, #16414, #17909, #37003, #39001, #18664, #11158, #29009, #25773, #7233, #11813, #35037, #42271, #11111, #25939, #33965, #35570, #6726, #27861, #40613, #36066, #40768, #13388, #7941, #38424, #40291, #26683, #15150, #27976, #30886, #2441, #34884, #31915, #9330, #29719, #40996, #5466, #19811, #12864, #12862, #17101, #24751, #17781, #19442, #31541, #10782, #38080, #29401, #29430, #28349, #31156, #31892, #3436, #29400, #21940, #4127, #29088, #33735, #17044, #9192, #29037, #42052, #34663, #6870, #34560, #37891, #7833, #4865, #36924, #30712, #37035, #29451, #19193, #38207, #5090, #16251, #15248, #3491, #35750, #3522, #6049, #8793, #6467, #39133, #9051, #1320, #13917, #10166, #28184, #10272, #37513, #15414, #21473, #28429, #21594, #34655, #42, #37081, #19611, #11635, #20462, #11442, #23977, #10111, #35334, #18992, #9166, #8426, #13119, #3645, #10002, #1219, #8862, #8060, #11001, #21207, #9477, #37293, #24579, #3438, #4851, #5869, #40728, #2005, #2397, #35569, #24427, #38944, #15132, #14179, #25222, #2607, #21725, #30119, #17805, #31527, #24414, #10239, #20463, #12685, #26111, #41322, #27693, #6152, #42015, #13263, #23427, #8046, #37946, #29028, #39260, #2809, #17528, #11484, #20378, #26476, #41840, #32276, #16243, #20352, #3327, #5245, #12843, #29125, #20565, #3331, #40620, #27971, #42586, #17321, #5822, #5995, #25536, #35623, #34931, #22793, #28134, #29238, #30021, #13649, #21239, #30341, #36969, #37355, #20200, #21273, #15185, #7193, #16682, #34642, #28348, #27257, #18210, #4551, #42171, #2863, #29976, #21211, #9747, #4988, #33478, #26354, #1218, #16737, #18064, #30834, #19602, #21483, #20302, #25013, #4443, #31373, #11091, #10268, #23237, #9064, #26952, #34723, #40885, #25175, #34826, #8732, #8705, #39715, #36857, #34510, #10328, #23132, #679, #18865, #8703, #26790, #2273, #37281, #40049, #8551, #25144, #21141, #25747, #5419, #14276, #10063, #6311, #23599, #37931, #42647, #29610, #24314 ) ) ;
#16829=CARTESIAN_POINT ( 'NONE',  ( 5.000000000000000000, 8.660254037844385522, -36.24999999999997868 ) ) ;
#16830=CARTESIAN_POINT ( 'NONE',  ( -2.121150477449813534E-15, -11.54700538379251284, -16.25000000409675849 ) ) ;
#16831=CARTESIAN_POINT ( 'NONE',  ( -10.81189881249999729, -6.242252689847864744, -45.65625000204837391 ) ) ;
#16834=CARTESIAN_POINT ( 'NONE',  ( -10.00000000000076916, 5.773502691895813221, -133.3749999999999716 ) ) ;
#16835=CARTESIAN_POINT ( 'NONE',  ( 7.644554776091147741E-16, 12.48450537969573659, -142.1562500020483810 ) ) ;
#16836=CARTESIAN_POINT ( 'NONE',  ( 10.00000000000154010, -5.773502691895370020, -15.62499999999993960 ) ) ;
#16837=ORIENTED_EDGE ( 'NONE', *, *, #23459, .F. ) ;
#16838=VERTEX_POINT ( 'NONE', #22845 ) ;
#16839=ADVANCED_FACE ( 'NONE', ( #36007 ), #39862, .T. ) ;
#16841=CARTESIAN_POINT ( 'NONE',  ( 7.070501591499376803E-16, 11.54700538379251284, -108.1249999999999858 ) ) ;
#16842=CARTESIAN_POINT ( 'NONE',  ( 9.999999999999998224, 0.000000000000000000, -200.0000000000000000 ) ) ;
#16843=CARTESIAN_POINT ( 'NONE',  ( -10.81189881249999729, 1.324075727343319199E-15, -171.5937500020484094 ) ) ;
#16846=CARTESIAN_POINT ( 'NONE',  ( 10.81189881249999551, -6.242252689847874514, -23.96875000204836681 ) ) ;
#16848=CARTESIAN_POINT ( 'NONE',  ( -8.660254037844442365, -15.00000000000010658, 49.99999999999998579 ) ) ;
#16849=CARTESIAN_POINT ( 'NONE',  ( -10.81189881249999729, 6.242252689847871849, -152.2187500020483810 ) ) ;
#16850=CARTESIAN_POINT ( 'NONE',  ( 10.81189881249999551, -6.242252689847874514, -133.4687500020483810 ) ) ;
#16851=CARTESIAN_POINT ( 'NONE',  ( -4.999999999999996447, 8.660254037844387298, -172.8750000040968189 ) ) ;
#16854=CARTESIAN_POINT ( 'NONE',  ( 5.405949406249999534, 9.363379034771803333, -11.59375000204834727 ) ) ;
#16857=DIRECTION ( 'NONE',  ( 1.000000000000000000, 0.000000000000000000, 0.000000000000000000 ) ) ;
#16859=CARTESIAN_POINT ( 'NONE',  ( -4.999999999999996447, 8.660254037844387298, -55.87500000409676204 ) ) ;
#16860=CARTESIAN_POINT ( 'NONE',  ( 10.81189881249999729, 0.000000000000000000, -86.84375000204836681 ) ) ;
#16861=CARTESIAN_POINT ( 'NONE',  ( -10.81189881249999729, 6.242252689847871849, -74.21875000204836681 ) ) ;
#16862=CARTESIAN_POINT ( 'NONE',  ( -10.81189881249999729, 6.242252689847871849, -39.90625000204835970 ) ) ;
#16864=CARTESIAN_POINT ( 'NONE',  ( -5.000000000000003553, -8.660254037844383745, -139.3750000040968189 ) ) ;
#16866=CARTESIAN_POINT ( 'NONE',  ( 5.000000000000000000, 8.660254037844385522, -132.2499999999999716 ) ) ;
#16867=CARTESIAN_POINT ( 'NONE',  ( 10.81189881249999729, 6.242252689847867408, -136.4062500020484094 ) ) ;
#16870=ORIENTED_EDGE ( 'NONE', *, *, #27900, .T. ) ;
#16874=CARTESIAN_POINT ( 'NONE',  ( 7.644554776091147741E-16, 12.48450537969573659, -167.6562500020483810 ) ) ;
#16875=CARTESIAN_POINT ( 'NONE',  ( -9.999999999999998224, 1.224646799147353059E-15, -43.62500000409677625 ) ) ;
#16878=FACE_OUTER_BOUND ( 'NONE', #7352, .T. ) ;
#16881=CARTESIAN_POINT ( 'NONE',  ( 7.070501591499376803E-16, 11.54700538379251284, -73.62499999999997158 ) ) ;
#16882=CARTESIAN_POINT ( 'NONE',  ( 10.81189881249999907, 6.242252689847868297, -158.9062500020483810 ) ) ;
#16883=CARTESIAN_POINT ( 'NONE',  ( 7.644554776091147741E-16, 12.48450537969573659, -137.4687500020483810 ) ) ;
#16884=LINE ( 'NONE', #16671, #11145 ) ;
#16885=CARTESIAN_POINT ( 'NONE',  ( -5.000000000000003553, -8.660254037844383745, -115.3750000040967905 ) ) ;
#16888=CARTESIAN_POINT ( 'NONE',  ( -2.293366432827344421E-15, -12.48450537969573659, -66.40625000204838102 ) ) ;
#16889=ORIENTED_EDGE ( 'NONE', *, *, #8533, .F. ) ;
#16891=CARTESIAN_POINT ( 'NONE',  ( -2.293366432827344421E-15, -12.48450537969573659, -115.7187500020483952 ) ) ;
#16892=ORIENTED_EDGE ( 'NONE', *, *, #19616, .T. ) ;
#16894=CARTESIAN_POINT ( 'NONE',  ( -10.81189881249999729, 6.242252689847871849, -23.21875000204835970 ) ) ;
#16895=CARTESIAN_POINT ( 'NONE',  ( 7.644554776091147741E-16, 12.48450537969573659, 0.3437499979516377424 ) ) ;
#16896=CARTESIAN_POINT ( 'NONE',  ( -5.405949406249996869, 9.363379034771805109, -47.34375000204838102 ) ) ;
#16897=FACE_OUTER_BOUND ( 'NONE', #2171, .T. ) ;
#16898=CARTESIAN_POINT ( 'NONE',  ( 9.999999999999998224, 0.000000000000000000, -192.8750000040967905 ) ) ;
#16899=CARTESIAN_POINT ( 'NONE',  ( -10.81189881249999729, 6.242252689847871849, -180.7187500020484379 ) ) ;
#16901=CARTESIAN_POINT ( 'NONE',  ( 5.405949406249999534, 9.363379034771803333, -170.5937500020484094 ) ) ;
#16905=CARTESIAN_POINT ( 'NONE',  ( 5.000000000000000000, 8.660254037844385522, -193.7500000000000000 ) ) ;
#16907=CARTESIAN_POINT ( 'NONE',  ( -2.293366432827344421E-15, -12.48450537969573659, -97.71875000204838102 ) ) ;
#16909=CARTESIAN_POINT ( 'NONE',  ( -5.405949406249996869, 9.363379034771805109, -62.53125000204837391 ) ) ;
#16910=CARTESIAN_POINT ( 'NONE',  ( 9.999999999999479527, 5.773502691896553074, -146.2500000040967905 ) ) ;
#16912=CARTESIAN_POINT ( 'NONE',  ( 10.81189881249999907, 6.242252689847868297, -125.9062500020483810 ) ) ;
#16913=CARTESIAN_POINT ( 'NONE',  ( 10.81189881249999729, 0.000000000000000000, -163.5312500020484094 ) ) ;
#16915=CARTESIAN_POINT ( 'NONE',  ( -9.999999999999998224, 1.224646799147353059E-15, -135.1250000040967620 ) ) ;
#16917=( BOUNDED_CURVE ( )  B_SPLINE_CURVE ( 2, ( #34248, #7909, #21057, #7475, #20626, #11338, #13924 ),
 .UNSPECIFIED., .F., .F. ) 
 B_SPLINE_CURVE_WITH_KNOTS ( ( 3, 2, 2, 3 ),
 ( 0.5298507462686568026, 0.5310945273631841879, 0.5323383084577115731, 0.5335820895522389584 ),
 .UNSPECIFIED. ) 
 CURVE ( )  GEOMETRIC_REPRESENTATION_ITEM ( )  RATIONAL_B_SPLINE_CURVE ( ( 0.9999999999999880096, 0.8660254037844506980, 1.000000000000000000, 0.8660254037844387076, 1.000000000000000000, 0.8660254037844267172, 1.000000000000011990 ) ) 
 REPRESENTATION_ITEM ( '' )  );
#16918=VERTEX_POINT ( 'NONE', #32569 ) ;
#16921=CARTESIAN_POINT ( 'NONE',  ( 10.81189881249999551, -6.242252689847874514, -190.6562500020484094 ) ) ;
#16924=ORIENTED_EDGE ( 'NONE', *, *, #32791, .T. ) ;
#16925=CARTESIAN_POINT ( 'NONE',  ( 10.00000000000000000, 5.773502691896255534, -54.37499999999997158 ) ) ;
#16927=CARTESIAN_POINT ( 'NONE',  ( -2.121150477449813534E-15, -11.54700538379251284, -68.75000000409679046 ) ) ;
#16928=ADVANCED_FACE ( 'NONE', ( #30175 ), #23055, .T. ) ;
#16929=CARTESIAN_POINT ( 'NONE',  ( 10.00000000000051159, -5.773502691895965988, -109.0000000040967620 ) ) ;
#16931=EDGE_CURVE ( 'NONE', #4387, #36434, #25871, .T. ) ;
#16933=VECTOR ( 'NONE', #41787, 1000.000000000000000 ) ;
#16934=CARTESIAN_POINT ( 'NONE',  ( 10.81189881249999729, 6.242252689847867408, -59.90625000204838813 ) ) ;
#16938=CARTESIAN_POINT ( 'NONE',  ( -5.000000000000003553, -8.660254037844383745, -151.3750000040967905 ) ) ;
#16939=CARTESIAN_POINT ( 'NONE',  ( 7.644554776091147741E-16, 12.48450537969573659, -182.6562500020484094 ) ) ;
#16941=CARTESIAN_POINT ( 'NONE',  ( 9.999999999999998224, 0.000000000000000000, -102.8750000040967763 ) ) ;
#16942=DIRECTION ( 'NONE',  ( -0.000000000000000000, -0.000000000000000000, 1.000000000000000000 ) ) ;
#16944=DIRECTION ( 'NONE',  ( -0.000000000000000000, -0.000000000000000000, 1.000000000000000000 ) ) ;
#16945=CARTESIAN_POINT ( 'NONE',  ( 10.81189881249999551, -6.242252689847874514, -93.15625000204838102 ) ) ;
#16946=EDGE_LOOP ( 'NONE', ( #10356, #17428, #21856, #20174 ) ) ;
#16947=CARTESIAN_POINT ( 'NONE',  ( 7.070501591499376803E-16, 11.54700538379251284, -24.50000000409676559 ) ) ;
#16948=EDGE_CURVE ( 'NONE', #4388, #28982, #34503, .T. ) ;
#16952=CARTESIAN_POINT ( 'NONE',  ( 10.81189881249999907, 6.242252689847868297, -37.21875000204835970 ) ) ;
#16953=CARTESIAN_POINT ( 'NONE',  ( 10.81189881249999729, 0.000000000000000000, -22.53125000204836326 ) ) ;
#16956=CARTESIAN_POINT ( 'NONE',  ( -5.405949406250003975, -9.363379034771801557, -72.34375000204836681 ) ) ;
#16957=CARTESIAN_POINT ( 'NONE',  ( -5.000000000000003553, -8.660254037844383745, -17.87500000409675138 ) ) ;
#16959=EDGE_CURVE ( 'NONE', #10102, #23552, #34428, .T. ) ;
#16960=CARTESIAN_POINT ( 'NONE',  ( 10.81189881249999551, -6.242252689847874514, -193.4687500020484094 ) ) ;
#16961=CARTESIAN_POINT ( 'NONE',  ( 5.405949406249992428, -9.363379034771808662, -148.5937500020483810 ) ) ;
#16962=AXIS2_PLACEMENT_3D ( 'NONE', #5838, #6051, #29350 ) ;
#16966=CARTESIAN_POINT ( 'NONE',  ( 10.00000000000000000, 5.773502691896255534, -5.250000004096769146 ) ) ;
#16967=CARTESIAN_POINT ( 'NONE',  ( 4.999999999999992006, -8.660254037844389075, -125.2500000000000000 ) ) ;
#16968=CARTESIAN_POINT ( 'NONE',  ( -10.81189881249999729, 1.324075727343319199E-15, -125.0937500020483668 ) ) ;
#16969=CARTESIAN_POINT ( 'NONE',  ( 7.070501591499376803E-16, 11.54700538379251284, -109.6249999999999858 ) ) ;
#16970=CARTESIAN_POINT ( 'NONE',  ( 5.405949406249992428, -9.363379034771808662, -88.78125000204838102 ) ) ;
#16971=CARTESIAN_POINT ( 'NONE',  ( -5.405949406249996869, 9.363379034771805109, -96.84375000204838102 ) ) ;
#16974=CARTESIAN_POINT ( 'NONE',  ( 5.000000000000000000, 8.660254037844385522, -158.1250000040967905 ) ) ;
#16978=CARTESIAN_POINT ( 'NONE',  ( -9.999999999999998224, 1.224646799147353059E-15, -37.24999999999997868 ) ) ;
#16979=CARTESIAN_POINT ( 'NONE',  ( -2.121150477449813534E-15, -11.54700538379251284, -53.75000000409677625 ) ) ;
#16981=CARTESIAN_POINT ( 'NONE',  ( 7.070501591499377789E-16, 11.54700538379251284, -84.12499999999997158 ) ) ;
#16983=CARTESIAN_POINT ( 'NONE',  ( -10.00000000000000000, -5.773502691896251982, -93.00000000409679046 ) ) ;
#16984=CARTESIAN_POINT ( 'NONE',  ( -5.000000000000003553, -8.660254037844383745, -95.87500000409677625 ) ) ;
#16986=CARTESIAN_POINT ( 'NONE',  ( 5.405949406249999534, 9.363379034771803333, -80.78125000204838102 ) ) ;
#16987=ORIENTED_EDGE ( 'NONE', *, *, #9860, .F. ) ;
#16988=EDGE_CURVE ( 'NONE', #24317, #25484, #5277, .T. ) ;
#16990=DIRECTION ( 'NONE',  ( -0.000000000000000000, -0.000000000000000000, 1.000000000000000000 ) ) ;
#16992=ORIENTED_EDGE ( 'NONE', *, *, #37881, .T. ) ;
#16993=CARTESIAN_POINT ( 'NONE',  ( 5.000000000000000000, 8.660254037844385522, -9.249999999999952038 ) ) ;
#16996=CARTESIAN_POINT ( 'NONE',  ( 10.00000000000000000, 5.773502691896255534, -148.8750000000000000 ) ) ;
#16999=CARTESIAN_POINT ( 'NONE',  ( 9.999999999999996447, -5.773502691896262640, -191.1250000000000000 ) ) ;
#17001=CARTESIAN_POINT ( 'NONE',  ( 5.405949406249999534, 9.363379034771803333, -121.2812500020483952 ) ) ;
#17002=EDGE_LOOP ( 'NONE', ( #38369, #14606, #39248, #37128 ) ) ;
#17004=DIRECTION ( 'NONE',  ( -0.000000000000000000, -0.000000000000000000, 1.000000000000000000 ) ) ;
#17005=VERTEX_POINT ( 'NONE', #11306 ) ;
#17006=ORIENTED_EDGE ( 'NONE', *, *, #19564, .T. ) ;
#17008=CARTESIAN_POINT ( 'NONE',  ( -10.81189881249999907, -6.242252689847864744, -47.15625000204836681 ) ) ;
#17010=CARTESIAN_POINT ( 'NONE',  ( 5.405949406249999534, 9.363379034771803333, -98.59375000204838102 ) ) ;
#17011=CARTESIAN_POINT ( 'NONE',  ( 5.405949406249992428, -9.363379034771808662, -124.7812500020483952 ) ) ;
#17012=ORIENTED_EDGE ( 'NONE', *, *, #27056, .T. ) ;
#17013=CARTESIAN_POINT ( 'NONE',  ( 0.000000000000000000, 0.000000000000000000, -200.0000000000000000 ) ) ;
#17014=CARTESIAN_POINT ( 'NONE',  ( 10.81189881249999729, 0.000000000000000000, -197.8437500020484094 ) ) ;
#17016=DIRECTION ( 'NONE',  ( -0.000000000000000000, -0.000000000000000000, 1.000000000000000000 ) ) ;
#17017=CARTESIAN_POINT ( 'NONE',  ( 5.405949406249999534, 9.363379034771803333, -136.0937500020483810 ) ) ;
#17020=CARTESIAN_POINT ( 'NONE',  ( 9.999999999999998224, 0.000000000000000000, -189.8750000040967905 ) ) ;
#17022=CARTESIAN_POINT ( 'NONE',  ( -10.81189881249999729, 1.324075727343319199E-15, -179.2812500020484094 ) ) ;
#17026=CARTESIAN_POINT ( 'NONE',  ( 5.405949406249992428, -9.363379034771808662, -60.09375000204835970 ) ) ;
#17027=CARTESIAN_POINT ( 'NONE',  ( -10.81189881249999729, 1.324075727343319199E-15, -44.09375000204837391 ) ) ;
#17029=CARTESIAN_POINT ( 'NONE',  ( 10.81189881249999729, 0.000000000000000000, -16.53125000204835970 ) ) ;
#17031=DIRECTION ( 'NONE',  ( -0.000000000000000000, -0.000000000000000000, 1.000000000000000000 ) ) ;
#17033=CARTESIAN_POINT ( 'NONE',  ( -5.000000000000003553, -8.660254037844383745, -105.9999999999999858 ) ) ;
#17035=CARTESIAN_POINT ( 'NONE',  ( -9.999999999999998224, 1.224646799147353059E-15, -198.1250000040967905 ) ) ;
#17038=CARTESIAN_POINT ( 'NONE',  ( -5.405949406249996869, 9.363379034771805109, -110.5312500020483810 ) ) ;
#17039=ORIENTED_EDGE ( 'NONE', *, *, #41692, .F. ) ;
#17040=DIRECTION ( 'NONE',  ( -0.000000000000000000, -0.000000000000000000, 1.000000000000000000 ) ) ;
#17044=ORIENTED_EDGE ( 'NONE', *, *, #5029, .T. ) ;
#17045=CARTESIAN_POINT ( 'NONE',  ( 5.000000000000000000, 8.660254037844385522, -31.74999999999997158 ) ) ;
#17046=CARTESIAN_POINT ( 'NONE',  ( 5.405949406249999534, 9.363379034771803333, -34.28125000204837391 ) ) ;
#17049=( BOUNDED_CURVE ( )  B_SPLINE_CURVE ( 2, ( #17799, #2071, #27964, #4439, #30779, #11752, #34236 ),
 .UNSPECIFIED., .F., .F. ) 
 B_SPLINE_CURVE_WITH_KNOTS ( ( 3, 2, 2, 3 ),
 ( 0.7910447761194031591, 0.7922885572139305443, 0.7935323383084578186, 0.7947761194029852039 ),
 .UNSPECIFIED. ) 
 CURVE ( )  GEOMETRIC_REPRESENTATION_ITEM ( )  RATIONAL_B_SPLINE_CURVE ( ( 0.9999999999999761302, 0.8660254037844625774, 1.000000000000000000, 0.8660254037844387076, 1.000000000000000000, 0.8660254037844267172, 1.000000000000011990 ) ) 
 REPRESENTATION_ITEM ( '' )  );
#17051=EDGE_CURVE ( 'NONE', #4845, #437, #590, .T. ) ;
#17052=CARTESIAN_POINT ( 'NONE',  ( 10.81189881249999729, 0.000000000000000000, -141.0312500020483810 ) ) ;
#17056=EDGE_LOOP ( 'NONE', ( #29332, #21029, #23401, #30190 ) ) ;
#17057=CARTESIAN_POINT ( 'NONE',  ( -5.000000000000003553, -8.660254037844383745, -106.3750000040967763 ) ) ;
#17058=ADVANCED_FACE ( 'NONE', ( #11518 ), #14965, .T. ) ;
#17059=DIRECTION ( 'NONE',  ( -0.000000000000000000, -0.000000000000000000, 1.000000000000000000 ) ) ;
#17060=CARTESIAN_POINT ( 'NONE',  ( 5.405949406249992428, -9.363379034771808662, -165.0937500020484094 ) ) ;
#17062=CARTESIAN_POINT ( 'NONE',  ( 10.81189881249999729, 0.000000000000000000, -23.84375000204835970 ) ) ;
#17063=CARTESIAN_POINT ( 'NONE',  ( 9.999999999999998224, 0.000000000000000000, -171.5000000000000000 ) ) ;
#17064=CARTESIAN_POINT ( 'NONE',  ( -10.81189881249999729, 1.324075727343319199E-15, -159.5937500020484094 ) ) ;
#17065=AXIS2_PLACEMENT_3D ( 'NONE', #323, #6369, #26847 ) ;
#17066=CARTESIAN_POINT ( 'NONE',  ( 5.405949406249992428, -9.363379034771808662, -139.5937500020483810 ) ) ;
#17071=CARTESIAN_POINT ( 'NONE',  ( 10.81189881249999551, -6.242252689847874514, -13.46875000204836503 ) ) ;
#17073=CARTESIAN_POINT ( 'NONE',  ( -4.999999999999996447, 8.660254037844387298, -63.37500000409676204 ) ) ;
#17074=CARTESIAN_POINT ( 'NONE',  ( -9.999999999999998224, 1.224646799147353059E-15, -4.625000004096769146 ) ) ;
#17077=CARTESIAN_POINT ( 'NONE',  ( -2.293366432827344421E-15, -12.48450537969573659, -85.71875000204838102 ) ) ;
#17078=CARTESIAN_POINT ( 'NONE',  ( -10.81189881249999729, 6.242252689847871849, -66.71875000204838102 ) ) ;
#17079=CARTESIAN_POINT ( 'NONE',  ( -10.81189881249999729, 1.324075727343319199E-15, -39.78125000204838102 ) ) ;
#17083=CARTESIAN_POINT ( 'NONE',  ( -5.000000000000003553, -8.660254037844383745, -133.0000000000000000 ) ) ;
#17084=CARTESIAN_POINT ( 'NONE',  ( -10.81189881249999729, 6.242252689847871849, -138.9062500020484094 ) ) ;
#17087=CARTESIAN_POINT ( 'NONE',  ( -10.81189881249999729, -6.242252689847864744, -21.65625000204837036 ) ) ;
#17088=ORIENTED_EDGE ( 'NONE', *, *, #34606, .T. ) ;
#17091=CARTESIAN_POINT ( 'NONE',  ( -9.999999999999678479, -5.773502691896439387, -185.6250000000000000 ) ) ;
#17092=CARTESIAN_POINT ( 'NONE',  ( -2.121150477449813534E-15, -11.54700538379251284, -38.75000000409676915 ) ) ;
#17093=CARTESIAN_POINT ( 'NONE',  ( -9.999999999999998224, 1.224646799147353059E-15, -106.2499999999999858 ) ) ;
#17095=EDGE_CURVE ( 'NONE', #25691, #38243, #31475, .T. ) ;
#17097=CARTESIAN_POINT ( 'NONE',  ( 10.81189881249999729, 0.000000000000000000, -150.0312500020483810 ) ) ;
#17098=CARTESIAN_POINT ( 'NONE',  ( 10.81189881249999907, 6.242252689847868297, -133.2187500020483810 ) ) ;
#17099=CARTESIAN_POINT ( 'NONE',  ( -9.999999999999998224, 1.224646799147353059E-15, -10.62500000409674605 ) ) ;
#17101=ORIENTED_EDGE ( 'NONE', *, *, #13277, .T. ) ;
#17103=CARTESIAN_POINT ( 'NONE',  ( 9.999999999999998224, 0.000000000000000000, -200.0000000000000000 ) ) ;
#17104=CARTESIAN_POINT ( 'NONE',  ( -10.81189881249999729, 1.324075727343319199E-15, -63.78125000204837391 ) ) ;
#17105=EDGE_LOOP ( 'NONE', ( #10875, #14828, #33785, #24097 ) ) ;
#17107=CARTESIAN_POINT ( 'NONE',  ( 5.405949406249999534, 9.363379034771803333, -112.0937500020483810 ) ) ;
#17108=ORIENTED_EDGE ( 'NONE', *, *, #30704, .T. ) ;
#17109=EDGE_CURVE ( 'NONE', #6874, #32468, #11951, .T. ) ;
#17110=CARTESIAN_POINT ( 'NONE',  ( 5.405949406249999534, 9.363379034771803333, -22.09375000204835615 ) ) ;
#17111=CARTESIAN_POINT ( 'NONE',  ( -10.81189881249999729, 6.242252689847871849, -188.2187500020483810 ) ) ;
#17112=CARTESIAN_POINT ( 'NONE',  ( -10.81189881249999729, 1.324075727343319199E-15, -47.09375000204838102 ) ) ;
#17113=CARTESIAN_POINT ( 'NONE',  ( 5.000000000000000000, 8.660254037844385522, -62.12500000409676204 ) ) ;
#17114=CARTESIAN_POINT ( 'NONE',  ( -9.999999999999479527, -5.773502691896549521, -31.50000000409673717 ) ) ;
#17115=CARTESIAN_POINT ( 'NONE',  ( -2.293366432827344421E-15, -12.48450537969573659, -181.7187500020484094 ) ) ;
#17116=CARTESIAN_POINT ( 'NONE',  ( -10.81189881249999729, 1.324075727343319199E-15, -159.5937500020484094 ) ) ;
#17119=CARTESIAN_POINT ( 'NONE',  ( 4.999999999999992006, -8.660254037844389075, -104.6250000040967763 ) ) ;
#17120=FACE_OUTER_BOUND ( 'NONE', #26107, .T. ) ;
#17122=CARTESIAN_POINT ( 'NONE',  ( 10.81189881249999729, 0.000000000000000000, -85.34375000204836681 ) ) ;
#17123=CARTESIAN_POINT ( 'NONE',  ( -9.999999999999742428, -5.773502691896402084, -101.6249999999999716 ) ) ;
#17124=CARTESIAN_POINT ( 'NONE',  ( -5.405949406249996869, 9.363379034771805109, -67.03125000204838102 ) ) ;
#17125=CARTESIAN_POINT ( 'NONE',  ( 9.999999999999998224, 0.000000000000000000, -200.0000000000000000 ) ) ;
#17127=CARTESIAN_POINT ( 'NONE',  ( 10.81189881249999907, 6.242252689847868297, -122.9062500020484094 ) ) ;
#17128=AXIS2_PLACEMENT_3D ( 'NONE', #5169, #18323, #26085 ) ;
#17129=CARTESIAN_POINT ( 'NONE',  ( 10.81189881249999551, -6.242252689847874514, -165.1562500020483526 ) ) ;
#17130=( BOUNDED_CURVE ( )  B_SPLINE_CURVE ( 2, ( #38813, #6016, #6230, #32142, #32564, #25452, #38597 ),
 .UNSPECIFIED., .F., .F. ) 
 B_SPLINE_CURVE_WITH_KNOTS ( ( 3, 2, 2, 3 ),
 ( 0.3246268656716419510, 0.3258706467661692807, 0.3271144278606965550, 0.3283582089552238847 ),
 .UNSPECIFIED. ) 
 CURVE ( )  GEOMETRIC_REPRESENTATION_ITEM ( )  RATIONAL_B_SPLINE_CURVE ( ( 0.9999999999999820144, 0.8660254037844566932, 1.000000000000000000, 0.8660254037844387076, 1.000000000000000000, 0.8660254037844387076, 1.000000000000000000 ) ) 
 REPRESENTATION_ITEM ( '' )  );
#17132=CARTESIAN_POINT ( 'NONE',  ( -2.121150477449813534E-15, -11.54700538379251284, -137.7500000040967905 ) ) ;
#17134=ORIENTED_EDGE ( 'NONE', *, *, #11456, .F. ) ;
#17137=AXIS2_PLACEMENT_3D ( 'NONE', #24345, #8365, #1247 ) ;
#17138=CARTESIAN_POINT ( 'NONE',  ( -10.81189881249999729, 1.324075727343319199E-15, -189.7812500020484094 ) ) ;
#17141=CARTESIAN_POINT ( 'NONE',  ( -5.000000000000003553, -8.660254037844383745, -50.49999999999998579 ) ) ;
#17143=CARTESIAN_POINT ( 'NONE',  ( -10.00000000000000000, -5.773502691896251982, -63.00000000409679757 ) ) ;
#17145=CARTESIAN_POINT ( 'NONE',  ( -10.00000000000000000, -5.773502691896252870, -166.1249999999999716 ) ) ;
#17147=CARTESIAN_POINT ( 'NONE',  ( -5.405949406249996869, 9.363379034771805109, -62.53125000204837391 ) ) ;
#17150=CARTESIAN_POINT ( 'NONE',  ( 4.999999999999992006, -8.660254037844389075, -35.24999999999997868 ) ) ;
#17151=CARTESIAN_POINT ( 'NONE',  ( -10.81189881249999907, -6.242252689847864744, -180.6562500020484094 ) ) ;
#17153=CARTESIAN_POINT ( 'NONE',  ( 9.999999999999998224, 0.000000000000000000, -147.8750000040967905 ) ) ;
#17157=CARTESIAN_POINT ( 'NONE',  ( 0.000000000000000000, 0.000000000000000000, -200.0000000000000000 ) ) ;
#17158=CARTESIAN_POINT ( 'NONE',  ( -10.81189881249999907, -6.242252689847864744, -89.15625000204839523 ) ) ;
#17159=EDGE_LOOP ( 'NONE', ( #9728, #1272, #18401, #31260 ) ) ;
#17160=DIRECTION ( 'NONE',  ( -0.000000000000000000, -0.000000000000000000, 1.000000000000000000 ) ) ;
#17161=CARTESIAN_POINT ( 'NONE',  ( 9.999999999999998224, 0.000000000000000000, -162.5000000000000000 ) ) ;
#17164=CARTESIAN_POINT ( 'NONE',  ( 5.405949406249999534, 9.363379034771803333, -28.09375000204836326 ) ) ;
#17165=CARTESIAN_POINT ( 'NONE',  ( 7.644554776091147741E-16, 12.48450537969573659, -19.15625000204837391 ) ) ;
#17166=VECTOR ( 'NONE', #33112, 1000.000000000000000 ) ;
#17167=CARTESIAN_POINT ( 'NONE',  ( -10.81189881249999907, -6.242252689847864744, -67.96875000204838102 ) ) ;
#17169=EDGE_CURVE ( 'NONE', #11948, #933, #8735, .T. ) ;
#17171=CARTESIAN_POINT ( 'NONE',  ( -10.81189881249999729, 1.324075727343319199E-15, -182.0937500020483810 ) ) ;
#17172=EDGE_CURVE ( 'NONE', #1841, #22659, #16805, .T. ) ;
#17173=( BOUNDED_CURVE ( )  B_SPLINE_CURVE ( 2, ( #13605, #34941, #41163, #37737, #21550, #21112, #26799 ),
 .UNSPECIFIED., .F., .F. ) 
 B_SPLINE_CURVE_WITH_KNOTS ( ( 3, 2, 2, 3 ),
 ( 0.3805970149253732338, 0.3818407960199006190, 0.3830845771144278933, 0.3843283582089552786 ),
 .UNSPECIFIED. ) 
 CURVE ( )  GEOMETRIC_REPRESENTATION_ITEM ( )  RATIONAL_B_SPLINE_CURVE ( ( 0.9999999999999880096, 0.8660254037844506980, 1.000000000000000000, 0.8660254037844387076, 1.000000000000000000, 0.8660254037844327124, 1.000000000000005995 ) ) 
 REPRESENTATION_ITEM ( '' )  );
#17174=CARTESIAN_POINT ( 'NONE',  ( 10.81189881249999907, 6.242252689847868297, -2.718750002048360592 ) ) ;
#17176=VECTOR ( 'NONE', #42354, 1000.000000000000000 ) ;
#17177=LINE ( 'NONE', #6427, #16382 ) ;
#17178=CARTESIAN_POINT ( 'NONE',  ( -9.999999999999998224, 1.224646799147353059E-15, -3.125000004096767370 ) ) ;
#17180=CARTESIAN_POINT ( 'NONE',  ( -5.405949406250003975, -9.363379034771801557, -120.3437500020483952 ) ) ;
#17181=CARTESIAN_POINT ( 'NONE',  ( -4.999999999999996447, 8.660254037844387298, -109.4999999999999858 ) ) ;
#17182=CARTESIAN_POINT ( 'NONE',  ( 5.405949406249999534, 9.363379034771803333, -86.78125000204838102 ) ) ;
#17183=CARTESIAN_POINT ( 'NONE',  ( -10.81189881249999729, 1.324075727343319199E-15, -98.09375000204838102 ) ) ;
#17186=CARTESIAN_POINT ( 'NONE',  ( 10.00000000000000000, 5.773502691896255534, -162.7500000040967905 ) ) ;
#17193=CARTESIAN_POINT ( 'NONE',  ( -4.999999999999996447, 8.660254037844387298, -70.49999999999998579 ) ) ;
#17195=CARTESIAN_POINT ( 'NONE',  ( 10.00000000000000000, 5.773502691896255534, -90.75000000409677625 ) ) ;
#17197=CARTESIAN_POINT ( 'NONE',  ( -2.293366432827344421E-15, -12.48450537969573659, -82.90625000204838102 ) ) ;
#17199=CARTESIAN_POINT ( 'NONE',  ( -10.00000000000154188, 5.773502691895366468, -20.87499999999993250 ) ) ;
#17202=CARTESIAN_POINT ( 'NONE',  ( 7.070501591499377789E-16, 11.54700538379251284, -7.624999999999972466 ) ) ;
#17204=CARTESIAN_POINT ( 'NONE',  ( 4.999999999999992006, -8.660254037844389075, -143.2500000000000000 ) ) ;
#17205=CARTESIAN_POINT ( 'NONE',  ( 4.999999999999992006, -8.660254037844389075, -14.62500000409674961 ) ) ;
#17207=CARTESIAN_POINT ( 'NONE',  ( -2.293366432827344421E-15, -12.48450537969573659, -135.4062500020483810 ) ) ;
#17208=CARTESIAN_POINT ( 'NONE',  ( -4.999999999999996447, 8.660254037844387298, -193.5000000000000000 ) ) ;
#17209=CARTESIAN_POINT ( 'NONE',  ( 0.000000000000000000, 0.000000000000000000, -200.0000000000000000 ) ) ;
#17210=CARTESIAN_POINT ( 'NONE',  ( 7.644554776091147741E-16, 12.48450537969573659, -121.1562500020483952 ) ) ;
#17211=ORIENTED_EDGE ( 'NONE', *, *, #30964, .T. ) ;
#17212=FACE_OUTER_BOUND ( 'NONE', #22971, .T. ) ;
#17215=CARTESIAN_POINT ( 'NONE',  ( 7.644554776091147741E-16, 12.48450537969573659, -46.15625000204837391 ) ) ;
#17217=CARTESIAN_POINT ( 'NONE',  ( 5.405949406249992428, -9.363379034771808662, -96.09375000204838102 ) ) ;
#17218=CARTESIAN_POINT ( 'NONE',  ( -5.405949406250003975, -9.363379034771801557, -123.5312500020483952 ) ) ;
#17221=CARTESIAN_POINT ( 'NONE',  ( -8.667397162551022660, -4.987630568095290151, -0.0003570992120843448142 ) ) ;
#17222=DIRECTION ( 'NONE',  ( 1.000000000000000000, 0.000000000000000000, 0.000000000000000000 ) ) ;
#17223=EDGE_CURVE ( 'NONE', #26104, #37116, #17952, .T. ) ;
#17225=DIRECTION ( 'NONE',  ( -0.000000000000000000, -0.000000000000000000, 1.000000000000000000 ) ) ;
#17228=CARTESIAN_POINT ( 'NONE',  ( -10.81189881249999729, 6.242252689847871849, -125.2187500020483810 ) ) ;
#17233=CARTESIAN_POINT ( 'NONE',  ( -4.999999999999996447, 8.660254037844387298, -187.8750000040967905 ) ) ;
#17235=CARTESIAN_POINT ( 'NONE',  ( -10.81189881249999729, 6.242252689847871849, -177.9062500020484094 ) ) ;
#17239=CARTESIAN_POINT ( 'NONE',  ( 5.405949406249999534, 9.363379034771803333, -52.09375000204835260 ) ) ;
#17240=CARTESIAN_POINT ( 'NONE',  ( -10.81189881249999729, 1.324075727343319199E-15, -42.59375000204837391 ) ) ;
#17242=CARTESIAN_POINT ( 'NONE',  ( -2.293366432827344421E-15, -12.48450537969573659, -9.406250002048375691 ) ) ;
#17246=CARTESIAN_POINT ( 'NONE',  ( -9.999999999999998224, 1.224646799147353059E-15, -103.2500000000000000 ) ) ;
#17248=CARTESIAN_POINT ( 'NONE',  ( 9.999999999999998224, 0.000000000000000000, -4.999999999999976907 ) ) ;
#17251=CARTESIAN_POINT ( 'NONE',  ( 5.405949406249999534, 9.363379034771803333, -106.2812500020483810 ) ) ;
#17255=CARTESIAN_POINT ( 'NONE',  ( 0.000000000000000000, 0.000000000000000000, -200.0000000000000000 ) ) ;
#17258=CARTESIAN_POINT ( 'NONE',  ( -10.00000000000000000, -5.773502691896251982, -32.62499999999995737 ) ) ;
#17259=CARTESIAN_POINT ( 'NONE',  ( -2.293366432827344421E-15, -12.48450537969573659, -36.40625000204835970 ) ) ;
#17260=CARTESIAN_POINT ( 'NONE',  ( -9.999999999999479527, -5.773502691896549521, -91.12499999999995737 ) ) ;
#17262=CARTESIAN_POINT ( 'NONE',  ( 9.999999999999998224, 0.000000000000000000, -12.49999999999995559 ) ) ;
#17264=CARTESIAN_POINT ( 'NONE',  ( -2.293366432827344421E-15, -12.48450537969573659, -139.9062500020484094 ) ) ;
#17265=AXIS2_PLACEMENT_3D ( 'NONE', #31801, #38042, #14713 ) ;
#17269=CARTESIAN_POINT ( 'NONE',  ( -4.999999999999996447, 8.660254037844387298, -113.9999999999999858 ) ) ;
#17270=DIRECTION ( 'NONE',  ( -1.062296840242595709E-16, 0.7071067811865493491, 0.7071067811865456854 ) ) ;
#17271=CARTESIAN_POINT ( 'NONE',  ( -2.293366432827344421E-15, -12.48450537969573659, -169.7187500020483810 ) ) ;
#17273=CARTESIAN_POINT ( 'NONE',  ( -10.81189881249999729, 6.242252689847871849, -18.71875000204837391 ) ) ;
#17274=CARTESIAN_POINT ( 'NONE',  ( 10.00000000000025402, -5.773502691896113426, -157.0000000040968189 ) ) ;
#17275=CARTESIAN_POINT ( 'NONE',  ( -10.81189881249999729, 1.324075727343319199E-15, -144.5937500020483810 ) ) ;
#17276=CARTESIAN_POINT ( 'NONE',  ( 10.81189881249999729, 0.000000000000000000, -134.8437500020484094 ) ) ;
#17277=CARTESIAN_POINT ( 'NONE',  ( -5.405949406249996869, 9.363379034771805109, -104.5312500020483810 ) ) ;
#17281=CARTESIAN_POINT ( 'NONE',  ( -10.81189881249999729, 6.242252689847871849, -9.718750002048363257 ) ) ;
#17285=CARTESIAN_POINT ( 'NONE',  ( -9.999999999999998224, 1.224646799147353059E-15, -70.62500000409677625 ) ) ;
#17289=ADVANCED_FACE ( 'NONE', ( #35909 ), #38721, .T. ) ;
#17290=CARTESIAN_POINT ( 'NONE',  ( 10.81189881249999729, 6.242252689847867408, -80.71875000204838102 ) ) ;
#17291=CARTESIAN_POINT ( 'NONE',  ( -5.405949406249996869, 9.363379034771805109, -65.34375000204836681 ) ) ;
#17293=CARTESIAN_POINT ( 'NONE',  ( 10.81189881249999551, -6.242252689847874514, -39.15625000204835260 ) ) ;
#17296=CARTESIAN_POINT ( 'NONE',  ( -2.121150477449813534E-15, -11.54700538379251284, -129.8750000000000000 ) ) ;
#17297=CARTESIAN_POINT ( 'NONE',  ( 5.405949406249992428, -9.363379034771808662, -132.2812500020483810 ) ) ;
#17298=CARTESIAN_POINT ( 'NONE',  ( 10.00000000000102318, -5.773502691895667560, -67.00000000409674783 ) ) ;
#17300=CARTESIAN_POINT ( 'NONE',  ( -10.81189881249999729, 1.324075727343319199E-15, -21.78125000204836326 ) ) ;
#17302=ORIENTED_EDGE ( 'NONE', *, *, #1806, .T. ) ;
#17306=CARTESIAN_POINT ( 'NONE',  ( -4.999999999999996447, 8.660254037844387298, -37.87500000409676915 ) ) ;
#17308=DIRECTION ( 'NONE',  ( -0.000000000000000000, -0.000000000000000000, 1.000000000000000000 ) ) ;
#17310=CARTESIAN_POINT ( 'NONE',  ( -2.121150477449813534E-15, -11.54700538379251284, -146.3749999999999716 ) ) ;
#17311=CARTESIAN_POINT ( 'NONE',  ( 10.81189881249999729, 0.000000000000000000, -154.5312500020484094 ) ) ;
#17312=CARTESIAN_POINT ( 'NONE',  ( 10.81189881249999729, 0.000000000000000000, -131.8437500020484094 ) ) ;
#17314=EDGE_LOOP ( 'NONE', ( #3423, #29448, #28610, #4496 ) ) ;
#17315=DIRECTION ( 'NONE',  ( -0.000000000000000000, -0.000000000000000000, 1.000000000000000000 ) ) ;
#17316=ORIENTED_EDGE ( 'NONE', *, *, #29405, .T. ) ;
#17320=CARTESIAN_POINT ( 'NONE',  ( -2.293366432827344421E-15, -12.48450537969573659, -112.7187500020483952 ) ) ;
#17321=ORIENTED_EDGE ( 'NONE', *, *, #38527, .T. ) ;
#17322=CARTESIAN_POINT ( 'NONE',  ( -2.121150477449813534E-15, -11.54700538379251284, -145.2500000040967905 ) ) ;
#17323=CARTESIAN_POINT ( 'NONE',  ( -10.81189881249999729, 6.242252689847871849, -191.2187500020484663 ) ) ;
#17325=CARTESIAN_POINT ( 'NONE',  ( 10.81189881249999907, 6.242252689847868297, -43.21875000204835970 ) ) ;
#17326=CARTESIAN_POINT ( 'NONE',  ( -9.999999999999998224, 1.224646799147353059E-15, -181.2500000000000284 ) ) ;
#17328=CARTESIAN_POINT ( 'NONE',  ( 5.405949406249999534, 9.363379034771803333, -182.5937500020483810 ) ) ;
#17329=CARTESIAN_POINT ( 'NONE',  ( -2.293366432827344421E-15, -12.48450537969573659, -160.7187500020483810 ) ) ;
#17330=CARTESIAN_POINT ( 'NONE',  ( -5.000000000000003553, -8.660254037844383745, -65.87500000409676204 ) ) ;
#17334=DIRECTION ( 'NONE',  ( -0.000000000000000000, -0.000000000000000000, 1.000000000000000000 ) ) ;
#17336=CARTESIAN_POINT ( 'NONE',  ( 10.81189881249999729, 0.000000000000000000, -88.34375000204838102 ) ) ;
#17338=CARTESIAN_POINT ( 'NONE',  ( 10.81189881249999907, 6.242252689847868297, -64.40625000204839523 ) ) ;
#17340=CARTESIAN_POINT ( 'NONE',  ( 5.405949406249992428, -9.363379034771808662, -123.2812500020483952 ) ) ;
#17341=CARTESIAN_POINT ( 'NONE',  ( 5.405949406249992428, -9.363379034771808662, -151.7812500020484094 ) ) ;
#17343=CARTESIAN_POINT ( 'NONE',  ( 5.000000000000000000, 8.660254037844385522, -126.6250000040967620 ) ) ;
#17345=VERTEX_POINT ( 'NONE', #5923 ) ;
#17349=CARTESIAN_POINT ( 'NONE',  ( -5.405949406249996869, 9.363379034771805109, -187.0312500020484094 ) ) ;
#17351=EDGE_LOOP ( 'NONE', ( #27058, #10310, #1429, #4972 ) ) ;
#17352=CARTESIAN_POINT ( 'NONE',  ( -10.00000000000000000, -5.773502691896251982, -49.12499999999997158 ) ) ;
#17354=CARTESIAN_POINT ( 'NONE',  ( 9.999999999999996447, -5.773502691896262640, -56.50000000409677625 ) ) ;
#17358=CARTESIAN_POINT ( 'NONE',  ( 10.81189881249999729, 0.000000000000000000, -61.53125000204837391 ) ) ;
#17359=EDGE_CURVE ( 'NONE', #20251, #27593, #9152, .T. ) ;
#17363=CARTESIAN_POINT ( 'NONE',  ( -5.405949406249996869, 9.363379034771805109, -175.0312500020484094 ) ) ;
#17365=LINE ( 'NONE', #14763, #12500 ) ;
#17366=CARTESIAN_POINT ( 'NONE',  ( -2.121150477449813534E-15, -11.54700538379251284, -81.87500000000000000 ) ) ;
#17368=CARTESIAN_POINT ( 'NONE',  ( 7.070501591499376803E-16, 11.54700538379251284, -105.5000000040967763 ) ) ;
#17369=CARTESIAN_POINT ( 'NONE',  ( -5.000000000000003553, -8.660254037844383745, -169.3750000040967905 ) ) ;
#17370=CARTESIAN_POINT ( 'NONE',  ( 10.81189881249999551, -6.242252689847874514, -88.65625000204838102 ) ) ;
#17371=VERTEX_POINT ( 'NONE', #15816 ) ;
#17372=DIRECTION ( 'NONE',  ( 0.000000000000000000, 0.000000000000000000, 1.000000000000000000 ) ) ;
#17373=CARTESIAN_POINT ( 'NONE',  ( -2.121150477449813534E-15, -11.54700538379251284, -69.87499999999998579 ) ) ;
#17377=CARTESIAN_POINT ( 'NONE',  ( 5.405949406249999534, 9.363379034771803333, -29.59375000204836326 ) ) ;
#17378=CARTESIAN_POINT ( 'NONE',  ( -5.405949406250003975, -9.363379034771801557, -15.53125000204835793 ) ) ;
#17379=CARTESIAN_POINT ( 'NONE',  ( 10.81189881249999907, 6.242252689847868297, -64.21875000204838102 ) ) ;
#17382=CARTESIAN_POINT ( 'NONE',  ( 7.644554776091147741E-16, 12.48450537969573659, -183.9687500020484094 ) ) ;
#17383=( BOUNDED_CURVE ( )  B_SPLINE_CURVE ( 2, ( #25859, #10285, #7067, #32973, #13302, #36199, #42450 ),
 .UNSPECIFIED., .F., .F. ) 
 B_SPLINE_CURVE_WITH_KNOTS ( ( 3, 2, 2, 3 ),
 ( 0.5932835820895523415, 0.5945273631840797268, 0.5957711442786072231, 0.5970149253731344974 ),
 .UNSPECIFIED. ) 
 CURVE ( )  GEOMETRIC_REPRESENTATION_ITEM ( )  RATIONAL_B_SPLINE_CURVE ( ( 0.9999999999999880096, 0.8660254037844506980, 1.000000000000000000, 0.8660254037844387076, 1.000000000000000000, 0.8660254037844148378, 1.000000000000023981 ) ) 
 REPRESENTATION_ITEM ( '' )  );
#17385=CARTESIAN_POINT ( 'NONE',  ( 9.999999999999998224, 0.000000000000000000, -21.87500000409675494 ) ) ;
#17388=CARTESIAN_POINT ( 'NONE',  ( -9.999999999999227285, -5.773502691896698735, -104.6249999999999574 ) ) ;
#17391=CARTESIAN_POINT ( 'NONE',  ( -2.293366432827344421E-15, -12.48450537969573659, -114.2187500020483668 ) ) ;
#17392=CARTESIAN_POINT ( 'NONE',  ( -9.999999999999998224, 1.224646799147353059E-15, -54.12500000409675494 ) ) ;
#17393=CARTESIAN_POINT ( 'NONE',  ( -10.81189881249999729, 1.324075727343319199E-15, -92.28125000204838102 ) ) ;
#17394=CARTESIAN_POINT ( 'NONE',  ( 5.405949406249992428, -9.363379034771808662, -103.5937500020483668 ) ) ;
#17397=CARTESIAN_POINT ( 'NONE',  ( 10.00000000000000000, 5.773502691896255534, -153.7500000040967905 ) ) ;
#17401=DIRECTION ( 'NONE',  ( 1.000000000000000000, 0.000000000000000000, 0.000000000000000000 ) ) ;
#17402=LINE ( 'NONE', #23913, #40118 ) ;
#17404=CARTESIAN_POINT ( 'NONE',  ( 9.999999999998969713, 5.773502691896851502, -10.87499999999993072 ) ) ;
#17405=CARTESIAN_POINT ( 'NONE',  ( -4.999999999999996447, 8.660254037844387298, -76.49999999999998579 ) ) ;
#17407=CARTESIAN_POINT ( 'NONE',  ( 7.070501591499377789E-16, 11.54700538379251284, -89.00000000409677625 ) ) ;
#17410=CARTESIAN_POINT ( 'NONE',  ( 7.644554776091147741E-16, 12.48450537969573659, -82.15625000204839523 ) ) ;
#17412=CARTESIAN_POINT ( 'NONE',  ( -9.999999999999998224, 1.224646799147353059E-15, -19.24999999999996092 ) ) ;
#17414=VERTEX_POINT ( 'NONE', #15397 ) ;
#17415=CARTESIAN_POINT ( 'NONE',  ( 4.999999999999992006, -8.660254037844389075, -3.749999999999975575 ) ) ;
#17417=ADVANCED_FACE ( 'NONE', ( #16025 ), #32048, .T. ) ;
#17418=CARTESIAN_POINT ( 'NONE',  ( -10.81189881249999729, -6.242252689847864744, -13.96875000204836681 ) ) ;
#17421=CARTESIAN_POINT ( 'NONE',  ( -5.405949406250003975, -9.363379034771801557, -134.0312500020484094 ) ) ;
#17422=CARTESIAN_POINT ( 'NONE',  ( 9.999999999999996447, -5.773502691896262640, -179.1250000000000284 ) ) ;
#17424=CARTESIAN_POINT ( 'NONE',  ( 10.81189881249999729, 0.000000000000000000, -111.0312500020483810 ) ) ;
#17426=CARTESIAN_POINT ( 'NONE',  ( -9.999999999999998224, 1.224646799147353059E-15, -194.7500000000000000 ) ) ;
#17427=ORIENTED_EDGE ( 'NONE', *, *, #21492, .F. ) ;
#17428=ORIENTED_EDGE ( 'NONE', *, *, #7910, .T. ) ;
#17430=CARTESIAN_POINT ( 'NONE',  ( 5.405949406249999534, 9.363379034771803333, -35.78125000204837391 ) ) ;
#17432=CARTESIAN_POINT ( 'NONE',  ( 7.644554776091147741E-16, 12.48450537969573659, -92.46875000204838102 ) ) ;
#17433=DIRECTION ( 'NONE',  ( -0.000000000000000000, -0.000000000000000000, 1.000000000000000000 ) ) ;
#17434=DIRECTION ( 'NONE',  ( -0.000000000000000000, -0.000000000000000000, 1.000000000000000000 ) ) ;
#17435=( BOUNDED_CURVE ( )  B_SPLINE_CURVE ( 2, ( #5516, #32068, #21488, #28190, #41750, #24963, #2502 ),
 .UNSPECIFIED., .F., .F. ) 
 B_SPLINE_CURVE_WITH_KNOTS ( ( 3, 2, 2, 3 ),
 ( 0.6194029850746269883, 0.6206467661691543736, 0.6218905472636816478, 0.6231343283582090331 ),
 .UNSPECIFIED. ) 
 CURVE ( )  GEOMETRIC_REPRESENTATION_ITEM ( )  RATIONAL_B_SPLINE_CURVE ( ( 0.9999999999999880096, 0.8660254037844506980, 1.000000000000000000, 0.8660254037844387076, 1.000000000000000000, 0.8660254037844267172, 1.000000000000011990 ) ) 
 REPRESENTATION_ITEM ( '' )  );
#17437=CARTESIAN_POINT ( 'NONE',  ( 9.999999999999998224, 0.000000000000000000, -58.99999999999997158 ) ) ;
#17438=CARTESIAN_POINT ( 'NONE',  ( 5.405949406249992428, -9.363379034771808662, -123.0937500020483952 ) ) ;
#17442=CARTESIAN_POINT ( 'NONE',  ( 9.999999999999998224, 0.000000000000000000, -183.8750000040967905 ) ) ;
#17444=CARTESIAN_POINT ( 'NONE',  ( -10.81189881249999729, 1.324075727343319199E-15, -182.2812500020483810 ) ) ;
#17445=CARTESIAN_POINT ( 'NONE',  ( -9.999999999999227285, -5.773502691896698735, -107.6249999999999574 ) ) ;
#17448=CARTESIAN_POINT ( 'NONE',  ( 10.81189881249999729, 6.242252689847867408, -50.71875000204835970 ) ) ;
#17449=CARTESIAN_POINT ( 'NONE',  ( -10.81189881249999729, 6.242252689847871849, -44.21875000204836681 ) ) ;
#17451=CARTESIAN_POINT ( 'NONE',  ( -5.405949406249996869, 9.363379034771805109, -10.03125000204835260 ) ) ;
#17455=CARTESIAN_POINT ( 'NONE',  ( -2.121150477449813534E-15, -11.54700538379251284, -98.37500000000000000 ) ) ;
#17457=CARTESIAN_POINT ( 'NONE',  ( 7.070501591499377789E-16, 11.54700538379251284, -111.5000000040967763 ) ) ;
#17461=CARTESIAN_POINT ( 'NONE',  ( -5.405949406250003975, -9.363379034771801557, -107.0312500020483810 ) ) ;
#17463=CARTESIAN_POINT ( 'NONE',  ( 9.999999999998456346, 5.773502691897149042, -8.250000004096712303 ) ) ;
#17465=CARTESIAN_POINT ( 'NONE',  ( 9.999999999999994671, -5.773502691896262640, -166.0000000040967905 ) ) ;
#17468=CARTESIAN_POINT ( 'NONE',  ( -9.999999999999998224, 5.773502691896259087, -28.37499999999997158 ) ) ;
#17469=EDGE_CURVE ( 'NONE', #32539, #13704, #21240, .T. ) ;
#17470=CARTESIAN_POINT ( 'NONE',  ( -10.81189881249999729, 6.242252689847871849, -32.40625000204835970 ) ) ;
#17471=CARTESIAN_POINT ( 'NONE',  ( -4.999999999999996447, 8.660254037844387298, -159.0000000000000000 ) ) ;
#17472=ADVANCED_FACE ( 'NONE', ( #28594 ), #29221, .T. ) ;
#17475=EDGE_CURVE ( 'NONE', #14562, #10196, #22893, .T. ) ;
#17476=EDGE_CURVE ( 'NONE', #21320, #1841, #24290, .T. ) ;
#17477=CARTESIAN_POINT ( 'NONE',  ( 7.644554776091147741E-16, 12.48450537969573659, -136.1562500020483810 ) ) ;
#17479=FACE_OUTER_BOUND ( 'NONE', #4324, .T. ) ;
#17483=EDGE_CURVE ( 'NONE', #41727, #35978, #30078, .T. ) ;
#17485=CARTESIAN_POINT ( 'NONE',  ( -9.999999999999998224, 1.224646799147353059E-15, -134.7499999999999716 ) ) ;
#17486=CARTESIAN_POINT ( 'NONE',  ( 5.405949406249992428, -9.363379034771808662, -163.5937500020484094 ) ) ;
#17489=CARTESIAN_POINT ( 'NONE',  ( 5.405949406249999534, 9.363379034771803333, -17.59375000204835260 ) ) ;
#17490=EDGE_CURVE ( 'NONE', #26632, #18779, #33530, .T. ) ;
#17491=CARTESIAN_POINT ( 'NONE',  ( -10.81189881249999729, 1.324075727343319199E-15, -150.5937500020483810 ) ) ;
#17492=CARTESIAN_POINT ( 'NONE',  ( -5.405949406249996869, 9.363379034771805109, -135.8437500020484094 ) ) ;
#17493=CARTESIAN_POINT ( 'NONE',  ( -2.293366432827344421E-15, -12.48450537969573659, -108.4062500020483810 ) ) ;
#17497=CARTESIAN_POINT ( 'NONE',  ( 5.405949406249999534, 9.363379034771803333, -13.09375000204834905 ) ) ;
#17499=CARTESIAN_POINT ( 'NONE',  ( 5.000000000000000000, 8.660254037844385522, -125.1250000040967620 ) ) ;
#17502=CARTESIAN_POINT ( 'NONE',  ( -10.81189881249999729, 1.324075727343319199E-15, -78.59375000204838102 ) ) ;
#17503=CARTESIAN_POINT ( 'NONE',  ( 10.81189881249999729, 0.000000000000000000, -67.34375000204836681 ) ) ;
#17504=CARTESIAN_POINT ( 'NONE',  ( -5.000000000000003553, -8.660254037844383745, -167.5000000000000000 ) ) ;
#17505=CARTESIAN_POINT ( 'NONE',  ( 5.405949406249992428, -9.363379034771808662, -34.78125000204837391 ) ) ;
#17507=CARTESIAN_POINT ( 'NONE',  ( 9.999999999999998224, 0.000000000000000000, -200.0000000000000000 ) ) ;
#17509=CARTESIAN_POINT ( 'NONE',  ( -9.999999999999998224, 1.224646799147353059E-15, -118.2500000000000000 ) ) ;
#17510=CARTESIAN_POINT ( 'NONE',  ( -10.81189881249999729, 6.242252689847871849, -132.9062500020483810 ) ) ;
#17511=EDGE_CURVE ( 'NONE', #24195, #33229, #36960, .T. ) ;
#17514=CARTESIAN_POINT ( 'NONE',  ( -10.81189881249999729, 6.242252689847871849, -20.40625000204838102 ) ) ;
#17518=CARTESIAN_POINT ( 'NONE',  ( 4.999999999999992006, -8.660254037844389075, -34.12500000409676915 ) ) ;
#17519=CARTESIAN_POINT ( 'NONE',  ( 9.999999999999998224, 0.000000000000000000, -98.37500000409677625 ) ) ;
#17521=CYLINDRICAL_SURFACE ( 'NONE', #7636, 9.999999999999998224 ) ;
#17522=CARTESIAN_POINT ( 'NONE',  ( -10.81189881249999729, 1.324075727343319199E-15, -156.7812500020484094 ) ) ;
#17523=CARTESIAN_POINT ( 'NONE',  ( 10.81189881249999551, -6.242252689847874514, -125.9687500020483810 ) ) ;
#17524=CARTESIAN_POINT ( 'NONE',  ( 9.999999999999998224, 0.000000000000000000, -200.0000000000000000 ) ) ;
#17525=ORIENTED_EDGE ( 'NONE', *, *, #15901, .F. ) ;
#17526=CARTESIAN_POINT ( 'NONE',  ( 9.999999999998969713, 5.773502691896851502, -31.87499999999993960 ) ) ;
#17527=VERTEX_POINT ( 'NONE', #30290 ) ;
#17528=ORIENTED_EDGE ( 'NONE', *, *, #9990, .T. ) ;
#17529=CARTESIAN_POINT ( 'NONE',  ( -10.81189881249999729, 1.324075727343319199E-15, -110.0937500020483810 ) ) ;
#17530=ORIENTED_EDGE ( 'NONE', *, *, #9304, .F. ) ;
#17532=CARTESIAN_POINT ( 'NONE',  ( 5.405949406249999534, 9.363379034771803333, -193.0937500020484094 ) ) ;
#17533=CARTESIAN_POINT ( 'NONE',  ( 10.81189881249999907, 6.242252689847868297, -40.21875000204835970 ) ) ;
#17534=CARTESIAN_POINT ( 'NONE',  ( -8.239685287916026724, -5.747359526181299749, -1.202135122527665920E-14 ) ) ;
#17535=CARTESIAN_POINT ( 'NONE',  ( 4.999999999999992006, -8.660254037844389075, -10.12500000409674605 ) ) ;
#17536=CARTESIAN_POINT ( 'NONE',  ( 10.81189881249999729, 6.242252689847867408, -173.7187500020483810 ) ) ;
#17537=CARTESIAN_POINT ( 'NONE',  ( -2.293366432827344421E-15, -12.48450537969573659, -157.7187500020484094 ) ) ;
#17538=CARTESIAN_POINT ( 'NONE',  ( -2.121150477449813534E-15, -11.54700538379251284, -65.75000000409677625 ) ) ;
#17542=CARTESIAN_POINT ( 'NONE',  ( -10.00000000000102496, 5.773502691895664007, -35.87499999999993605 ) ) ;
#17544=CARTESIAN_POINT ( 'NONE',  ( 10.81189881249999551, -6.242252689847874514, -91.46875000204838102 ) ) ;
#17546=CARTESIAN_POINT ( 'NONE',  ( 7.644554776091147741E-16, 12.48450537969573659, -55.15625000204837391 ) ) ;
#17547=CARTESIAN_POINT ( 'NONE',  ( -10.00000000000102496, 5.773502691895664007, -87.25000000409674783 ) ) ;
#17549=CARTESIAN_POINT ( 'NONE',  ( 7.644554776091147741E-16, 12.48450537969573659, -122.6562500020483952 ) ) ;
#17550=CARTESIAN_POINT ( 'NONE',  ( 5.405949406249992428, -9.363379034771808662, -157.7812500020484094 ) ) ;
#17553=CARTESIAN_POINT ( 'NONE',  ( 4.999999999999992006, -8.660254037844389075, -128.6250000040967620 ) ) ;
#17555=EDGE_LOOP ( 'NONE', ( #33918, #24425, #2587, #20764 ) ) ;
#17556=AXIS2_PLACEMENT_3D ( 'NONE', #14970, #14756, #18435 ) ;
#17560=CARTESIAN_POINT ( 'NONE',  ( 10.81189881249999907, 6.242252689847868297, -188.9062500020484379 ) ) ;
#17561=VERTEX_POINT ( 'NONE', #23602 ) ;
#17562=CARTESIAN_POINT ( 'NONE',  ( -2.121150477449813534E-15, -11.54700538379251284, -48.87499999999997868 ) ) ;
#17564=CARTESIAN_POINT ( 'NONE',  ( 9.999999999999998224, 0.000000000000000000, -54.87500000409675494 ) ) ;
#17565=CYLINDRICAL_SURFACE ( 'NONE', #31372, 9.999999999999998224 ) ;
#17566=CARTESIAN_POINT ( 'NONE',  ( 9.999999999999998224, 0.000000000000000000, -179.3750000040967905 ) ) ;
#17568=CARTESIAN_POINT ( 'NONE',  ( 5.405949406249999534, 9.363379034771803333, -50.78125000204835970 ) ) ;
#17571=CARTESIAN_POINT ( 'NONE',  ( -9.999999999999998224, 1.224646799147353059E-15, -35.74999999999997868 ) ) ;
#17572=CARTESIAN_POINT ( 'NONE',  ( 10.81189881249999907, 6.242252689847868297, -175.4062500020484094 ) ) ;
#17575=CARTESIAN_POINT ( 'NONE',  ( 0.000000000000000000, 0.000000000000000000, -200.0000000000000000 ) ) ;
#17576=LINE ( 'NONE', #27746, #6313 ) ;
#17578=VECTOR ( 'NONE', #9523, 1000.000000000000000 ) ;
#17579=CARTESIAN_POINT ( 'NONE',  ( 9.999999999999998224, 0.000000000000000000, -186.8750000040967905 ) ) ;
#17581=CARTESIAN_POINT ( 'NONE',  ( 7.644554776091147741E-16, 12.48450537969573659, -83.65625000204838102 ) ) ;
#17583=CARTESIAN_POINT ( 'NONE',  ( -9.999999999999998224, 1.224646799147353059E-15, -80.74999999999998579 ) ) ;
#17584=ORIENTED_EDGE ( 'NONE', *, *, #23366, .T. ) ;
#17586=ORIENTED_EDGE ( 'NONE', *, *, #29989, .T. ) ;
#17587=CARTESIAN_POINT ( 'NONE',  ( 7.644554776091147741E-16, 12.48450537969573659, -38.46875000204835970 ) ) ;
#17588=CARTESIAN_POINT ( 'NONE',  ( 7.644554776091147741E-16, 12.48450537969573659, -24.96875000204837036 ) ) ;
#17589=CARTESIAN_POINT ( 'NONE',  ( 5.405949406249992428, -9.363379034771808662, -15.28125000204835793 ) ) ;
#17590=CARTESIAN_POINT ( 'NONE',  ( 7.644554776091147741E-16, 12.48450537969573659, -65.46875000204836681 ) ) ;
#17591=CARTESIAN_POINT ( 'NONE',  ( -5.000000000000003553, -8.660254037844383745, -131.5000000000000000 ) ) ;
#17593=CARTESIAN_POINT ( 'NONE',  ( 10.81189881249999551, -6.242252689847874514, -181.4687500020484094 ) ) ;
#17597=CARTESIAN_POINT ( 'NONE',  ( -9.999999999999998224, 1.224646799147353059E-15, -199.2500000000000000 ) ) ;
#17599=CARTESIAN_POINT ( 'NONE',  ( 5.000000000000000000, 8.660254037844385522, 0.8749999959032361829 ) ) ;
#17600=DIRECTION ( 'NONE',  ( 0.000000000000000000, 0.000000000000000000, -1.000000000000000000 ) ) ;
#17601=CARTESIAN_POINT ( 'NONE',  ( -5.405949406250003975, -9.363379034771801557, -109.8437500020483810 ) ) ;
#17603=CARTESIAN_POINT ( 'NONE',  ( 5.405949406249999534, 9.363379034771803333, -92.78125000204838102 ) ) ;
#17604=CARTESIAN_POINT ( 'NONE',  ( -5.405949406249996869, 9.363379034771805109, -101.3437500020483810 ) ) ;
#17607=CARTESIAN_POINT ( 'NONE',  ( 7.070501591499377789E-16, 11.54700538379251284, -156.5000000040968189 ) ) ;
#17612=CARTESIAN_POINT ( 'NONE',  ( -9.999999999999998224, 1.224646799147353059E-15, -153.1250000040967905 ) ) ;
#17613=CARTESIAN_POINT ( 'NONE',  ( -2.121150477449813534E-15, -11.54700538379251284, -197.3750000000000000 ) ) ;
#17615=CARTESIAN_POINT ( 'NONE',  ( -9.999999999999998224, 1.224646799147353059E-15, -130.6250000040967620 ) ) ;
#17616=CARTESIAN_POINT ( 'NONE',  ( -2.121150477449813534E-15, -11.54700538379251284, -75.87500000000000000 ) ) ;
#17618=CARTESIAN_POINT ( 'NONE',  ( 9.999999999999998224, 0.000000000000000000, -81.87500000409676204 ) ) ;
#17620=CARTESIAN_POINT ( 'NONE',  ( 7.070501591499376803E-16, 11.54700538379251284, -115.6249999999999858 ) ) ;
#17622=CARTESIAN_POINT ( 'NONE',  ( -10.81189881249999729, -6.242252689847864744, -87.65625000204836681 ) ) ;
#17624=CARTESIAN_POINT ( 'NONE',  ( 9.999999999999998224, 0.000000000000000000, -58.99999999999997158 ) ) ;
#17626=EDGE_LOOP ( 'NONE', ( #15300, #4125, #34022, #25590 ) ) ;
#17627=CARTESIAN_POINT ( 'NONE',  ( -4.999999999999996447, 8.660254037844387298, -2.999999999999975131 ) ) ;
#17629=CARTESIAN_POINT ( 'NONE',  ( -5.405949406249996869, 9.363379034771805109, -17.34375000204835260 ) ) ;
#17630=CARTESIAN_POINT ( 'NONE',  ( -2.121150477449813534E-15, -11.54700538379251284, -176.7500000040967620 ) ) ;
#17632=CARTESIAN_POINT ( 'NONE',  ( -5.405949406250003975, -9.363379034771801557, -132.5312500020484094 ) ) ;
#17633=EDGE_CURVE ( 'NONE', #37834, #14232, #25675, .T. ) ;
#17634=CARTESIAN_POINT ( 'NONE',  ( -10.00000000000000000, -5.773502691896251982, -184.1250000000000284 ) ) ;
#17636=CARTESIAN_POINT ( 'NONE',  ( 10.81189881249999551, -6.242252689847874514, -111.1562500020483952 ) ) ;
#17637=EDGE_LOOP ( 'NONE', ( #15736, #11653, #39150, #18295 ) ) ;
#17638=CARTESIAN_POINT ( 'NONE',  ( -10.00000000000076916, 5.773502691895813221, -138.2500000040967905 ) ) ;
#17639=VERTEX_POINT ( 'NONE', #26616 ) ;
#17640=( BOUNDED_CURVE ( )  B_SPLINE_CURVE ( 2, ( #7574, #23561, #4759, #30469, #13809, #11225, #27208 ),
 .UNSPECIFIED., .F., .F. ) 
 B_SPLINE_CURVE_WITH_KNOTS ( ( 3, 2, 2, 3 ),
 ( 0.3917910447761194792, 0.3930348258706468090, 0.3942786069651742498, 0.3955223880597015795 ),
 .UNSPECIFIED. ) 
 CURVE ( )  GEOMETRIC_REPRESENTATION_ITEM ( )  RATIONAL_B_SPLINE_CURVE ( ( 0.9999999999999940048, 0.8660254037844447028, 1.000000000000000000, 0.8660254037844387076, 1.000000000000000000, 0.8660254037844267172, 1.000000000000011990 ) ) 
 REPRESENTATION_ITEM ( '' )  );
#17642=CARTESIAN_POINT ( 'NONE',  ( 5.405949406249999534, 9.363379034771803333, -40.28125000204838102 ) ) ;
#17644=CARTESIAN_POINT ( 'NONE',  ( 7.644554776091147741E-16, 12.48450537969573659, -86.46875000204838102 ) ) ;
#17646=CARTESIAN_POINT ( 'NONE',  ( 9.999999999999998224, 0.000000000000000000, -32.37500000409676204 ) ) ;
#17649=CARTESIAN_POINT ( 'NONE',  ( -5.405949406249996869, 9.363379034771805109, -125.3437500020483952 ) ) ;
#17651=CARTESIAN_POINT ( 'NONE',  ( 10.81189881249999729, 0.7537365248293982356, -0.01615656218219799906 ) ) ;
#17654=CARTESIAN_POINT ( 'NONE',  ( 9.999999999999996447, -5.773502691896262640, -176.5000000040968189 ) ) ;
#17656=CARTESIAN_POINT ( 'NONE',  ( 10.81189881249999729, 6.242252689847867408, -181.4062500020484379 ) ) ;
#17657=LINE ( 'NONE', #1289, #17859 ) ;
#17658=CARTESIAN_POINT ( 'NONE',  ( 9.999999999999479527, 5.773502691896553074, -122.2500000040967763 ) ) ;
#17660=CARTESIAN_POINT ( 'NONE',  ( 5.405949406249999534, 9.363379034771803333, -53.59375000204835970 ) ) ;
#17661=CARTESIAN_POINT ( 'NONE',  ( -10.81189881249999729, 1.324075727343319199E-15, -41.09375000204837391 ) ) ;
#17663=CARTESIAN_POINT ( 'NONE',  ( 10.81189881249999551, -6.242252689847874514, -10.65625000204838280 ) ) ;
#17665=LINE ( 'NONE', #31727, #8203 ) ;
#17667=CARTESIAN_POINT ( 'NONE',  ( 9.999999999999998224, 0.000000000000000000, -96.49999999999998579 ) ) ;
#17669=CARTESIAN_POINT ( 'NONE',  ( -2.121150477449813534E-15, -11.54700538379251284, -104.7500000040967763 ) ) ;
#17672=CARTESIAN_POINT ( 'NONE',  ( 5.405949406249999534, 9.363379034771803333, -107.7812500020483810 ) ) ;
#17674=FACE_OUTER_BOUND ( 'NONE', #10746, .T. ) ;
#17677=CARTESIAN_POINT ( 'NONE',  ( -10.81189881249999729, 6.242252689847871849, -165.9062500020483810 ) ) ;
#17679=VERTEX_POINT ( 'NONE', #13210 ) ;
#17680=CARTESIAN_POINT ( 'NONE',  ( -5.000000000000003553, -8.660254037844383745, -27.99999999999996803 ) ) ;
#17681=CARTESIAN_POINT ( 'NONE',  ( -10.81189881249999729, 1.324075727343319199E-15, -38.28125000204838102 ) ) ;
#17682=CARTESIAN_POINT ( 'NONE',  ( -4.999999999999996447, 8.660254037844387298, -165.0000000000000000 ) ) ;
#17685=( BOUNDED_CURVE ( )  B_SPLINE_CURVE ( 2, ( #34514, #31487, #1921, #23942, #12034, #39007, #38162 ),
 .UNSPECIFIED., .F., .F. ) 
 B_SPLINE_CURVE_WITH_KNOTS ( ( 3, 2, 2, 3 ),
 ( 0.3507462686567164867, 0.3519900497512438720, 0.3532338308457712572, 0.3544776119402986980 ),
 .UNSPECIFIED. ) 
 CURVE ( )  GEOMETRIC_REPRESENTATION_ITEM ( )  RATIONAL_B_SPLINE_CURVE ( ( 0.9999999999999940048, 0.8660254037844447028, 1.000000000000000000, 0.8660254037844387076, 1.000000000000000000, 0.8660254037844207220, 1.000000000000017986 ) ) 
 REPRESENTATION_ITEM ( '' )  );
#17686=FACE_OUTER_BOUND ( 'NONE', #25520, .T. ) ;
#17687=CARTESIAN_POINT ( 'NONE',  ( -5.405949406250003975, -9.363379034771801557, -134.0312500020484094 ) ) ;
#17688=CARTESIAN_POINT ( 'NONE',  ( 9.794892170062176717, 4.319011525664689266, 3.656666817559538189E-15 ) ) ;
#17690=VERTEX_POINT ( 'NONE', #33099 ) ;
#17691=( BOUNDED_CURVE ( )  B_SPLINE_CURVE ( 2, ( #5093, #12185, #28408, #41960, #22130, #38315, #38523 ),
 .UNSPECIFIED., .F., .F. ) 
 B_SPLINE_CURVE_WITH_KNOTS ( ( 3, 2, 2, 3 ),
 ( 0.7276119402985077311, 0.7288557213930350054, 0.7300995024875623907, 0.7313432835820897759 ),
 .UNSPECIFIED. ) 
 CURVE ( )  GEOMETRIC_REPRESENTATION_ITEM ( )  RATIONAL_B_SPLINE_CURVE ( ( 0.9999999999999761302, 0.8660254037844625774, 1.000000000000000000, 0.8660254037844387076, 1.000000000000000000, 0.8660254037844148378, 1.000000000000023981 ) ) 
 REPRESENTATION_ITEM ( '' )  );
#17692=EDGE_LOOP ( 'NONE', ( #12484, #3694, #42433, #18601 ) ) ;
#17694=CARTESIAN_POINT ( 'NONE',  ( -9.999999999999998224, 1.224646799147353059E-15, -123.1250000040967905 ) ) ;
#17695=CARTESIAN_POINT ( 'NONE',  ( 10.00000000000154010, -5.773502691895370020, -55.00000000409672651 ) ) ;
#17696=CARTESIAN_POINT ( 'NONE',  ( -2.293366432827344421E-15, -12.48450537969573659, -168.2187500020483810 ) ) ;
#17698=CARTESIAN_POINT ( 'NONE',  ( -5.405949406250003975, -9.363379034771801557, -15.34375000204835082 ) ) ;
#17699=CARTESIAN_POINT ( 'NONE',  ( -5.000000000000003553, -8.660254037844383745, -157.3750000040967905 ) ) ;
#17700=EDGE_CURVE ( 'NONE', #18552, #14343, #300, .T. ) ;
#17701=CARTESIAN_POINT ( 'NONE',  ( 5.405949406249992428, -9.363379034771808662, -145.5937500020483810 ) ) ;
#17702=CARTESIAN_POINT ( 'NONE',  ( -2.293366432827344421E-15, -12.48450537969573659, -138.2187500020483810 ) ) ;
#17704=CARTESIAN_POINT ( 'NONE',  ( -5.405949406250003975, -9.363379034771801557, -107.0312500020483810 ) ) ;
#17708=CARTESIAN_POINT ( 'NONE',  ( -4.999999999999996447, 8.660254037844387298, -198.3750000040967905 ) ) ;
#17710=CARTESIAN_POINT ( 'NONE',  ( -5.000000000000003553, -8.660254037844383745, -54.99999999999996447 ) ) ;
#17711=CARTESIAN_POINT ( 'NONE',  ( -10.00000000000102496, 5.773502691895664007, -4.750000004096740724 ) ) ;
#17714=CARTESIAN_POINT ( 'NONE',  ( 5.405949406249992428, -9.363379034771808662, -76.59375000204838102 ) ) ;
#17715=CARTESIAN_POINT ( 'NONE',  ( -10.81189881249999729, 1.324075727343319199E-15, -68.09375000204836681 ) ) ;
#17716=CARTESIAN_POINT ( 'NONE',  ( -9.999999999998456346, -5.773502691897145489, -19.50000000409673717 ) ) ;
#17717=CARTESIAN_POINT ( 'NONE',  ( -10.81189881249999729, 6.242252689847871849, -32.40625000204835970 ) ) ;
#17719=CARTESIAN_POINT ( 'NONE',  ( 0.000000000000000000, 0.000000000000000000, -200.0000000000000000 ) ) ;
#17721=CARTESIAN_POINT ( 'NONE',  ( 4.999999999999992006, -8.660254037844389075, -120.7500000000000000 ) ) ;
#17722=CARTESIAN_POINT ( 'NONE',  ( 10.81189881249999551, -6.242252689847874514, -132.1562500020483810 ) ) ;
#17725=CARTESIAN_POINT ( 'NONE',  ( 10.81189881249999729, 0.000000000000000000, -19.53125000204835970 ) ) ;
#17726=ORIENTED_EDGE ( 'NONE', *, *, #2245, .F. ) ;
#17729=CARTESIAN_POINT ( 'NONE',  ( 0.000000000000000000, 0.000000000000000000, -200.0000000000000000 ) ) ;
#17730=CARTESIAN_POINT ( 'NONE',  ( -2.121150477449813534E-15, -11.54700538379251284, -32.75000000409674783 ) ) ;
#17731=ADVANCED_FACE ( 'NONE', ( #11691 ), #11262, .T. ) ;
#17734=CARTESIAN_POINT ( 'NONE',  ( -5.000000000000003553, -8.660254037844383745, -146.5000000000000000 ) ) ;
#17735=CARTESIAN_POINT ( 'NONE',  ( -2.293366432827344421E-15, -12.48450537969573659, -154.9062500020483810 ) ) ;
#17736=CARTESIAN_POINT ( 'NONE',  ( -10.81189881249999907, -6.242252689847864744, -126.4687500020483810 ) ) ;
#17737=CARTESIAN_POINT ( 'NONE',  ( 5.000000000000000000, 8.660254037844385522, -3.625000004096767814 ) ) ;
#17738=EDGE_CURVE ( 'NONE', #21791, #8991, #30083, .T. ) ;
#17739=ORIENTED_EDGE ( 'NONE', *, *, #2344, .F. ) ;
#17740=CARTESIAN_POINT ( 'NONE',  ( 9.999999999999998224, 0.000000000000000000, -22.99999999999996447 ) ) ;
#17742=VERTEX_POINT ( 'NONE', #34170 ) ;
#17743=AXIS2_PLACEMENT_3D ( 'NONE', #4890, #37474, #7701 ) ;
#17744=CARTESIAN_POINT ( 'NONE',  ( 10.81189881249999729, 0.000000000000000000, -112.3437500020483810 ) ) ;
#17745=ORIENTED_EDGE ( 'NONE', *, *, #11167, .T. ) ;
#17747=CARTESIAN_POINT ( 'NONE',  ( 9.999999999999742428, 5.773502691896404748, -129.7500000040967905 ) ) ;
#17748=CARTESIAN_POINT ( 'NONE',  ( 5.405949406249992428, -9.363379034771808662, -192.0937500020484094 ) ) ;
#17749=CARTESIAN_POINT ( 'NONE',  ( 5.405949406249999534, 9.363379034771803333, -38.59375000204837391 ) ) ;
#17751=CARTESIAN_POINT ( 'NONE',  ( -9.999999999999998224, 1.224646799147353059E-15, -74.74999999999998579 ) ) ;
#17753=CARTESIAN_POINT ( 'NONE',  ( -10.81189881249999729, 6.242252689847871849, -168.7187500020483810 ) ) ;
#17754=CARTESIAN_POINT ( 'NONE',  ( 7.644554776091147741E-16, 12.48450537969573659, -164.4687500020483810 ) ) ;
#17756=DIRECTION ( 'NONE',  ( -0.000000000000000000, -0.000000000000000000, 1.000000000000000000 ) ) ;
#17761=CARTESIAN_POINT ( 'NONE',  ( 9.999999999999998224, 0.000000000000000000, -189.8750000040967905 ) ) ;
#17764=EDGE_CURVE ( 'NONE', #27810, #7227, #4995, .T. ) ;
#17765=CARTESIAN_POINT ( 'NONE',  ( 10.81189881249999729, 0.000000000000000000, -86.84375000204836681 ) ) ;
#17766=CARTESIAN_POINT ( 'NONE',  ( -4.999999999999996447, 8.660254037844387298, -180.3750000040967905 ) ) ;
#17767=CARTESIAN_POINT ( 'NONE',  ( 10.81189881249999729, 0.000000000000000000, -60.03125000204836681 ) ) ;
#17768=CARTESIAN_POINT ( 'NONE',  ( -9.999999999999998224, 1.224646799147353059E-15, -97.62500000409677625 ) ) ;
#17770=CARTESIAN_POINT ( 'NONE',  ( -10.81189881249999729, 6.242252689847871849, -116.4062500020483810 ) ) ;
#17771=CARTESIAN_POINT ( 'NONE',  ( -5.405949406250003975, -9.363379034771801557, -153.5312500020484094 ) ) ;
#17774=CARTESIAN_POINT ( 'NONE',  ( 4.999999999999992006, -8.660254037844389075, -133.1250000040967620 ) ) ;
#17776=ORIENTED_EDGE ( 'NONE', *, *, #18083, .F. ) ;
#17780=CARTESIAN_POINT ( 'NONE',  ( 5.405949406249999534, 9.363379034771803333, -179.7812500020484094 ) ) ;
#17781=ORIENTED_EDGE ( 'NONE', *, *, #38855, .T. ) ;
#17782=CARTESIAN_POINT ( 'NONE',  ( 9.999999999999998224, 0.000000000000000000, -51.49999999999996447 ) ) ;
#17784=CARTESIAN_POINT ( 'NONE',  ( -9.999999999999998224, 5.773502691896259087, -61.75000000409678336 ) ) ;
#17785=AXIS2_PLACEMENT_3D ( 'NONE', #21871, #11718, #25760 ) ;
#17786=CYLINDRICAL_SURFACE ( 'NONE', #17556, 9.999999999999998224 ) ;
#17787=CARTESIAN_POINT ( 'NONE',  ( 7.070501591499376803E-16, 11.54700538379251284, -171.5000000040967905 ) ) ;
#17789=CARTESIAN_POINT ( 'NONE',  ( 5.405949406249992428, -9.363379034771808662, -52.78125000204836681 ) ) ;
#17790=EDGE_CURVE ( 'NONE', #5420, #23886, #28121, .T. ) ;
#17793=CARTESIAN_POINT ( 'NONE',  ( -2.121150477449813534E-15, -11.54700538379251284, -29.75000000409675494 ) ) ;
#17794=CARTESIAN_POINT ( 'NONE',  ( -5.405949406250003975, -9.363379034771801557, -179.0312500020483810 ) ) ;
#17795=CARTESIAN_POINT ( 'NONE',  ( -10.00000000000051337, 5.773502691895962435, -147.2500000040967905 ) ) ;
#17797=DIRECTION ( 'NONE',  ( 0.9961946980917455452, 0.000000000000000000, -0.08715574274765837404 ) ) ;
#17798=CARTESIAN_POINT ( 'NONE',  ( 5.000000000000000000, 8.660254037844385522, -105.6250000040967763 ) ) ;
#17799=CARTESIAN_POINT ( 'NONE',  ( 9.999999999999998224, 0.000000000000000000, -39.87500000409676915 ) ) ;
#17800=CARTESIAN_POINT ( 'NONE',  ( 7.644554776091147741E-16, 12.48450537969573659, -89.65625000204839523 ) ) ;
#17802=DIRECTION ( 'NONE',  ( -0.000000000000000000, -0.000000000000000000, 1.000000000000000000 ) ) ;
#17805=ORIENTED_EDGE ( 'NONE', *, *, #12168, .T. ) ;
#17806=( BOUNDED_CURVE ( )  B_SPLINE_CURVE ( 2, ( #822, #27136, #23057, #615, #23267, #6861, #19799 ),
 .UNSPECIFIED., .F., .F. ) 
 B_SPLINE_CURVE_WITH_KNOTS ( ( 3, 2, 2, 3 ),
 ( 0.2500000000000001110, 0.2512437810945274963, 0.2524875621890548261, 0.2537313432835822113 ),
 .UNSPECIFIED. ) 
 CURVE ( )  GEOMETRIC_REPRESENTATION_ITEM ( )  RATIONAL_B_SPLINE_CURVE ( ( 0.9999999999999880096, 0.8660254037844506980, 1.000000000000000000, 0.8660254037844387076, 1.000000000000000000, 0.8660254037844267172, 1.000000000000011990 ) ) 
 REPRESENTATION_ITEM ( '' )  );
#17807=CARTESIAN_POINT ( 'NONE',  ( 10.81189881249999551, -6.242252689847874514, -34.46875000204835260 ) ) ;
#17808=CARTESIAN_POINT ( 'NONE',  ( 10.81189881249999907, 6.242252689847868297, -28.21875000204838457 ) ) ;
#17809=CARTESIAN_POINT ( 'NONE',  ( 10.81189881249999729, 0.000000000000000000, -16.53125000204835970 ) ) ;
#17810=CARTESIAN_POINT ( 'NONE',  ( -10.81189881249999907, -6.242252689847864744, -61.96875000204838813 ) ) ;
#17811=CARTESIAN_POINT ( 'NONE',  ( -9.999999999999998224, 1.224646799147353059E-15, -162.1250000040967905 ) ) ;
#17813=VECTOR ( 'NONE', #36736, 1000.000000000000000 ) ;
#17814=CARTESIAN_POINT ( 'NONE',  ( 5.405949406249999534, 9.363379034771803333, -185.5937500020483810 ) ) ;
#17818=CARTESIAN_POINT ( 'NONE',  ( 0.000000000000000000, 0.000000000000000000, -200.0000000000000000 ) ) ;
#17819=CARTESIAN_POINT ( 'NONE',  ( 4.999999999999992006, -8.660254037844389075, -104.2499999999999858 ) ) ;
#17820=CARTESIAN_POINT ( 'NONE',  ( -9.999999999999998224, 1.224646799147353059E-15, -200.0000000000000000 ) ) ;
#17821=CARTESIAN_POINT ( 'NONE',  ( -10.81189881249999729, 6.242252689847871849, -113.2187500020483952 ) ) ;
#17822=DIRECTION ( 'NONE',  ( 1.000000000000000000, 0.000000000000000000, 0.000000000000000000 ) ) ;
#17823=CARTESIAN_POINT ( 'NONE',  ( 5.405949406249992428, -9.363379034771808662, -84.28125000204838102 ) ) ;
#17824=CARTESIAN_POINT ( 'NONE',  ( 10.81189881249999729, 0.000000000000000000, -98.84375000204838102 ) ) ;
#17827=CARTESIAN_POINT ( 'NONE',  ( -2.121150477449813534E-15, -11.54700538379251284, -157.2500000040967620 ) ) ;
#17831=EDGE_CURVE ( 'NONE', #33370, #31274, #41249, .T. ) ;
#17834=CARTESIAN_POINT ( 'NONE',  ( 5.000000000000000000, 8.660254037844385522, -10.74999999999995381 ) ) ;
#17835=CARTESIAN_POINT ( 'NONE',  ( 9.999999999999998224, 0.000000000000000000, -75.49999999999998579 ) ) ;
#17837=CARTESIAN_POINT ( 'NONE',  ( -9.999999999999998224, 1.224646799147353059E-15, -81.12500000409677625 ) ) ;
#17838=CARTESIAN_POINT ( 'NONE',  ( -2.121150477449813534E-15, -11.54700538379251284, -142.2500000040967905 ) ) ;
#17840=CARTESIAN_POINT ( 'NONE',  ( 10.81189881249999729, 6.242252689847867408, -71.90625000204836681 ) ) ;
#17842=CARTESIAN_POINT ( 'NONE',  ( 9.999999999998456346, 5.773502691897149042, -21.37499999999993605 ) ) ;
#17845=CARTESIAN_POINT ( 'NONE',  ( -10.81189881249999729, 1.324075727343319199E-15, -198.7812500020484094 ) ) ;
#17847=CARTESIAN_POINT ( 'NONE',  ( 5.405949406249992428, -9.363379034771808662, -10.59375000204834727 ) ) ;
#17848=CARTESIAN_POINT ( 'NONE',  ( 9.999999999999479527, 5.773502691896553074, -142.8749999999999716 ) ) ;
#17850=CARTESIAN_POINT ( 'NONE',  ( 5.405949406249999534, 9.363379034771803333, -130.2812500020483810 ) ) ;
#17851=CARTESIAN_POINT ( 'NONE',  ( 5.000000000000000000, 8.660254037844385522, -183.2500000000000000 ) ) ;
#17852=CARTESIAN_POINT ( 'NONE',  ( -9.999999999999998224, 1.224646799147353059E-15, -109.2499999999999858 ) ) ;
#17853=AXIS2_PLACEMENT_3D ( 'NONE', #26031, #39184, #38769 ) ;
#17854=CARTESIAN_POINT ( 'NONE',  ( 10.81189881249999729, 0.000000000000000000, -106.5312500020483810 ) ) ;
#17855=ORIENTED_EDGE ( 'NONE', *, *, #7199, .T. ) ;
#17856=CARTESIAN_POINT ( 'NONE',  ( 9.999999999999998224, 0.000000000000000000, -200.0000000000000000 ) ) ;
#17857=VERTEX_POINT ( 'NONE', #18386 ) ;
#17858=EDGE_LOOP ( 'NONE', ( #7445, #35918, #42225, #41594 ) ) ;
#17859=VECTOR ( 'NONE', #3888, 1000.000000000000114 ) ;
#17860=CARTESIAN_POINT ( 'NONE',  ( 10.81189881249999907, 6.242252689847868297, -35.90625000204835260 ) ) ;
#17862=CARTESIAN_POINT ( 'NONE',  ( -5.405949406249996869, 9.363379034771805109, -84.84375000204836681 ) ) ;
#17864=CARTESIAN_POINT ( 'NONE',  ( -4.999999999999996447, 8.660254037844387298, -174.0000000000000284 ) ) ;
#17867=CARTESIAN_POINT ( 'NONE',  ( -5.000000000000003553, -8.660254037844383745, -68.49999999999997158 ) ) ;
#17868=CARTESIAN_POINT ( 'NONE',  ( 10.81189881249999729, 0.000000000000000000, -127.3437500020483952 ) ) ;
#17870=CARTESIAN_POINT ( 'NONE',  ( 10.81189881249999729, 6.242252689847867408, -1.406250002048370584 ) ) ;
#17873=CARTESIAN_POINT ( 'NONE',  ( -2.121150477449813534E-15, -11.54700538379251284, -178.2500000040967620 ) ) ;
#17875=CARTESIAN_POINT ( 'NONE',  ( 10.81189881249999729, 6.242252689847867408, -175.4062500020484094 ) ) ;
#17876=CARTESIAN_POINT ( 'NONE',  ( 10.00000000000102318, -5.773502691895667560, -28.00000000409675494 ) ) ;
#17877=CARTESIAN_POINT ( 'NONE',  ( 9.999999999999998224, 0.000000000000000000, -182.0000000000000000 ) ) ;
#17879=CARTESIAN_POINT ( 'NONE',  ( 10.81189881249999729, 6.242252689847867408, -49.21875000204835970 ) ) ;
#17881=CARTESIAN_POINT ( 'NONE',  ( 5.405949406249999534, 9.363379034771803333, -11.78125000204835438 ) ) ;
#17884=CARTESIAN_POINT ( 'NONE',  ( 10.00000000000000000, 5.773502691896255534, -96.37499999999998579 ) ) ;
#17886=CARTESIAN_POINT ( 'NONE',  ( 4.999999999999992006, -8.660254037844389075, -109.1250000040967763 ) ) ;
#17887=CARTESIAN_POINT ( 'NONE',  ( -9.999999999999998224, 1.224646799147353059E-15, -27.12500000409676204 ) ) ;
#17890=CARTESIAN_POINT ( 'NONE',  ( -10.81189881249999729, 6.242252689847871849, -101.4062500020483952 ) ) ;
#17891=VERTEX_POINT ( 'NONE', #21633 ) ;
#17894=CARTESIAN_POINT ( 'NONE',  ( -5.405949406250003975, -9.363379034771801557, -161.0312500020484094 ) ) ;
#17896=VERTEX_POINT ( 'NONE', #34811 ) ;
#17897=CARTESIAN_POINT ( 'NONE',  ( -4.999999999999996447, 8.660254037844387298, -22.49999999999996447 ) ) ;
#17899=CARTESIAN_POINT ( 'NONE',  ( -10.81189881249999729, 1.324075727343319199E-15, -32.28125000204837391 ) ) ;
#17900=CARTESIAN_POINT ( 'NONE',  ( 9.999999999999996447, -5.773502691896262640, -159.6250000000000284 ) ) ;
#17902=CARTESIAN_POINT ( 'NONE',  ( -5.000000000000003553, -8.660254037844383745, -92.49999999999998579 ) ) ;
#17903=( BOUNDED_CURVE ( )  B_SPLINE_CURVE ( 2, ( #40454, #10899, #14337, #11107, #28821, #2488, #25159 ),
 .UNSPECIFIED., .F., .F. ) 
 B_SPLINE_CURVE_WITH_KNOTS ( ( 3, 2, 2, 3 ),
 ( 0.1119402985074627876, 0.1131840796019901035, 0.1144278606965174333, 0.1156716417910447492 ),
 .UNSPECIFIED. ) 
 CURVE ( )  GEOMETRIC_REPRESENTATION_ITEM ( )  RATIONAL_B_SPLINE_CURVE ( ( 0.9999999999999894529, 0.8660254037844491437, 1.000000000000000000, 0.8660254037844387076, 1.000000000000000000, 0.8660254037844417052, 0.9999999999999970024 ) ) 
 REPRESENTATION_ITEM ( '' )  );
#17906=CARTESIAN_POINT ( 'NONE',  ( -5.405949406249996869, 9.363379034771805109, -133.0312500020484094 ) ) ;
#17907=CARTESIAN_POINT ( 'NONE',  ( 9.999999999999998224, 0.000000000000000000, -111.4999999999999858 ) ) ;
#17909=ORIENTED_EDGE ( 'NONE', *, *, #23720, .T. ) ;
#17910=CARTESIAN_POINT ( 'NONE',  ( 7.644554776091147741E-16, 12.48450537969573659, -64.15625000204838102 ) ) ;
#17911=VECTOR ( 'NONE', #2549, 1000.000000000000000 ) ;
#17913=ORIENTED_EDGE ( 'NONE', *, *, #598, .F. ) ;
#17914=CARTESIAN_POINT ( 'NONE',  ( 9.999999999999998224, 0.000000000000000000, -120.5000000000000000 ) ) ;
#17915=FACE_OUTER_BOUND ( 'NONE', #14099, .T. ) ;
#17916=CARTESIAN_POINT ( 'NONE',  ( -5.405949406249996869, 9.363379034771805109, -165.8437500020484094 ) ) ;
#17918=CARTESIAN_POINT ( 'NONE',  ( 7.644554776091147741E-16, 12.48450537969573659, -14.46875000204836859 ) ) ;
#17919=CYLINDRICAL_SURFACE ( 'NONE', #11556, 9.999999999999998224 ) ;
#17920=CARTESIAN_POINT ( 'NONE',  ( 5.405949406249992428, -9.363379034771808662, -151.5937500020483810 ) ) ;
#17921=CARTESIAN_POINT ( 'NONE',  ( -10.81189881249999729, 6.242252689847871849, -125.2187500020483810 ) ) ;
#17922=CARTESIAN_POINT ( 'NONE',  ( -5.405949406250003975, -9.363379034771801557, -105.5312500020483810 ) ) ;
#17924=CARTESIAN_POINT ( 'NONE',  ( 9.999999999999834799, 5.773502691896347905, -191.2500000040968473 ) ) ;
#17926=CARTESIAN_POINT ( 'NONE',  ( -5.405949406249996869, 9.363379034771805109, -2.343750002048366810 ) ) ;
#17929=CARTESIAN_POINT ( 'NONE',  ( 4.999999999999992006, -8.660254037844389075, -178.1250000040968189 ) ) ;
#17932=CARTESIAN_POINT ( 'NONE',  ( -10.81189881249999729, 1.324075727343319199E-15, -77.09375000204838102 ) ) ;
#17933=CARTESIAN_POINT ( 'NONE',  ( 10.81189881249999907, 6.242252689847868297, -62.71875000204838813 ) ) ;
#17934=LINE ( 'NONE', #40593, #24288 ) ;
#17935=CARTESIAN_POINT ( 'NONE',  ( 10.81189881249999729, 0.000000000000000000, -33.03125000204837391 ) ) ;
#17937=CYLINDRICAL_SURFACE ( 'NONE', #33701, 9.999999999999998224 ) ;
#17939=CARTESIAN_POINT ( 'NONE',  ( 7.070501591499377789E-16, 11.54700538379251284, -124.6249999999999858 ) ) ;
#17940=CARTESIAN_POINT ( 'NONE',  ( 10.81189881249999551, -6.242252689847874514, -130.6562500020483810 ) ) ;
#17941=CARTESIAN_POINT ( 'NONE',  ( 7.070501591499376803E-16, 11.54700538379251284, -94.62500000000000000 ) ) ;
#17943=CARTESIAN_POINT ( 'NONE',  ( -2.293366432827344421E-15, -12.48450537969573659, -10.90625000204838102 ) ) ;
#17944=ORIENTED_EDGE ( 'NONE', *, *, #41978, .T. ) ;
#17945=( BOUNDED_CURVE ( )  B_SPLINE_CURVE ( 2, ( #4365, #30699, #17504, #27815, #40309, #24375, #4501 ),
 .UNSPECIFIED., .F., .F. ) 
 B_SPLINE_CURVE_WITH_KNOTS ( ( 3, 2, 2, 3 ),
 ( 0.1604477611940298698, 0.1616915422885572551, 0.1629353233830845848, 0.1641791044776119424 ),
 .UNSPECIFIED. ) 
 CURVE ( )  GEOMETRIC_REPRESENTATION_ITEM ( )  RATIONAL_B_SPLINE_CURVE ( ( 0.9999999999999970024, 0.8660254037844417052, 1.000000000000000000, 0.8660254037844387076, 1.000000000000000000, 0.8660254037844387076, 1.000000000000000000 ) ) 
 REPRESENTATION_ITEM ( '' )  );
#17948=CARTESIAN_POINT ( 'NONE',  ( 4.999999999999992006, -8.660254037844389075, -56.62500000409676204 ) ) ;
#17949=CARTESIAN_POINT ( 'NONE',  ( -2.121150477449813534E-15, -11.54700538379251284, -34.25000000409674783 ) ) ;
#17952=( BOUNDED_CURVE ( )  B_SPLINE_CURVE ( 2, ( #41940, #39341, #32676, #5716, #25569, #32255, #42574 ),
 .UNSPECIFIED., .F., .F. ) 
 B_SPLINE_CURVE_WITH_KNOTS ( ( 3, 2, 2, 3 ),
 ( 0.8768656716417913000, 0.8781094527363186852, 0.8793532338308460705, 0.8805970149253734558 ),
 .UNSPECIFIED. ) 
 CURVE ( )  GEOMETRIC_REPRESENTATION_ITEM ( )  RATIONAL_B_SPLINE_CURVE ( ( 0.9999999999999761302, 0.8660254037844625774, 1.000000000000000000, 0.8660254037844387076, 1.000000000000000000, 0.8660254037844028474, 1.000000000000035971 ) ) 
 REPRESENTATION_ITEM ( '' )  );
#17953=CARTESIAN_POINT ( 'NONE',  ( 9.999999999999998224, 0.000000000000000000, -126.8750000040967905 ) ) ;
#17954=CARTESIAN_POINT ( 'NONE',  ( 5.405949406249999534, 9.363379034771803333, -151.2812500020484094 ) ) ;
#17955=CARTESIAN_POINT ( 'NONE',  ( -10.81189881249999729, 1.324075727343319199E-15, -125.0937500020483668 ) ) ;
#17956=CARTESIAN_POINT ( 'NONE',  ( 9.999999999999998224, 0.000000000000000000, -191.0000000000000000 ) ) ;
#17957=EDGE_CURVE ( 'NONE', #34507, #39040, #27049, .T. ) ;
#17958=EDGE_LOOP ( 'NONE', ( #40090, #22527, #38575, #15886 ) ) ;
#17959=CARTESIAN_POINT ( 'NONE',  ( 0.000000000000000000, 0.000000000000000000, -200.0000000000000000 ) ) ;
#17960=ORIENTED_EDGE ( 'NONE', *, *, #33366, .T. ) ;
#17962=ORIENTED_EDGE ( 'NONE', *, *, #39591, .F. ) ;
#17963=CARTESIAN_POINT ( 'NONE',  ( 9.999999999999998224, 0.000000000000000000, -189.5000000000000000 ) ) ;
#17964=CARTESIAN_POINT ( 'NONE',  ( 7.644554776091147741E-16, 12.48450537969573659, -189.9687500020484094 ) ) ;
#17966=CARTESIAN_POINT ( 'NONE',  ( 5.405949406249999534, 9.363379034771803333, -37.09375000204836681 ) ) ;
#17967=CARTESIAN_POINT ( 'NONE',  ( 2.944358404844418686, -10.14388074307273691, -1.167351363741249440E-15 ) ) ;
#17968=CARTESIAN_POINT ( 'NONE',  ( 9.999999999998456346, 5.773502691897149042, -14.25000000409672651 ) ) ;
#17969=CARTESIAN_POINT ( 'NONE',  ( -2.293366432827344421E-15, -12.48450537969573659, -171.2187500020483810 ) ) ;
#17970=CARTESIAN_POINT ( 'NONE',  ( -10.81189881249999729, 1.324075727343319199E-15, -161.0937500020484094 ) ) ;
#17971=CARTESIAN_POINT ( 'NONE',  ( -23.09401076758503280, 0.000000000000000000, 45.00000000000009237 ) ) ;
#17975=CARTESIAN_POINT ( 'NONE',  ( 9.999999999999998224, 0.000000000000000000, -93.49999999999998579 ) ) ;
#17978=CARTESIAN_POINT ( 'NONE',  ( 5.405949406249999534, 9.363379034771803333, -91.09375000204838102 ) ) ;
#17980=CARTESIAN_POINT ( 'NONE',  ( -10.81189881249999729, 1.324075727343319199E-15, -54.78125000204836681 ) ) ;
#17981=CARTESIAN_POINT ( 'NONE',  ( -5.000000000000003553, -8.660254037844383745, -16.37500000409675138 ) ) ;
#17983=CARTESIAN_POINT ( 'NONE',  ( 10.81189881249999907, 6.242252689847868297, -112.4062500020483952 ) ) ;
#17984=CARTESIAN_POINT ( 'NONE',  ( 10.81189881249999551, -6.242252689847874514, -156.1562500020483526 ) ) ;
#17985=CARTESIAN_POINT ( 'NONE',  ( -9.999999999999998224, 1.224646799147353059E-15, -182.7500000000000000 ) ) ;
#17987=CARTESIAN_POINT ( 'NONE',  ( 9.999999999999998224, 0.000000000000000000, -132.8750000040967905 ) ) ;
#17993=CARTESIAN_POINT ( 'NONE',  ( 5.405949406249992428, -9.363379034771808662, -181.7812500020483810 ) ) ;
#17994=ORIENTED_EDGE ( 'NONE', *, *, #29405, .F. ) ;
#17996=CARTESIAN_POINT ( 'NONE',  ( 4.999999999999992006, -8.660254037844389075, -56.62500000409676204 ) ) ;
#17998=CARTESIAN_POINT ( 'NONE',  ( -4.999999999999996447, 8.660254037844387298, -135.3750000040967905 ) ) ;
#18000=CARTESIAN_POINT ( 'NONE',  ( 10.81189881249999551, -6.242252689847874514, -54.15625000204837391 ) ) ;
#18003=CARTESIAN_POINT ( 'NONE',  ( 9.999999999999998224, 0.000000000000000000, -34.99999999999997868 ) ) ;
#18004=CARTESIAN_POINT ( 'NONE',  ( -5.405949406249996869, 9.363379034771805109, -179.5312500020483810 ) ) ;
#18006=ADVANCED_FACE ( 'NONE', ( #35235 ), #19234, .T. ) ;
#18008=DIRECTION ( 'NONE',  ( -0.000000000000000000, -0.000000000000000000, 1.000000000000000000 ) ) ;
#18009=EDGE_CURVE ( 'NONE', #22602, #6595, #36121, .T. ) ;
#18010=ORIENTED_EDGE ( 'NONE', *, *, #8704, .F. ) ;
#18011=CARTESIAN_POINT ( 'NONE',  ( 9.999999999999998224, 0.000000000000000000, -0.4999999999999726885 ) ) ;
#18013=CARTESIAN_POINT ( 'NONE',  ( -6.964452268037473637, 6.964452268037472749, -201.2186212422413689 ) ) ;
#18017=CARTESIAN_POINT ( 'NONE',  ( 10.81189881249999729, 0.000000000000000000, -84.03125000204838102 ) ) ;
#18018=VERTEX_POINT ( 'NONE', #9525 ) ;
#18019=CARTESIAN_POINT ( 'NONE',  ( 9.999999999999998224, 0.000000000000000000, -17.37500000409675138 ) ) ;
#18020=VERTEX_POINT ( 'NONE', #28550 ) ;
#18021=( BOUNDED_CURVE ( )  B_SPLINE_CURVE ( 2, ( #19068, #41512, #12364, #12155, #15175, #21882, #9354 ),
 .UNSPECIFIED., .F., .F. ) 
 B_SPLINE_CURVE_WITH_KNOTS ( ( 3, 2, 2, 3 ),
 ( 0.8470149253731346084, 0.8482587064676619937, 0.8495024875621892679, 0.8507462686567166532 ),
 .UNSPECIFIED. ) 
 CURVE ( )  GEOMETRIC_REPRESENTATION_ITEM ( )  RATIONAL_B_SPLINE_CURVE ( ( 0.9999999999999641398, 0.8660254037844745678, 1.000000000000000000, 0.8660254037844387076, 1.000000000000000000, 0.8660254037844148378, 1.000000000000023981 ) ) 
 REPRESENTATION_ITEM ( '' )  );
#18023=VERTEX_POINT ( 'NONE', #22695 ) ;
#18024=CARTESIAN_POINT ( 'NONE',  ( -10.81189881249999729, 6.242252689847871849, -33.71875000204834549 ) ) ;
#18026=CARTESIAN_POINT ( 'NONE',  ( 7.644554776091147741E-16, 12.48450537969573659, -17.65625000204836681 ) ) ;
#18027=CARTESIAN_POINT ( 'NONE',  ( -5.405949406250003975, -9.363379034771801557, -61.84375000204836681 ) ) ;
#18029=CARTESIAN_POINT ( 'NONE',  ( 5.000000000000000000, 8.660254037844385522, -28.74999999999997158 ) ) ;
#18031=CARTESIAN_POINT ( 'NONE',  ( 10.81189881249999551, -6.242252689847874514, -184.4687500020483810 ) ) ;
#18039=CARTESIAN_POINT ( 'NONE',  ( -2.293366432827344421E-15, -12.48450537969573659, -111.2187500020483668 ) ) ;
#18040=FACE_OUTER_BOUND ( 'NONE', #36544, .T. ) ;
#18041=CARTESIAN_POINT ( 'NONE',  ( 5.405949406249999534, 9.363379034771803333, -80.78125000204838102 ) ) ;
#18042=CARTESIAN_POINT ( 'NONE',  ( 10.81189881249999729, 0.000000000000000000, -88.34375000204838102 ) ) ;
#18045=CARTESIAN_POINT ( 'NONE',  ( -5.000000000000003553, -8.660254037844383745, -155.8750000040967905 ) ) ;
#18049=VECTOR ( 'NONE', #37022, 1000.000000000000000 ) ;
#18050=CYLINDRICAL_SURFACE ( 'NONE', #42652, 9.999999999999998224 ) ;
#18051=CARTESIAN_POINT ( 'NONE',  ( 7.070501591499376803E-16, 11.54700538379251284, -172.6249999999999716 ) ) ;
#18053=CARTESIAN_POINT ( 'NONE',  ( 9.999999999999479527, 5.773502691896553074, -42.75000000409674072 ) ) ;
#18054=CARTESIAN_POINT ( 'NONE',  ( 10.00000000000000000, 5.773502691896255534, -72.37499999999997158 ) ) ;
#18056=CARTESIAN_POINT ( 'NONE',  ( 9.999999999999998224, 0.000000000000000000, -78.87500000409677625 ) ) ;
#18057=EDGE_CURVE ( 'NONE', #8228, #12293, #6376, .T. ) ;
#18060=CARTESIAN_POINT ( 'NONE',  ( 7.644554776091147741E-16, 12.48450537969573659, -76.15625000204838102 ) ) ;
#18064=ORIENTED_EDGE ( 'NONE', *, *, #37845, .T. ) ;
#18065=CARTESIAN_POINT ( 'NONE',  ( 10.00000000000000000, 5.773502691896255534, -3.374999999999951594 ) ) ;
#18067=CARTESIAN_POINT ( 'NONE',  ( -5.405949406249996869, 9.363379034771805109, -14.34375000204834905 ) ) ;
#18070=CARTESIAN_POINT ( 'NONE',  ( -23.09401076758503280, 0.000000000000000000, 0.000000000000000000 ) ) ;
#18071=CARTESIAN_POINT ( 'NONE',  ( -5.405949406250003975, -9.363379034771801557, -129.5312500020484094 ) ) ;
#18073=( BOUNDED_CURVE ( )  B_SPLINE_CURVE ( 2, ( #40541, #4314, #36477, #33892, #36687, #7342, #16601 ),
 .UNSPECIFIED., .F., .F. ) 
 B_SPLINE_CURVE_WITH_KNOTS ( ( 3, 2, 2, 3 ),
 ( 0.5261194029850747578, 0.5273631840796021431, 0.5286069651741294173, 0.5298507462686568026 ),
 .UNSPECIFIED. ) 
 CURVE ( )  GEOMETRIC_REPRESENTATION_ITEM ( )  RATIONAL_B_SPLINE_CURVE ( ( 0.9999999999999880096, 0.8660254037844506980, 1.000000000000000000, 0.8660254037844387076, 1.000000000000000000, 0.8660254037844267172, 1.000000000000011990 ) ) 
 REPRESENTATION_ITEM ( '' )  );
#18074=CARTESIAN_POINT ( 'NONE',  ( 9.999999999999998224, 0.000000000000000000, -185.0000000000000000 ) ) ;
#18075=CARTESIAN_POINT ( 'NONE',  ( 9.999999999999998224, 0.000000000000000000, -152.3750000040967905 ) ) ;
#18076=CARTESIAN_POINT ( 'NONE',  ( 7.644554776091147741E-16, 12.48450537969573659, -106.1562500020483952 ) ) ;
#18077=ORIENTED_EDGE ( 'NONE', *, *, #22874, .F. ) ;
#18078=CARTESIAN_POINT ( 'NONE',  ( 5.000000000000000000, 8.660254037844385522, -195.2500000000000000 ) ) ;
#18079=EDGE_LOOP ( 'NONE', ( #9904, #26028, #12211, #1808 ) ) ;
#18081=CARTESIAN_POINT ( 'NONE',  ( 10.81189881249999907, 6.242252689847868297, -40.40625000204836681 ) ) ;
#18083=EDGE_CURVE ( 'NONE', #2342, #30674, #10765, .T. ) ;
#18084=CARTESIAN_POINT ( 'NONE',  ( -10.81189881249999729, 6.242252689847871849, -86.21875000204838102 ) ) ;
#18087=CARTESIAN_POINT ( 'NONE',  ( -9.999999999999998224, 1.224646799147353059E-15, -169.6250000040967905 ) ) ;
#18089=CARTESIAN_POINT ( 'NONE',  ( 9.999999999999998224, 0.000000000000000000, -67.99999999999997158 ) ) ;
#18090=CARTESIAN_POINT ( 'NONE',  ( -5.405949406250003975, -9.363379034771801557, -123.3437500020483952 ) ) ;
#18092=LINE ( 'NONE', #31287, #7478 ) ;
#18095=CARTESIAN_POINT ( 'NONE',  ( -5.000000000000003553, -8.660254037844383745, -178.3750000040967905 ) ) ;
#18096=CARTESIAN_POINT ( 'NONE',  ( 5.405949406249992428, -9.363379034771808662, -168.2812500020484094 ) ) ;
#18097=CARTESIAN_POINT ( 'NONE',  ( -2.121150477449813534E-15, -11.54700538379251284, -1.250000004096749384 ) ) ;
#18100=CARTESIAN_POINT ( 'NONE',  ( 10.81189881249999729, 6.242252689847867408, -52.21875000204837391 ) ) ;
#18102=CARTESIAN_POINT ( 'NONE',  ( -5.405949406250003975, -9.363379034771801557, -9.531250002048352599 ) ) ;
#18104=CARTESIAN_POINT ( 'NONE',  ( -9.999999999999998224, 1.224646799147353059E-15, -159.1250000040967905 ) ) ;
#18106=CARTESIAN_POINT ( 'NONE',  ( -2.121150477449813534E-15, -11.54700538379251284, -99.87500000000000000 ) ) ;
#18108=CARTESIAN_POINT ( 'NONE',  ( -9.999999999999998224, 5.773502691896259087, -109.7500000040967763 ) ) ;
#18109=LINE ( 'NONE', #41832, #29328 ) ;
#18112=CARTESIAN_POINT ( 'NONE',  ( 10.81189881249999551, -6.242252689847874514, -100.6562500020483952 ) ) ;
#18113=ORIENTED_EDGE ( 'NONE', *, *, #21754, .F. ) ;
#18115=DIRECTION ( 'NONE',  ( -0.000000000000000000, -0.000000000000000000, 1.000000000000000000 ) ) ;
#18116=CARTESIAN_POINT ( 'NONE',  ( -10.81189881249999907, -6.242252689847864744, -168.6562500020483810 ) ) ;
#18118=ORIENTED_EDGE ( 'NONE', *, *, #21578, .T. ) ;
#18119=CARTESIAN_POINT ( 'NONE',  ( 9.999999999999996447, -5.773502691896262640, -21.62499999999997158 ) ) ;
#18120=CARTESIAN_POINT ( 'NONE',  ( 5.405949406249992428, -9.363379034771808662, -25.78125000204836681 ) ) ;
#18121=CARTESIAN_POINT ( 'NONE',  ( -5.000000000000003553, -8.660254037844383745, -164.5000000000000000 ) ) ;
#18122=CARTESIAN_POINT ( 'NONE',  ( -2.121150477449813534E-15, -11.54700538379251284, -102.8749999999999858 ) ) ;
#18125=CARTESIAN_POINT ( 'NONE',  ( 7.644554776091147741E-16, 12.48450537969573659, -134.6562500020483810 ) ) ;
#18126=CARTESIAN_POINT ( 'NONE',  ( 6.220988656785935156, 8.439441497390092195, -8.678191841965558546E-15 ) ) ;
#18127=CARTESIAN_POINT ( 'NONE',  ( -5.000000000000003553, -8.660254037844383745, -188.5000000000000000 ) ) ;
#18128=VERTEX_POINT ( 'NONE', #26144 ) ;
#18129=CARTESIAN_POINT ( 'NONE',  ( -10.81189881249999729, 1.324075727343319199E-15, -60.78125000204836681 ) ) ;
#18130=ADVANCED_FACE ( 'NONE', ( #35447 ), #29176, .T. ) ;
#18135=PLANE ( 'NONE',  #15276 ) ;
#18136=CARTESIAN_POINT ( 'NONE',  ( -10.81189881249999729, 6.242252689847871849, -156.7187500020483810 ) ) ;
#18138=CARTESIAN_POINT ( 'NONE',  ( 7.644554776091147741E-16, 12.48450537969573659, -8.468750002048357928 ) ) ;
#18139=CARTESIAN_POINT ( 'NONE',  ( 9.999999999999998224, 0.000000000000000000, -42.87500000409677625 ) ) ;
#18140=CARTESIAN_POINT ( 'NONE',  ( 10.81189881249999551, -6.242252689847874514, -149.9687500020483810 ) ) ;
#18141=CARTESIAN_POINT ( 'NONE',  ( 7.644554776091147741E-16, 12.48450537969573659, -107.6562500020483810 ) ) ;
#18145=CARTESIAN_POINT ( 'NONE',  ( -5.405949406250003975, -9.363379034771801557, -1.843750002048366587 ) ) ;
#18148=CARTESIAN_POINT ( 'NONE',  ( -5.405949406249996869, 9.363379034771805109, -196.0312500020484094 ) ) ;
#18149=CARTESIAN_POINT ( 'NONE',  ( -9.999999999999998224, 1.224646799147353059E-15, -11.74999999999995559 ) ) ;
#18152=CARTESIAN_POINT ( 'NONE',  ( 10.81189881249999729, 6.242252689847867408, -77.71875000204838102 ) ) ;
#18153=CARTESIAN_POINT ( 'NONE',  ( -2.293366432827344421E-15, -12.48450537969573659, -58.71875000204836681 ) ) ;
#18155=CARTESIAN_POINT ( 'NONE',  ( -5.405949406249996869, 9.363379034771805109, -37.03125000204837391 ) ) ;
#18157=CARTESIAN_POINT ( 'NONE',  ( 5.000000000000000000, 8.660254037844385522, -136.7499999999999716 ) ) ;
#18159=CARTESIAN_POINT ( 'NONE',  ( 4.999999999999992006, -8.660254037844389075, -125.2500000000000000 ) ) ;
#18161=CARTESIAN_POINT ( 'NONE',  ( -2.121150477449813534E-15, -11.54700538379251284, -170.3750000000000000 ) ) ;
#18163=CARTESIAN_POINT ( 'NONE',  ( -10.81189881249999729, 1.324075727343319199E-15, -6.781250002048377468 ) ) ;
#18164=ORIENTED_EDGE ( 'NONE', *, *, #19331, .F. ) ;
#18169=CARTESIAN_POINT ( 'NONE',  ( 9.999999999999998224, 0.000000000000000000, -32.37500000409676204 ) ) ;
#18170=CARTESIAN_POINT ( 'NONE',  ( 9.999999999999998224, 0.000000000000000000, -200.0000000000000000 ) ) ;
#18173=DIRECTION ( 'NONE',  ( -0.000000000000000000, -0.000000000000000000, 1.000000000000000000 ) ) ;
#18174=CARTESIAN_POINT ( 'NONE',  ( 5.405949406249992428, -9.363379034771808662, -145.7812500020483810 ) ) ;
#18175=EDGE_CURVE ( 'NONE', #19929, #18454, #5453, .T. ) ;
#18176=CARTESIAN_POINT ( 'NONE',  ( -10.81189881249999729, 1.324075727343319199E-15, -128.0937500020483810 ) ) ;
#18177=DIRECTION ( 'NONE',  ( -0.000000000000000000, -0.000000000000000000, 1.000000000000000000 ) ) ;
#18181=ORIENTED_EDGE ( 'NONE', *, *, #9949, .F. ) ;
#18182=EDGE_LOOP ( 'NONE', ( #30074, #35294, #8158, #27109 ) ) ;
#18183=( BOUNDED_CURVE ( )  B_SPLINE_CURVE ( 2, ( #15314, #12698, #41641, #25893, #12077, #9485, #22653 ),
 .UNSPECIFIED., .F., .F. ) 
 B_SPLINE_CURVE_WITH_KNOTS ( ( 3, 2, 2, 3 ),
 ( 0.8843283582089555006, 0.8855721393034827749, 0.8868159203980102712, 0.8880597014925376564 ),
 .UNSPECIFIED. ) 
 CURVE ( )  GEOMETRIC_REPRESENTATION_ITEM ( )  RATIONAL_B_SPLINE_CURVE ( ( 0.9999999999999761302, 0.8660254037844625774, 1.000000000000000000, 0.8660254037844387076, 1.000000000000000000, 0.8660254037844028474, 1.000000000000035971 ) ) 
 REPRESENTATION_ITEM ( '' )  );
#18185=CARTESIAN_POINT ( 'NONE',  ( 10.81189881249999551, -6.242252689847874514, -184.4687500020483810 ) ) ;
#18186=CARTESIAN_POINT ( 'NONE',  ( -10.81189881249999907, -6.242252689847864744, -40.96875000204834549 ) ) ;
#18188=CARTESIAN_POINT ( 'NONE',  ( -10.81189881249999729, 6.242252689847871849, -174.7187500020484379 ) ) ;
#18189=CARTESIAN_POINT ( 'NONE',  ( -10.81189881249999729, 6.242252689847871849, -156.7187500020483810 ) ) ;
#18190=CARTESIAN_POINT ( 'NONE',  ( -9.999999999999479527, -5.773502691896549521, -76.50000000409674783 ) ) ;
#18196=CARTESIAN_POINT ( 'NONE',  ( -4.999999999999996447, 8.660254037844387298, -169.5000000000000000 ) ) ;
#18198=CARTESIAN_POINT ( 'NONE',  ( -5.405949406250003975, -9.363379034771801557, -78.34375000204838102 ) ) ;
#18200=CARTESIAN_POINT ( 'NONE',  ( 10.81189881249999551, -6.242252689847874514, -61.65625000204838813 ) ) ;
#18201=CARTESIAN_POINT ( 'NONE',  ( 9.999999999999998224, 0.000000000000000000, -64.99999999999997158 ) ) ;
#18204=CARTESIAN_POINT ( 'NONE',  ( 10.81189881249999907, 6.242252689847868297, -110.9062500020483952 ) ) ;
#18205=CARTESIAN_POINT ( 'NONE',  ( 10.81189881249999551, -6.242252689847874514, -154.6562500020484094 ) ) ;
#18206=CARTESIAN_POINT ( 'NONE',  ( 4.999999999999992006, -8.660254037844389075, -11.24999999999995381 ) ) ;
#18208=CARTESIAN_POINT ( 'NONE',  ( -10.00000000000000000, -5.773502691896251982, -132.0000000040967905 ) ) ;
#18210=ORIENTED_EDGE ( 'NONE', *, *, #17633, .T. ) ;
#18211=( BOUNDED_CURVE ( )  B_SPLINE_CURVE ( 2, ( #39408, #33383, #23662, #36390, #3597, #3377, #3802 ),
 .UNSPECIFIED., .F., .F. ) 
 B_SPLINE_CURVE_WITH_KNOTS ( ( 3, 2, 2, 3 ),
 ( 0.7910447761194031591, 0.7922885572139305443, 0.7935323383084578186, 0.7947761194029852039 ),
 .UNSPECIFIED. ) 
 CURVE ( )  GEOMETRIC_REPRESENTATION_ITEM ( )  RATIONAL_B_SPLINE_CURVE ( ( 0.9999999999999761302, 0.8660254037844625774, 1.000000000000000000, 0.8660254037844387076, 1.000000000000000000, 0.8660254037844267172, 1.000000000000011990 ) ) 
 REPRESENTATION_ITEM ( '' )  );
#18215=CARTESIAN_POINT ( 'NONE',  ( 10.81189881249999729, 0.000000000000000000, -181.5312500020483810 ) ) ;
#18216=ORIENTED_EDGE ( 'NONE', *, *, #22997, .F. ) ;
#18218=CARTESIAN_POINT ( 'NONE',  ( 10.00000000000000000, 5.773502691896255534, -59.25000000409676915 ) ) ;
#18225=CARTESIAN_POINT ( 'NONE',  ( -10.81189881249999729, 1.324075727343319199E-15, -165.7812500020484094 ) ) ;
#18227=CARTESIAN_POINT ( 'NONE',  ( -10.00000000000005329, 5.773502691896226224, -197.8750000000000000 ) ) ;
#18229=DIRECTION ( 'NONE',  ( -0.5000000000000007772, 0.8660254037844381525, 0.000000000000000000 ) ) ;
#18230=CARTESIAN_POINT ( 'NONE',  ( 9.999999999999998224, 0.000000000000000000, -105.8750000040967763 ) ) ;
#18231=DIRECTION ( 'NONE',  ( -0.000000000000000000, -0.000000000000000000, 1.000000000000000000 ) ) ;
#18232=CARTESIAN_POINT ( 'NONE',  ( -5.405949406249996869, 9.363379034771805109, -80.53125000204838102 ) ) ;
#18234=( NAMED_UNIT ( * ) SI_UNIT ( $, .STERADIAN. ) SOLID_ANGLE_UNIT ( ) );
#18235=DIRECTION ( 'NONE',  ( -0.000000000000000000, -0.000000000000000000, 1.000000000000000000 ) ) ;
#18237=ORIENTED_EDGE ( 'NONE', *, *, #9293, .F. ) ;
#18238=CARTESIAN_POINT ( 'NONE',  ( -2.293366432827344421E-15, -12.48450537969573659, -40.71875000204834549 ) ) ;
#18239=CARTESIAN_POINT ( 'NONE',  ( -9.999999999999742428, -5.773502691896402084, -187.1250000000000000 ) ) ;
#18240=CARTESIAN_POINT ( 'NONE',  ( 5.405949406249999534, 9.363379034771803333, -16.28125000204835970 ) ) ;
#18241=CARTESIAN_POINT ( 'NONE',  ( 10.81189881249999551, -6.242252689847874514, -61.46875000204838102 ) ) ;
#18242=ORIENTED_EDGE ( 'NONE', *, *, #3634, .F. ) ;
#18245=CARTESIAN_POINT ( 'NONE',  ( -5.405949406250003975, -9.363379034771801557, -195.3437500020484094 ) ) ;
#18246=CARTESIAN_POINT ( 'NONE',  ( -10.81189881249999729, 6.242252689847871849, -173.2187500020483810 ) ) ;
#18249=CARTESIAN_POINT ( 'NONE',  ( -9.999999999999998224, 1.224646799147353059E-15, -58.62500000409676204 ) ) ;
#18252=CARTESIAN_POINT ( 'NONE',  ( -10.81189881249999729, 6.242252689847871849, -114.7187500020483810 ) ) ;
#18254=CARTESIAN_POINT ( 'NONE',  ( 10.81189881249999907, 6.242252689847868297, -85.40625000204839523 ) ) ;
#18255=EDGE_CURVE ( 'NONE', #10744, #34185, #2855, .T. ) ;
#18256=CARTESIAN_POINT ( 'NONE',  ( 5.405949406249992428, -9.363379034771808662, -96.09375000204838102 ) ) ;
#18260=CARTESIAN_POINT ( 'NONE',  ( -9.999999999999998224, 5.773502691896259087, -154.7500000040967620 ) ) ;
#18264=CARTESIAN_POINT ( 'NONE',  ( 9.999999999999998224, 0.000000000000000000, -98.37500000409677625 ) ) ;
#18265=CARTESIAN_POINT ( 'NONE',  ( -2.121150477449813534E-15, -11.54700538379251284, -182.3750000000000000 ) ) ;
#18268=CARTESIAN_POINT ( 'NONE',  ( 10.00000000000000000, 5.773502691896255534, -63.37499999999998579 ) ) ;
#18270=CARTESIAN_POINT ( 'NONE',  ( 10.00000000000000000, 5.773502691896255534, -81.75000000409677625 ) ) ;
#18271=CARTESIAN_POINT ( 'NONE',  ( 9.999999999998969713, 5.773502691896851502, -26.25000000409674783 ) ) ;
#18273=CARTESIAN_POINT ( 'NONE',  ( -2.293366432827344421E-15, -12.48450537969573659, -76.90625000204839523 ) ) ;
#18275=FACE_OUTER_BOUND ( 'NONE', #24259, .T. ) ;
#18278=CARTESIAN_POINT ( 'NONE',  ( 5.000000000000000000, 8.660254037844385522, -4.749999999999976907 ) ) ;
#18280=CARTESIAN_POINT ( 'NONE',  ( -5.405949406249996869, 9.363379034771805109, -9.843750002048345493 ) ) ;
#18283=CARTESIAN_POINT ( 'NONE',  ( 5.405949406249992428, -9.363379034771808662, -141.0937500020483810 ) ) ;
#18286=CARTESIAN_POINT ( 'NONE',  ( 9.999999999999998224, 0.000000000000000000, -134.0000000000000000 ) ) ;
#18287=CARTESIAN_POINT ( 'NONE',  ( 10.81189881249999907, 6.242252689847868297, -130.4062500020483810 ) ) ;
#18288=AXIS2_PLACEMENT_3D ( 'NONE', #29808, #39289, #23328 ) ;
#18289=CARTESIAN_POINT ( 'NONE',  ( 9.999999999999996447, -5.773502691896262640, -183.6250000000000000 ) ) ;
#18290=CARTESIAN_POINT ( 'NONE',  ( 9.999999999999998224, 0.000000000000000000, -35.37500000409676915 ) ) ;
#18291=CARTESIAN_POINT ( 'NONE',  ( -5.405949406250003975, -9.363379034771801557, -105.5312500020483810 ) ) ;
#18292=ORIENTED_EDGE ( 'NONE', *, *, #38102, .F. ) ;
#18293=DIRECTION ( 'NONE',  ( -0.000000000000000000, -0.000000000000000000, 1.000000000000000000 ) ) ;
#18294=EDGE_CURVE ( 'NONE', #7309, #5725, #39718, .T. ) ;
#18295=ORIENTED_EDGE ( 'NONE', *, *, #18835, .F. ) ;
#18296=ORIENTED_EDGE ( 'NONE', *, *, #31197, .F. ) ;
#18297=CARTESIAN_POINT ( 'NONE',  ( -10.81189881249999907, -6.242252689847864744, -35.15625000204837391 ) ) ;
#18299=CARTESIAN_POINT ( 'NONE',  ( -2.293366432827344421E-15, -12.48450537969573659, -90.21875000204838102 ) ) ;
#18300=CARTESIAN_POINT ( 'NONE',  ( -9.999999999999998224, 1.224646799147353059E-15, -55.62500000409676204 ) ) ;
#18303=AXIS2_PLACEMENT_3D ( 'NONE', #39616, #36393, #41092 ) ;
#18306=CARTESIAN_POINT ( 'NONE',  ( -9.999999999999998224, 1.224646799147353059E-15, -100.2499999999999858 ) ) ;
#18307=CARTESIAN_POINT ( 'NONE',  ( -10.81189881249999729, 6.242252689847871849, -117.7187500020483952 ) ) ;
#18310=CARTESIAN_POINT ( 'NONE',  ( -10.81189881249999729, 1.324075727343319199E-15, -5.281250002048376579 ) ) ;
#18313=CARTESIAN_POINT ( 'NONE',  ( -4.999999999999996447, 8.660254037844387298, -180.3750000040967905 ) ) ;
#18314=CARTESIAN_POINT ( 'NONE',  ( -10.81189881249999729, 1.324075727343319199E-15, -170.2812500020484094 ) ) ;
#18315=EDGE_CURVE ( 'NONE', #16498, #15872, #19097, .T. ) ;
#18318=CARTESIAN_POINT ( 'NONE',  ( 5.405949406249992428, -9.363379034771808662, -45.09375000204837391 ) ) ;
#18319=ADVANCED_FACE ( 'NONE', ( #36909 ), #7355, .T. ) ;
#18321=CARTESIAN_POINT ( 'NONE',  ( -5.405949406250003975, -9.363379034771801557, -5.031250002048376579 ) ) ;
#18323=DIRECTION ( 'NONE',  ( -0.000000000000000000, -0.000000000000000000, 1.000000000000000000 ) ) ;
#18325=CARTESIAN_POINT ( 'NONE',  ( 9.999999999999998224, 0.000000000000000000, -100.9999999999999858 ) ) ;
#18327=CARTESIAN_POINT ( 'NONE',  ( -5.000000000000003553, -8.660254037844383745, -109.3750000040967763 ) ) ;
#18328=DIRECTION ( 'NONE',  ( -0.000000000000000000, -0.000000000000000000, 1.000000000000000000 ) ) ;
#18331=CARTESIAN_POINT ( 'NONE',  ( -2.293366432827344421E-15, -12.48450537969573659, -102.4062500020484094 ) ) ;
#18332=ORIENTED_EDGE ( 'NONE', *, *, #36970, .F. ) ;
#18333=( BOUNDED_CURVE ( )  B_SPLINE_CURVE ( 2, ( #9674, #19381, #36009, #22632, #19588, #25665, #35805 ),
 .UNSPECIFIED., .F., .F. ) 
 B_SPLINE_CURVE_WITH_KNOTS ( ( 3, 2, 2, 3 ),
 ( 0.6902985074626868389, 0.6915422885572141132, 0.6927860696517414985, 0.6940298507462688837 ),
 .UNSPECIFIED. ) 
 CURVE ( )  GEOMETRIC_REPRESENTATION_ITEM ( )  RATIONAL_B_SPLINE_CURVE ( ( 0.9999999999999761302, 0.8660254037844625774, 1.000000000000000000, 0.8660254037844387076, 1.000000000000000000, 0.8660254037844148378, 1.000000000000023981 ) ) 
 REPRESENTATION_ITEM ( '' )  );
#18335=CARTESIAN_POINT ( 'NONE',  ( 9.999999999999479527, 5.773502691896553074, -91.87499999999998579 ) ) ;
#18336=CARTESIAN_POINT ( 'NONE',  ( 10.81189881249999551, -6.242252689847874514, -157.6562500020484094 ) ) ;
#18339=CARTESIAN_POINT ( 'NONE',  ( 9.999999999999998224, 0.000000000000000000, -24.49999999999996447 ) ) ;
#18340=CARTESIAN_POINT ( 'NONE',  ( 7.644554776091147741E-16, 12.48450537969573659, -26.65625000204837747 ) ) ;
#18341=CARTESIAN_POINT ( 'NONE',  ( 4.999999999999992006, -8.660254037844389075, -159.7500000000000000 ) ) ;
#18342=DIRECTION ( 'NONE',  ( -0.000000000000000000, -0.000000000000000000, 1.000000000000000000 ) ) ;
#18346=CARTESIAN_POINT ( 'NONE',  ( -9.999999999999998224, 1.224646799147353059E-15, -81.12500000409677625 ) ) ;
#18347=CARTESIAN_POINT ( 'NONE',  ( 10.81189881249999551, -6.242252689847874514, -133.6562500020483810 ) ) ;
#18348=CARTESIAN_POINT ( 'NONE',  ( -9.999999999999998224, 1.224646799147353059E-15, -139.6250000040967905 ) ) ;
#18350=VERTEX_POINT ( 'NONE', #1953 ) ;
#18351=CARTESIAN_POINT ( 'NONE',  ( 5.405949406249999534, 9.363379034771803333, -58.28125000204836681 ) ) ;
#18355=CARTESIAN_POINT ( 'NONE',  ( 4.999999999999992006, -8.660254037844389075, -46.12500000409677625 ) ) ;
#18357=CARTESIAN_POINT ( 'NONE',  ( 5.405949406249999534, 9.363379034771803333, -160.0937500020484094 ) ) ;
#18359=CARTESIAN_POINT ( 'NONE',  ( 5.405949406249999534, 9.363379034771803333, -4.093750002048368586 ) ) ;
#18360=CARTESIAN_POINT ( 'NONE',  ( -10.81189881249999729, -6.242252689847864744, -136.9687500020483810 ) ) ;
#18361=CARTESIAN_POINT ( 'NONE',  ( 10.81189881249999907, 6.242252689847868297, -101.9062500020484094 ) ) ;
#18363=DIRECTION ( 'NONE',  ( -0.000000000000000000, -0.000000000000000000, 1.000000000000000000 ) ) ;
#18366=CARTESIAN_POINT ( 'NONE',  ( 10.81189881249999907, 6.242252689847868297, -4.218750002048367698 ) ) ;
#18368=CARTESIAN_POINT ( 'NONE',  ( 5.405949406249992428, -9.363379034771808662, -195.2812500020484094 ) ) ;
#18369=CARTESIAN_POINT ( 'NONE',  ( -9.999999999999479527, -5.773502691896549521, -6.000000004096727402 ) ) ;
#18372=CARTESIAN_POINT ( 'NONE',  ( 10.81189881249999729, 0.000000000000000000, -73.34375000204838102 ) ) ;
#18373=CARTESIAN_POINT ( 'NONE',  ( 10.81189881249999729, 0.000000000000000000, -56.84375000204835970 ) ) ;
#18375=CARTESIAN_POINT ( 'NONE',  ( -10.81189881249999907, -6.242252689847864744, -38.15625000204835260 ) ) ;
#18377=CARTESIAN_POINT ( 'NONE',  ( 5.000000000000000000, 8.660254037844385522, -53.12500000409675494 ) ) ;
#18379=CARTESIAN_POINT ( 'NONE',  ( -2.121150477449813534E-15, -11.54700538379251284, -122.3750000000000142 ) ) ;
#18383=CARTESIAN_POINT ( 'NONE',  ( -2.293366432827344421E-15, -12.48450537969573659, -12.40625000204835793 ) ) ;
#18386=CARTESIAN_POINT ( 'NONE',  ( 9.999999999999998224, 0.000000000000000000, -60.49999999999997158 ) ) ;
#18388=EDGE_CURVE ( 'NONE', #3950, #31053, #28065, .T. ) ;
#18389=CARTESIAN_POINT ( 'NONE',  ( -4.999999999999996447, 8.660254037844387298, -28.87500000409676204 ) ) ;
#18391=DIRECTION ( 'NONE',  ( -0.000000000000000000, -0.000000000000000000, 1.000000000000000000 ) ) ;
#18393=CARTESIAN_POINT ( 'NONE',  ( 0.000000000000000000, 0.000000000000000000, -200.0000000000000000 ) ) ;
#18394=CARTESIAN_POINT ( 'NONE',  ( 10.81189881249999907, 6.242252689847868297, -143.9062500020484094 ) ) ;
#18395=CARTESIAN_POINT ( 'NONE',  ( 7.644554776091147741E-16, 12.48450537969573659, -125.4687500020483952 ) ) ;
#18397=CARTESIAN_POINT ( 'NONE',  ( 9.999999999999998224, 0.000000000000000000, -0.4999999999999726885 ) ) ;
#18398=ORIENTED_EDGE ( 'NONE', *, *, #13277, .F. ) ;
#18400=VERTEX_POINT ( 'NONE', #1525 ) ;
#18401=ORIENTED_EDGE ( 'NONE', *, *, #34286, .T. ) ;
#18402=CARTESIAN_POINT ( 'NONE',  ( -9.999999999999998224, 1.224646799147353059E-15, -7.625000004096743389 ) ) ;
#18403=CARTESIAN_POINT ( 'NONE',  ( -5.405949406249996869, 9.363379034771805109, -183.8437500020483810 ) ) ;
#18404=CARTESIAN_POINT ( 'NONE',  ( -10.81189881249999729, 1.324075727343319199E-15, -32.09375000204836681 ) ) ;
#18406=CARTESIAN_POINT ( 'NONE',  ( 5.405949406249992428, -9.363379034771808662, -171.0937500020484094 ) ) ;
#18407=CARTESIAN_POINT ( 'NONE',  ( 10.81189881249999551, -6.242252689847874514, -149.9687500020483810 ) ) ;
#18408=CARTESIAN_POINT ( 'NONE',  ( 9.999999999999998224, 0.000000000000000000, -200.0000000000000000 ) ) ;
#18413=CARTESIAN_POINT ( 'NONE',  ( -10.00000000000025580, 5.773502691896109873, -157.3750000000000000 ) ) ;
#18415=CARTESIAN_POINT ( 'NONE',  ( -5.405949406250003975, -9.363379034771801557, -82.84375000204836681 ) ) ;
#18416=CARTESIAN_POINT ( 'NONE',  ( -10.00000000000001421, 5.773502691896249317, -198.2500000040967905 ) ) ;
#18417=CARTESIAN_POINT ( 'NONE',  ( -2.293366432827344421E-15, -12.48450537969573659, -58.90625000204838813 ) ) ;
#18420=CARTESIAN_POINT ( 'NONE',  ( 10.81189881249999907, 6.242252689847868297, -115.4062500020484094 ) ) ;
#18421=CARTESIAN_POINT ( 'NONE',  ( 7.644554776091147741E-16, 12.48450537969573659, -145.1562500020484094 ) ) ;
#18422=CYLINDRICAL_SURFACE ( 'NONE', #26166, 9.999999999999998224 ) ;
#18424=CARTESIAN_POINT ( 'NONE',  ( 9.999999999999996447, -5.773502691896262640, -119.5000000040967763 ) ) ;
#18430=CARTESIAN_POINT ( 'NONE',  ( 9.999999999999872102, 5.773502691896329253, -192.7500000040968473 ) ) ;
#18431=CARTESIAN_POINT ( 'NONE',  ( 10.81189881249999729, 0.000000000000000000, -177.0312500020483810 ) ) ;
#18434=CARTESIAN_POINT ( 'NONE',  ( -9.999999999999998224, 1.224646799147353059E-15, -49.62500000409675494 ) ) ;
#18435=DIRECTION ( 'NONE',  ( 1.000000000000000000, 0.000000000000000000, 0.000000000000000000 ) ) ;
#18440=CARTESIAN_POINT ( 'NONE',  ( -4.999999999999996447, 8.660254037844387298, -83.99999999999997158 ) ) ;
#18441=CARTESIAN_POINT ( 'NONE',  ( -10.81189881249999907, -6.242252689847864744, -168.6562500020483810 ) ) ;
#18443=CARTESIAN_POINT ( 'NONE',  ( 9.999999999999998224, 0.000000000000000000, -2.375000004096766482 ) ) ;
#18444=CARTESIAN_POINT ( 'NONE',  ( -2.121150477449813534E-15, -11.54700538379251284, -177.8750000000000000 ) ) ;
#18445=EDGE_CURVE ( 'NONE', #33430, #33047, #4480, .T. ) ;
#18446=ORIENTED_EDGE ( 'NONE', *, *, #6276, .F. ) ;
#18447=CARTESIAN_POINT ( 'NONE',  ( -2.121150477449813534E-15, -11.54700538379251284, -0.8749999999999721334 ) ) ;
#18450=CARTESIAN_POINT ( 'NONE',  ( -9.999999999999998224, 1.224646799147353059E-15, -20.74999999999996447 ) ) ;
#18451=CARTESIAN_POINT ( 'NONE',  ( 10.81189881249999729, 0.000000000000000000, -78.03125000204838102 ) ) ;
#18452=ORIENTED_EDGE ( 'NONE', *, *, #13647, .F. ) ;
#18454=VERTEX_POINT ( 'NONE', #27631 ) ;
#18455=CARTESIAN_POINT ( 'NONE',  ( -10.81189881249999729, -6.242252689847864744, -34.96875000204835260 ) ) ;
#18457=CARTESIAN_POINT ( 'NONE',  ( 9.999999999999994671, -5.773502691896262640, -170.5000000040967905 ) ) ;
#18458=CARTESIAN_POINT ( 'NONE',  ( 5.405949406249999534, 9.363379034771803333, -8.781250002048352599 ) ) ;
#18459=CARTESIAN_POINT ( 'NONE',  ( -5.405949406250003975, -9.363379034771801557, -55.84375000204835970 ) ) ;
#18460=ORIENTED_EDGE ( 'NONE', *, *, #5480, .T. ) ;
#18463=CARTESIAN_POINT ( 'NONE',  ( 10.81189881249999729, 0.000000000000000000, -196.3437500020484094 ) ) ;
#18464=CARTESIAN_POINT ( 'NONE',  ( -10.81189881249999729, 6.242252689847871849, -180.7187500020483810 ) ) ;
#18467=CARTESIAN_POINT ( 'NONE',  ( 9.999999999998969713, 5.773502691896851502, -18.75000000409674428 ) ) ;
#18468=( BOUNDED_CURVE ( )  B_SPLINE_CURVE ( 2, ( #34339, #40990, #36756, #41426, #11433, #24631, #14668 ),
 .UNSPECIFIED., .F., .F. ) 
 B_SPLINE_CURVE_WITH_KNOTS ( ( 3, 2, 2, 3 ),
 ( 0.8768656716417913000, 0.8781094527363186852, 0.8793532338308460705, 0.8805970149253734558 ),
 .UNSPECIFIED. ) 
 CURVE ( )  GEOMETRIC_REPRESENTATION_ITEM ( )  RATIONAL_B_SPLINE_CURVE ( ( 0.9999999999999761302, 0.8660254037844625774, 1.000000000000000000, 0.8660254037844387076, 1.000000000000000000, 0.8660254037844028474, 1.000000000000035971 ) ) 
 REPRESENTATION_ITEM ( '' )  );
#18471=CARTESIAN_POINT ( 'NONE',  ( 10.81189881249999907, 6.242252689847868297, -104.7187500020483810 ) ) ;
#18472=CARTESIAN_POINT ( 'NONE',  ( 0.000000000000000000, 0.000000000000000000, -200.0000000000000000 ) ) ;
#18474=CARTESIAN_POINT ( 'NONE',  ( -5.405949406249996869, 9.363379034771805109, -80.53125000204838102 ) ) ;
#18475=CARTESIAN_POINT ( 'NONE',  ( 10.81189881249999729, 0.000000000000000000, -95.84375000204838102 ) ) ;
#18477=CARTESIAN_POINT ( 'NONE',  ( 9.999999999999998224, 0.000000000000000000, -143.3750000040967905 ) ) ;
#18482=CARTESIAN_POINT ( 'NONE',  ( -9.999999999999998224, 1.224646799147353059E-15, -40.24999999999997868 ) ) ;
#18483=CARTESIAN_POINT ( 'NONE',  ( -9.999999999999996447, 5.773502691896259975, -172.3750000000000568 ) ) ;
#18486=CARTESIAN_POINT ( 'NONE',  ( 7.070501591499377789E-16, 11.54700538379251284, -66.12500000000000000 ) ) ;
#18488=CARTESIAN_POINT ( 'NONE',  ( -4.999999999999996447, 8.660254037844387298, -82.87500000409676204 ) ) ;
#18490=CARTESIAN_POINT ( 'NONE',  ( -9.999999999999998224, 1.224646799147353059E-15, -106.6250000040967763 ) ) ;
#18492=CARTESIAN_POINT ( 'NONE',  ( 5.405949406249992428, -9.363379034771808662, -72.28125000204838102 ) ) ;
#18497=CARTESIAN_POINT ( 'NONE',  ( -5.405949406250003975, -9.363379034771801557, -194.0312500020484094 ) ) ;
#18499=CARTESIAN_POINT ( 'NONE',  ( -2.293366432827344421E-15, -12.48450537969573659, -4.718750002048370362 ) ) ;
#18501=CARTESIAN_POINT ( 'NONE',  ( -5.405949406250003975, -9.363379034771801557, -145.8437500020483810 ) ) ;
#18502=CARTESIAN_POINT ( 'NONE',  ( 9.999999999999834799, 5.773502691896347905, -192.3750000000000284 ) ) ;
#18503=CARTESIAN_POINT ( 'NONE',  ( 23.09401076758504345, 1.040834085586084257E-14, 49.99999999999998579 ) ) ;
#18504=CARTESIAN_POINT ( 'NONE',  ( -9.999999999999998224, 5.773502691896259087, -170.8750000000000000 ) ) ;
#18505=CARTESIAN_POINT ( 'NONE',  ( 9.999999999999227285, 5.773502691896701400, -106.8749999999999432 ) ) ;
#18506=CARTESIAN_POINT ( 'NONE',  ( 10.81189881249999551, -6.242252689847874514, -100.6562500020483952 ) ) ;
#18507=EDGE_LOOP ( 'NONE', ( #28935, #31467, #22867, #41847 ) ) ;
#18511=ORIENTED_EDGE ( 'NONE', *, *, #1167, .F. ) ;
#18513=VERTEX_POINT ( 'NONE', #21360 ) ;
#18514=CARTESIAN_POINT ( 'NONE',  ( 10.81189881249999729, 0.000000000000000000, -28.53125000204837036 ) ) ;
#18516=CARTESIAN_POINT ( 'NONE',  ( 10.81189881249999729, 0.000000000000000000, -88.34375000204838102 ) ) ;
#18517=CARTESIAN_POINT ( 'NONE',  ( 10.00000000000102318, -5.773502691895667560, -4.000000004096737172 ) ) ;
#18518=CARTESIAN_POINT ( 'NONE',  ( 7.070501591499376803E-16, 11.54700538379251284, -126.1249999999999858 ) ) ;
#18519=CARTESIAN_POINT ( 'NONE',  ( -9.999999999999998224, 1.224646799147353059E-15, -200.0000000000000000 ) ) ;
#18521=CARTESIAN_POINT ( 'NONE',  ( -2.121150477449813534E-15, -11.54700538379251284, -13.25000000409675849 ) ) ;
#18523=CARTESIAN_POINT ( 'NONE',  ( -2.293366432827344421E-15, -12.48450537969573659, -114.2187500020483668 ) ) ;
#18527=CARTESIAN_POINT ( 'NONE',  ( -9.999999999999998224, 5.773502691896259087, -180.2500000040967905 ) ) ;
#18528=CARTESIAN_POINT ( 'NONE',  ( -2.293366432827344421E-15, -12.48450537969573659, -174.4062500020484379 ) ) ;
#18529=CARTESIAN_POINT ( 'NONE',  ( -9.999999999999998224, 1.224646799147353059E-15, -68.74999999999997158 ) ) ;
#18532=CARTESIAN_POINT ( 'NONE',  ( 10.81189881249999729, 6.242252689847867408, -46.21875000204838102 ) ) ;
#18534=CARTESIAN_POINT ( 'NONE',  ( -5.405949406250003975, -9.363379034771801557, -3.531250002048374803 ) ) ;
#18536=DIRECTION ( 'NONE',  ( 1.000000000000000000, 0.000000000000000000, 0.000000000000000000 ) ) ;
#18538=CARTESIAN_POINT ( 'NONE',  ( 9.999999999999996447, -5.773502691896262640, -90.62499999999998579 ) ) ;
#18540=CARTESIAN_POINT ( 'NONE',  ( -5.000000000000003553, -8.660254037844383745, -107.8750000040967763 ) ) ;
#18543=DIRECTION ( 'NONE',  ( 1.000000000000000000, 0.000000000000000000, 0.000000000000000000 ) ) ;
#18546=CARTESIAN_POINT ( 'NONE',  ( 5.405949406249999534, 9.363379034771803333, -98.78125000204839523 ) ) ;
#18547=ORIENTED_EDGE ( 'NONE', *, *, #41692, .T. ) ;
#18550=CARTESIAN_POINT ( 'NONE',  ( 10.81189881249999907, 6.242252689847868297, -155.9062500020484094 ) ) ;
#18552=VERTEX_POINT ( 'NONE', #34543 ) ;
#18553=CARTESIAN_POINT ( 'NONE',  ( 4.999999999999992006, -8.660254037844389075, -14.24999999999995737 ) ) ;
#18555=CARTESIAN_POINT ( 'NONE',  ( 5.405949406249992428, -9.363379034771808662, -30.28125000204837036 ) ) ;
#18556=CARTESIAN_POINT ( 'NONE',  ( 10.00000000000000000, 5.773502691896255534, -156.3749999999999716 ) ) ;
#18560=CARTESIAN_POINT ( 'NONE',  ( 10.81189881249999907, 6.242252689847868297, -124.4062500020483810 ) ) ;
#18561=DIRECTION ( 'NONE',  ( -0.000000000000000000, -0.000000000000000000, 1.000000000000000000 ) ) ;
#18562=EDGE_CURVE ( 'NONE', #8113, #14562, #7253, .T. ) ;
#18564=ORIENTED_EDGE ( 'NONE', *, *, #42227, .F. ) ;
#18566=CARTESIAN_POINT ( 'NONE',  ( -10.81189881249999729, 6.242252689847871849, -62.40625000204838813 ) ) ;
#18568=EDGE_CURVE ( 'NONE', #35978, #35357, #24917, .T. ) ;
#18569=CARTESIAN_POINT ( 'NONE',  ( -10.81189881249999907, -6.242252689847864744, -112.9687500020483810 ) ) ;
#18570=VERTEX_POINT ( 'NONE', #37119 ) ;
#18574=CARTESIAN_POINT ( 'NONE',  ( -9.999999999999998224, 1.224646799147353059E-15, -200.0000000000000000 ) ) ;
#18575=CARTESIAN_POINT ( 'NONE',  ( 7.644554776091147741E-16, 12.48450537969573659, -155.4687500020484094 ) ) ;
#18577=CARTESIAN_POINT ( 'NONE',  ( 5.405949406249992428, -9.363379034771808662, -9.093750002048345493 ) ) ;
#18578=CARTESIAN_POINT ( 'NONE',  ( -2.293366432827344421E-15, -12.48450537969573659, -138.2187500020483810 ) ) ;
#18580=CARTESIAN_POINT ( 'NONE',  ( -9.999999999999998224, 1.224646799147353059E-15, -55.24999999999996447 ) ) ;
#18582=CARTESIAN_POINT ( 'NONE',  ( 5.405949406249992428, -9.363379034771808662, -1.593750002048366365 ) ) ;
#18584=CARTESIAN_POINT ( 'NONE',  ( -5.405949406250003975, -9.363379034771801557, -197.0312500020484094 ) ) ;
#18585=( BOUNDED_CURVE ( )  B_SPLINE_CURVE ( 2, ( #15220, #25597, #38755, #22352, #35528, #35935, #42605 ),
 .UNSPECIFIED., .F., .F. ) 
 B_SPLINE_CURVE_WITH_KNOTS ( ( 3, 2, 2, 3 ),
 ( 0.7835820895522389584, 0.7848258706467662327, 0.7860696517412937290, 0.7873134328358211143 ),
 .UNSPECIFIED. ) 
 CURVE ( )  GEOMETRIC_REPRESENTATION_ITEM ( )  RATIONAL_B_SPLINE_CURVE ( ( 0.9999999999999880096, 0.8660254037844506980, 1.000000000000000000, 0.8660254037844387076, 1.000000000000000000, 0.8660254037844148378, 1.000000000000023981 ) ) 
 REPRESENTATION_ITEM ( '' )  );
#18589=EDGE_CURVE ( 'NONE', #11765, #16918, #11649, .T. ) ;
#18590=CARTESIAN_POINT ( 'NONE',  ( -5.405949406250003975, -9.363379034771801557, -69.34375000204836681 ) ) ;
#18591=CARTESIAN_POINT ( 'NONE',  ( 10.81189881249999907, 6.242252689847868297, -53.71875000204838102 ) ) ;
#18593=CARTESIAN_POINT ( 'NONE',  ( 10.81189881249999729, 0.000000000000000000, -25.53125000204836681 ) ) ;
#18596=CARTESIAN_POINT ( 'NONE',  ( -2.121150477449813534E-15, -11.54700538379251284, -110.3749999999999858 ) ) ;
#18600=CARTESIAN_POINT ( 'NONE',  ( 10.81189881249999551, -6.242252689847874514, -12.15625000204835615 ) ) ;
#18601=ORIENTED_EDGE ( 'NONE', *, *, #15615, .F. ) ;
#18605=CARTESIAN_POINT ( 'NONE',  ( -10.00000000000000000, -5.773502691896251982, -47.62499999999997158 ) ) ;
#18606=CARTESIAN_POINT ( 'NONE',  ( -2.121150477449813534E-15, -11.54700538379251284, -26.75000000409677270 ) ) ;
#18607=CARTESIAN_POINT ( 'NONE',  ( 9.999999999999998224, 0.000000000000000000, -2.375000004096766482 ) ) ;
#18609=CARTESIAN_POINT ( 'NONE',  ( -10.81189881249999907, -6.242252689847864744, -147.6562500020483810 ) ) ;
#18610=AXIS2_PLACEMENT_3D ( 'NONE', #37725, #5142, #24366 ) ;
#18611=CARTESIAN_POINT ( 'NONE',  ( 10.81189881249999907, 6.242252689847868297, -152.9062500020483810 ) ) ;
#18612=CARTESIAN_POINT ( 'NONE',  ( -5.000000000000003553, -8.660254037844383745, -65.49999999999997158 ) ) ;
#18614=EDGE_LOOP ( 'NONE', ( #39357, #38341, #29722, #38468 ) ) ;
#18615=VERTEX_POINT ( 'NONE', #12482 ) ;
#18616=CARTESIAN_POINT ( 'NONE',  ( 4.999999999999992006, -8.660254037844389075, -7.125000004096743389 ) ) ;
#18617=CARTESIAN_POINT ( 'NONE',  ( 5.405949406249992428, -9.363379034771808662, -178.5937500020484094 ) ) ;
#18618=CARTESIAN_POINT ( 'NONE',  ( 5.405949406249999534, 9.363379034771803333, -28.09375000204836326 ) ) ;
#18620=CARTESIAN_POINT ( 'NONE',  ( 4.999999999999992006, -8.660254037844389075, -41.24999999999997868 ) ) ;
#18621=CARTESIAN_POINT ( 'NONE',  ( 5.405949406249992428, -9.363379034771808662, -166.5937500020484094 ) ) ;
#18622=CARTESIAN_POINT ( 'NONE',  ( 5.405949406249999534, 9.363379034771803333, -149.5937500020483810 ) ) ;
#18627=CARTESIAN_POINT ( 'NONE',  ( 7.070501591499376803E-16, 11.54700538379251284, -129.1250000000000000 ) ) ;
#18628=DIRECTION ( 'NONE',  ( -0.000000000000000000, -0.000000000000000000, 1.000000000000000000 ) ) ;
#18631=CARTESIAN_POINT ( 'NONE',  ( 7.644554776091147741E-16, 12.48450537969573659, -84.96875000204835260 ) ) ;
#18632=FACE_OUTER_BOUND ( 'NONE', #9174, .T. ) ;
#18633=CARTESIAN_POINT ( 'NONE',  ( -10.81189881249999907, -6.242252689847864744, -50.15625000204837391 ) ) ;
#18636=CARTESIAN_POINT ( 'NONE',  ( 5.405949406249992428, -9.363379034771808662, -112.7812500020483952 ) ) ;
#18637=CARTESIAN_POINT ( 'NONE',  ( -10.81189881249999729, 6.242252689847871849, -146.4062500020484094 ) ) ;
#18638=CARTESIAN_POINT ( 'NONE',  ( -10.00000000000051337, 5.773502691895962435, -142.7500000040967905 ) ) ;
#18640=CARTESIAN_POINT ( 'NONE',  ( 10.00000000000000000, 5.773502691896255534, -125.2500000040967905 ) ) ;
#18642=ORIENTED_EDGE ( 'NONE', *, *, #22547, .T. ) ;
#18645=CARTESIAN_POINT ( 'NONE',  ( 7.070501591499376803E-16, 11.54700538379251284, -184.6250000000000000 ) ) ;
#18646=CARTESIAN_POINT ( 'NONE',  ( -10.81189881249999729, 1.324075727343319199E-15, -182.2812500020483810 ) ) ;
#18648=CARTESIAN_POINT ( 'NONE',  ( -2.121150477449813534E-15, -11.54700538379251284, -50.75000000409676204 ) ) ;
#18649=FACE_OUTER_BOUND ( 'NONE', #3753, .T. ) ;
#18652=CARTESIAN_POINT ( 'NONE',  ( -5.405949406249996869, 9.363379034771805109, -169.0312500020484094 ) ) ;
#18653=CARTESIAN_POINT ( 'NONE',  ( -4.999999999999996447, 8.660254037844387298, -7.499999999999978684 ) ) ;
#18654=DIRECTION ( 'NONE',  ( 1.000000000000000000, 0.000000000000000000, 0.000000000000000000 ) ) ;
#18657=CARTESIAN_POINT ( 'NONE',  ( -9.999999999998969713, -5.773502691896847949, -52.50000000409674072 ) ) ;
#18660=CARTESIAN_POINT ( 'NONE',  ( -10.81189881249999907, -6.242252689847864744, -78.65625000204839523 ) ) ;
#18661=ORIENTED_EDGE ( 'NONE', *, *, #39253, .F. ) ;
#18662=AXIS2_PLACEMENT_3D ( 'NONE', #42423, #29492, #23018 ) ;
#18664=ORIENTED_EDGE ( 'NONE', *, *, #13238, .T. ) ;
#18666=CARTESIAN_POINT ( 'NONE',  ( -5.405949406249996869, 9.363379034771805109, -32.34375000204836681 ) ) ;
#18668=CARTESIAN_POINT ( 'NONE',  ( 5.405949406249992428, -9.363379034771808662, -3.281250002048374803 ) ) ;
#18669=CARTESIAN_POINT ( 'NONE',  ( -5.405949406249996869, 9.363379034771805109, -57.84375000204835970 ) ) ;
#18671=DIRECTION ( 'NONE',  ( 0.4999999999999997780, 0.8660254037844388186, 0.000000000000000000 ) ) ;
#18673=CARTESIAN_POINT ( 'NONE',  ( 10.81189881249999729, 6.242252689847867408, -184.2187500020483810 ) ) ;
#18674=CARTESIAN_POINT ( 'NONE',  ( 10.81189881249999551, -6.242252689847874514, -178.4687500020484094 ) ) ;
#18677=DIRECTION ( 'NONE',  ( -0.000000000000000000, -0.000000000000000000, 1.000000000000000000 ) ) ;
#18680=CARTESIAN_POINT ( 'NONE',  ( 5.405949406249999534, 9.363379034771803333, -101.5937500020483810 ) ) ;
#18681=CARTESIAN_POINT ( 'NONE',  ( -5.000000000000003553, -8.660254037844383745, -84.99999999999997158 ) ) ;
#18682=CARTESIAN_POINT ( 'NONE',  ( -5.405949406250003975, -9.363379034771801557, -71.03125000204838102 ) ) ;
#18683=CARTESIAN_POINT ( 'NONE',  ( 10.81189881249999729, 6.242252689847867408, -94.21875000204838102 ) ) ;
#18685=CARTESIAN_POINT ( 'NONE',  ( 7.070501591499377789E-16, 11.54700538379251284, -143.0000000040967905 ) ) ;
#18693=DIRECTION ( 'NONE',  ( -0.000000000000000000, -0.000000000000000000, 1.000000000000000000 ) ) ;
#18696=ORIENTED_EDGE ( 'NONE', *, *, #2253, .T. ) ;
#18697=CARTESIAN_POINT ( 'NONE',  ( -5.000000000000003553, -8.660254037844383745, -68.49999999999997158 ) ) ;
#18699=CARTESIAN_POINT ( 'NONE',  ( 9.999999999999996447, -5.773502691896262640, -77.50000000409677625 ) ) ;
#18701=CARTESIAN_POINT ( 'NONE',  ( 9.999999999999998224, 0.000000000000000000, -11.37500000409674783 ) ) ;
#18703=CARTESIAN_POINT ( 'NONE',  ( 10.81189881249999551, -6.242252689847874514, -67.65625000204839523 ) ) ;
#18704=( BOUNDED_CURVE ( )  B_SPLINE_CURVE ( 2, ( #2750, #21955, #29283, #35972, #35561, #9007, #25215 ),
 .UNSPECIFIED., .F., .F. ) 
 B_SPLINE_CURVE_WITH_KNOTS ( ( 3, 2, 2, 3 ),
 ( 0.05970149253731348721, 0.06094527363184085167, 0.06218905472636821613, 0.06343283582089558059 ),
 .UNSPECIFIED. ) 
 CURVE ( )  GEOMETRIC_REPRESENTATION_ITEM ( )  RATIONAL_B_SPLINE_CURVE ( ( 0.9999999999999940048, 0.8660254037844447028, 1.000000000000000000, 0.8660254037844387076, 1.000000000000000000, 0.8660254037844327124, 1.000000000000005995 ) ) 
 REPRESENTATION_ITEM ( '' )  );
#18706=LINE ( 'NONE', #5770, #16933 ) ;
#18708=CARTESIAN_POINT ( 'NONE',  ( 9.999999999999998224, 0.000000000000000000, -182.0000000000000000 ) ) ;
#18709=CARTESIAN_POINT ( 'NONE',  ( -5.405949406250003975, -9.363379034771801557, -191.0312500020484094 ) ) ;
#18712=CARTESIAN_POINT ( 'NONE',  ( -10.81189881249999729, 1.324075727343319199E-15, -2.093750002048366810 ) ) ;
#18713=CARTESIAN_POINT ( 'NONE',  ( 9.999999999999998224, 0.000000000000000000, -149.3750000040967905 ) ) ;
#18714=CARTESIAN_POINT ( 'NONE',  ( -10.00000000000015987, 5.773502691896167605, -191.8750000000000000 ) ) ;
#18715=CARTESIAN_POINT ( 'NONE',  ( -2.121150477449813534E-15, -11.54700538379251284, -173.3750000000000000 ) ) ;
#18716=CARTESIAN_POINT ( 'NONE',  ( 4.999999999999992006, -8.660254037844389075, -174.7500000000000284 ) ) ;
#18717=CARTESIAN_POINT ( 'NONE',  ( -9.999999999998969713, -5.773502691896847949, -37.12499999999993605 ) ) ;
#18718=CARTESIAN_POINT ( 'NONE',  ( -5.405949406249996869, 9.363379034771805109, -103.0312500020483952 ) ) ;
#18719=VERTEX_POINT ( 'NONE', #25471 ) ;
#18725=CARTESIAN_POINT ( 'NONE',  ( 5.405949406249992428, -9.363379034771808662, -33.28125000204837391 ) ) ;
#18727=CARTESIAN_POINT ( 'NONE',  ( 10.81189881249999551, -6.242252689847874514, -76.46875000204838102 ) ) ;
#18729=CARTESIAN_POINT ( 'NONE',  ( -5.405949406250003975, -9.363379034771801557, -198.3437500020484094 ) ) ;
#18732=CARTESIAN_POINT ( 'NONE',  ( -2.121150477449813534E-15, -11.54700538379251284, -11.75000000409676737 ) ) ;
#18734=CARTESIAN_POINT ( 'NONE',  ( -9.999999999999998224, 1.224646799147353059E-15, -91.62500000409677625 ) ) ;
#18735=CARTESIAN_POINT ( 'NONE',  ( -2.293366432827344421E-15, -12.48450537969573659, -127.7187500020483668 ) ) ;
#18736=CARTESIAN_POINT ( 'NONE',  ( 5.405949406249999534, 9.363379034771803333, -115.0937500020483810 ) ) ;
#18740=CARTESIAN_POINT ( 'NONE',  ( -5.000000000000003553, -8.660254037844383745, -170.8750000040968189 ) ) ;
#18741=CARTESIAN_POINT ( 'NONE',  ( -5.405949406250003975, -9.363379034771801557, -170.0312500020484094 ) ) ;
#18742=CARTESIAN_POINT ( 'NONE',  ( 4.999999999999992006, -8.660254037844389075, -70.12500000409677625 ) ) ;
#18745=CARTESIAN_POINT ( 'NONE',  ( 10.81189881249999729, 0.000000000000000000, -47.84375000204838102 ) ) ;
#18747=CARTESIAN_POINT ( 'NONE',  ( 10.81189881249999729, 0.000000000000000000, -4.531250002048375691 ) ) ;
#18749=CARTESIAN_POINT ( 'NONE',  ( -9.999999999999998224, 1.224646799147353059E-15, -5.749999999999976907 ) ) ;
#18751=EDGE_CURVE ( 'NONE', #30149, #29666, #30713, .T. ) ;
#18752=CARTESIAN_POINT ( 'NONE',  ( -10.00000000000000000, -5.773502691896251982, -86.62499999999997158 ) ) ;
#18754=CARTESIAN_POINT ( 'NONE',  ( -2.121150477449813534E-15, -11.54700538379251284, -94.25000000409677625 ) ) ;
#18757=CARTESIAN_POINT ( 'NONE',  ( 10.81189881249999729, 6.242252689847867408, -101.9062500020483952 ) ) ;
#18758=ORIENTED_EDGE ( 'NONE', *, *, #39117, .T. ) ;
#18762=CARTESIAN_POINT ( 'NONE',  ( -10.81189881249999729, 6.242252689847871849, -156.9062500020483810 ) ) ;
#18764=ORIENTED_EDGE ( 'NONE', *, *, #30335, .T. ) ;
#18765=CARTESIAN_POINT ( 'NONE',  ( 5.000000000000000000, 8.660254037844385522, -18.24999999999996092 ) ) ;
#18766=CARTESIAN_POINT ( 'NONE',  ( 5.405949406249992428, -9.363379034771808662, -28.78125000204837036 ) ) ;
#18767=CARTESIAN_POINT ( 'NONE',  ( -4.999999999999996447, 8.660254037844387298, -153.0000000000000000 ) ) ;
#18769=VECTOR ( 'NONE', #19600, 1000.000000000000000 ) ;
#18770=CARTESIAN_POINT ( 'NONE',  ( 4.999999999999992006, -8.660254037844389075, -198.7500000000000000 ) ) ;
#18771=CARTESIAN_POINT ( 'NONE',  ( 7.644554776091147741E-16, 12.48450537969573659, -125.6562500020483810 ) ) ;
#18776=CARTESIAN_POINT ( 'NONE',  ( 5.405949406249992428, -9.363379034771808662, -54.28125000204836681 ) ) ;
#18778=CARTESIAN_POINT ( 'NONE',  ( -5.405949406249996869, 9.363379034771805109, -102.8437500020483810 ) ) ;
#18779=VERTEX_POINT ( 'NONE', #8847 ) ;
#18780=VERTEX_POINT ( 'NONE', #18974 ) ;
#18781=CARTESIAN_POINT ( 'NONE',  ( -9.999999999999998224, 1.224646799147353059E-15, -175.6250000040968189 ) ) ;
#18783=CARTESIAN_POINT ( 'NONE',  ( -5.405949406250003975, -9.363379034771801557, -159.3437500020484094 ) ) ;
#18785=CARTESIAN_POINT ( 'NONE',  ( -5.405949406250003975, -9.363379034771801557, -4.843750002048369474 ) ) ;
#18786=CARTESIAN_POINT ( 'NONE',  ( -5.000000000000003553, -8.660254037844383745, -74.49999999999998579 ) ) ;
#18787=CARTESIAN_POINT ( 'NONE',  ( -10.81189881249999729, 1.324075727343319199E-15, -141.5937500020483810 ) ) ;
#18788=( BOUNDED_CURVE ( )  B_SPLINE_CURVE ( 2, ( #37403, #17526, #14277, #7846, #27481, #34181, #5681 ),
 .UNSPECIFIED., .F., .F. ) 
 B_SPLINE_CURVE_WITH_KNOTS ( ( 3, 2, 2, 3 ),
 ( 0.8358208955223882519, 0.8370646766169156372, 0.8383084577114430225, 0.8395522388059704078 ),
 .UNSPECIFIED. ) 
 CURVE ( )  GEOMETRIC_REPRESENTATION_ITEM ( )  RATIONAL_B_SPLINE_CURVE ( ( 0.9999999999999761302, 0.8660254037844625774, 1.000000000000000000, 0.8660254037844387076, 1.000000000000000000, 0.8660254037844148378, 1.000000000000023981 ) ) 
 REPRESENTATION_ITEM ( '' )  );
#18790=CARTESIAN_POINT ( 'NONE',  ( 9.999999999999998224, 0.000000000000000000, -191.3750000040967905 ) ) ;
#18792=CARTESIAN_POINT ( 'NONE',  ( -10.00000000000000000, -5.773502691896251982, -198.0000000040968189 ) ) ;
#18794=CARTESIAN_POINT ( 'NONE',  ( 10.81189881249999729, 6.242252689847867408, -193.4062500020484094 ) ) ;
#18798=VECTOR ( 'NONE', #16990, 1000.000000000000000 ) ;
#18799=CARTESIAN_POINT ( 'NONE',  ( 10.81189881249999729, 0.000000000000000000, -67.34375000204836681 ) ) ;
#18800=CARTESIAN_POINT ( 'NONE',  ( -2.293366432827344421E-15, -12.48450537969573659, -55.71875000204837391 ) ) ;
#18802=CARTESIAN_POINT ( 'NONE',  ( -10.81189881249999729, 1.324075727343319199E-15, -29.28125000204837036 ) ) ;
#18804=CARTESIAN_POINT ( 'NONE',  ( 9.999999999999998224, 0.000000000000000000, -32.37500000409676204 ) ) ;
#18807=CARTESIAN_POINT ( 'NONE',  ( 10.00000000000000000, 5.773502691896255534, -117.3750000000000000 ) ) ;
#18810=ADVANCED_FACE ( 'NONE', ( #39038 ), #19391, .T. ) ;
#18813=CARTESIAN_POINT ( 'NONE',  ( -5.405949406249996869, 9.363379034771805109, -10.03125000204835260 ) ) ;
#18816=CARTESIAN_POINT ( 'NONE',  ( -9.999999999999998224, 1.224646799147353059E-15, -83.74999999999997158 ) ) ;
#18818=CARTESIAN_POINT ( 'NONE',  ( 4.999999999999992006, -8.660254037844389075, -38.62500000409676915 ) ) ;
#18820=CARTESIAN_POINT ( 'NONE',  ( -4.999999999999996447, 8.660254037844387298, -38.99999999999997868 ) ) ;
#18821=CARTESIAN_POINT ( 'NONE',  ( -10.00000000000000000, -5.773502691896251982, -24.00000000409677625 ) ) ;
#18822=CARTESIAN_POINT ( 'NONE',  ( -10.81189881249999729, -6.242252689847864744, -50.15625000204837391 ) ) ;
#18826=CARTESIAN_POINT ( 'NONE',  ( 5.405949406249992428, -9.363379034771808662, -141.2812500020483810 ) ) ;
#18827=CARTESIAN_POINT ( 'NONE',  ( 10.81189881249999551, -6.242252689847874514, -147.1562500020484094 ) ) ;
#18829=EDGE_CURVE ( 'NONE', #26311, #27538, #20730, .T. ) ;
#18830=CARTESIAN_POINT ( 'NONE',  ( -9.999999999999998224, 1.224646799147353059E-15, -200.0000000000000000 ) ) ;
#18831=ORIENTED_EDGE ( 'NONE', *, *, #4082, .T. ) ;
#18833=VERTEX_POINT ( 'NONE', #7089 ) ;
#18834=ORIENTED_EDGE ( 'NONE', *, *, #32055, .T. ) ;
#18835=EDGE_CURVE ( 'NONE', #8170, #4745, #20239, .T. ) ;
#18836=DIRECTION ( 'NONE',  ( -0.000000000000000000, -0.000000000000000000, 1.000000000000000000 ) ) ;
#18838=CARTESIAN_POINT ( 'NONE',  ( 10.81189881249999551, -6.242252689847874514, -179.9687500020484094 ) ) ;
#18839=CARTESIAN_POINT ( 'NONE',  ( -2.293366432827344421E-15, -12.48450537969573659, -30.21875000204834905 ) ) ;
#18840=LINE ( 'NONE', #32231, #6734 ) ;
#18841=CARTESIAN_POINT ( 'NONE',  ( -5.405949406249996869, 9.363379034771805109, -162.8437500020484094 ) ) ;
#18842=CARTESIAN_POINT ( 'NONE',  ( 10.81189881249999551, -6.242252689847874514, -154.4687500020484094 ) ) ;
#18844=CARTESIAN_POINT ( 'NONE',  ( 9.999999999999998224, 0.000000000000000000, -89.37500000409677625 ) ) ;
#18849=CARTESIAN_POINT ( 'NONE',  ( -9.999999999999998224, 1.224646799147353059E-15, -200.0000000000000000 ) ) ;
#18850=( BOUNDED_CURVE ( )  B_SPLINE_CURVE ( 2, ( #30888, #11443, #27647, #1975, #18355, #11654, #24854 ),
 .UNSPECIFIED., .F., .F. ) 
 B_SPLINE_CURVE_WITH_KNOTS ( ( 3, 2, 2, 3 ),
 ( 0.7574626865671643117, 0.7587064676616916969, 0.7599502487562190822, 0.7611940298507464675 ),
 .UNSPECIFIED. ) 
 CURVE ( )  GEOMETRIC_REPRESENTATION_ITEM ( )  RATIONAL_B_SPLINE_CURVE ( ( 0.9999999999999880096, 0.8660254037844506980, 1.000000000000000000, 0.8660254037844387076, 1.000000000000000000, 0.8660254037844148378, 1.000000000000023981 ) ) 
 REPRESENTATION_ITEM ( '' )  );
#18851=CARTESIAN_POINT ( 'NONE',  ( -4.999999999999996447, 8.660254037844387298, -33.37500000409676915 ) ) ;
#18853=CARTESIAN_POINT ( 'NONE',  ( 5.405949406249992428, -9.363379034771808662, -82.59375000204836681 ) ) ;
#18854=CYLINDRICAL_SURFACE ( 'NONE', #34834, 9.999999999999998224 ) ;
#18855=CARTESIAN_POINT ( 'NONE',  ( -10.81189881249999729, 6.242252689847871849, -50.40625000204837391 ) ) ;
#18856=FACE_OUTER_BOUND ( 'NONE', #7560, .T. ) ;
#18858=CARTESIAN_POINT ( 'NONE',  ( 9.999999999999996447, -5.773502691896262640, -135.6250000000000000 ) ) ;
#18859=CARTESIAN_POINT ( 'NONE',  ( -5.405949406250003975, -9.363379034771801557, -143.0312500020483810 ) ) ;
#18860=DIRECTION ( 'NONE',  ( 1.000000000000000000, 0.000000000000000000, 0.000000000000000000 ) ) ;
#18862=CARTESIAN_POINT ( 'NONE',  ( 9.999999999999998224, 0.000000000000000000, -125.3750000040967905 ) ) ;
#18864=EDGE_CURVE ( 'NONE', #27593, #12898, #32603, .T. ) ;
#18865=ORIENTED_EDGE ( 'NONE', *, *, #10403, .T. ) ;
#18868=DIRECTION ( 'NONE',  ( -0.000000000000000000, -0.000000000000000000, 1.000000000000000000 ) ) ;
#18869=CARTESIAN_POINT ( 'NONE',  ( 10.81189881249999907, 6.242252689847868297, -172.4062500020484094 ) ) ;
#18870=CARTESIAN_POINT ( 'NONE',  ( -9.999999999999998224, 1.224646799147353059E-15, -52.62500000409675494 ) ) ;
#18874=CARTESIAN_POINT ( 'NONE',  ( 5.405949406249992428, -9.363379034771808662, -171.2812500020484094 ) ) ;
#18876=CARTESIAN_POINT ( 'NONE',  ( 4.999999999999992006, -8.660254037844389075, -56.24999999999996447 ) ) ;
#18877=ORIENTED_EDGE ( 'NONE', *, *, #6560, .T. ) ;
#18878=CARTESIAN_POINT ( 'NONE',  ( -9.999999999999998224, 1.224646799147353059E-15, -194.7500000000000000 ) ) ;
#18879=ADVANCED_FACE ( 'NONE', ( #22857 ), #39459, .T. ) ;
#18880=CARTESIAN_POINT ( 'NONE',  ( -9.999999999999998224, 1.224646799147353059E-15, -26.74999999999996803 ) ) ;
#18881=CARTESIAN_POINT ( 'NONE',  ( -5.405949406249996869, 9.363379034771805109, -74.53125000204838102 ) ) ;
#18884=CARTESIAN_POINT ( 'NONE',  ( -9.999999999999998224, 1.224646799147353059E-15, -189.1250000040967905 ) ) ;
#18885=ORIENTED_EDGE ( 'NONE', *, *, #40947, .F. ) ;
#18887=CARTESIAN_POINT ( 'NONE',  ( 5.405949406249992428, -9.363379034771808662, -28.59375000204836326 ) ) ;
#18888=CARTESIAN_POINT ( 'NONE',  ( 7.070501591499376803E-16, 11.54700538379251284, -77.00000000409677625 ) ) ;
#18889=CARTESIAN_POINT ( 'NONE',  ( 5.405949406249999534, 9.363379034771803333, -7.281250002048378356 ) ) ;
#18890=CARTESIAN_POINT ( 'NONE',  ( 10.81189881249999907, 6.242252689847868297, -53.71875000204838102 ) ) ;
#18891=EDGE_LOOP ( 'NONE', ( #16360, #21245, #6501 ) ) ;
#18892=CARTESIAN_POINT ( 'NONE',  ( -10.00000000000154188, 5.773502691895366468, -28.37499999999993605 ) ) ;
#18894=CARTESIAN_POINT ( 'NONE',  ( -5.405949406250003975, -9.363379034771801557, -189.3437500020483810 ) ) ;
#18895=CARTESIAN_POINT ( 'NONE',  ( 5.405949406249999534, 9.363379034771803333, -175.0937500020484094 ) ) ;
#18898=LINE ( 'NONE', #21922, #24725 ) ;
#18901=CARTESIAN_POINT ( 'NONE',  ( 5.405949406249999534, 9.363379034771803333, -103.0937500020483810 ) ) ;
#18902=CARTESIAN_POINT ( 'NONE',  ( 9.999999999999932498, 5.773502691896291950, -196.8750000000000284 ) ) ;
#18903=CARTESIAN_POINT ( 'NONE',  ( -10.81189881249999729, 1.324075727343319199E-15, -77.28125000204838102 ) ) ;
#18904=CARTESIAN_POINT ( 'NONE',  ( 5.405949406249999534, 9.363379034771803333, -92.59375000204838102 ) ) ;
#18906=CARTESIAN_POINT ( 'NONE',  ( -4.999999999999996447, 8.660254037844387298, -144.3750000040967905 ) ) ;
#18908=ORIENTED_EDGE ( 'NONE', *, *, #11028, .T. ) ;
#18911=CARTESIAN_POINT ( 'NONE',  ( -2.293366432827344421E-15, -12.48450537969573659, -196.9062500020484094 ) ) ;
#18914=VERTEX_POINT ( 'NONE', #6872 ) ;
#18915=CARTESIAN_POINT ( 'NONE',  ( -2.121150477449813534E-15, -11.54700538379251284, -68.37499999999998579 ) ) ;
#18917=CARTESIAN_POINT ( 'NONE',  ( 5.000000000000000000, 8.660254037844385522, -71.12500000409677625 ) ) ;
#18921=CARTESIAN_POINT ( 'NONE',  ( 5.405949406249992428, -9.363379034771808662, -64.78125000204838102 ) ) ;
#18923=CARTESIAN_POINT ( 'NONE',  ( 9.999999999999479527, 5.773502691896553074, -93.75000000409674783 ) ) ;
#18926=CARTESIAN_POINT ( 'NONE',  ( -5.405949406249996869, 9.363379034771805109, -193.0312500020484094 ) ) ;
#18929=CARTESIAN_POINT ( 'NONE',  ( -2.293366432827344421E-15, -12.48450537969573659, -6.218750002048345493 ) ) ;
#18931=CARTESIAN_POINT ( 'NONE',  ( 4.999999999999992006, -8.660254037844389075, -50.24999999999998579 ) ) ;
#18932=CARTESIAN_POINT ( 'NONE',  ( 10.00000000000076916, -5.773502691895816774, -112.0000000040967620 ) ) ;
#18933=CARTESIAN_POINT ( 'NONE',  ( -9.999999999999998224, 5.773502691896259087, -178.3750000000000000 ) ) ;
#18935=CARTESIAN_POINT ( 'NONE',  ( -2.293366432827344421E-15, -12.48450537969573659, -99.40625000204839523 ) ) ;
#18936=VERTEX_POINT ( 'NONE', #9893 ) ;
#18937=CARTESIAN_POINT ( 'NONE',  ( 9.999999999999998224, 0.000000000000000000, -164.0000000000000000 ) ) ;
#18939=VERTEX_POINT ( 'NONE', #29974 ) ;
#18940=ADVANCED_FACE ( 'NONE', ( #32997 ), #26722, .T. ) ;
#18941=CARTESIAN_POINT ( 'NONE',  ( 10.81189881249999551, -6.242252689847874514, -31.65625000204834905 ) ) ;
#18942=CARTESIAN_POINT ( 'NONE',  ( -2.293366432827344421E-15, -12.48450537969573659, -81.21875000204838102 ) ) ;
#18944=CARTESIAN_POINT ( 'NONE',  ( -5.405949406249996869, 9.363379034771805109, -197.3437500020484094 ) ) ;
#18948=CARTESIAN_POINT ( 'NONE',  ( 5.000000000000000000, 8.660254037844385522, -8.125000004096744277 ) ) ;
#18949=CARTESIAN_POINT ( 'NONE',  ( -10.81189881249999729, 1.324075727343319199E-15, -126.5937500020483668 ) ) ;
#18950=CARTESIAN_POINT ( 'NONE',  ( -5.405949406250003975, -9.363379034771801557, -118.8437500020483810 ) ) ;
#18953=CARTESIAN_POINT ( 'NONE',  ( -2.121150477449813534E-15, -11.54700538379251284, -167.7500000040968189 ) ) ;
#18955=CARTESIAN_POINT ( 'NONE',  ( 10.00000000000102318, -5.773502691895667560, -66.62499999999995737 ) ) ;
#18958=CARTESIAN_POINT ( 'NONE',  ( -2.293366432827344421E-15, -12.48450537969573659, -43.71875000204835970 ) ) ;
#18960=CARTESIAN_POINT ( 'NONE',  ( -2.293366432827344421E-15, -12.48450537969573659, -6.406250002048362369 ) ) ;
#18962=DIRECTION ( 'NONE',  ( 1.000000000000000000, 0.000000000000000000, 0.000000000000000000 ) ) ;
#18964=CARTESIAN_POINT ( 'NONE',  ( 5.000000000000000000, 8.660254037844385522, -87.24999999999998579 ) ) ;
#18966=CARTESIAN_POINT ( 'NONE',  ( 9.999999999999998224, 0.000000000000000000, -101.3750000040967905 ) ) ;
#18967=CARTESIAN_POINT ( 'NONE',  ( -9.999999999999998224, 1.224646799147353059E-15, -190.6250000040967905 ) ) ;
#18969=CARTESIAN_POINT ( 'NONE',  ( -5.405949406249996869, 9.363379034771805109, -89.53125000204838102 ) ) ;
#18971=EDGE_CURVE ( 'NONE', #6595, #3659, #32781, .T. ) ;
#18972=AXIS2_PLACEMENT_3D ( 'NONE', #39191, #25826, #6599 ) ;
#18974=CARTESIAN_POINT ( 'NONE',  ( 9.999999999999998224, 0.000000000000000000, -197.3750000040967905 ) ) ;
#18975=CARTESIAN_POINT ( 'NONE',  ( 10.81189881249999551, -6.242252689847874514, -160.6562500020484379 ) ) ;
#18977=ORIENTED_EDGE ( 'NONE', *, *, #39009, .T. ) ;
#18978=CARTESIAN_POINT ( 'NONE',  ( -9.999999999999998224, 1.224646799147353059E-15, -20.74999999999996447 ) ) ;
#18979=CARTESIAN_POINT ( 'NONE',  ( 5.405949406249999534, 9.363379034771803333, -26.78125000204836681 ) ) ;
#18980=CARTESIAN_POINT ( 'NONE',  ( 9.999999999999998224, 0.000000000000000000, -152.0000000000000000 ) ) ;
#18982=CARTESIAN_POINT ( 'NONE',  ( -4.999999999999996447, 8.660254037844387298, -199.5000000000000000 ) ) ;
#18983=CARTESIAN_POINT ( 'NONE',  ( -5.405949406249996869, 9.363379034771805109, -125.5312500020483952 ) ) ;
#18984=ORIENTED_EDGE ( 'NONE', *, *, #14043, .T. ) ;
#18986=VECTOR ( 'NONE', #5335, 1000.000000000000000 ) ;
#18988=CARTESIAN_POINT ( 'NONE',  ( 10.81189881249999907, 6.242252689847868297, -50.90625000204838102 ) ) ;
#18990=CARTESIAN_POINT ( 'NONE',  ( -5.405949406250003975, -9.363379034771801557, -106.8437500020483810 ) ) ;
#18991=EDGE_CURVE ( 'NONE', #21406, #7623, #3008, .T. ) ;
#18992=ORIENTED_EDGE ( 'NONE', *, *, #21916, .T. ) ;
#18993=ORIENTED_EDGE ( 'NONE', *, *, #26217, .F. ) ;
#18994=AXIS2_PLACEMENT_3D ( 'NONE', #33282, #26369, #9951 ) ;
#18995=CARTESIAN_POINT ( 'NONE',  ( 0.000000000000000000, 0.000000000000000000, -200.0000000000000000 ) ) ;
#18996=CARTESIAN_POINT ( 'NONE',  ( 0.000000000000000000, 0.000000000000000000, -200.0000000000000000 ) ) ;
#18997=CARTESIAN_POINT ( 'NONE',  ( -10.81189881249999729, 6.242252689847871849, -159.7187500020483526 ) ) ;
#18999=CARTESIAN_POINT ( 'NONE',  ( -10.81189881249999907, -6.242252689847864744, -6.468750002048346381 ) ) ;
#19000=CARTESIAN_POINT ( 'NONE',  ( -9.999999999999998224, 1.224646799147353059E-15, -139.2499999999999716 ) ) ;
#19001=CARTESIAN_POINT ( 'NONE',  ( -10.81189881249999729, -6.242252689847864744, -142.9687500020483810 ) ) ;
#19005=CARTESIAN_POINT ( 'NONE',  ( -4.999999999999996447, 8.660254037844387298, -192.3750000040967905 ) ) ;
#19007=CARTESIAN_POINT ( 'NONE',  ( 10.81189881249999729, 0.000000000000000000, -196.5312500020484094 ) ) ;
#19008=CARTESIAN_POINT ( 'NONE',  ( -9.999999999999998224, 1.224646799147353059E-15, -47.74999999999998579 ) ) ;
#19011=CARTESIAN_POINT ( 'NONE',  ( -5.405949406250003975, -9.363379034771801557, -66.34375000204836681 ) ) ;
#19012=CARTESIAN_POINT ( 'NONE',  ( -5.405949406250003975, -9.363379034771801557, -54.34375000204835970 ) ) ;
#19014=CARTESIAN_POINT ( 'NONE',  ( 7.644554776091147741E-16, 12.48450537969573659, -23.65625000204838102 ) ) ;
#19018=CARTESIAN_POINT ( 'NONE',  ( 5.000000000000000000, 8.660254037844385522, -109.7499999999999858 ) ) ;
#19022=CARTESIAN_POINT ( 'NONE',  ( 5.405949406249992428, -9.363379034771808662, -112.7812500020483952 ) ) ;
#19023=ORIENTED_EDGE ( 'NONE', *, *, #26692, .T. ) ;
#19024=VECTOR ( 'NONE', #39519, 1000.000000000000000 ) ;
#19025=CARTESIAN_POINT ( 'NONE',  ( -10.00000000000025580, 5.773502691896109873, -121.3749999999999858 ) ) ;
#19027=CARTESIAN_POINT ( 'NONE',  ( -9.999999999998969713, -5.773502691896847949, -87.00000000409676204 ) ) ;
#19029=CARTESIAN_POINT ( 'NONE',  ( 4.999999999999992006, -8.660254037844389075, -41.24999999999997868 ) ) ;
#19030=CARTESIAN_POINT ( 'NONE',  ( 4.999999999999992006, -8.660254037844389075, -22.12500000409675494 ) ) ;
#19031=CARTESIAN_POINT ( 'NONE',  ( -5.405949406250003975, -9.363379034771801557, -53.03125000204836681 ) ) ;
#19032=AXIS2_PLACEMENT_3D ( 'NONE', #25907, #12510, #25704 ) ;
#19035=CARTESIAN_POINT ( 'NONE',  ( -9.999999999999998224, 1.224646799147353059E-15, -106.2499999999999858 ) ) ;
#19036=CARTESIAN_POINT ( 'NONE',  ( 10.81189881249999551, -6.242252689847874514, -144.1562500020484094 ) ) ;
#19037=CARTESIAN_POINT ( 'NONE',  ( -10.81189881249999729, 6.242252689847871849, -150.9062500020484094 ) ) ;
#19038=DIRECTION ( 'NONE',  ( 1.000000000000000000, 0.000000000000000000, 0.000000000000000000 ) ) ;
#19042=EDGE_LOOP ( 'NONE', ( #14230, #22170, #20717, #3023 ) ) ;
#19043=( BOUNDED_CURVE ( )  B_SPLINE_CURVE ( 2, ( #38166, #28251, #41813, #41387, #28475, #31926, #21766 ),
 .UNSPECIFIED., .F., .F. ) 
 B_SPLINE_CURVE_WITH_KNOTS ( ( 3, 2, 2, 3 ),
 ( 0.003731343283582092950, 0.004975124378109457846, 0.006218905472636822307, 0.007462686567164185901 ),
 .UNSPECIFIED. ) 
 CURVE ( )  GEOMETRIC_REPRESENTATION_ITEM ( )  RATIONAL_B_SPLINE_CURVE ( ( 0.9999999999999996669, 0.8660254037844390407, 1.000000000000000000, 0.8660254037844387076, 1.000000000000000000, 0.8660254037844379305, 1.000000000000000666 ) ) 
 REPRESENTATION_ITEM ( '' )  );
#19045=AXIS2_PLACEMENT_3D ( 'NONE', #17013, #36247, #3665 ) ;
#19046=CARTESIAN_POINT ( 'NONE',  ( 9.999999999999998224, 0.000000000000000000, -99.87500000409679046 ) ) ;
#19047=CARTESIAN_POINT ( 'NONE',  ( 10.81189881249999729, 0.000000000000000000, -182.8437500020483810 ) ) ;
#19048=CARTESIAN_POINT ( 'NONE',  ( -5.405949406249996869, 9.363379034771805109, -32.34375000204836681 ) ) ;
#19049=CARTESIAN_POINT ( 'NONE',  ( -9.999999999999998224, 1.224646799147353059E-15, -118.2500000000000000 ) ) ;
#19050=CARTESIAN_POINT ( 'NONE',  ( -10.81189881249999729, 1.324075727343319199E-15, -161.0937500020484094 ) ) ;
#19051=CARTESIAN_POINT ( 'NONE',  ( 10.81189881249999907, 6.242252689847868297, -152.7187500020483810 ) ) ;
#19055=CARTESIAN_POINT ( 'NONE',  ( -5.405949406250003975, -9.363379034771801557, -16.84375000204835260 ) ) ;
#19058=CARTESIAN_POINT ( 'NONE',  ( 7.070501591499376803E-16, 11.54700538379251284, -177.5000000040967905 ) ) ;
#19060=CARTESIAN_POINT ( 'NONE',  ( 10.81189881249999907, 6.242252689847868297, -80.71875000204838102 ) ) ;
#19061=CARTESIAN_POINT ( 'NONE',  ( -18.76388374866292708, -2.499999999999947153, 49.99999999999998579 ) ) ;
#19062=CARTESIAN_POINT ( 'NONE',  ( 10.81189881249999729, 0.000000000000000000, -46.53125000204838813 ) ) ;
#19064=CARTESIAN_POINT ( 'NONE',  ( 5.000000000000000000, 8.660254037844385522, -90.62500000409677625 ) ) ;
#19066=CARTESIAN_POINT ( 'NONE',  ( -9.999999999999998224, 1.224646799147353059E-15, -134.7499999999999716 ) ) ;
#19067=CARTESIAN_POINT ( 'NONE',  ( 10.81189881249999551, -6.242252689847874514, -147.1562500020484379 ) ) ;
#19068=CARTESIAN_POINT ( 'NONE',  ( -9.999999999999998224, 1.224646799147353059E-15, -29.74999999999997158 ) ) ;
#19069=CARTESIAN_POINT ( 'NONE',  ( 9.999999999999998224, 0.000000000000000000, -119.3750000040967905 ) ) ;
#19071=ORIENTED_EDGE ( 'NONE', *, *, #23823, .T. ) ;
#19074=CARTESIAN_POINT ( 'NONE',  ( 4.999999999999992006, -8.660254037844389075, -48.74999999999998579 ) ) ;
#19075=CARTESIAN_POINT ( 'NONE',  ( -10.81189881249999907, -6.242252689847864744, -171.6562500020484094 ) ) ;
#19076=CARTESIAN_POINT ( 'NONE',  ( 7.070501591499377789E-16, 11.54700538379251284, -50.00000000409675494 ) ) ;
#19078=CARTESIAN_POINT ( 'NONE',  ( -9.999999999999998224, 1.224646799147353059E-15, -135.1250000040967620 ) ) ;
#19080=DIRECTION ( 'NONE',  ( -0.000000000000000000, -0.000000000000000000, 1.000000000000000000 ) ) ;
#19081=CARTESIAN_POINT ( 'NONE',  ( 5.405949406249999534, 9.363379034771803333, -167.7812500020484094 ) ) ;
#19082=CARTESIAN_POINT ( 'NONE',  ( -4.999999999999996447, 8.660254037844387298, -183.3750000040967905 ) ) ;
#19083=ORIENTED_EDGE ( 'NONE', *, *, #39777, .T. ) ;
#19084=( BOUNDED_CURVE ( )  B_SPLINE_CURVE ( 2, ( #36823, #39428, #3187, #7265, #33605, #12870, #7058 ),
 .UNSPECIFIED., .F., .F. ) 
 B_SPLINE_CURVE_WITH_KNOTS ( ( 3, 2, 2, 3 ),
 ( 0.5708955223880599616, 0.5721393034825872359, 0.5733830845771146212, 0.5746268656716420065 ),
 .UNSPECIFIED. ) 
 CURVE ( )  GEOMETRIC_REPRESENTATION_ITEM ( )  RATIONAL_B_SPLINE_CURVE ( ( 0.9999999999999761302, 0.8660254037844625774, 1.000000000000000000, 0.8660254037844387076, 1.000000000000000000, 0.8660254037844148378, 1.000000000000023981 ) ) 
 REPRESENTATION_ITEM ( '' )  );
#19085=CARTESIAN_POINT ( 'NONE',  ( 10.00000000000000000, 5.773502691896255534, -137.2500000040967905 ) ) ;
#19086=CARTESIAN_POINT ( 'NONE',  ( -5.405949406250003975, -9.363379034771801557, -78.53125000204838102 ) ) ;
#19087=ORIENTED_EDGE ( 'NONE', *, *, #32185, .F. ) ;
#19089=EDGE_CURVE ( 'NONE', #26720, #21669, #38387, .T. ) ;
#19090=CARTESIAN_POINT ( 'NONE',  ( 9.999999999998456346, 5.773502691897149042, -30.37499999999991829 ) ) ;
#19091=VERTEX_POINT ( 'NONE', #14381 ) ;
#19092=VERTEX_POINT ( 'NONE', #27794 ) ;
#19093=EDGE_CURVE ( 'NONE', #21961, #14889, #29562, .T. ) ;
#19094=CARTESIAN_POINT ( 'NONE',  ( -10.81189881249999729, 1.324075727343319199E-15, -26.09375000204835970 ) ) ;
#19095=CARTESIAN_POINT ( 'NONE',  ( -9.999999999999998224, 1.224646799147353059E-15, -158.7500000000000000 ) ) ;
#19096=CARTESIAN_POINT ( 'NONE',  ( 10.81189881249999551, -6.242252689847874514, -7.656250002048367698 ) ) ;
#19097=( BOUNDED_CURVE ( )  B_SPLINE_CURVE ( 2, ( #23756, #23550, #6504, #33271, #6924, #10570, #33689 ),
 .UNSPECIFIED., .F., .F. ) 
 B_SPLINE_CURVE_WITH_KNOTS ( ( 3, 2, 2, 3 ),
 ( 0.3097014925373136052, 0.3109452736318408794, 0.3121890547263682092, 0.3134328358208955390 ),
 .UNSPECIFIED. ) 
 CURVE ( )  GEOMETRIC_REPRESENTATION_ITEM ( )  RATIONAL_B_SPLINE_CURVE ( ( 0.9999999999999820144, 0.8660254037844566932, 1.000000000000000000, 0.8660254037844387076, 1.000000000000000000, 0.8660254037844387076, 1.000000000000000000 ) ) 
 REPRESENTATION_ITEM ( '' )  );
#19098=CARTESIAN_POINT ( 'NONE',  ( -10.81189881249999907, -6.242252689847864744, -55.96875000204836681 ) ) ;
#19099=VERTEX_POINT ( 'NONE', #24565 ) ;
#19100=EDGE_CURVE ( 'NONE', #5730, #35357, #20659, .T. ) ;
#19103=CARTESIAN_POINT ( 'NONE',  ( -10.81189881249999729, 1.324075727343319199E-15, -188.0937500020483810 ) ) ;
#19104=CARTESIAN_POINT ( 'NONE',  ( -2.293366432827344421E-15, -12.48450537969573659, -180.2187500020484094 ) ) ;
#19108=CARTESIAN_POINT ( 'NONE',  ( 4.999999999999992006, -8.660254037844389075, -191.6250000040967905 ) ) ;
#19110=CARTESIAN_POINT ( 'NONE',  ( -10.81189881249999729, 1.324075727343319199E-15, -108.5937500020483810 ) ) ;
#19112=CARTESIAN_POINT ( 'NONE',  ( 7.644554776091147741E-16, 12.48450537969573659, -71.65625000204836681 ) ) ;
#19113=CARTESIAN_POINT ( 'NONE',  ( -5.405949406249996869, 9.363379034771805109, -1.031250002048372805 ) ) ;
#19114=CARTESIAN_POINT ( 'NONE',  ( -5.405949406249996869, 9.363379034771805109, -80.34375000204838102 ) ) ;
#19116=CARTESIAN_POINT ( 'NONE',  ( -10.00000000000000000, -5.773502691896251982, -147.0000000040967905 ) ) ;
#19118=EDGE_CURVE ( 'NONE', #31902, #31053, #7507, .T. ) ;
#19119=ORIENTED_EDGE ( 'NONE', *, *, #14286, .T. ) ;
#19122=CARTESIAN_POINT ( 'NONE',  ( -5.405949406250003975, -9.363379034771801557, -194.0312500020484094 ) ) ;
#19123=CARTESIAN_POINT ( 'NONE',  ( 4.999999999999992006, -8.660254037844389075, -51.74999999999996447 ) ) ;
#19125=ORIENTED_EDGE ( 'NONE', *, *, #17469, .F. ) ;
#19126=CARTESIAN_POINT ( 'NONE',  ( -5.000000000000003553, -8.660254037844383745, -63.99999999999997158 ) ) ;
#19128=CARTESIAN_POINT ( 'NONE',  ( -5.000000000000003553, -8.660254037844383745, -74.87500000409677625 ) ) ;
#19129=DIRECTION ( 'NONE',  ( 1.000000000000000000, 0.000000000000000000, 0.000000000000000000 ) ) ;
#19132=CARTESIAN_POINT ( 'NONE',  ( 7.644554776091147741E-16, 12.48450537969573659, -65.65625000204839523 ) ) ;
#19135=FACE_OUTER_BOUND ( 'NONE', #36605, .T. ) ;
#19136=CARTESIAN_POINT ( 'NONE',  ( 5.405949406249999534, 9.363379034771803333, -193.2812500020484094 ) ) ;
#19138=CARTESIAN_POINT ( 'NONE',  ( -10.81189881249999729, 1.324075727343319199E-15, -8.093750002048343717 ) ) ;
#19140=CARTESIAN_POINT ( 'NONE',  ( 9.999999999999998224, 0.000000000000000000, -180.5000000000000000 ) ) ;
#19141=CARTESIAN_POINT ( 'NONE',  ( 7.070501591499376803E-16, 11.54700538379251284, -159.5000000040968189 ) ) ;
#19142=CARTESIAN_POINT ( 'NONE',  ( -5.000000000000003553, -8.660254037844383745, -176.5000000000000000 ) ) ;
#19143=CARTESIAN_POINT ( 'NONE',  ( 5.405949406249992428, -9.363379034771808662, -103.7812500020483810 ) ) ;
#19144=ORIENTED_EDGE ( 'NONE', *, *, #5309, .F. ) ;
#19145=FACE_OUTER_BOUND ( 'NONE', #38953, .T. ) ;
#19146=EDGE_LOOP ( 'NONE', ( #37769, #33779, #14067, #12278 ) ) ;
#19147=ORIENTED_EDGE ( 'NONE', *, *, #22665, .F. ) ;
#19148=CARTESIAN_POINT ( 'NONE',  ( -5.405949406249996869, 9.363379034771805109, -28.03125000204837036 ) ) ;
#19150=CARTESIAN_POINT ( 'NONE',  ( -5.405949406250003975, -9.363379034771801557, -76.84375000204838102 ) ) ;
#19151=CYLINDRICAL_SURFACE ( 'NONE', #30513, 9.999999999999998224 ) ;
#19156=CARTESIAN_POINT ( 'NONE',  ( -5.000000000000003553, -8.660254037844383745, -13.37500000409674783 ) ) ;
#19157=CARTESIAN_POINT ( 'NONE',  ( -9.999999999999227285, -5.773502691896698735, -125.6249999999999574 ) ) ;
#19158=EDGE_CURVE ( 'NONE', #33970, #27845, #16049, .T. ) ;
#19159=CARTESIAN_POINT ( 'NONE',  ( 10.81189881249999551, -6.242252689847874514, -128.9687500020483810 ) ) ;
#19160=CARTESIAN_POINT ( 'NONE',  ( 7.644554776091147741E-16, 12.48450537969573659, -98.65625000204838102 ) ) ;
#19161=CARTESIAN_POINT ( 'NONE',  ( 7.644554776091147741E-16, 12.48450537969573659, -113.4687500020483668 ) ) ;
#19162=( BOUNDED_CURVE ( )  B_SPLINE_CURVE ( 2, ( #1615, #41066, #37645, #10085, #18206, #21449, #5059 ),
 .UNSPECIFIED., .F., .F. ) 
 B_SPLINE_CURVE_WITH_KNOTS ( ( 3, 2, 2, 3 ),
 ( 0.9365671641791047941, 0.9378109452736321794, 0.9390547263681594536, 0.9402985074626868389 ),
 .UNSPECIFIED. ) 
 CURVE ( )  GEOMETRIC_REPRESENTATION_ITEM ( )  RATIONAL_B_SPLINE_CURVE ( ( 0.9999999999999641398, 0.8660254037844745678, 1.000000000000000000, 0.8660254037844387076, 1.000000000000000000, 0.8660254037844148378, 1.000000000000023981 ) ) 
 REPRESENTATION_ITEM ( '' )  );
#19165=CARTESIAN_POINT ( 'NONE',  ( -2.121150477449813534E-15, -11.54700538379251284, -172.2500000040968189 ) ) ;
#19166=DIRECTION ( 'NONE',  ( 1.000000000000000000, 0.000000000000000000, 0.000000000000000000 ) ) ;
#19169=CARTESIAN_POINT ( 'NONE',  ( -10.81189881249999729, 1.324075727343319199E-15, -44.09375000204837391 ) ) ;
#19171=CARTESIAN_POINT ( 'NONE',  ( 5.405949406249992428, -9.363379034771808662, -0.2812500020483721386 ) ) ;
#19173=CARTESIAN_POINT ( 'NONE',  ( -9.999999999999998224, 1.224646799147353059E-15, -200.0000000000000000 ) ) ;
#19175=CARTESIAN_POINT ( 'NONE',  ( 9.999999999999998224, 0.000000000000000000, -90.49999999999998579 ) ) ;
#19177=CARTESIAN_POINT ( 'NONE',  ( -9.999999999999998224, 5.773502691896259087, -100.7500000040967905 ) ) ;
#19178=CARTESIAN_POINT ( 'NONE',  ( 9.999999999999998224, 0.000000000000000000, -128.0000000000000000 ) ) ;
#19180=CARTESIAN_POINT ( 'NONE',  ( 10.81189881249999729, 6.242252689847867408, -94.40625000204836681 ) ) ;
#19181=ORIENTED_EDGE ( 'NONE', *, *, #8554, .F. ) ;
#19186=CARTESIAN_POINT ( 'NONE',  ( -10.00000000000000000, -5.773502691896251982, -17.62499999999997158 ) ) ;
#19187=CARTESIAN_POINT ( 'NONE',  ( -4.999999999999996447, 8.660254037844387298, -156.0000000000000000 ) ) ;
#19188=VECTOR ( 'NONE', #18677, 1000.000000000000000 ) ;
#19191=CARTESIAN_POINT ( 'NONE',  ( -4.999999999999996447, 8.660254037844387298, -195.0000000000000000 ) ) ;
#19192=CARTESIAN_POINT ( 'NONE',  ( 7.644554776091147741E-16, 12.48450537969573659, -122.6562500020483952 ) ) ;
#19193=ORIENTED_EDGE ( 'NONE', *, *, #32820, .T. ) ;
#19194=CARTESIAN_POINT ( 'NONE',  ( 9.999999999999479527, 5.773502691896553074, -117.7500000040968189 ) ) ;
#19195=ORIENTED_EDGE ( 'NONE', *, *, #2245, .T. ) ;
#19196=CARTESIAN_POINT ( 'NONE',  ( -10.81189881249999907, -6.242252689847864744, -50.15625000204837391 ) ) ;
#19198=CARTESIAN_POINT ( 'NONE',  ( -10.81189881249999907, -6.242252689847864744, -105.4687500020483668 ) ) ;
#19201=FACE_OUTER_BOUND ( 'NONE', #6360, .T. ) ;
#19202=CARTESIAN_POINT ( 'NONE',  ( -10.00000000000051337, 5.773502691895962435, -144.2500000040967905 ) ) ;
#19203=( BOUNDED_CURVE ( )  B_SPLINE_CURVE ( 2, ( #5327, #31245, #37918, #31889, #21514, #1673, #24774 ),
 .UNSPECIFIED., .F., .F. ) 
 B_SPLINE_CURVE_WITH_KNOTS ( ( 3, 2, 2, 3 ),
 ( 0.9216417910447763928, 0.9228855721393036671, 0.9241293532338311634, 0.9253731343283585487 ),
 .UNSPECIFIED. ) 
 CURVE ( )  GEOMETRIC_REPRESENTATION_ITEM ( )  RATIONAL_B_SPLINE_CURVE ( ( 0.9999999999999761302, 0.8660254037844625774, 1.000000000000000000, 0.8660254037844387076, 1.000000000000000000, 0.8660254037844028474, 1.000000000000035971 ) ) 
 REPRESENTATION_ITEM ( '' )  );
#19204=CARTESIAN_POINT ( 'NONE',  ( -10.81189881249999907, -6.242252689847864744, -147.4687500020484094 ) ) ;
#19206=CARTESIAN_POINT ( 'NONE',  ( 10.00000000000154010, -5.773502691895370020, -26.12499999999993960 ) ) ;
#19207=LINE ( 'NONE', #32395, #22485 ) ;
#19208=CARTESIAN_POINT ( 'NONE',  ( -5.405949406250003975, -9.363379034771801557, -142.8437500020483810 ) ) ;
#19212=CARTESIAN_POINT ( 'NONE',  ( 9.999999999999998224, 0.000000000000000000, -194.3750000040967905 ) ) ;
#19214=CARTESIAN_POINT ( 'NONE',  ( 7.644554776091147741E-16, 12.48450537969573659, -185.6562500020484094 ) ) ;
#19215=DIRECTION ( 'NONE',  ( 0.8660254037844384856, 0.5000000000000004441, -0.000000000000000000 ) ) ;
#19218=CARTESIAN_POINT ( 'NONE',  ( -5.405949406249996869, 9.363379034771805109, -69.84375000204836681 ) ) ;
#19219=CARTESIAN_POINT ( 'NONE',  ( 10.81189881249999551, -6.242252689847874514, -49.46875000204835970 ) ) ;
#19221=CARTESIAN_POINT ( 'NONE',  ( 7.644554776091147741E-16, 12.48450537969573659, -29.65625000204835970 ) ) ;
#19225=CARTESIAN_POINT ( 'NONE',  ( 9.999999999999996447, -5.773502691896262640, -114.6249999999999858 ) ) ;
#19226=CARTESIAN_POINT ( 'NONE',  ( 9.999999999999998224, 0.000000000000000000, -119.3750000040967905 ) ) ;
#19229=CARTESIAN_POINT ( 'NONE',  ( -2.293366432827344421E-15, -12.48450537969573659, -118.9062500020483952 ) ) ;
#19232=CARTESIAN_POINT ( 'NONE',  ( -5.000000000000003553, -8.660254037844383745, -176.5000000000000000 ) ) ;
#19234=PLANE ( 'NONE',  #29819 ) ;
#19236=CARTESIAN_POINT ( 'NONE',  ( -4.999999999999996447, 8.660254037844387298, -43.49999999999998579 ) ) ;
#19237=CARTESIAN_POINT ( 'NONE',  ( -9.999999999999998224, 5.773502691896259087, -27.25000000409677625 ) ) ;
#19238=CARTESIAN_POINT ( 'NONE',  ( 10.81189881249999551, -6.242252689847874514, -46.65625000204835970 ) ) ;
#19239=DIRECTION ( 'NONE',  ( -0.000000000000000000, -0.000000000000000000, 1.000000000000000000 ) ) ;
#19242=LINE ( 'NONE', #22922, #19024 ) ;
#19243=CARTESIAN_POINT ( 'NONE',  ( 10.81189881249999729, 0.000000000000000000, -133.5312500020484094 ) ) ;
#19244=CARTESIAN_POINT ( 'NONE',  ( 10.81189881249999551, -6.242252689847874514, -153.1562500020484379 ) ) ;
#19245=CARTESIAN_POINT ( 'NONE',  ( 10.00000000000102318, -5.773502691895667560, -65.12499999999994316 ) ) ;
#19247=VERTEX_POINT ( 'NONE', #11156 ) ;
#19248=ORIENTED_EDGE ( 'NONE', *, *, #21208, .T. ) ;
#19249=ORIENTED_EDGE ( 'NONE', *, *, #41532, .T. ) ;
#19250=CARTESIAN_POINT ( 'NONE',  ( -10.81189881249999907, -6.242252689847864744, -169.9687500020484094 ) ) ;
#19251=AXIS2_PLACEMENT_3D ( 'NONE', #16545, #29743, #9458 ) ;
#19252=CARTESIAN_POINT ( 'NONE',  ( 10.81189881249999551, -6.242252689847874514, -29.96875000204834549 ) ) ;
#19253=CARTESIAN_POINT ( 'NONE',  ( -5.000000000000003553, -8.660254037844383745, -61.37500000409676204 ) ) ;
#19254=CARTESIAN_POINT ( 'NONE',  ( -2.293366432827344421E-15, -12.48450537969573659, -162.2187500020483810 ) ) ;
#19255=CARTESIAN_POINT ( 'NONE',  ( -5.405949406249996869, 9.363379034771805109, -146.3437500020483810 ) ) ;
#19256=CARTESIAN_POINT ( 'NONE',  ( 0.000000000000000000, 0.000000000000000000, -200.0000000000000000 ) ) ;
#19259=CARTESIAN_POINT ( 'NONE',  ( 5.405949406249992428, -9.363379034771808662, -16.59375000204835260 ) ) ;
#19263=CARTESIAN_POINT ( 'NONE',  ( -5.405949406249996869, 9.363379034771805109, -71.34375000204836681 ) ) ;
#19264=CARTESIAN_POINT ( 'NONE',  ( -10.81189881249999907, -6.242252689847864744, -48.65625000204836681 ) ) ;
#19266=CARTESIAN_POINT ( 'NONE',  ( -9.999999999999998224, 1.224646799147353059E-15, -200.0000000000000000 ) ) ;
#19268=CARTESIAN_POINT ( 'NONE',  ( 9.999999999999998224, 0.000000000000000000, -134.0000000000000000 ) ) ;
#19269=CARTESIAN_POINT ( 'NONE',  ( 5.405949406249992428, -9.363379034771808662, -148.7812500020483810 ) ) ;
#19270=CARTESIAN_POINT ( 'NONE',  ( 4.999999999999992006, -8.660254037844389075, -119.6250000040967905 ) ) ;
#19276=CARTESIAN_POINT ( 'NONE',  ( -5.405949406250003975, -9.363379034771801557, -174.5312500020484094 ) ) ;
#19277=CARTESIAN_POINT ( 'NONE',  ( -9.999999999999998224, 5.773502691896259087, -48.25000000409676915 ) ) ;
#19279=CARTESIAN_POINT ( 'NONE',  ( 9.999999999999998224, 0.000000000000000000, -200.0000000000000000 ) ) ;
#19280=EDGE_CURVE ( 'NONE', #30868, #35982, #33981, .T. ) ;
#19282=CARTESIAN_POINT ( 'NONE',  ( -4.999999999999996447, 8.660254037844387298, -44.99999999999998579 ) ) ;
#19283=CARTESIAN_POINT ( 'NONE',  ( -10.81189881249999729, 6.242252689847871849, -158.4062500020483810 ) ) ;
#19284=CARTESIAN_POINT ( 'NONE',  ( 10.81189881249999551, -6.242252689847874514, -140.9687500020483810 ) ) ;
#19285=CARTESIAN_POINT ( 'NONE',  ( 9.999999999999998224, 0.000000000000000000, -100.9999999999999858 ) ) ;
#19286=DIRECTION ( 'NONE',  ( -0.000000000000000000, -0.000000000000000000, 1.000000000000000000 ) ) ;
#19287=ORIENTED_EDGE ( 'NONE', *, *, #29928, .T. ) ;
#19288=( BOUNDED_CURVE ( )  B_SPLINE_CURVE ( 2, ( #32269, #29659, #23175, #20350, #39989, #36128, #9581 ),
 .UNSPECIFIED., .F., .F. ) 
 B_SPLINE_CURVE_WITH_KNOTS ( ( 3, 2, 2, 3 ),
 ( 0.6007462686567165422, 0.6019900497512439275, 0.6032338308457712017, 0.6044776119402985870 ),
 .UNSPECIFIED. ) 
 CURVE ( )  GEOMETRIC_REPRESENTATION_ITEM ( )  RATIONAL_B_SPLINE_CURVE ( ( 0.9999999999999880096, 0.8660254037844506980, 1.000000000000000000, 0.8660254037844387076, 1.000000000000000000, 0.8660254037844267172, 1.000000000000011990 ) ) 
 REPRESENTATION_ITEM ( '' )  );
#19289=CARTESIAN_POINT ( 'NONE',  ( 10.00000000000102318, -5.773502691895667560, -52.00000000409674072 ) ) ;
#19290=CARTESIAN_POINT ( 'NONE',  ( -10.81189881249999907, -6.242252689847864744, -68.15625000204840944 ) ) ;
#19292=CARTESIAN_POINT ( 'NONE',  ( -9.999999999999804601, -5.773502691896363892, -189.0000000040968473 ) ) ;
#19293=ORIENTED_EDGE ( 'NONE', *, *, #19400, .T. ) ;
#19294=EDGE_LOOP ( 'NONE', ( #33595, #38311, #22028, #3919 ) ) ;
#19295=CARTESIAN_POINT ( 'NONE',  ( -10.81189881249999729, 6.242252689847871849, -27.71875000204838102 ) ) ;
#19297=CARTESIAN_POINT ( 'NONE',  ( 7.644554776091147741E-16, 12.48450537969573659, -4.156250002048351710 ) ) ;
#19298=CARTESIAN_POINT ( 'NONE',  ( -10.81189881249999729, 1.324075727343319199E-15, -53.09375000204835970 ) ) ;
#19301=CARTESIAN_POINT ( 'NONE',  ( 10.81189881249999729, 6.242252689847867408, -187.2187500020484094 ) ) ;
#19302=CARTESIAN_POINT ( 'NONE',  ( -10.81189881249999729, 6.242252689847871849, -170.2187500020483810 ) ) ;
#19305=CARTESIAN_POINT ( 'NONE',  ( 7.070501591499376803E-16, 11.54700538379251284, -124.6249999999999858 ) ) ;
#19306=CARTESIAN_POINT ( 'NONE',  ( 9.999999999999998224, 0.000000000000000000, -194.0000000000000000 ) ) ;
#19308=CARTESIAN_POINT ( 'NONE',  ( -10.81189881249999729, 6.242252689847871849, -104.2187500020483810 ) ) ;
#19310=CARTESIAN_POINT ( 'NONE',  ( -9.999999999999998224, 1.224646799147353059E-15, -196.2500000000000000 ) ) ;
#19311=CARTESIAN_POINT ( 'NONE',  ( 10.81189881249999551, -6.242252689847874514, -76.65625000204838102 ) ) ;
#19312=CARTESIAN_POINT ( 'NONE',  ( -4.999999999999996447, 8.660254037844387298, -96.37500000409677625 ) ) ;
#19313=CARTESIAN_POINT ( 'NONE',  ( 10.81189881249999551, -6.242252689847874514, -86.96875000204836681 ) ) ;
#19315=CARTESIAN_POINT ( 'NONE',  ( 9.999999999999998224, 0.000000000000000000, -149.3750000040967905 ) ) ;
#19317=ORIENTED_EDGE ( 'NONE', *, *, #25815, .T. ) ;
#19320=CARTESIAN_POINT ( 'NONE',  ( -10.81189881249999729, 6.242252689847871849, -192.9062500020484094 ) ) ;
#19324=CARTESIAN_POINT ( 'NONE',  ( 10.00000000000000000, 5.773502691896255534, -57.37499999999997868 ) ) ;
#19326=CARTESIAN_POINT ( 'NONE',  ( 10.00000000000000000, 5.773502691896255534, -77.25000000409677625 ) ) ;
#19327=EDGE_CURVE ( 'NONE', #35521, #23854, #15027, .T. ) ;
#19331=EDGE_CURVE ( 'NONE', #14889, #31836, #28657, .T. ) ;
#19333=CARTESIAN_POINT ( 'NONE',  ( -10.81189881249999729, 6.242252689847871849, -66.90625000204839523 ) ) ;
#19334=EDGE_CURVE ( 'NONE', #19666, #32484, #5339, .T. ) ;
#19338=VERTEX_POINT ( 'NONE', #12222 ) ;
#19339=CARTESIAN_POINT ( 'NONE',  ( 10.81189881249999551, -6.242252689847874514, -192.1562500020484094 ) ) ;
#19342=CARTESIAN_POINT ( 'NONE',  ( 10.81189881249999729, 0.000000000000000000, -5.843750002048370362 ) ) ;
#19344=CIRCLE ( 'NONE', #41389, 9.999999999999998224 ) ;
#19349=CARTESIAN_POINT ( 'NONE',  ( -9.999999999999998224, 5.773502691896259087, -176.8750000000000000 ) ) ;
#19351=CARTESIAN_POINT ( 'NONE',  ( 10.81189881249999729, 0.000000000000000000, -90.03125000204838102 ) ) ;
#19352=ORIENTED_EDGE ( 'NONE', *, *, #25815, .F. ) ;
#19354=ADVANCED_FACE ( 'NONE', ( #2116 ), #21738, .T. ) ;
#19357=CARTESIAN_POINT ( 'NONE',  ( 5.405949406249999534, 9.363379034771803333, -37.09375000204836681 ) ) ;
#19358=CARTESIAN_POINT ( 'NONE',  ( 10.81189881249999907, 6.242252689847868297, -32.90625000204835970 ) ) ;
#19360=EDGE_CURVE ( 'NONE', #1371, #28132, #4227, .T. ) ;
#19361=CARTESIAN_POINT ( 'NONE',  ( 10.81189881249999729, 0.000000000000000000, -77.84375000204838102 ) ) ;
#19363=CARTESIAN_POINT ( 'NONE',  ( 10.81189881249999907, 6.242252689847868297, -191.7187500020484094 ) ) ;
#19364=DIRECTION ( 'NONE',  ( -0.000000000000000000, -0.000000000000000000, 1.000000000000000000 ) ) ;
#19365=CARTESIAN_POINT ( 'NONE',  ( 9.999999999999998224, 0.000000000000000000, -200.0000000000000000 ) ) ;
#19367=CARTESIAN_POINT ( 'NONE',  ( 9.999999999999998224, 0.000000000000000000, -9.875000004096746054 ) ) ;
#19369=CARTESIAN_POINT ( 'NONE',  ( 10.81189881249999907, 6.242252689847868297, -127.2187500020483668 ) ) ;
#19370=CARTESIAN_POINT ( 'NONE',  ( -10.81189881249999729, 6.242252689847871849, -101.4062500020483952 ) ) ;
#19371=CARTESIAN_POINT ( 'NONE',  ( -10.81189881249999729, -6.242252689847864744, -108.4687500020483810 ) ) ;
#19375=CARTESIAN_POINT ( 'NONE',  ( 10.00000000000000000, 5.773502691896255534, -171.7500000040967905 ) ) ;
#19381=CARTESIAN_POINT ( 'NONE',  ( -9.999999999998969713, -5.773502691896847949, -60.00000000409674072 ) ) ;
#19383=CARTESIAN_POINT ( 'NONE',  ( 7.070501591499377789E-16, 11.54700538379251284, -87.12499999999997158 ) ) ;
#19385=CARTESIAN_POINT ( 'NONE',  ( -9.999999999999998224, 1.224646799147353059E-15, -96.12500000409677625 ) ) ;
#19386=FACE_OUTER_BOUND ( 'NONE', #13075, .T. ) ;
#19388=CARTESIAN_POINT ( 'NONE',  ( 7.644554776091147741E-16, 12.48450537969573659, -89.65625000204838102 ) ) ;
#19389=ORIENTED_EDGE ( 'NONE', *, *, #1611, .F. ) ;
#19391=CYLINDRICAL_SURFACE ( 'NONE', #5689, 9.999999999999998224 ) ;
#19393=EDGE_LOOP ( 'NONE', ( #9995, #37181, #25679, #38669 ) ) ;
#19394=CARTESIAN_POINT ( 'NONE',  ( -10.00000000000000000, -5.773502691896251982, -16.12499999999998224 ) ) ;
#19395=CARTESIAN_POINT ( 'NONE',  ( -5.000000000000003553, -8.660254037844383745, -155.5000000000000000 ) ) ;
#19400=EDGE_CURVE ( 'NONE', #38971, #30360, #18706, .T. ) ;
#19401=CARTESIAN_POINT ( 'NONE',  ( -2.293366432827344421E-15, -12.48450537969573659, -124.9062500020483810 ) ) ;
#19402=VERTEX_POINT ( 'NONE', #31465 ) ;
#19403=CARTESIAN_POINT ( 'NONE',  ( 9.999999999999998224, 0.000000000000000000, -90.49999999999998579 ) ) ;
#19405=CARTESIAN_POINT ( 'NONE',  ( -10.81189881249999729, 6.242252689847871849, -54.90625000204836681 ) ) ;
#19408=CARTESIAN_POINT ( 'NONE',  ( 10.81189881249999729, 0.000000000000000000, -100.3437500020483810 ) ) ;
#19409=EDGE_LOOP ( 'NONE', ( #27089, #29142, #6250, #16075 ) ) ;
#19412=CARTESIAN_POINT ( 'NONE',  ( 9.999999999999998224, 0.000000000000000000, -174.8750000040967905 ) ) ;
#19413=LINE ( 'NONE', #16153, #31147 ) ;
#19415=CARTESIAN_POINT ( 'NONE',  ( -10.81189881249999907, -6.242252689847864744, -1.968750002048357262 ) ) ;
#19416=CARTESIAN_POINT ( 'NONE',  ( 7.644554776091147741E-16, 12.48450537969573659, -128.4687500020483810 ) ) ;
#19420=CARTESIAN_POINT ( 'NONE',  ( 9.999999999999996447, -5.773502691896262640, -196.0000000040968189 ) ) ;
#19422=AXIS2_PLACEMENT_3D ( 'NONE', #35421, #18363, #21388 ) ;
#19423=CARTESIAN_POINT ( 'NONE',  ( 10.81189881249999551, -6.242252689847874514, -189.1562500020484094 ) ) ;
#19424=CARTESIAN_POINT ( 'NONE',  ( -2.121150477449813534E-15, -11.54700538379251284, -185.7500000040967905 ) ) ;
#19427=CARTESIAN_POINT ( 'NONE',  ( 10.81189881249999729, 0.000000000000000000, -68.84375000204836681 ) ) ;
#19428=CARTESIAN_POINT ( 'NONE',  ( -2.293366432827344421E-15, -12.48450537969573659, -51.21875000204836681 ) ) ;
#19430=CARTESIAN_POINT ( 'NONE',  ( -2.293366432827344421E-15, -12.48450537969573659, -16.90625000204838102 ) ) ;
#19433=CARTESIAN_POINT ( 'NONE',  ( -5.000000000000003553, -8.660254037844383745, -116.4999999999999858 ) ) ;
#19436=CARTESIAN_POINT ( 'NONE',  ( -5.405949406249996869, 9.363379034771805109, -115.0312500020483952 ) ) ;
#19437=ORIENTED_EDGE ( 'NONE', *, *, #42029, .T. ) ;
#19438=CARTESIAN_POINT ( 'NONE',  ( 9.999999999999998224, 0.000000000000000000, -161.0000000000000000 ) ) ;
#19440=CARTESIAN_POINT ( 'NONE',  ( -5.000000000000003553, -8.660254037844383745, -128.5000000000000000 ) ) ;
#19442=ORIENTED_EDGE ( 'NONE', *, *, #10897, .T. ) ;
#19443=CARTESIAN_POINT ( 'NONE',  ( 5.000000000000000000, 8.660254037844385522, -45.24999999999998579 ) ) ;
#19444=AXIS2_PLACEMENT_3D ( 'NONE', #19586, #613, #16331 ) ;
#19445=CARTESIAN_POINT ( 'NONE',  ( 9.999999999999996447, -5.773502691896262640, -22.00000000409676915 ) ) ;
#19446=CARTESIAN_POINT ( 'NONE',  ( -10.81189881249999729, 1.324075727343319199E-15, -45.78125000204838813 ) ) ;
#19447=CARTESIAN_POINT ( 'NONE',  ( 9.999999999999998224, 0.000000000000000000, -41.37500000409677625 ) ) ;
#19451=CARTESIAN_POINT ( 'NONE',  ( 5.405949406249992428, -9.363379034771808662, -138.2812500020483810 ) ) ;
#19452=EDGE_CURVE ( 'NONE', #38772, #19609, #29312, .T. ) ;
#19453=CARTESIAN_POINT ( 'NONE',  ( -10.81189881249999729, 1.324075727343319199E-15, -153.7812500020484094 ) ) ;
#19454=CARTESIAN_POINT ( 'NONE',  ( 10.00000000000051159, -5.773502691895965988, -110.1249999999999858 ) ) ;
#19455=ORIENTED_EDGE ( 'NONE', *, *, #38668, .F. ) ;
#19456=VECTOR ( 'NONE', #3393, 1000.000000000000000 ) ;
#19457=( BOUNDED_CURVE ( )  B_SPLINE_CURVE ( 2, ( #42610, #29468, #22993, #39379, #2720, #29684, #29255 ),
 .UNSPECIFIED., .F., .F. ) 
 B_SPLINE_CURVE_WITH_KNOTS ( ( 3, 2, 2, 3 ),
 ( 0.5447761194029852039, 0.5460199004975125892, 0.5472636815920398634, 0.5485074626865672487 ),
 .UNSPECIFIED. ) 
 CURVE ( )  GEOMETRIC_REPRESENTATION_ITEM ( )  RATIONAL_B_SPLINE_CURVE ( ( 0.9999999999999880096, 0.8660254037844506980, 1.000000000000000000, 0.8660254037844387076, 1.000000000000000000, 0.8660254037844267172, 1.000000000000011990 ) ) 
 REPRESENTATION_ITEM ( '' )  );
#19458=ORIENTED_EDGE ( 'NONE', *, *, #36440, .F. ) ;
#19460=ADVANCED_FACE ( 'NONE', ( #2329 ), #31682, .T. ) ;
#19462=CARTESIAN_POINT ( 'NONE',  ( -5.405949406249996869, 9.363379034771805109, -176.3437500020483810 ) ) ;
#19463=VECTOR ( 'NONE', #13848, 1000.000000000000000 ) ;
#19464=CARTESIAN_POINT ( 'NONE',  ( 5.405949406249992428, -9.363379034771808662, -21.09375000204835615 ) ) ;
#19465=CARTESIAN_POINT ( 'NONE',  ( 10.00000000000102318, -5.773502691895667560, -61.00000000409674072 ) ) ;
#19466=CARTESIAN_POINT ( 'NONE',  ( 10.81189881249999551, -6.242252689847874514, -166.4687500020483810 ) ) ;
#19467=CARTESIAN_POINT ( 'NONE',  ( -5.405949406250003975, -9.363379034771801557, -145.8437500020483810 ) ) ;
#19471=CARTESIAN_POINT ( 'NONE',  ( 10.81189881249999907, 6.242252689847868297, -14.71875000204837036 ) ) ;
#19475=CARTESIAN_POINT ( 'NONE',  ( 9.999999999999998224, 0.000000000000000000, -99.87500000409679046 ) ) ;
#19476=CARTESIAN_POINT ( 'NONE',  ( -2.293366432827344421E-15, -12.48450537969573659, -72.21875000204835260 ) ) ;
#19477=CARTESIAN_POINT ( 'NONE',  ( 5.405949406249992428, -9.363379034771808662, -49.78125000204838813 ) ) ;
#19479=DIRECTION ( 'NONE',  ( -0.000000000000000000, -0.000000000000000000, 1.000000000000000000 ) ) ;
#19481=CARTESIAN_POINT ( 'NONE',  ( -9.999999999999998224, 5.773502691896259087, -140.8750000000000000 ) ) ;
#19482=CARTESIAN_POINT ( 'NONE',  ( 7.644554776091147741E-16, 12.48450537969573659, -142.1562500020484094 ) ) ;
#19483=CARTESIAN_POINT ( 'NONE',  ( -9.999999999999479527, -5.773502691896549521, -99.00000000409677625 ) ) ;
#19484=CARTESIAN_POINT ( 'NONE',  ( -9.999999999999998224, 1.224646799147353059E-15, -111.1250000040967763 ) ) ;
#19489=CARTESIAN_POINT ( 'NONE',  ( -5.000000000000003553, -8.660254037844383745, -140.8750000040967905 ) ) ;
#19490=EDGE_CURVE ( 'NONE', #26724, #16786, #15246, .T. ) ;
#19491=CARTESIAN_POINT ( 'NONE',  ( -10.81189881249999907, -6.242252689847864744, -176.1562500020483810 ) ) ;
#19492=CARTESIAN_POINT ( 'NONE',  ( 9.999999999999998224, 0.000000000000000000, -38.37500000409676915 ) ) ;
#19493=CARTESIAN_POINT ( 'NONE',  ( -9.999999999999998224, 1.224646799147353059E-15, -158.7500000000000000 ) ) ;
#19495=ADVANCED_FACE ( 'NONE', ( #18275 ), #25209, .T. ) ;
#19496=CARTESIAN_POINT ( 'NONE',  ( -9.999999999998969713, -5.773502691896847949, -64.12499999999997158 ) ) ;
#19497=CARTESIAN_POINT ( 'NONE',  ( -10.81189881249999729, 6.242252689847871849, -161.4062500020483810 ) ) ;
#19498=CARTESIAN_POINT ( 'NONE',  ( 10.81189881249999551, -6.242252689847874514, -142.4687500020483810 ) ) ;
#19500=CARTESIAN_POINT ( 'NONE',  ( 9.999999999999998224, 0.000000000000000000, -114.8750000040967905 ) ) ;
#19501=VERTEX_POINT ( 'NONE', #14730 ) ;
#19502=LINE ( 'NONE', #23613, #409 ) ;
#19503=CARTESIAN_POINT ( 'NONE',  ( -5.405949406249996869, 9.363379034771805109, -73.03125000204838102 ) ) ;
#19506=CARTESIAN_POINT ( 'NONE',  ( 10.81189881249999907, 6.242252689847868297, -118.2187500020483810 ) ) ;
#19507=ORIENTED_EDGE ( 'NONE', *, *, #39410, .F. ) ;
#19508=ORIENTED_EDGE ( 'NONE', *, *, #523, .F. ) ;
#19509=CARTESIAN_POINT ( 'NONE',  ( 10.81189881249999729, 0.000000000000000000, -23.84375000204835970 ) ) ;
#19510=CARTESIAN_POINT ( 'NONE',  ( 5.405949406249999534, 9.363379034771803333, -199.0937500020484094 ) ) ;
#19511=CARTESIAN_POINT ( 'NONE',  ( 7.644554776091147741E-16, 12.48450537969573659, -47.46875000204836681 ) ) ;
#19513=EDGE_CURVE ( 'NONE', #6937, #30149, #34832, .T. ) ;
#19515=CARTESIAN_POINT ( 'NONE',  ( 7.644554776091147741E-16, 12.48450537969573659, -186.9687500020484094 ) ) ;
#19516=CARTESIAN_POINT ( 'NONE',  ( -10.81189881249999907, -6.242252689847864744, -168.4687500020483526 ) ) ;
#19522=CARTESIAN_POINT ( 'NONE',  ( 5.405949406249999534, 9.363379034771803333, -100.0937500020483810 ) ) ;
#19523=CARTESIAN_POINT ( 'NONE',  ( 5.000000000000000000, 8.660254037844385522, -108.6250000040967763 ) ) ;
#19524=CARTESIAN_POINT ( 'NONE',  ( -5.405949406249996869, 9.363379034771805109, -76.03125000204838102 ) ) ;
#19527=CARTESIAN_POINT ( 'NONE',  ( -5.405949406249996869, 9.363379034771805109, -160.0312500020484094 ) ) ;
#19529=CARTESIAN_POINT ( 'NONE',  ( 9.999999999999996447, -5.773502691896262640, -134.5000000040967905 ) ) ;
#19534=CARTESIAN_POINT ( 'NONE',  ( -5.405949406250003975, -9.363379034771801557, -195.5312500020484094 ) ) ;
#19537=ORIENTED_EDGE ( 'NONE', *, *, #32848, .T. ) ;
#19538=CARTESIAN_POINT ( 'NONE',  ( 9.999999999999998224, 0.000000000000000000, -55.99999999999996447 ) ) ;
#19540=CARTESIAN_POINT ( 'NONE',  ( -2.121150477449813534E-15, -11.54700538379251284, -73.25000000409674783 ) ) ;
#19541=( BOUNDED_CURVE ( )  B_SPLINE_CURVE ( 2, ( #22757, #39565, #26837, #16245, #29445, #3539, #6987 ),
 .UNSPECIFIED., .F., .F. ) 
 B_SPLINE_CURVE_WITH_KNOTS ( ( 3, 2, 2, 3 ),
 ( 0.4179104477611941260, 0.4191542288557215112, 0.4203980099502488965, 0.4216417910447762818 ),
 .UNSPECIFIED. ) 
 CURVE ( )  GEOMETRIC_REPRESENTATION_ITEM ( )  RATIONAL_B_SPLINE_CURVE ( ( 0.9999999999999880096, 0.8660254037844506980, 1.000000000000000000, 0.8660254037844387076, 1.000000000000000000, 0.8660254037844207220, 1.000000000000017986 ) ) 
 REPRESENTATION_ITEM ( '' )  );
#19542=FACE_OUTER_BOUND ( 'NONE', #24787, .T. ) ;
#19544=CARTESIAN_POINT ( 'NONE',  ( -5.405949406250003975, -9.363379034771801557, -66.53125000204838102 ) ) ;
#19548=CARTESIAN_POINT ( 'NONE',  ( -2.293366432827344421E-15, -12.48450537969573659, -184.9062500020484094 ) ) ;
#19550=CARTESIAN_POINT ( 'NONE',  ( -4.999999999999996447, 8.660254037844387298, -85.49999999999998579 ) ) ;
#19552=DIRECTION ( 'NONE',  ( 0.000000000000000000, 0.000000000000000000, 1.000000000000000000 ) ) ;
#19553=CARTESIAN_POINT ( 'NONE',  ( -9.999999999999998224, 1.224646799147353059E-15, -167.7500000000000000 ) ) ;
#19555=CARTESIAN_POINT ( 'NONE',  ( -2.293366432827344421E-15, -12.48450537969573659, -97.90625000204839523 ) ) ;
#19556=ORIENTED_EDGE ( 'NONE', *, *, #36546, .T. ) ;
#19557=CARTESIAN_POINT ( 'NONE',  ( 4.999999999999992006, -8.660254037844389075, -181.1250000040967905 ) ) ;
#19559=ORIENTED_EDGE ( 'NONE', *, *, #19569, .T. ) ;
#19561=CARTESIAN_POINT ( 'NONE',  ( 5.405949406249992428, -9.363379034771808662, -34.59375000204836681 ) ) ;
#19562=CARTESIAN_POINT ( 'NONE',  ( -10.81189881249999907, -6.242252689847864744, -21.65625000204837036 ) ) ;
#19564=EDGE_CURVE ( 'NONE', #4695, #18570, #36990, .T. ) ;
#19565=CARTESIAN_POINT ( 'NONE',  ( 5.405949406249999534, 9.363379034771803333, -76.09375000204838102 ) ) ;
#19566=CYLINDRICAL_SURFACE ( 'NONE', #16666, 9.999999999999998224 ) ;
#19568=CARTESIAN_POINT ( 'NONE',  ( -10.81189881249999907, -6.242252689847864744, -193.9687500020484094 ) ) ;
#19569=EDGE_CURVE ( 'NONE', #27433, #20021, #33736, .T. ) ;
#19570=CARTESIAN_POINT ( 'NONE',  ( 9.999999999999998224, 0.000000000000000000, -99.49999999999998579 ) ) ;
#19571=CYLINDRICAL_SURFACE ( 'NONE', #14317, 9.999999999999998224 ) ;
#19573=CARTESIAN_POINT ( 'NONE',  ( 10.00000000000000000, 5.773502691896255534, -0.7500000040967473858 ) ) ;
#19575=CARTESIAN_POINT ( 'NONE',  ( -10.81189881249999729, 6.242252689847871849, -119.2187500020483810 ) ) ;
#19576=CARTESIAN_POINT ( 'NONE',  ( 5.405949406249992428, -9.363379034771808662, -97.78125000204839523 ) ) ;
#19577=CARTESIAN_POINT ( 'NONE',  ( 7.644554776091147741E-16, 12.48450537969573659, -104.4687500020483668 ) ) ;
#19580=CARTESIAN_POINT ( 'NONE',  ( -5.000000000000003553, -8.660254037844383745, -169.3750000040967905 ) ) ;
#19582=FACE_OUTER_BOUND ( 'NONE', #31788, .T. ) ;
#19586=CARTESIAN_POINT ( 'NONE',  ( 0.000000000000000000, 0.000000000000000000, -200.0000000000000000 ) ) ;
#19588=CARTESIAN_POINT ( 'NONE',  ( 4.999999999999992006, -8.660254037844389075, -59.62500000409676204 ) ) ;
#19590=CARTESIAN_POINT ( 'NONE',  ( -9.999999999999998224, 1.224646799147353059E-15, -85.24999999999997158 ) ) ;
#19592=CARTESIAN_POINT ( 'NONE',  ( -5.000000000000003553, -8.660254037844383745, -100.3750000040967905 ) ) ;
#19593=EDGE_CURVE ( 'NONE', #20886, #2600, #41397, .T. ) ;
#19594=DIRECTION ( 'NONE',  ( -0.000000000000000000, -0.000000000000000000, 1.000000000000000000 ) ) ;
#19596=CARTESIAN_POINT ( 'NONE',  ( 7.644554776091147741E-16, 12.48450537969573659, -95.65625000204838102 ) ) ;
#19598=( BOUNDED_CURVE ( )  B_SPLINE_CURVE ( 2, ( #15738, #25070, #28938, #11874, #5200, #38214, #28521 ),
 .UNSPECIFIED., .F., .F. ) 
 B_SPLINE_CURVE_WITH_KNOTS ( ( 3, 2, 2, 3 ),
 ( 0.07835820895522395413, 0.07960199004975131165, 0.08084577114427868305, 0.08208955223880604057 ),
 .UNSPECIFIED. ) 
 CURVE ( )  GEOMETRIC_REPRESENTATION_ITEM ( )  RATIONAL_B_SPLINE_CURVE ( ( 0.9999999999999924505, 0.8660254037844461461, 1.000000000000000000, 0.8660254037844387076, 1.000000000000000000, 0.8660254037844312691, 1.000000000000007550 ) ) 
 REPRESENTATION_ITEM ( '' )  );
#19600=DIRECTION ( 'NONE',  ( -0.000000000000000000, -0.000000000000000000, 1.000000000000000000 ) ) ;
#19602=ORIENTED_EDGE ( 'NONE', *, *, #29664, .T. ) ;
#19603=CARTESIAN_POINT ( 'NONE',  ( -5.000000000000003553, -8.660254037844383745, -9.999999999999953815 ) ) ;
#19604=CARTESIAN_POINT ( 'NONE',  ( 10.00000000000000000, 5.773502691896255534, -145.8750000000000284 ) ) ;
#19605=EDGE_CURVE ( 'NONE', #26580, #26059, #38140, .T. ) ;
#19607=CARTESIAN_POINT ( 'NONE',  ( 10.00000000000000000, 5.773502691896255534, -199.8750000000000284 ) ) ;
#19608=CARTESIAN_POINT ( 'NONE',  ( -10.81189881249999729, 1.324075727343319199E-15, -116.2812500020483952 ) ) ;
#19609=VERTEX_POINT ( 'NONE', #21007 ) ;
#19610=CARTESIAN_POINT ( 'NONE',  ( 9.999999999999998224, 0.000000000000000000, -94.99999999999998579 ) ) ;
#19611=ORIENTED_EDGE ( 'NONE', *, *, #22023, .T. ) ;
#19612=CARTESIAN_POINT ( 'NONE',  ( 5.405949406249992428, -9.363379034771808662, -43.78125000204838102 ) ) ;
#19614=CARTESIAN_POINT ( 'NONE',  ( 10.81189881249999907, 6.242252689847868297, -100.2187500020483810 ) ) ;
#19615=CARTESIAN_POINT ( 'NONE',  ( 5.405949406249999534, 9.363379034771803333, -124.2812500020483952 ) ) ;
#19616=EDGE_CURVE ( 'NONE', #39684, #414, #21220, .T. ) ;
#19617=ORIENTED_EDGE ( 'NONE', *, *, #7041, .F. ) ;
#19618=CYLINDRICAL_SURFACE ( 'NONE', #19045, 9.999999999999998224 ) ;
#19619=CARTESIAN_POINT ( 'NONE',  ( -9.999999999999998224, 1.224646799147353059E-15, -85.24999999999997158 ) ) ;
#19620=EDGE_CURVE ( 'NONE', #32541, #14017, #10858, .T. ) ;
#19622=DIRECTION ( 'NONE',  ( -0.000000000000000000, -0.000000000000000000, 1.000000000000000000 ) ) ;
#19623=CARTESIAN_POINT ( 'NONE',  ( -9.999999999999998224, 1.224646799147353059E-15, -24.12500000409675849 ) ) ;
#19624=EDGE_CURVE ( 'NONE', #38740, #3867, #23261, .T. ) ;
#19625=CARTESIAN_POINT ( 'NONE',  ( -5.405949406250003975, -9.363379034771801557, -135.3437500020484094 ) ) ;
#19628=PLANE ( 'NONE',  #34609 ) ;
#19630=CARTESIAN_POINT ( 'NONE',  ( 9.999999999999998224, 0.000000000000000000, -192.8750000040967905 ) ) ;
#19632=CARTESIAN_POINT ( 'NONE',  ( -10.81189881249999729, 6.242252689847871849, -183.9062500020484094 ) ) ;
#19633=AXIS2_PLACEMENT_3D ( 'NONE', #2584, #15713, #32576 ) ;
#19634=CARTESIAN_POINT ( 'NONE',  ( 9.999999999997939426, 5.773502691897446581, -6.750000004096692763 ) ) ;
#19637=CARTESIAN_POINT ( 'NONE',  ( -2.293366432827344421E-15, -12.48450537969573659, -63.21875000204839523 ) ) ;
#19638=CARTESIAN_POINT ( 'NONE',  ( 10.81189881249999907, 6.242252689847868297, -50.71875000204835970 ) ) ;
#19640=CARTESIAN_POINT ( 'NONE',  ( -2.293366432827344421E-15, -12.48450537969573659, -19.90625000204837747 ) ) ;
#19642=CARTESIAN_POINT ( 'NONE',  ( 9.999999999998969713, 5.773502691896851502, -27.75000000409675494 ) ) ;
#19644=CARTESIAN_POINT ( 'NONE',  ( -4.999999999999996447, 8.660254037844387298, -103.5000000000000000 ) ) ;
#19646=CARTESIAN_POINT ( 'NONE',  ( -9.999999999999227285, -5.773502691896698735, -115.1249999999999574 ) ) ;
#19649=CARTESIAN_POINT ( 'NONE',  ( -2.293366432827344421E-15, -12.48450537969573659, -112.9062500020483952 ) ) ;
#19657=CARTESIAN_POINT ( 'NONE',  ( 9.999999999999998224, 0.000000000000000000, -39.49999999999997868 ) ) ;
#19658=CARTESIAN_POINT ( 'NONE',  ( 7.070501591499377789E-16, 11.54700538379251284, -15.50000000409676915 ) ) ;
#19659=CARTESIAN_POINT ( 'NONE',  ( 10.81189881249999729, 0.000000000000000000, -43.53125000204838102 ) ) ;
#19663=CARTESIAN_POINT ( 'NONE',  ( -10.81189881249999729, 1.324075727343319199E-15, -140.2812500020483810 ) ) ;
#19664=CARTESIAN_POINT ( 'NONE',  ( 5.405949406249999534, 9.363379034771803333, -140.7812500020483810 ) ) ;
#19665=( BOUNDED_CURVE ( )  B_SPLINE_CURVE ( 2, ( #14640, #40961, #8191, #41613, #34312, #17876, #2361 ),
 .UNSPECIFIED., .F., .F. ) 
 B_SPLINE_CURVE_WITH_KNOTS ( ( 3, 2, 2, 3 ),
 ( 0.8470149253731346084, 0.8482587064676619937, 0.8495024875621892679, 0.8507462686567166532 ),
 .UNSPECIFIED. ) 
 CURVE ( )  GEOMETRIC_REPRESENTATION_ITEM ( )  RATIONAL_B_SPLINE_CURVE ( ( 0.9999999999999641398, 0.8660254037844745678, 1.000000000000000000, 0.8660254037844387076, 1.000000000000000000, 0.8660254037844148378, 1.000000000000023981 ) ) 
 REPRESENTATION_ITEM ( '' )  );
#19666=VERTEX_POINT ( 'NONE', #17971 ) ;
#19668=ORIENTED_EDGE ( 'NONE', *, *, #29337, .F. ) ;
#19670=CARTESIAN_POINT ( 'NONE',  ( 0.000000000000000000, 0.000000000000000000, -200.0000000000000000 ) ) ;
#19671=CARTESIAN_POINT ( 'NONE',  ( 10.81189881249999907, 6.242252689847868297, -175.2187500020484094 ) ) ;
#19672=CARTESIAN_POINT ( 'NONE',  ( 7.644554776091147741E-16, 12.48450537969573659, -23.46875000204836326 ) ) ;
#19673=CARTESIAN_POINT ( 'NONE',  ( -9.999999999999998224, 1.224646799147353059E-15, -46.62500000409677625 ) ) ;
#19674=CARTESIAN_POINT ( 'NONE',  ( -5.405949406249996869, 9.363379034771805109, -153.8437500020483810 ) ) ;
#19675=CARTESIAN_POINT ( 'NONE',  ( -10.81189881249999907, -6.242252689847864744, -147.4687500020484094 ) ) ;
#19676=CARTESIAN_POINT ( 'NONE',  ( 9.999999999999998224, 0.000000000000000000, -67.99999999999997158 ) ) ;
#19678=AXIS2_PLACEMENT_3D ( 'NONE', #19256, #41495, #5473 ) ;
#19680=CARTESIAN_POINT ( 'NONE',  ( -10.81189881249999729, 6.242252689847871849, -20.21875000204836326 ) ) ;
#19684=FACE_OUTER_BOUND ( 'NONE', #13588, .T. ) ;
#19688=CARTESIAN_POINT ( 'NONE',  ( 5.405949406249999534, 9.363379034771803333, -74.59375000204838102 ) ) ;
#19689=CARTESIAN_POINT ( 'NONE',  ( -10.81189881249999907, -6.242252689847864744, -39.65625000204835970 ) ) ;
#19691=CARTESIAN_POINT ( 'NONE',  ( 9.999999999999998224, 0.000000000000000000, -194.3750000040967905 ) ) ;
#19693=CARTESIAN_POINT ( 'NONE',  ( 9.999999999999998224, 0.000000000000000000, -138.5000000000000000 ) ) ;
#19694=VECTOR ( 'NONE', #4810, 1000.000000000000000 ) ;
#19695=CARTESIAN_POINT ( 'NONE',  ( -2.293366432827344421E-15, -12.48450537969573659, -138.4062500020484094 ) ) ;
#19697=CARTESIAN_POINT ( 'NONE',  ( -9.999999999999998224, 1.224646799147353059E-15, -117.1250000040967905 ) ) ;
#19699=ORIENTED_EDGE ( 'NONE', *, *, #33101, .T. ) ;
#19702=CARTESIAN_POINT ( 'NONE',  ( 0.000000000000000000, 0.000000000000000000, -200.0000000000000000 ) ) ;
#19703=CARTESIAN_POINT ( 'NONE',  ( 7.644554776091147741E-16, 12.48450537969573659, -170.6562500020484094 ) ) ;
#19704=CARTESIAN_POINT ( 'NONE',  ( -10.00000000000000000, -5.773502691896251982, -42.00000000409674783 ) ) ;
#19707=EDGE_CURVE ( 'NONE', #27322, #29348, #9338, .T. ) ;
#19708=( BOUNDED_CURVE ( )  B_SPLINE_CURVE ( 2, ( #38709, #34417, #17981, #76, #35484, #6336, #22733 ),
 .UNSPECIFIED., .F., .F. ) 
 B_SPLINE_CURVE_WITH_KNOTS ( ( 3, 2, 2, 3 ),
 ( 0.9067164179104481025, 0.9079601990049754878, 0.9092039800995028731, 0.9104477611940301474 ),
 .UNSPECIFIED. ) 
 CURVE ( )  GEOMETRIC_REPRESENTATION_ITEM ( )  RATIONAL_B_SPLINE_CURVE ( ( 0.9999999999999641398, 0.8660254037844745678, 1.000000000000000000, 0.8660254037844387076, 1.000000000000000000, 0.8660254037844028474, 1.000000000000035971 ) ) 
 REPRESENTATION_ITEM ( '' )  );
#19709=CARTESIAN_POINT ( 'NONE',  ( -4.999999999999996447, 8.660254037844387298, -73.49999999999998579 ) ) ;
#19710=CARTESIAN_POINT ( 'NONE',  ( -2.293366432827344421E-15, -12.48450537969573659, -157.9062500020483810 ) ) ;
#19711=CARTESIAN_POINT ( 'NONE',  ( -10.81189881249999729, 6.242252689847871849, -140.2187500020483810 ) ) ;
#19716=AXIS2_PLACEMENT_3D ( 'NONE', #8770, #4892, #5106 ) ;
#19717=CARTESIAN_POINT ( 'NONE',  ( 7.644554776091147741E-16, 12.48450537969573659, -70.15625000204839523 ) ) ;
#19720=CARTESIAN_POINT ( 'NONE',  ( 5.405949406249999534, 9.363379034771803333, -122.5937500020483952 ) ) ;
#19721=ORIENTED_EDGE ( 'NONE', *, *, #19707, .T. ) ;
#19722=ORIENTED_EDGE ( 'NONE', *, *, #22707, .T. ) ;
#19723=CARTESIAN_POINT ( 'NONE',  ( -10.81189881249999729, -6.242252689847864744, -22.96875000204837747 ) ) ;
#19724=CARTESIAN_POINT ( 'NONE',  ( -5.405949406250003975, -9.363379034771801557, -198.3437500020484094 ) ) ;
#19725=CARTESIAN_POINT ( 'NONE',  ( 7.644554776091147741E-16, 12.48450537969573659, -50.46875000204835970 ) ) ;
#19726=CARTESIAN_POINT ( 'NONE',  ( -9.999999999999998224, 1.224646799147353059E-15, -200.0000000000000000 ) ) ;
#19728=CARTESIAN_POINT ( 'NONE',  ( -10.81189881249999729, 6.242252689847871849, -182.2187500020484379 ) ) ;
#19729=CARTESIAN_POINT ( 'NONE',  ( -10.81189881249999907, -6.242252689847864744, -166.9687500020484094 ) ) ;
#19732=ADVANCED_FACE ( 'NONE', ( #6109 ), #22085, .T. ) ;
#19734=CARTESIAN_POINT ( 'NONE',  ( -4.999999999999996447, 8.660254037844387298, -193.5000000000000000 ) ) ;
#19736=CARTESIAN_POINT ( 'NONE',  ( -10.81189881249999729, 1.324075727343319199E-15, -93.59375000204838102 ) ) ;
#19737=CARTESIAN_POINT ( 'NONE',  ( 9.999999999999998224, 0.000000000000000000, -198.8750000040967905 ) ) ;
#19738=CARTESIAN_POINT ( 'NONE',  ( 5.405949406249999534, 9.363379034771803333, -68.78125000204838102 ) ) ;
#19739=CARTESIAN_POINT ( 'NONE',  ( -2.121150477449813534E-15, -11.54700538379251284, -159.8750000000000000 ) ) ;
#19741=CARTESIAN_POINT ( 'NONE',  ( -2.293366432827344421E-15, -12.48450537969573659, -160.9062500020483810 ) ) ;
#19743=CARTESIAN_POINT ( 'NONE',  ( -4.999999999999996447, 8.660254037844387298, -139.8750000040968189 ) ) ;
#19749=CARTESIAN_POINT ( 'NONE',  ( 10.81189881249999551, -6.242252689847874514, -198.1562500020484379 ) ) ;
#19752=CARTESIAN_POINT ( 'NONE',  ( -9.999999999999998224, 5.773502691896259087, -58.37499999999999289 ) ) ;
#19754=CARTESIAN_POINT ( 'NONE',  ( -5.000000000000003553, -8.660254037844383745, -64.37500000409676204 ) ) ;
#19755=EDGE_CURVE ( 'NONE', #9902, #39730, #32024, .T. ) ;
#19756=CARTESIAN_POINT ( 'NONE',  ( 0.000000000000000000, 0.000000000000000000, -200.0000000000000000 ) ) ;
#19758=CARTESIAN_POINT ( 'NONE',  ( -10.81189881249999729, 6.242252689847871849, -59.40625000204838813 ) ) ;
#19761=DIRECTION ( 'NONE',  ( -0.000000000000000000, -0.000000000000000000, 1.000000000000000000 ) ) ;
#19762=CARTESIAN_POINT ( 'NONE',  ( 10.81189881249999729, 0.000000000000000000, -187.5312500020484094 ) ) ;
#19764=CARTESIAN_POINT ( 'NONE',  ( 9.999999999999998224, 0.000000000000000000, -79.99999999999998579 ) ) ;
#19765=CARTESIAN_POINT ( 'NONE',  ( -4.999999999999996447, 8.660254037844387298, -165.0000000000000000 ) ) ;
#19766=CARTESIAN_POINT ( 'NONE',  ( 10.00000000000051159, -5.773502691895965988, -45.62499999999994316 ) ) ;
#19767=CARTESIAN_POINT ( 'NONE',  ( -5.000020801129981152, 8.660290040615111096, 0.000000000000000000 ) ) ;
#19768=CARTESIAN_POINT ( 'NONE',  ( -2.121150477449813534E-15, -11.54700538379251284, -165.8750000000000000 ) ) ;
#19769=CARTESIAN_POINT ( 'NONE',  ( -9.999999999998969713, -5.773502691896847949, -62.62499999999996447 ) ) ;
#19770=CARTESIAN_POINT ( 'NONE',  ( -10.81189881249999729, 1.324075727343319199E-15, -96.78125000204839523 ) ) ;
#19771=EDGE_LOOP ( 'NONE', ( #1407, #562, #32066, #14063 ) ) ;
#19772=FACE_OUTER_BOUND ( 'NONE', #19409, .T. ) ;
#19775=ORIENTED_EDGE ( 'NONE', *, *, #15202, .F. ) ;
#19776=CARTESIAN_POINT ( 'NONE',  ( -5.405949406250003975, -9.363379034771801557, -31.84375000204836681 ) ) ;
#19777=CARTESIAN_POINT ( 'NONE',  ( -10.81189881249999729, 6.242252689847871849, -24.90625000204838813 ) ) ;
#19779=CARTESIAN_POINT ( 'NONE',  ( 5.405949406249992428, -9.363379034771808662, -75.09375000204838102 ) ) ;
#19781=CARTESIAN_POINT ( 'NONE',  ( 7.644554776091147741E-16, 12.48450537969573659, -189.9687500020484094 ) ) ;
#19782=CARTESIAN_POINT ( 'NONE',  ( -9.999999999999998224, 1.224646799147353059E-15, -132.1250000040967620 ) ) ;
#19783=DIRECTION ( 'NONE',  ( -0.000000000000000000, -0.000000000000000000, 1.000000000000000000 ) ) ;
#19785=CARTESIAN_POINT ( 'NONE',  ( -9.999999999999998224, 1.224646799147353059E-15, -1.625000004096766038 ) ) ;
#19786=DIRECTION ( 'NONE',  ( -0.000000000000000000, -0.000000000000000000, 1.000000000000000000 ) ) ;
#19787=CARTESIAN_POINT ( 'NONE',  ( -5.405949406250003975, -9.363379034771801557, -123.3437500020483952 ) ) ;
#19788=CARTESIAN_POINT ( 'NONE',  ( 10.81189881249999729, 0.000000000000000000, -99.03125000204839523 ) ) ;
#19789=CARTESIAN_POINT ( 'NONE',  ( 10.81189881249999729, 0.000000000000000000, -107.8437500020483810 ) ) ;
#19792=CARTESIAN_POINT ( 'NONE',  ( -4.999999999999996447, 8.660254037844387298, -163.8750000040967905 ) ) ;
#19793=CYLINDRICAL_SURFACE ( 'NONE', #36486, 9.999999999999998224 ) ;
#19799=CARTESIAN_POINT ( 'NONE',  ( 9.999999999999998224, 0.000000000000000000, -149.0000000000000000 ) ) ;
#19801=CARTESIAN_POINT ( 'NONE',  ( 7.070501591499377789E-16, 11.54700538379251284, -81.12499999999997158 ) ) ;
#19803=CARTESIAN_POINT ( 'NONE',  ( -10.00000000000000000, -5.773502691896251982, -87.00000000409677625 ) ) ;
#19804=DIRECTION ( 'NONE',  ( -0.000000000000000000, -0.000000000000000000, 1.000000000000000000 ) ) ;
#19806=CARTESIAN_POINT ( 'NONE',  ( -5.405949406249996869, 9.363379034771805109, -94.03125000204838102 ) ) ;
#19807=ORIENTED_EDGE ( 'NONE', *, *, #4732, .F. ) ;
#19811=ORIENTED_EDGE ( 'NONE', *, *, #32446, .T. ) ;
#19812=CARTESIAN_POINT ( 'NONE',  ( 4.999999999999992006, -8.660254037844389075, -11.24999999999995381 ) ) ;
#19814=CARTESIAN_POINT ( 'NONE',  ( -2.121150477449813534E-15, -11.54700538379251284, -149.3750000000000000 ) ) ;
#19816=EDGE_CURVE ( 'NONE', #36111, #18400, #23178, .T. ) ;
#19817=CARTESIAN_POINT ( 'NONE',  ( 9.999999999999998224, 0.000000000000000000, -189.5000000000000000 ) ) ;
#19818=CARTESIAN_POINT ( 'NONE',  ( -10.81189881249999729, 6.242252689847871849, -116.4062500020483810 ) ) ;
#19821=CARTESIAN_POINT ( 'NONE',  ( -9.999999999999998224, 1.224646799147353059E-15, -200.0000000000000000 ) ) ;
#19822=VECTOR ( 'NONE', #41971, 1000.000000000000000 ) ;
#19824=( BOUNDED_CURVE ( )  B_SPLINE_CURVE ( 2, ( #16735, #13072, #32955, #10478, #16522, #32742, #3180 ),
 .UNSPECIFIED., .F., .F. ) 
 B_SPLINE_CURVE_WITH_KNOTS ( ( 3, 2, 2, 3 ),
 ( 0.1828358208955224162, 0.1840796019900497738, 0.1853233830845771313, 0.1865671641791045166 ),
 .UNSPECIFIED. ) 
 CURVE ( )  GEOMETRIC_REPRESENTATION_ITEM ( )  RATIONAL_B_SPLINE_CURVE ( ( 0.9999999999999970024, 0.8660254037844417052, 1.000000000000000000, 0.8660254037844387076, 1.000000000000000000, 0.8660254037844357100, 1.000000000000002887 ) ) 
 REPRESENTATION_ITEM ( '' )  );
#19825=CARTESIAN_POINT ( 'NONE',  ( -2.293366432827344421E-15, -12.48450537969573659, -43.90625000204838102 ) ) ;
#19827=CARTESIAN_POINT ( 'NONE',  ( 5.405949406249999534, 9.363379034771803333, -94.09375000204838102 ) ) ;
#19828=CARTESIAN_POINT ( 'NONE',  ( 7.644554776091147741E-16, 12.48450537969573659, -124.1562500020483810 ) ) ;
#19829=ORIENTED_EDGE ( 'NONE', *, *, #28465, .T. ) ;
#19830=CARTESIAN_POINT ( 'NONE',  ( 10.81189881249999729, 0.000000000000000000, -199.5312500020484094 ) ) ;
#19831=DIRECTION ( 'NONE',  ( 0.08715574274765837404, 0.000000000000000000, -0.9961946980917455452 ) ) ;
#19835=CARTESIAN_POINT ( 'NONE',  ( -5.405949406250003975, -9.363379034771801557, -133.8437500020484094 ) ) ;
#19837=DIRECTION ( 'NONE',  ( 1.000000000000000000, 0.000000000000000000, 0.000000000000000000 ) ) ;
#19839=CARTESIAN_POINT ( 'NONE',  ( -5.000000000000003553, -8.660254037844383745, -185.8750000040967905 ) ) ;
#19841=CARTESIAN_POINT ( 'NONE',  ( 10.81189881249999729, 6.242252689847867408, -190.4062500020483810 ) ) ;
#19842=( BOUNDED_CURVE ( )  B_SPLINE_CURVE ( 2, ( #2366, #29114, #15493, #28698, #41825, #38603, #9042 ),
 .UNSPECIFIED., .F., .F. ) 
 B_SPLINE_CURVE_WITH_KNOTS ( ( 3, 2, 2, 3 ),
 ( 0.5597014925373136052, 0.5609452736318409904, 0.5621890547263683757, 0.5634328358208957610 ),
 .UNSPECIFIED. ) 
 CURVE ( )  GEOMETRIC_REPRESENTATION_ITEM ( )  RATIONAL_B_SPLINE_CURVE ( ( 0.9999999999999761302, 0.8660254037844625774, 1.000000000000000000, 0.8660254037844387076, 1.000000000000000000, 0.8660254037844148378, 1.000000000000023981 ) ) 
 REPRESENTATION_ITEM ( '' )  );
#19847=CARTESIAN_POINT ( 'NONE',  ( 10.81189881249999729, 6.242252689847867408, -56.71875000204838813 ) ) ;
#19848=CARTESIAN_POINT ( 'NONE',  ( 10.81189881249999551, -6.242252689847874514, -52.46875000204837391 ) ) ;
#19850=CARTESIAN_POINT ( 'NONE',  ( -5.405949406249996869, 9.363379034771805109, -14.53125000204835615 ) ) ;
#19853=CARTESIAN_POINT ( 'NONE',  ( -9.999999999999998224, 1.224646799147353059E-15, -27.12500000409676204 ) ) ;
#19855=CARTESIAN_POINT ( 'NONE',  ( 4.999999999999992006, -8.660254037844389075, -108.7499999999999858 ) ) ;
#19858=CARTESIAN_POINT ( 'NONE',  ( -2.121150477449813534E-15, -11.54700538379251284, -27.87499999999999289 ) ) ;
#19861=CARTESIAN_POINT ( 'NONE',  ( 10.81189881249999729, 6.242252689847867408, -115.4062500020484094 ) ) ;
#19867=ORIENTED_EDGE ( 'NONE', *, *, #11329, .F. ) ;
#19868=CARTESIAN_POINT ( 'NONE',  ( -9.999999999999998224, 5.773502691896259087, -34.37499999999997158 ) ) ;
#19869=CARTESIAN_POINT ( 'NONE',  ( -2.121150477449813534E-15, -11.54700538379251284, -19.25000000409676915 ) ) ;
#19870=ADVANCED_FACE ( 'NONE', ( #15159 ), #35046, .T. ) ;
#19871=CARTESIAN_POINT ( 'NONE',  ( 5.405949406249992428, -9.363379034771808662, -46.78125000204838813 ) ) ;
#19872=CARTESIAN_POINT ( 'NONE',  ( -9.999999999998969713, -5.773502691896847949, -2.624999999999922728 ) ) ;
#19875=FACE_OUTER_BOUND ( 'NONE', #12628, .T. ) ;
#19876=CARTESIAN_POINT ( 'NONE',  ( 10.81189881249999729, 0.000000000000000000, -138.0312500020484094 ) ) ;
#19878=CARTESIAN_POINT ( 'NONE',  ( 4.999999999999992006, -8.660254037844389075, -15.74999999999995914 ) ) ;
#19880=ORIENTED_EDGE ( 'NONE', *, *, #7750, .F. ) ;
#19882=VECTOR ( 'NONE', #19902, 1000.000000000000000 ) ;
#19883=CARTESIAN_POINT ( 'NONE',  ( -9.999999999999998224, 1.224646799147353059E-15, -38.74999999999997868 ) ) ;
#19884=CARTESIAN_POINT ( 'NONE',  ( -5.405949406249996869, 9.363379034771805109, -177.8437500020483810 ) ) ;
#19885=ADVANCED_FACE ( 'NONE', ( #2873 ), #12561, .T. ) ;
#19886=CARTESIAN_POINT ( 'NONE',  ( -2.293366432827344421E-15, -12.48450537969573659, -24.21875000204836326 ) ) ;
#19887=CARTESIAN_POINT ( 'NONE',  ( -9.999999999999227285, -5.773502691896698735, -129.0000000040967620 ) ) ;
#19888=CARTESIAN_POINT ( 'NONE',  ( -10.81189881249999729, -6.242252689847864744, -157.9687500020484379 ) ) ;
#19889=CARTESIAN_POINT ( 'NONE',  ( -10.81189881249999729, 6.242252689847871849, -147.7187500020484094 ) ) ;
#19890=CARTESIAN_POINT ( 'NONE',  ( 10.00000000000154010, -5.773502691895370020, -9.624999999999943157 ) ) ;
#19893=CARTESIAN_POINT ( 'NONE',  ( -10.81189881249999729, 1.324075727343319199E-15, -20.09375000204835615 ) ) ;
#19895=CARTESIAN_POINT ( 'NONE',  ( -9.999999999999998224, 1.224646799147353059E-15, -31.62500000409676559 ) ) ;
#19896=CARTESIAN_POINT ( 'NONE',  ( -4.999999999999996447, 8.660254037844387298, -120.0000000000000000 ) ) ;
#19898=CARTESIAN_POINT ( 'NONE',  ( 5.000000000000000000, 8.660254037844385522, -99.62500000409679046 ) ) ;
#19899=CARTESIAN_POINT ( 'NONE',  ( 7.644554776091147741E-16, 12.48450537969573659, -75.96875000204838102 ) ) ;
#19900=CARTESIAN_POINT ( 'NONE',  ( 7.644554776091147741E-16, 12.48450537969573659, -41.65625000204837391 ) ) ;
#19902=DIRECTION ( 'NONE',  ( -0.000000000000000000, -0.000000000000000000, 1.000000000000000000 ) ) ;
#19904=CARTESIAN_POINT ( 'NONE',  ( -9.999999999999998224, 5.773502691896259087, -127.3750000000000000 ) ) ;
#19905=CARTESIAN_POINT ( 'NONE',  ( -10.81189881249999729, -6.242252689847864744, -141.6562500020484094 ) ) ;
#19906=FACE_OUTER_BOUND ( 'NONE', #35925, .T. ) ;
#19907=CARTESIAN_POINT ( 'NONE',  ( 7.070501591499377789E-16, 11.54700538379251284, -113.0000000040967905 ) ) ;
#19909=EDGE_LOOP ( 'NONE', ( #12622, #11788, #31161, #20620 ) ) ;
#19912=CARTESIAN_POINT ( 'NONE',  ( -10.00000000000051337, 5.773502691895962435, -38.87499999999994316 ) ) ;
#19913=CARTESIAN_POINT ( 'NONE',  ( -2.293366432827344421E-15, -12.48450537969573659, -168.4062500020483810 ) ) ;
#19914=CARTESIAN_POINT ( 'NONE',  ( 9.999999999999996447, -5.773502691896262640, -46.00000000409676915 ) ) ;
#19915=( BOUNDED_CURVE ( )  B_SPLINE_CURVE ( 2, ( #4306, #40324, #10766, #23955, #7542, #20696, #33884 ),
 .UNSPECIFIED., .F., .F. ) 
 B_SPLINE_CURVE_WITH_KNOTS ( ( 3, 2, 2, 3 ),
 ( 0.09701492537313441411, 0.09825870646766173000, 0.09950248756218905977, 0.1007462686567163757 ),
 .UNSPECIFIED. ) 
 CURVE ( )  GEOMETRIC_REPRESENTATION_ITEM ( )  RATIONAL_B_SPLINE_CURVE ( ( 0.9999999999999910072, 0.8660254037844477004, 1.000000000000000000, 0.8660254037844387076, 1.000000000000000000, 0.8660254037844431485, 0.9999999999999955591 ) ) 
 REPRESENTATION_ITEM ( '' )  );
#19916=CARTESIAN_POINT ( 'NONE',  ( 4.999999999999992006, -8.660254037844389075, -58.12500000409676204 ) ) ;
#19918=CARTESIAN_POINT ( 'NONE',  ( -10.00000000000102496, 5.773502691895664007, -44.87499999999994316 ) ) ;
#19919=CARTESIAN_POINT ( 'NONE',  ( 5.405949406249992428, -9.363379034771808662, -162.2812500020484094 ) ) ;
#19920=VECTOR ( 'NONE', #41989, 1000.000000000000000 ) ;
#19921=CARTESIAN_POINT ( 'NONE',  ( -5.405949406249996869, 9.363379034771805109, -131.3437500020484094 ) ) ;
#19922=CARTESIAN_POINT ( 'NONE',  ( -1.040834085586084257E-14, 20.00000000000000711, 22.49999999999999289 ) ) ;
#19925=CARTESIAN_POINT ( 'NONE',  ( 9.999999999999776179, 5.773502691896386985, -189.7500000040968189 ) ) ;
#19928=CARTESIAN_POINT ( 'NONE',  ( -5.405949406249996869, 9.363379034771805109, -70.03125000204838102 ) ) ;
#19929=VERTEX_POINT ( 'NONE', #18844 ) ;
#19931=CARTESIAN_POINT ( 'NONE',  ( 5.405949406249992428, -9.363379034771808662, -123.0937500020483952 ) ) ;
#19932=ORIENTED_EDGE ( 'NONE', *, *, #8126, .F. ) ;
#19934=CARTESIAN_POINT ( 'NONE',  ( -2.293366432827344421E-15, -12.48450537969573659, -19.71875000204837747 ) ) ;
#19935=CARTESIAN_POINT ( 'NONE',  ( 10.81189881249999729, 0.000000000000000000, -196.3437500020484094 ) ) ;
#19936=CARTESIAN_POINT ( 'NONE',  ( -10.81189881249999729, 1.324075727343319199E-15, -45.59375000204838102 ) ) ;
#19939=CARTESIAN_POINT ( 'NONE',  ( -5.405949406250003975, -9.363379034771801557, -180.3437500020483810 ) ) ;
#19940=CARTESIAN_POINT ( 'NONE',  ( -5.405949406250003975, -9.363379034771801557, -172.8437500020484094 ) ) ;
#19944=CARTESIAN_POINT ( 'NONE',  ( 5.000000000000000000, 8.660254037844385522, -194.1250000040967905 ) ) ;
#19947=CARTESIAN_POINT ( 'NONE',  ( 10.81189881249999907, 6.242252689847868297, -97.21875000204836681 ) ) ;
#19949=CARTESIAN_POINT ( 'NONE',  ( -5.405949406249996869, 9.363379034771805109, -64.03125000204836681 ) ) ;
#19952=CARTESIAN_POINT ( 'NONE',  ( 5.405949406249999534, 9.363379034771803333, -124.2812500020483952 ) ) ;
#19953=CARTESIAN_POINT ( 'NONE',  ( -10.81189881249999729, -6.242252689847864744, -161.1562500020484094 ) ) ;
#19955=CARTESIAN_POINT ( 'NONE',  ( 9.999999999999996447, -5.773502691896262640, -136.0000000040967905 ) ) ;
#19957=( BOUNDED_CURVE ( )  B_SPLINE_CURVE ( 2, ( #22090, #41707, #41280, #14947, #35477, #12353, #28577 ),
 .UNSPECIFIED., .F., .F. ) 
 B_SPLINE_CURVE_WITH_KNOTS ( ( 3, 2, 2, 3 ),
 ( 0.2350746268656717097, 0.2363184079601990950, 0.2375621890547264525, 0.2388059701492538378 ),
 .UNSPECIFIED. ) 
 CURVE ( )  GEOMETRIC_REPRESENTATION_ITEM ( )  RATIONAL_B_SPLINE_CURVE ( ( 0.9999999999999940048, 0.8660254037844447028, 1.000000000000000000, 0.8660254037844387076, 1.000000000000000000, 0.8660254037844267172, 1.000000000000011990 ) ) 
 REPRESENTATION_ITEM ( '' )  );
#19958=ORIENTED_EDGE ( 'NONE', *, *, #38584, .T. ) ;
#19962=CARTESIAN_POINT ( 'NONE',  ( 10.81189881249999907, 6.242252689847868297, -191.9062500020484094 ) ) ;
#19963=DIRECTION ( 'NONE',  ( -0.000000000000000000, -0.000000000000000000, 1.000000000000000000 ) ) ;
#19966=CARTESIAN_POINT ( 'NONE',  ( 10.00000000000000000, 5.773502691896255534, -60.37499999999997868 ) ) ;
#19968=CARTESIAN_POINT ( 'NONE',  ( -9.999999999999998224, 1.224646799147353059E-15, -66.12500000409676204 ) ) ;
#19969=CARTESIAN_POINT ( 'NONE',  ( 7.070501591499376803E-16, 11.54700538379251284, -153.1250000000000000 ) ) ;
#19970=CARTESIAN_POINT ( 'NONE',  ( -5.000000000000003553, -8.660254037844383745, -145.0000000000000000 ) ) ;
#19972=CARTESIAN_POINT ( 'NONE',  ( 5.405949406249992428, -9.363379034771808662, -57.28125000204836681 ) ) ;
#19975=CARTESIAN_POINT ( 'NONE',  ( 10.81189881249999907, 6.242252689847868297, -187.4062500020484379 ) ) ;
#19981=CARTESIAN_POINT ( 'NONE',  ( -9.999999999999998224, 5.773502691896259087, -169.3750000000000000 ) ) ;
#19983=CARTESIAN_POINT ( 'NONE',  ( 5.405949406249999534, 9.363379034771803333, -97.28125000204839523 ) ) ;
#19984=ORIENTED_EDGE ( 'NONE', *, *, #11850, .T. ) ;
#19985=CARTESIAN_POINT ( 'NONE',  ( 7.070501591499376803E-16, 11.54700538379251284, -83.00000000409676204 ) ) ;
#19986=ORIENTED_EDGE ( 'NONE', *, *, #42543, .T. ) ;
#19987=ORIENTED_EDGE ( 'NONE', *, *, #25157, .F. ) ;
#19988=CARTESIAN_POINT ( 'NONE',  ( -10.81189881249999907, -6.242252689847864744, -36.46875000204835970 ) ) ;
#19989=CARTESIAN_POINT ( 'NONE',  ( -5.405949406249996869, 9.363379034771805109, -19.03125000204835970 ) ) ;
#19991=CARTESIAN_POINT ( 'NONE',  ( 10.81189881249999729, 0.000000000000000000, -70.34375000204836681 ) ) ;
#19993=CARTESIAN_POINT ( 'NONE',  ( -5.405949406250003975, -9.363379034771801557, -189.3437500020483810 ) ) ;
#19994=CARTESIAN_POINT ( 'NONE',  ( -10.81189881249999729, 6.242252689847871849, -149.2187500020484379 ) ) ;
#19995=EDGE_CURVE ( 'NONE', #1371, #34292, #39111, .T. ) ;
#19996=CARTESIAN_POINT ( 'NONE',  ( -4.999999999999996447, 8.660254037844387298, -132.3750000040967905 ) ) ;
#19997=CARTESIAN_POINT ( 'NONE',  ( 9.999999999999998224, 0.000000000000000000, -56.37500000409676204 ) ) ;
#19999=CARTESIAN_POINT ( 'NONE',  ( 4.999999999999992006, -8.660254037844389075, -2.625000004096766926 ) ) ;
#20000=CARTESIAN_POINT ( 'NONE',  ( 5.321294541346989426, 5.321294541346989426, -220.0000000000000000 ) ) ;
#20001=CARTESIAN_POINT ( 'NONE',  ( -10.81189881249999729, 1.324075727343319199E-15, -120.5937500020483952 ) ) ;
#20003=CARTESIAN_POINT ( 'NONE',  ( -5.405949406249996869, 9.363379034771805109, -86.53125000204838102 ) ) ;
#20004=CARTESIAN_POINT ( 'NONE',  ( -10.81189881249999729, 1.324075727343319199E-15, -110.0937500020483810 ) ) ;
#20007=CARTESIAN_POINT ( 'NONE',  ( -9.999999999999998224, 1.224646799147353059E-15, -160.6250000040967905 ) ) ;
#20008=LINE ( 'NONE', #40858, #29614 ) ;
#20013=CARTESIAN_POINT ( 'NONE',  ( 10.00000000000076916, -5.773502691895816774, -108.6249999999999858 ) ) ;
#20015=CARTESIAN_POINT ( 'NONE',  ( 9.999999999999996447, -5.773502691896262640, -78.62499999999998579 ) ) ;
#20017=CARTESIAN_POINT ( 'NONE',  ( 5.000000000000000000, 8.660254037844385522, -92.12500000409677625 ) ) ;
#20018=CYLINDRICAL_SURFACE ( 'NONE', #19633, 9.999999999999998224 ) ;
#20020=CARTESIAN_POINT ( 'NONE',  ( -5.405949406249996869, 9.363379034771805109, -85.03125000204838102 ) ) ;
#20021=VERTEX_POINT ( 'NONE', #5694 ) ;
#20022=EDGE_CURVE ( 'NONE', #21267, #11337, #2254, .T. ) ;
#20026=EDGE_LOOP ( 'NONE', ( #30935, #34115, #37863, #13043 ) ) ;
#20027=CARTESIAN_POINT ( 'NONE',  ( 9.999999999999998224, 0.000000000000000000, -10.99999999999995381 ) ) ;
#20028=ADVANCED_FACE ( 'NONE', ( #2660 ), #31597, .T. ) ;
#20029=CARTESIAN_POINT ( 'NONE',  ( 7.070501591499377789E-16, 11.54700538379251284, -148.6250000000000000 ) ) ;
#20032=CARTESIAN_POINT ( 'NONE',  ( -9.999999999999998224, 1.224646799147353059E-15, -187.2500000000000000 ) ) ;
#20033=CARTESIAN_POINT ( 'NONE',  ( -4.999999999999996447, 8.660254037844387298, -95.99999999999998579 ) ) ;
#20034=CARTESIAN_POINT ( 'NONE',  ( -10.81189881249999907, -6.242252689847864744, -119.1562500020484237 ) ) ;
#20035=VERTEX_POINT ( 'NONE', #28990 ) ;
#20036=DIRECTION ( 'NONE',  ( -0.000000000000000000, -0.000000000000000000, 1.000000000000000000 ) ) ;
#20037=ORIENTED_EDGE ( 'NONE', *, *, #2566, .T. ) ;
#20038=CARTESIAN_POINT ( 'NONE',  ( -5.405949406250003975, -9.363379034771801557, -48.53125000204838813 ) ) ;
#20041=CARTESIAN_POINT ( 'NONE',  ( 10.81189881249999551, -6.242252689847874514, -95.96875000204838102 ) ) ;
#20042=CARTESIAN_POINT ( 'NONE',  ( 10.81189881249999729, 0.000000000000000000, -126.0312500020483952 ) ) ;
#20043=VERTEX_POINT ( 'NONE', #25755 ) ;
#20045=CYLINDRICAL_SURFACE ( 'NONE', #39406, 9.999999999999998224 ) ;
#20048=EDGE_CURVE ( 'NONE', #32999, #25200, #16301, .T. ) ;
#20049=CARTESIAN_POINT ( 'NONE',  ( -10.81189881249999729, 1.324075727343319199E-15, -129.5937500020483810 ) ) ;
#20051=CYLINDRICAL_SURFACE ( 'NONE', #24255, 9.999999999999998224 ) ;
#20053=CARTESIAN_POINT ( 'NONE',  ( 9.999999999999996447, -5.773502691896262640, -188.5000000040968189 ) ) ;
#20055=CARTESIAN_POINT ( 'NONE',  ( 5.405949406249999534, 9.363379034771803333, -188.7812500020484094 ) ) ;
#20060=CARTESIAN_POINT ( 'NONE',  ( 5.405949406249999534, 9.363379034771803333, -59.59375000204835970 ) ) ;
#20061=CARTESIAN_POINT ( 'NONE',  ( -5.405949406249996869, 9.363379034771805109, -45.84375000204838102 ) ) ;
#20063=CARTESIAN_POINT ( 'NONE',  ( 10.81189881249999907, 6.242252689847868297, -14.90625000204837036 ) ) ;
#20065=CARTESIAN_POINT ( 'NONE',  ( 9.999999999999998224, 0.000000000000000000, -146.0000000000000000 ) ) ;
#20067=CARTESIAN_POINT ( 'NONE',  ( 9.999999999999998224, 0.000000000000000000, -102.5000000000000000 ) ) ;
#20069=CARTESIAN_POINT ( 'NONE',  ( -4.999999999999996447, 8.660254037844387298, -118.8750000040967905 ) ) ;
#20072=CARTESIAN_POINT ( 'NONE',  ( -10.81189881249999729, -6.242252689847864744, -110.1562500020483952 ) ) ;
#20073=ORIENTED_EDGE ( 'NONE', *, *, #40070, .T. ) ;
#20074=AXIS2_PLACEMENT_3D ( 'NONE', #24727, #41729, #15401 ) ;
#20080=CARTESIAN_POINT ( 'NONE',  ( 7.070501591499377789E-16, 11.54700538379251284, -31.62499999999995737 ) ) ;
#20082=CARTESIAN_POINT ( 'NONE',  ( -10.00000000000000000, -5.773502691896251982, -16.50000000409675849 ) ) ;
#20083=CARTESIAN_POINT ( 'NONE',  ( -10.81189881249999729, 6.242252689847871849, -47.40625000204836681 ) ) ;
#20086=( BOUNDED_CURVE ( )  B_SPLINE_CURVE ( 2, ( #28668, #32537, #3177, #22387, #25426, #42431, #15881 ),
 .UNSPECIFIED., .F., .F. ) 
 B_SPLINE_CURVE_WITH_KNOTS ( ( 3, 2, 2, 3 ),
 ( 0.1641791044776119424, 0.1654228855721392999, 0.1666666666666666574, 0.1679104477611940427 ),
 .UNSPECIFIED. ) 
 CURVE ( )  GEOMETRIC_REPRESENTATION_ITEM ( )  RATIONAL_B_SPLINE_CURVE ( ( 1.000000000000000000, 0.8660254037844387076, 1.000000000000000000, 0.8660254037844387076, 1.000000000000000000, 0.8660254037844387076, 1.000000000000000000 ) ) 
 REPRESENTATION_ITEM ( '' )  );
#20089=CARTESIAN_POINT ( 'NONE',  ( -10.81189881249999729, 1.324075727343319199E-15, -143.2812500020483810 ) ) ;
#20091=ORIENTED_EDGE ( 'NONE', *, *, #14883, .F. ) ;
#20093=VERTEX_POINT ( 'NONE', #13399 ) ;
#20095=DIRECTION ( 'NONE',  ( 1.000000000000000000, 0.000000000000000000, 0.000000000000000000 ) ) ;
#20096=CARTESIAN_POINT ( 'NONE',  ( 10.81189881249999729, 0.000000000000000000, -175.3437500020483810 ) ) ;
#20097=EDGE_CURVE ( 'NONE', #25539, #5420, #85, .T. ) ;
#20098=CARTESIAN_POINT ( 'NONE',  ( 5.405949406249992428, -9.363379034771808662, -22.59375000204835615 ) ) ;
#20103=CARTESIAN_POINT ( 'NONE',  ( 7.644554776091147741E-16, 12.48450537969573659, -156.9687500020484094 ) ) ;
#20104=CARTESIAN_POINT ( 'NONE',  ( -5.405949406250003975, -9.363379034771801557, -136.8437500020484094 ) ) ;
#20105=EDGE_CURVE ( 'NONE', #37673, #33065, #26292, .T. ) ;
#20109=CARTESIAN_POINT ( 'NONE',  ( -2.293366432827344421E-15, -12.48450537969573659, -13.71875000204836503 ) ) ;
#20116=VECTOR ( 'NONE', #30087, 1000.000000000000000 ) ;
#20117=CARTESIAN_POINT ( 'NONE',  ( -5.405949406250003975, -9.363379034771801557, -84.34375000204836681 ) ) ;
#20118=CARTESIAN_POINT ( 'NONE',  ( 7.644554776091147741E-16, 12.48450537969573659, -69.96875000204838102 ) ) ;
#20119=CARTESIAN_POINT ( 'NONE',  ( 5.405949406249999534, 9.363379034771803333, -46.28125000204838813 ) ) ;
#20121=CARTESIAN_POINT ( 'NONE',  ( 9.999999999999998224, 0.000000000000000000, -138.8750000040968189 ) ) ;
#20123=CARTESIAN_POINT ( 'NONE',  ( 9.999999999999998224, 0.000000000000000000, -129.5000000000000000 ) ) ;
#20124=CARTESIAN_POINT ( 'NONE',  ( 10.81189881249999729, 6.242252689847867408, -139.4062500020484094 ) ) ;
#20131=CARTESIAN_POINT ( 'NONE',  ( -5.405949406249996869, 9.363379034771805109, -164.5312500020484094 ) ) ;
#20132=CARTESIAN_POINT ( 'NONE',  ( 9.999999999999998224, 0.000000000000000000, -41.37500000409677625 ) ) ;
#20133=EDGE_CURVE ( 'NONE', #21791, #29783, #6736, .T. ) ;
#20134=CARTESIAN_POINT ( 'NONE',  ( -9.999999999999998224, 1.224646799147353059E-15, -154.6250000040967905 ) ) ;
#20136=CARTESIAN_POINT ( 'NONE',  ( -9.999999999999998224, 1.224646799147353059E-15, -64.24999999999997158 ) ) ;
#20137=CARTESIAN_POINT ( 'NONE',  ( -2.293366432827344421E-15, -12.48450537969573659, -160.9062500020483810 ) ) ;
#20138=EDGE_CURVE ( 'NONE', #24966, #6565, #39518, .T. ) ;
#20139=CARTESIAN_POINT ( 'NONE',  ( 10.81189881249999551, -6.242252689847874514, -136.4687500020483810 ) ) ;
#20140=DIRECTION ( 'NONE',  ( -0.000000000000000000, -0.000000000000000000, 1.000000000000000000 ) ) ;
#20141=CARTESIAN_POINT ( 'NONE',  ( 9.999999999999998224, 0.000000000000000000, -152.0000000000000000 ) ) ;
#20144=PLANE ( 'NONE',  #25901 ) ;
#20146=CARTESIAN_POINT ( 'NONE',  ( -5.405949406249996869, 9.363379034771805109, -71.53125000204838102 ) ) ;
#20147=ORIENTED_EDGE ( 'NONE', *, *, #33532, .F. ) ;
#20148=CARTESIAN_POINT ( 'NONE',  ( -10.81189881249999729, 6.242252689847871849, -116.2187500020483810 ) ) ;
#20149=ORIENTED_EDGE ( 'NONE', *, *, #26939, .F. ) ;
#20150=CARTESIAN_POINT ( 'NONE',  ( 10.81189881249999729, 0.000000000000000000, -22.34375000204835615 ) ) ;
#20151=CARTESIAN_POINT ( 'NONE',  ( -10.81189881249999907, -6.242252689847864744, -195.4687500020484094 ) ) ;
#20152=CARTESIAN_POINT ( 'NONE',  ( 5.405949406249992428, -9.363379034771808662, -45.09375000204837391 ) ) ;
#20153=CARTESIAN_POINT ( 'NONE',  ( 9.999999999999998224, 0.000000000000000000, -200.0000000000000000 ) ) ;
#20155=CARTESIAN_POINT ( 'NONE',  ( 5.405949406249992428, -9.363379034771808662, -177.0937500020484094 ) ) ;
#20156=CARTESIAN_POINT ( 'NONE',  ( -10.81189881249999907, -6.242252689847864744, -171.4687500020484094 ) ) ;
#20159=EDGE_CURVE ( 'NONE', #13374, #34507, #13023, .T. ) ;
#20161=CARTESIAN_POINT ( 'NONE',  ( 9.999999999999998224, 0.000000000000000000, -141.8750000040967905 ) ) ;
#20163=CARTESIAN_POINT ( 'NONE',  ( -10.81189881249999729, 1.324075727343319199E-15, -98.09375000204838102 ) ) ;
#20165=CARTESIAN_POINT ( 'NONE',  ( -2.293366432827344421E-15, -12.48450537969573659, -64.90625000204838102 ) ) ;
#20168=CARTESIAN_POINT ( 'NONE',  ( -5.405949406250003975, -9.363379034771801557, -119.0312500020483952 ) ) ;
#20169=CARTESIAN_POINT ( 'NONE',  ( -10.81189881249999729, 1.324075727343319199E-15, -159.7812500020484094 ) ) ;
#20170=( BOUNDED_CURVE ( )  B_SPLINE_CURVE ( 2, ( #3488, #16625, #12754, #482, #19878, #16836, #29828 ),
 .UNSPECIFIED., .F., .F. ) 
 B_SPLINE_CURVE_WITH_KNOTS ( ( 3, 2, 2, 3 ),
 ( 0.9141791044776121922, 0.9154228855721395774, 0.9166666666666669627, 0.9179104477611943480 ),
 .UNSPECIFIED. ) 
 CURVE ( )  GEOMETRIC_REPRESENTATION_ITEM ( )  RATIONAL_B_SPLINE_CURVE ( ( 0.9999999999999761302, 0.8660254037844625774, 1.000000000000000000, 0.8660254037844387076, 1.000000000000000000, 0.8660254037844028474, 1.000000000000035971 ) ) 
 REPRESENTATION_ITEM ( '' )  );
#20172=CARTESIAN_POINT ( 'NONE',  ( 5.000000000000000000, 8.660254037844385522, -134.1250000040967620 ) ) ;
#20174=ORIENTED_EDGE ( 'NONE', *, *, #27900, .F. ) ;
#20177=CARTESIAN_POINT ( 'NONE',  ( 7.644554776091147741E-16, 12.48450537969573659, -191.6562500020484094 ) ) ;
#20180=VERTEX_POINT ( 'NONE', #29840 ) ;
#20181=CARTESIAN_POINT ( 'NONE',  ( 7.070501591499377789E-16, 11.54700538379251284, -55.62499999999997868 ) ) ;
#20183=CARTESIAN_POINT ( 'NONE',  ( -9.999999999999998224, 5.773502691896259087, -66.25000000409677625 ) ) ;
#20184=DIRECTION ( 'NONE',  ( 1.000000000000000000, 0.000000000000000000, 0.000000000000000000 ) ) ;
#20187=CARTESIAN_POINT ( 'NONE',  ( -10.81189881249999729, 1.324075727343319199E-15, -59.28125000204836681 ) ) ;
#20192=CARTESIAN_POINT ( 'NONE',  ( -10.81189881249999729, 6.242252689847871849, -183.9062500020484094 ) ) ;
#20194=CARTESIAN_POINT ( 'NONE',  ( -5.000000000000003553, -8.660254037844383745, -172.3750000040968189 ) ) ;
#20196=CARTESIAN_POINT ( 'NONE',  ( -9.999999999999998224, 1.224646799147353059E-15, -46.24999999999998579 ) ) ;
#20197=CARTESIAN_POINT ( 'NONE',  ( 0.000000000000000000, 0.000000000000000000, -200.0000000000000000 ) ) ;
#20198=CARTESIAN_POINT ( 'NONE',  ( 10.00000000000025402, -5.773502691896113426, -122.1250000000000000 ) ) ;
#20199=CARTESIAN_POINT ( 'NONE',  ( 10.81189881249999729, 0.000000000000000000, -96.03125000204838102 ) ) ;
#20200=ORIENTED_EDGE ( 'NONE', *, *, #948, .T. ) ;
#20201=CARTESIAN_POINT ( 'NONE',  ( 5.000000000000000000, 8.660254037844385522, -24.62500000409675849 ) ) ;
#20202=CARTESIAN_POINT ( 'NONE',  ( -4.999999999999996447, 8.660254037844387298, -162.0000000000000000 ) ) ;
#20203=EDGE_LOOP ( 'NONE', ( #32721, #16248, #37404, #11594, #22240, #4416 ) ) ;
#20204=VERTEX_POINT ( 'NONE', #15209 ) ;
#20205=CARTESIAN_POINT ( 'NONE',  ( -2.293366432827344421E-15, -12.48450537969573659, -31.71875000204834905 ) ) ;
#20206=CARTESIAN_POINT ( 'NONE',  ( -10.81189881249999907, -6.242252689847864744, -20.15625000204838102 ) ) ;
#20207=CARTESIAN_POINT ( 'NONE',  ( 10.81189881249999907, 6.242252689847868297, -71.71875000204838102 ) ) ;
#20208=CARTESIAN_POINT ( 'NONE',  ( -9.999999999999998224, 1.224646799147353059E-15, -18.12500000409675138 ) ) ;
#20210=CARTESIAN_POINT ( 'NONE',  ( 10.81189881249999729, 0.000000000000000000, -194.8437500020484094 ) ) ;
#20211=CARTESIAN_POINT ( 'NONE',  ( -5.405949406250003975, -9.363379034771801557, -148.8437500020483810 ) ) ;
#20213=CARTESIAN_POINT ( 'NONE',  ( 4.999999999999992006, -8.660254037844389075, -79.12500000409677625 ) ) ;
#20214=CARTESIAN_POINT ( 'NONE',  ( 5.000000000000000000, 8.660254037844385522, -112.7499999999999858 ) ) ;
#20216=CARTESIAN_POINT ( 'NONE',  ( 9.999999999999996447, -5.773502691896262640, -4.000000004096762929 ) ) ;
#20217=CARTESIAN_POINT ( 'NONE',  ( 10.81189881249999551, -6.242252689847874514, -124.4687500020483952 ) ) ;
#20218=CARTESIAN_POINT ( 'NONE',  ( 9.999999999999998224, 0.000000000000000000, -200.0000000000000000 ) ) ;
#20219=CARTESIAN_POINT ( 'NONE',  ( -10.81189881249999907, -6.242252689847864744, -89.15625000204839523 ) ) ;
#20220=CARTESIAN_POINT ( 'NONE',  ( -2.293366432827344421E-15, -12.48450537969573659, -105.2187500020483952 ) ) ;
#20223=CARTESIAN_POINT ( 'NONE',  ( 9.999999999999998224, 0.000000000000000000, -158.3750000040967905 ) ) ;
#20226=EDGE_CURVE ( 'NONE', #28132, #4695, #13281, .T. ) ;
#20231=CARTESIAN_POINT ( 'NONE',  ( 5.000000000000000000, 8.660254037844385522, -82.74999999999997158 ) ) ;
#20233=CARTESIAN_POINT ( 'NONE',  ( -9.999999999999998224, 1.224646799147353059E-15, -90.12500000409677625 ) ) ;
#20234=CARTESIAN_POINT ( 'NONE',  ( 9.999999999999998224, 0.000000000000000000, -168.8750000040967905 ) ) ;
#20236=CARTESIAN_POINT ( 'NONE',  ( 10.81189881249999729, 6.242252689847867408, -83.90625000204836681 ) ) ;
#20237=ORIENTED_EDGE ( 'NONE', *, *, #11922, .F. ) ;
#20239=LINE ( 'NONE', #33428, #13226 ) ;
#20242=CARTESIAN_POINT ( 'NONE',  ( 7.070501591499377789E-16, 11.54700538379251284, -10.62499999999995381 ) ) ;
#20244=CARTESIAN_POINT ( 'NONE',  ( 5.000000000000000000, 8.660254037844385522, -145.7500000000000000 ) ) ;
#20245=CARTESIAN_POINT ( 'NONE',  ( 10.00000000000154010, -5.773502691895370020, -14.50000000409672296 ) ) ;
#20247=EDGE_CURVE ( 'NONE', #37944, #32539, #17691, .T. ) ;
#20248=CARTESIAN_POINT ( 'NONE',  ( -4.999999999999996447, 8.660254037844387298, -189.0000000000000000 ) ) ;
#20250=CARTESIAN_POINT ( 'NONE',  ( -10.81189881249999729, 6.242252689847871849, -117.9062500020483952 ) ) ;
#20251=VERTEX_POINT ( 'NONE', #8548 ) ;
#20252=CARTESIAN_POINT ( 'NONE',  ( -2.121150477449813534E-15, -11.54700538379251284, -74.75000000409677625 ) ) ;
#20254=B_SPLINE_CURVE_WITH_KNOTS ( 'NONE', 3,
 ( #5192, #40783, #11864, #24633, #25062, #4547, #27430, #31104, #1536, #14671, #37778, #11646, #20942, #34984, #21371, #18126, #21592, #24203, #4982, #8441, #40564, #1754, #34127, #24848, #17688, #14882, #37995, #26105 ),
 .UNSPECIFIED., .F., .F.,
 ( 4, 2, 2, 2, 2, 2, 2, 2, 2, 2, 2, 2, 2, 4 ),
 ( 0.000000000000000000, 0.001274091078800513406, 0.002548182157601026811, 0.005096364315202054490, 0.006370455394002568980, 0.007644546472803081735, 0.01019272863040411072, 0.01146681970920462521, 0.01274091078800513796, 0.01401500186680565245, 0.01528909294560616347, 0.01656318402440667623, 0.01783727510320719245, 0.02038545726080821796 ),
 .UNSPECIFIED. ) ;
#20255=ORIENTED_EDGE ( 'NONE', *, *, #11922, .T. ) ;
#20256=CARTESIAN_POINT ( 'NONE',  ( 10.81189881249999729, 0.000000000000000000, -46.53125000204838813 ) ) ;
#20259=CARTESIAN_POINT ( 'NONE',  ( -5.405949406249996869, 9.363379034771805109, -93.84375000204838102 ) ) ;
#20260=CARTESIAN_POINT ( 'NONE',  ( -10.81189881249999729, 6.242252689847871849, -120.9062500020483952 ) ) ;
#20261=EDGE_LOOP ( 'NONE', ( #11114, #2243, #2760, #2814 ) ) ;
#20262=CARTESIAN_POINT ( 'NONE',  ( -9.999999999998456346, -5.773502691897145489, -83.62499999999994316 ) ) ;
#20263=CARTESIAN_POINT ( 'NONE',  ( 10.81189881249999729, 6.242252689847867408, -197.7187500020484094 ) ) ;
#20265=CARTESIAN_POINT ( 'NONE',  ( 5.000000000000000000, 8.660254037844385522, -0.6250000040967651493 ) ) ;
#20266=CARTESIAN_POINT ( 'NONE',  ( 5.405949406249999534, 9.363379034771803333, -133.0937500020483810 ) ) ;
#20268=CARTESIAN_POINT ( 'NONE',  ( -9.999999999999998224, 1.224646799147353059E-15, -17.74999999999996092 ) ) ;
#20270=CARTESIAN_POINT ( 'NONE',  ( -4.999999999999996447, 8.660254037844387298, -184.8750000040967905 ) ) ;
#20272=CARTESIAN_POINT ( 'NONE',  ( -5.405949406249996869, 9.363379034771805109, -178.0312500020483810 ) ) ;
#20273=EDGE_CURVE ( 'NONE', #13430, #6396, #22132, .T. ) ;
#20275=CARTESIAN_POINT ( 'NONE',  ( 9.999999999999998224, 0.000000000000000000, -122.3750000040967905 ) ) ;
#20277=CARTESIAN_POINT ( 'NONE',  ( -10.81189881249999729, 1.324075727343319199E-15, -59.09375000204835970 ) ) ;
#20278=CARTESIAN_POINT ( 'NONE',  ( -5.405949406250003975, -9.363379034771801557, -43.84375000204837391 ) ) ;
#20280=CARTESIAN_POINT ( 'NONE',  ( 10.81189881249999551, -6.242252689847874514, -21.15625000204836681 ) ) ;
#20283=CARTESIAN_POINT ( 'NONE',  ( 5.000000000000000000, 8.660254037844385522, -108.2499999999999858 ) ) ;
#20288=CARTESIAN_POINT ( 'NONE',  ( 10.81189881249999729, 0.000000000000000000, -109.5312500020483810 ) ) ;
#20289=EDGE_LOOP ( 'NONE', ( #31160, #11275, #35249, #41264 ) ) ;
#20290=CARTESIAN_POINT ( 'NONE',  ( -9.999999999999998224, 1.224646799147353059E-15, -160.2500000000000000 ) ) ;
#20293=ORIENTED_EDGE ( 'NONE', *, *, #15218, .F. ) ;
#20294=CARTESIAN_POINT ( 'NONE',  ( -9.999999999999998224, 5.773502691896259087, -37.37499999999995026 ) ) ;
#20295=CARTESIAN_POINT ( 'NONE',  ( 7.644554776091147741E-16, 12.48450537969573659, -34.15625000204836681 ) ) ;
#20296=CARTESIAN_POINT ( 'NONE',  ( 7.070501591499376803E-16, 11.54700538379251284, -111.5000000040967763 ) ) ;
#20299=CARTESIAN_POINT ( 'NONE',  ( 10.81189881249999907, 6.242252689847868297, -140.9062500020484094 ) ) ;
#20302=ORIENTED_EDGE ( 'NONE', *, *, #40683, .T. ) ;
#20305=DIRECTION ( 'NONE',  ( -0.000000000000000000, -0.000000000000000000, 1.000000000000000000 ) ) ;
#20306=CARTESIAN_POINT ( 'NONE',  ( 10.81189881249999729, 0.000000000000000000, -166.3437500020484094 ) ) ;
#20308=CARTESIAN_POINT ( 'NONE',  ( 5.405949406249992428, -9.363379034771808662, -27.09375000204835970 ) ) ;
#20309=LINE ( 'NONE', #27217, #6074 ) ;
#20310=CARTESIAN_POINT ( 'NONE',  ( -10.81189881249999729, 6.242252689847871849, -156.7187500020483810 ) ) ;
#20311=CARTESIAN_POINT ( 'NONE',  ( -5.405949406250003975, -9.363379034771801557, -138.3437500020484094 ) ) ;
#20312=CARTESIAN_POINT ( 'NONE',  ( -9.999999999999479527, -5.773502691896549521, -88.50000000409676204 ) ) ;
#20316=CARTESIAN_POINT ( 'NONE',  ( 10.81189881249999907, 6.242252689847868297, -13.21875000204836148 ) ) ;
#20318=LINE ( 'NONE', #20748, #20558 ) ;
#20319=CARTESIAN_POINT ( 'NONE',  ( -4.999999999999996447, 8.660254037844387298, -124.8750000040967763 ) ) ;
#20322=CARTESIAN_POINT ( 'NONE',  ( -10.81189881249999729, -6.242252689847864744, -87.46875000204836681 ) ) ;
#20323=CARTESIAN_POINT ( 'NONE',  ( 5.405949406249992428, -9.363379034771808662, -66.09375000204836681 ) ) ;
#20324=CARTESIAN_POINT ( 'NONE',  ( 10.81189881249999907, 6.242252689847868297, -40.40625000204836681 ) ) ;
#20326=CARTESIAN_POINT ( 'NONE',  ( -9.999999999999998224, 1.224646799147353059E-15, -185.7500000000000000 ) ) ;
#20328=CARTESIAN_POINT ( 'NONE',  ( 9.999999999999998224, 0.000000000000000000, -132.5000000000000000 ) ) ;
#20329=CARTESIAN_POINT ( 'NONE',  ( -5.405949406250003975, -9.363379034771801557, -140.0312500020484094 ) ) ;
#20331=AXIS2_PLACEMENT_3D ( 'NONE', #26981, #39716, #9730 ) ;
#20333=CARTESIAN_POINT ( 'NONE',  ( -5.405949406250003975, -9.363379034771801557, -20.03125000204836326 ) ) ;
#20338=CARTESIAN_POINT ( 'NONE',  ( 10.00000000000031619, -5.773502691896077010, -185.1250000000000000 ) ) ;
#20339=CARTESIAN_POINT ( 'NONE',  ( 5.000000000000000000, 8.660254037844385522, -45.62500000409677625 ) ) ;
#20340=CARTESIAN_POINT ( 'NONE',  ( 9.999999999999612754, 5.773502691896477579, -155.2500000040967905 ) ) ;
#20342=AXIS2_PLACEMENT_3D ( 'NONE', #22472, #23112, #29373 ) ;
#20343=CARTESIAN_POINT ( 'NONE',  ( -9.999999999999998224, 1.224646799147353059E-15, -40.62500000409677625 ) ) ;
#20344=CARTESIAN_POINT ( 'NONE',  ( -10.81189881249999907, -6.242252689847864744, -150.6562500020484094 ) ) ;
#20345=CARTESIAN_POINT ( 'NONE',  ( 5.405949406249992428, -9.363379034771808662, -133.5937500020483810 ) ) ;
#20346=CARTESIAN_POINT ( 'NONE',  ( 0.000000000000000000, 0.000000000000000000, -200.0000000000000000 ) ) ;
#20348=ORIENTED_EDGE ( 'NONE', *, *, #7198, .T. ) ;
#20349=EDGE_CURVE ( 'NONE', #8431, #18936, #17435, .T. ) ;
#20350=CARTESIAN_POINT ( 'NONE',  ( -2.121150477449813534E-15, -11.54700538379251284, -78.87500000000000000 ) ) ;
#20351=CARTESIAN_POINT ( 'NONE',  ( 7.644554776091147741E-16, 12.48450537969573659, -65.65625000204838102 ) ) ;
#20352=ORIENTED_EDGE ( 'NONE', *, *, #901, .T. ) ;
#20354=CARTESIAN_POINT ( 'NONE',  ( 10.81189881249999729, 0.000000000000000000, -116.8437500020483810 ) ) ;
#20356=CARTESIAN_POINT ( 'NONE',  ( -5.405949406250003975, -9.363379034771801557, -19.84375000204835615 ) ) ;
#20357=CARTESIAN_POINT ( 'NONE',  ( -5.405949406249996869, 9.363379034771805109, -188.3437500020483810 ) ) ;
#20358=CARTESIAN_POINT ( 'NONE',  ( -5.405949406249996869, 9.363379034771805109, -48.84375000204838102 ) ) ;
#20359=CARTESIAN_POINT ( 'NONE',  ( -9.999999999999998224, 1.224646799147353059E-15, -151.6250000040967905 ) ) ;
#20360=CARTESIAN_POINT ( 'NONE',  ( 10.81189881249999551, -6.242252689847874514, -182.9687500020484094 ) ) ;
#20361=VECTOR ( 'NONE', #41041, 1000.000000000000000 ) ;
#20362=CARTESIAN_POINT ( 'NONE',  ( 10.81189881249999551, -6.242252689847874514, -160.4687500020484094 ) ) ;
#20366=CARTESIAN_POINT ( 'NONE',  ( -4.999999999999996447, 8.660254037844387298, -35.99999999999997868 ) ) ;
#20368=CARTESIAN_POINT ( 'NONE',  ( -2.293366432827344421E-15, -12.48450537969573659, -96.21875000204839523 ) ) ;
#20370=CARTESIAN_POINT ( 'NONE',  ( 5.405949406249999534, 9.363379034771803333, -67.28125000204838102 ) ) ;
#20373=CARTESIAN_POINT ( 'NONE',  ( 10.81189881249999551, -6.242252689847874514, -118.6562500020483952 ) ) ;
#20374=CARTESIAN_POINT ( 'NONE',  ( -5.405949406249996869, 9.363379034771805109, -158.5312500020484094 ) ) ;
#20376=CARTESIAN_POINT ( 'NONE',  ( 9.999999999999998224, 0.000000000000000000, -141.8750000040967905 ) ) ;
#20378=ORIENTED_EDGE ( 'NONE', *, *, #20138, .T. ) ;
#20381=CARTESIAN_POINT ( 'NONE',  ( -10.81189881249999729, 1.324075727343319199E-15, -191.2812500020484094 ) ) ;
#20383=ORIENTED_EDGE ( 'NONE', *, *, #13519, .T. ) ;
#20384=CARTESIAN_POINT ( 'NONE',  ( 10.00000000000000000, 5.773502691896255534, -49.87499999999997868 ) ) ;
#20386=CARTESIAN_POINT ( 'NONE',  ( 10.00000000000000000, 5.773502691896255534, -68.25000000409679046 ) ) ;
#20387=CARTESIAN_POINT ( 'NONE',  ( 10.00000000000051159, -5.773502691895965988, -179.1250000000000000 ) ) ;
#20388=DIRECTION ( 'NONE',  ( 0.000000000000000000, 0.000000000000000000, -1.000000000000000000 ) ) ;
#20390=AXIS2_PLACEMENT_3D ( 'NONE', #1020, #14140, #10498 ) ;
#20391=CARTESIAN_POINT ( 'NONE',  ( -2.293366432827344421E-15, -12.48450537969573659, -58.90625000204838813 ) ) ;
#20394=CARTESIAN_POINT ( 'NONE',  ( -9.999999999998969713, -5.773502691896847949, -35.62499999999994316 ) ) ;
#20395=CARTESIAN_POINT ( 'NONE',  ( -10.81189881249999729, 1.324075727343319199E-15, -182.2812500020483810 ) ) ;
#20397=CARTESIAN_POINT ( 'NONE',  ( -5.000000000000003553, -8.660254037844383745, -87.99999999999998579 ) ) ;
#20398=CARTESIAN_POINT ( 'NONE',  ( -9.999999999999998224, 1.224646799147353059E-15, -164.7500000000000000 ) ) ;
#20399=EDGE_CURVE ( 'NONE', #33370, #24961, #21872, .T. ) ;
#20402=CARTESIAN_POINT ( 'NONE',  ( -9.999999999999998224, 1.224646799147353059E-15, -105.1250000040967763 ) ) ;
#20406=CARTESIAN_POINT ( 'NONE',  ( 5.405949406249999534, 9.363379034771803333, -89.78125000204838102 ) ) ;
#20407=ORIENTED_EDGE ( 'NONE', *, *, #32820, .F. ) ;
#20408=LINE ( 'NONE', #26473, #41364 ) ;
#20410=ORIENTED_EDGE ( 'NONE', *, *, #26988, .T. ) ;
#20413=CARTESIAN_POINT ( 'NONE',  ( -10.81189881249999907, -6.242252689847864744, -25.96875000204837391 ) ) ;
#20414=CARTESIAN_POINT ( 'NONE',  ( -5.405949406249996869, 9.363379034771805109, -22.03125000204836326 ) ) ;
#20416=CARTESIAN_POINT ( 'NONE',  ( 5.405949406249992428, -9.363379034771808662, -70.59375000204836681 ) ) ;
#20417=CARTESIAN_POINT ( 'NONE',  ( -9.999999999999998224, 1.224646799147353059E-15, -62.74999999999997158 ) ) ;
#20420=CARTESIAN_POINT ( 'NONE',  ( -2.293366432827344421E-15, -12.48450537969573659, -187.7187500020484094 ) ) ;
#20421=CARTESIAN_POINT ( 'NONE',  ( -5.405949406249996869, 9.363379034771805109, -149.3437500020483810 ) ) ;
#20422=( BOUNDED_CURVE ( )  B_SPLINE_CURVE ( 2, ( #26330, #9914, #20265, #9704, #26115, #36459, #6681 ),
 .UNSPECIFIED., .F., .F. ) 
 B_SPLINE_CURVE_WITH_KNOTS ( ( 3, 2, 2, 3 ),
 ( 0.9850746268656718208, 0.9863184079601992060, 0.9875621890547265913, 0.9888059701492539766 ),
 .UNSPECIFIED. ) 
 CURVE ( )  GEOMETRIC_REPRESENTATION_ITEM ( )  RATIONAL_B_SPLINE_CURVE ( ( 0.9999999999999761302, 0.8660254037844625774, 1.000000000000000000, 0.8660254037844387076, 1.000000000000000000, 0.8660254037844148378, 1.000000000000023981 ) ) 
 REPRESENTATION_ITEM ( '' )  );
#20423=VECTOR ( 'NONE', #14582, 1000.000000000000000 ) ;
#20424=EDGE_CURVE ( 'NONE', #30625, #1760, #35128, .T. ) ;
#20426=DIRECTION ( 'NONE',  ( 1.000000000000000000, 0.000000000000000000, 0.000000000000000000 ) ) ;
#20427=CARTESIAN_POINT ( 'NONE',  ( 5.000000000000000000, 8.660254037844385522, -2.125000004096766482 ) ) ;
#20429=CARTESIAN_POINT ( 'NONE',  ( 10.81189881249999729, 0.000000000000000000, -121.3437500020483952 ) ) ;
#20431=CARTESIAN_POINT ( 'NONE',  ( 10.81189881249999551, -6.242252689847874514, -91.65625000204838102 ) ) ;
#20432=CARTESIAN_POINT ( 'NONE',  ( -10.81189881249999729, -6.242252689847864744, -103.9687500020483810 ) ) ;
#20435=CARTESIAN_POINT ( 'NONE',  ( -9.999999999999998224, 5.773502691896259087, -159.2500000040967905 ) ) ;
#20442=CARTESIAN_POINT ( 'NONE',  ( -2.121150477449813534E-15, -11.54700538379251284, -83.37499999999997158 ) ) ;
#20444=CARTESIAN_POINT ( 'NONE',  ( 10.00000000000000000, 5.773502691896255534, -92.25000000409679046 ) ) ;
#20446=CARTESIAN_POINT ( 'NONE',  ( 5.405949406249999534, 9.363379034771803333, -83.78125000204838102 ) ) ;
#20448=DIRECTION ( 'NONE',  ( 1.000000000000000000, 0.000000000000000000, 0.000000000000000000 ) ) ;
#20450=ORIENTED_EDGE ( 'NONE', *, *, #35036, .T. ) ;
#20451=CARTESIAN_POINT ( 'NONE',  ( 4.999999999999992006, -8.660254037844389075, -8.249999999999952038 ) ) ;
#20453=CARTESIAN_POINT ( 'NONE',  ( 10.00000000000000000, 5.773502691896255534, -147.3750000000000000 ) ) ;
#20454=CARTESIAN_POINT ( 'NONE',  ( 7.070501591499376803E-16, 11.54700538379251284, -45.50000000409676915 ) ) ;
#20456=CARTESIAN_POINT ( 'NONE',  ( 7.644554776091147741E-16, 12.48450537969573659, -136.1562500020483810 ) ) ;
#20457=CARTESIAN_POINT ( 'NONE',  ( -9.999999999999998224, 1.224646799147353059E-15, -191.7500000000000000 ) ) ;
#20459=CARTESIAN_POINT ( 'NONE',  ( -10.81189881249999907, -6.242252689847864744, -114.6562500020483952 ) ) ;
#20461=CARTESIAN_POINT ( 'NONE',  ( 7.070501591499376803E-16, 11.54700538379251284, -36.50000000409675494 ) ) ;
#20462=ORIENTED_EDGE ( 'NONE', *, *, #20424, .T. ) ;
#20463=ORIENTED_EDGE ( 'NONE', *, *, #15202, .T. ) ;
#20464=( BOUNDED_CURVE ( )  B_SPLINE_CURVE ( 2, ( #41686, #9317, #42111, #12545, #12125, #25737, #22486 ),
 .UNSPECIFIED., .F., .F. ) 
 B_SPLINE_CURVE_WITH_KNOTS ( ( 3, 2, 2, 3 ),
 ( 0.2873134328358210032, 0.2885572139303483885, 0.2898009950248757183, 0.2910447761194031036 ),
 .UNSPECIFIED. ) 
 CURVE ( )  GEOMETRIC_REPRESENTATION_ITEM ( )  RATIONAL_B_SPLINE_CURVE ( ( 0.9999999999999880096, 0.8660254037844506980, 1.000000000000000000, 0.8660254037844387076, 1.000000000000000000, 0.8660254037844267172, 1.000000000000011990 ) ) 
 REPRESENTATION_ITEM ( '' )  );
#20465=CARTESIAN_POINT ( 'NONE',  ( -2.293366432827344421E-15, -12.48450537969573659, -42.40625000204837391 ) ) ;
#20468=CARTESIAN_POINT ( 'NONE',  ( -5.405949406249996869, 9.363379034771805109, -98.34375000204838102 ) ) ;
#20469=CARTESIAN_POINT ( 'NONE',  ( 10.81189881249999729, 0.000000000000000000, -127.5312500020483952 ) ) ;
#20471=CARTESIAN_POINT ( 'NONE',  ( 10.00000000000102318, -5.773502691895667560, -85.00000000409674783 ) ) ;
#20472=CARTESIAN_POINT ( 'NONE',  ( -10.81189881249999729, 6.242252689847871849, -194.2187500020484379 ) ) ;
#20475=CARTESIAN_POINT ( 'NONE',  ( 9.999999999999998224, 0.000000000000000000, -54.87500000409675494 ) ) ;
#20476=CARTESIAN_POINT ( 'NONE',  ( 10.81189881249999551, -6.242252689847874514, -122.9687500020483952 ) ) ;
#20478=DIRECTION ( 'NONE',  ( -0.000000000000000000, -0.000000000000000000, 1.000000000000000000 ) ) ;
#20480=CARTESIAN_POINT ( 'NONE',  ( -10.00000000000000000, -5.773502691896251982, -186.0000000040967905 ) ) ;
#20482=CARTESIAN_POINT ( 'NONE',  ( 7.644554776091147741E-16, 12.48450537969573659, -179.6562500020484094 ) ) ;
#20486=CARTESIAN_POINT ( 'NONE',  ( 10.81189881249999729, 6.242252689847867408, -59.71875000204836681 ) ) ;
#20487=CARTESIAN_POINT ( 'NONE',  ( -2.293366432827344421E-15, -12.48450537969573659, -39.21875000204835970 ) ) ;
#20489=CARTESIAN_POINT ( 'NONE',  ( -2.293366432827344421E-15, -12.48450537969573659, -7.906250002048370362 ) ) ;
#20491=CARTESIAN_POINT ( 'NONE',  ( 9.999999999999998224, 0.000000000000000000, -123.8750000040967905 ) ) ;
#20493=CARTESIAN_POINT ( 'NONE',  ( -4.999999999999996447, 8.660254037844387298, -106.4999999999999858 ) ) ;
#20495=CARTESIAN_POINT ( 'NONE',  ( 9.999999999999998224, 0.000000000000000000, -200.0000000000000000 ) ) ;
#20498=CARTESIAN_POINT ( 'NONE',  ( -10.81189881249999729, -6.242252689847864744, -107.1562500020483952 ) ) ;
#20499=ORIENTED_EDGE ( 'NONE', *, *, #17109, .F. ) ;
#20500=CARTESIAN_POINT ( 'NONE',  ( -9.999999999999998224, 1.224646799147353059E-15, -153.1250000040967905 ) ) ;
#20504=ORIENTED_EDGE ( 'NONE', *, *, #26372, .F. ) ;
#20505=CARTESIAN_POINT ( 'NONE',  ( 10.00000000000000000, 5.773502691896255534, -34.87499999999995026 ) ) ;
#20506=VECTOR ( 'NONE', #17225, 1000.000000000000000 ) ;
#20507=CARTESIAN_POINT ( 'NONE',  ( -10.81189881249999729, 6.242252689847871849, -36.90625000204835970 ) ) ;
#20511=CARTESIAN_POINT ( 'NONE',  ( -5.405949406249996869, 9.363379034771805109, -139.0312500020484094 ) ) ;
#20513=ORIENTED_EDGE ( 'NONE', *, *, #41905, .F. ) ;
#20515=CARTESIAN_POINT ( 'NONE',  ( -9.999999999999227285, -5.773502691896698735, -106.5000000040967336 ) ) ;
#20516=CARTESIAN_POINT ( 'NONE',  ( -9.999999999999998224, 1.224646799147353059E-15, -4.625000004096769146 ) ) ;
#20517=CARTESIAN_POINT ( 'NONE',  ( 5.405949406249992428, -9.363379034771808662, -169.5937500020484094 ) ) ;
#20519=CARTESIAN_POINT ( 'NONE',  ( 5.405949406249999534, 9.363379034771803333, -14.59375000204835082 ) ) ;
#20521=CARTESIAN_POINT ( 'NONE',  ( 10.81189881249999729, 0.000000000000000000, -155.8437500020483810 ) ) ;
#20522=CARTESIAN_POINT ( 'NONE',  ( -5.405949406250003975, -9.363379034771801557, -135.3437500020484094 ) ) ;
#20523=CARTESIAN_POINT ( 'NONE',  ( -10.81189881249999729, 1.324075727343319199E-15, -102.7812500020483952 ) ) ;
#20527=CARTESIAN_POINT ( 'NONE',  ( -10.81189881249999907, -6.242252689847864744, -9.468750002048359704 ) ) ;
#20530=DIRECTION ( 'NONE',  ( 1.000000000000000000, 0.000000000000000000, 0.000000000000000000 ) ) ;
#20531=CARTESIAN_POINT ( 'NONE',  ( -5.000000000000003553, -8.660254037844383745, -96.99999999999998579 ) ) ;
#20534=CARTESIAN_POINT ( 'NONE',  ( -5.405949406250003975, -9.363379034771801557, -81.34375000204838102 ) ) ;
#20535=CARTESIAN_POINT ( 'NONE',  ( 5.405949406249992428, -9.363379034771808662, -64.59375000204836681 ) ) ;
#20537=CARTESIAN_POINT ( 'NONE',  ( 7.644554776091147741E-16, 12.48450537969573659, -44.65625000204836681 ) ) ;
#20541=CARTESIAN_POINT ( 'NONE',  ( 4.999999999999992006, -8.660254037844389075, -132.7499999999999716 ) ) ;
#20542=CARTESIAN_POINT ( 'NONE',  ( 5.405949406249999534, 9.363379034771803333, -131.7812500020483810 ) ) ;
#20543=( BOUNDED_CURVE ( )  B_SPLINE_CURVE ( 2, ( #22906, #19646, #6497, #33264, #25928, #39710, #35649 ),
 .UNSPECIFIED., .F., .F. ) 
 B_SPLINE_CURVE_WITH_KNOTS ( ( 3, 2, 2, 3 ),
 ( 0.4216417910447762818, 0.4228855721393036671, 0.4241293532338309413, 0.4253731343283583266 ),
 .UNSPECIFIED. ) 
 CURVE ( )  GEOMETRIC_REPRESENTATION_ITEM ( )  RATIONAL_B_SPLINE_CURVE ( ( 0.9999999999999820144, 0.8660254037844566932, 1.000000000000000000, 0.8660254037844387076, 1.000000000000000000, 0.8660254037844267172, 1.000000000000011990 ) ) 
 REPRESENTATION_ITEM ( '' )  );
#20546=CARTESIAN_POINT ( 'NONE',  ( 10.81189881249999729, 6.242252689847867408, -17.90625000204837036 ) ) ;
#20550=CARTESIAN_POINT ( 'NONE',  ( -2.121150477449813534E-15, -11.54700538379251284, -185.3750000000000000 ) ) ;
#20551=CARTESIAN_POINT ( 'NONE',  ( 5.000000000000000000, 8.660254037844385522, -30.62500000409676559 ) ) ;
#20552=DIRECTION ( 'NONE',  ( -0.000000000000000000, -0.000000000000000000, 1.000000000000000000 ) ) ;
#20554=CARTESIAN_POINT ( 'NONE',  ( -10.00000000000102496, 5.773502691895664007, -76.37499999999992895 ) ) ;
#20555=CARTESIAN_POINT ( 'NONE',  ( 7.644554776091147741E-16, 12.48450537969573659, -157.1562500020484094 ) ) ;
#20556=CARTESIAN_POINT ( 'NONE',  ( 7.644554776091147741E-16, 12.48450537969573659, -134.4687500020483810 ) ) ;
#20557=CARTESIAN_POINT ( 'NONE',  ( -10.00000000000076916, 5.773502691895813221, -103.7500000040967763 ) ) ;
#20558=VECTOR ( 'NONE', #40372, 1000.000000000000000 ) ;
#20559=ORIENTED_EDGE ( 'NONE', *, *, #40135, .T. ) ;
#20561=ORIENTED_EDGE ( 'NONE', *, *, #18009, .F. ) ;
#20562=ORIENTED_EDGE ( 'NONE', *, *, #5190, .T. ) ;
#20564=CARTESIAN_POINT ( 'NONE',  ( 10.81189881249999729, 0.000000000000000000, -113.8437500020483810 ) ) ;
#20565=ORIENTED_EDGE ( 'NONE', *, *, #39253, .T. ) ;
#20566=DIRECTION ( 'NONE',  ( -0.000000000000000000, -0.000000000000000000, 1.000000000000000000 ) ) ;
#20567=CARTESIAN_POINT ( 'NONE',  ( 10.81189881249999729, 0.000000000000000000, -188.8437500020483810 ) ) ;
#20568=CARTESIAN_POINT ( 'NONE',  ( -2.293366432827344421E-15, -12.48450537969573659, -36.21875000204835970 ) ) ;
#20569=CARTESIAN_POINT ( 'NONE',  ( -4.888400856004290418, -8.992219867142372536, 2.111525036386560869E-16 ) ) ;
#20571=CARTESIAN_POINT ( 'NONE',  ( 7.644554776091147741E-16, 12.48450537969573659, -177.9687500020484094 ) ) ;
#20572=CARTESIAN_POINT ( 'NONE',  ( -10.81189881249999729, 6.242252689847871849, -159.7187500020483526 ) ) ;
#20574=( BOUNDED_CURVE ( )  B_SPLINE_CURVE ( 2, ( #37452, #14980, #4225, #17366, #24514, #27530, #37667 ),
 .UNSPECIFIED., .F., .F. ) 
 B_SPLINE_CURVE_WITH_KNOTS ( ( 3, 2, 2, 3 ),
 ( 0.5858208955223881409, 0.5870646766169155262, 0.5883084577114429115, 0.5895522388059702967 ),
 .UNSPECIFIED. ) 
 CURVE ( )  GEOMETRIC_REPRESENTATION_ITEM ( )  RATIONAL_B_SPLINE_CURVE ( ( 0.9999999999999880096, 0.8660254037844506980, 1.000000000000000000, 0.8660254037844387076, 1.000000000000000000, 0.8660254037844267172, 1.000000000000011990 ) ) 
 REPRESENTATION_ITEM ( '' )  );
#20577=CARTESIAN_POINT ( 'NONE',  ( 9.999999999999998224, 0.000000000000000000, -36.49999999999997868 ) ) ;
#20579=CARTESIAN_POINT ( 'NONE',  ( -10.81189881249999729, 1.324075727343319199E-15, -90.59375000204838102 ) ) ;
#20581=CARTESIAN_POINT ( 'NONE',  ( 7.644554776091147741E-16, 12.48450537969573659, -64.15625000204838102 ) ) ;
#20583=ADVANCED_FACE ( 'NONE', ( #42382 ), #38950, .T. ) ;
#20585=CARTESIAN_POINT ( 'NONE',  ( 5.405949406249999534, 9.363379034771803333, -122.7812500020483952 ) ) ;
#20587=CARTESIAN_POINT ( 'NONE',  ( -10.81189881249999729, 6.242252689847871849, -152.4062500020483810 ) ) ;
#20589=CARTESIAN_POINT ( 'NONE',  ( -4.999999999999996447, 8.660254037844387298, -126.3750000040967905 ) ) ;
#20591=ORIENTED_EDGE ( 'NONE', *, *, #1854, .T. ) ;
#20596=CARTESIAN_POINT ( 'NONE',  ( -10.81189881249999907, -6.242252689847864744, -191.1562500020484094 ) ) ;
#20598=ORIENTED_EDGE ( 'NONE', *, *, #19755, .T. ) ;
#20599=CARTESIAN_POINT ( 'NONE',  ( 10.00000000000000000, 5.773502691896255534, -48.37499999999997158 ) ) ;
#20601=CARTESIAN_POINT ( 'NONE',  ( 5.000000000000000000, 8.660254037844385522, -68.12500000409677625 ) ) ;
#20602=CARTESIAN_POINT ( 'NONE',  ( -10.00000000000019362, -5.773502691896140959, -179.6250000000000568 ) ) ;
#20603=CARTESIAN_POINT ( 'NONE',  ( -9.999999999999998224, 1.224646799147353059E-15, -166.2500000000000000 ) ) ;
#20605=CARTESIAN_POINT ( 'NONE',  ( -2.293366432827344421E-15, -12.48450537969573659, -60.40625000204838813 ) ) ;
#20609=FACE_OUTER_BOUND ( 'NONE', #17958, .T. ) ;
#20610=CARTESIAN_POINT ( 'NONE',  ( 10.81189881249999551, -6.242252689847874514, -175.6562500020484094 ) ) ;
#20612=CARTESIAN_POINT ( 'NONE',  ( 7.070501591499376803E-16, 11.54700538379251284, -147.5000000040967905 ) ) ;
#20614=DIRECTION ( 'NONE',  ( -0.000000000000000000, -0.000000000000000000, 1.000000000000000000 ) ) ;
#20615=DIRECTION ( 'NONE',  ( -0.000000000000000000, -0.000000000000000000, 1.000000000000000000 ) ) ;
#20616=CARTESIAN_POINT ( 'NONE',  ( 5.405949406249992428, -9.363379034771808662, -87.28125000204838102 ) ) ;
#20618=CARTESIAN_POINT ( 'NONE',  ( -9.999999999999998224, 1.224646799147353059E-15, -91.62500000409677625 ) ) ;
#20619=ORIENTED_EDGE ( 'NONE', *, *, #33818, .T. ) ;
#20620=ORIENTED_EDGE ( 'NONE', *, *, #24095, .F. ) ;
#20621=CARTESIAN_POINT ( 'NONE',  ( -5.405949406249996869, 9.363379034771805109, -23.34375000204835970 ) ) ;
#20622=CARTESIAN_POINT ( 'NONE',  ( -5.405949406249996869, 9.363379034771805109, -16.03125000204835970 ) ) ;
#20625=CARTESIAN_POINT ( 'NONE',  ( -5.405949406249996869, 9.363379034771805109, -68.34375000204836681 ) ) ;
#20626=CARTESIAN_POINT ( 'NONE',  ( -4.999999999999996447, 8.660254037844387298, -92.99999999999998579 ) ) ;
#20628=CARTESIAN_POINT ( 'NONE',  ( 5.405949406249992428, -9.363379034771808662, -189.0937500020483810 ) ) ;
#20631=CARTESIAN_POINT ( 'NONE',  ( -9.999999999999998224, 1.224646799147353059E-15, -200.0000000000000000 ) ) ;
#20632=AXIS2_PLACEMENT_3D ( 'NONE', #28801, #42146, #22102 ) ;
#20633=CARTESIAN_POINT ( 'NONE',  ( -4.999999999999996447, 8.660254037844387298, -70.87500000409677625 ) ) ;
#20634=CARTESIAN_POINT ( 'NONE',  ( -4.999999999999996447, 8.660254037844387298, 1.124999995903236405 ) ) ;
#20635=CARTESIAN_POINT ( 'NONE',  ( -2.121150477449813534E-15, -11.54700538379251284, -89.75000000409677625 ) ) ;
#20636=CARTESIAN_POINT ( 'NONE',  ( -5.405949406250003975, -9.363379034771801557, -114.3437500020483810 ) ) ;
#20637=LINE ( 'NONE', #7276, #30091 ) ;
#20638=CARTESIAN_POINT ( 'NONE',  ( -10.81189881249999729, 1.324075727343319199E-15, -89.28125000204838102 ) ) ;
#20639=EDGE_CURVE ( 'NONE', #30470, #10633, #1212, .T. ) ;
#20640=CARTESIAN_POINT ( 'NONE',  ( 5.405949406249992428, -9.363379034771808662, -102.0937500020483810 ) ) ;
#20642=ADVANCED_FACE ( 'NONE', ( #12814 ), #42173, .T. ) ;
#20644=CARTESIAN_POINT ( 'NONE',  ( -5.000000000000003553, -8.660254037844383745, -163.3750000040967905 ) ) ;
#20645=EDGE_CURVE ( 'NONE', #5415, #25371, #26538, .T. ) ;
#20649=CARTESIAN_POINT ( 'NONE',  ( -9.999999999999998224, 1.224646799147353059E-15, -0.1250000040967647053 ) ) ;
#20651=CARTESIAN_POINT ( 'NONE',  ( 9.999999999999998224, 0.000000000000000000, -70.99999999999998579 ) ) ;
#20653=CARTESIAN_POINT ( 'NONE',  ( -10.00000000000000000, -5.773502691896251982, -88.50000000409679046 ) ) ;
#20654=DIRECTION ( 'NONE',  ( -0.4999999999999997224, -0.8660254037844388186, 0.000000000000000000 ) ) ;
#20655=PRODUCT_DEFINITION ( 'UNKNOWN', '', #36620, #42507 ) ;
#20657=CARTESIAN_POINT ( 'NONE',  ( -2.293366432827344421E-15, -12.48450537969573659, -85.90625000204839523 ) ) ;
#20659=LINE ( 'NONE', #1038, #213 ) ;
#20662=CARTESIAN_POINT ( 'NONE',  ( -10.81189881249999729, 6.242252689847871849, -197.4062500020484379 ) ) ;
#20664=CARTESIAN_POINT ( 'NONE',  ( -2.293366432827344421E-15, -12.48450537969573659, -15.21875000204835615 ) ) ;
#20665=CARTESIAN_POINT ( 'NONE',  ( 0.000000000000000000, 0.000000000000000000, -200.0000000000000000 ) ) ;
#20668=CARTESIAN_POINT ( 'NONE',  ( 5.405949406249999534, 9.363379034771803333, -134.7812500020483810 ) ) ;
#20669=EDGE_CURVE ( 'NONE', #24317, #4916, #5624, .T. ) ;
#20670=CARTESIAN_POINT ( 'NONE',  ( 9.999999999999998224, 0.000000000000000000, -192.5000000000000000 ) ) ;
#20672=CARTESIAN_POINT ( 'NONE',  ( -10.81189881249999729, 6.242252689847871849, -108.9062500020483810 ) ) ;
#20674=CARTESIAN_POINT ( 'NONE',  ( -9.999999999999998224, 1.224646799147353059E-15, -48.12500000409677625 ) ) ;
#20675=ORIENTED_EDGE ( 'NONE', *, *, #24808, .F. ) ;
#20676=( BOUNDED_CURVE ( )  B_SPLINE_CURVE ( 2, ( #23583, #29629, #39121, #72, #10184, #36731, #29206 ),
 .UNSPECIFIED., .F., .F. ) 
 B_SPLINE_CURVE_WITH_KNOTS ( ( 3, 2, 2, 3 ),
 ( 0.9067164179104481025, 0.9079601990049754878, 0.9092039800995028731, 0.9104477611940301474 ),
 .UNSPECIFIED. ) 
 CURVE ( )  GEOMETRIC_REPRESENTATION_ITEM ( )  RATIONAL_B_SPLINE_CURVE ( ( 0.9999999999999641398, 0.8660254037844745678, 1.000000000000000000, 0.8660254037844387076, 1.000000000000000000, 0.8660254037844028474, 1.000000000000035971 ) ) 
 REPRESENTATION_ITEM ( '' )  );
#20677=ORIENTED_EDGE ( 'NONE', *, *, #30325, .T. ) ;
#20678=CARTESIAN_POINT ( 'NONE',  ( -10.81189881249999729, 6.242252689847871849, -36.90625000204835970 ) ) ;
#20680=CARTESIAN_POINT ( 'NONE',  ( -2.293366432827344421E-15, -12.48450537969573659, -94.71875000204838102 ) ) ;
#20681=CARTESIAN_POINT ( 'NONE',  ( 9.999999999999998224, 0.000000000000000000, -115.9999999999999858 ) ) ;
#20685=CARTESIAN_POINT ( 'NONE',  ( -10.81189881249999729, 1.324075727343319199E-15, -192.5937500020484094 ) ) ;
#20687=CARTESIAN_POINT ( 'NONE',  ( -10.00000000000076916, 5.773502691895813221, -137.8750000000000000 ) ) ;
#20689=CARTESIAN_POINT ( 'NONE',  ( -10.81189881249999729, 6.242252689847871849, -126.7187500020483810 ) ) ;
#20693=CARTESIAN_POINT ( 'NONE',  ( -5.000000000000003553, -8.660254037844383745, -188.8750000040967905 ) ) ;
#20695=CARTESIAN_POINT ( 'NONE',  ( -10.81189881249999729, 6.242252689847871849, -176.4062500020484094 ) ) ;
#20696=CARTESIAN_POINT ( 'NONE',  ( -9.999999999999804601, 5.773502691896371886, -179.8750000000000000 ) ) ;
#20697=DIRECTION ( 'NONE',  ( -0.000000000000000000, -0.000000000000000000, 1.000000000000000000 ) ) ;
#20699=CARTESIAN_POINT ( 'NONE',  ( -5.405949406250003975, -9.363379034771801557, -49.84375000204838102 ) ) ;
#20700=CARTESIAN_POINT ( 'NONE',  ( 7.644554776091147741E-16, 12.48450537969573659, -38.46875000204835260 ) ) ;
#20702=CARTESIAN_POINT ( 'NONE',  ( 10.81189881249999551, -6.242252689847874514, -13.65625000204836503 ) ) ;
#20704=CARTESIAN_POINT ( 'NONE',  ( 9.999999999999998224, 0.000000000000000000, -27.49999999999996803 ) ) ;
#20706=CARTESIAN_POINT ( 'NONE',  ( 10.00000000000000000, 5.773502691896255534, -94.87499999999998579 ) ) ;
#20708=CARTESIAN_POINT ( 'NONE',  ( 10.00000000000000000, 5.773502691896255534, -113.2500000040967905 ) ) ;
#20712=CARTESIAN_POINT ( 'NONE',  ( -10.81189881249999729, -6.242252689847864744, -104.1562500020483952 ) ) ;
#20713=ORIENTED_EDGE ( 'NONE', *, *, #8063, .F. ) ;
#20717=ORIENTED_EDGE ( 'NONE', *, *, #10069, .T. ) ;
#20718=CARTESIAN_POINT ( 'NONE',  ( 4.999999999999992006, -8.660254037844389075, -35.24999999999997868 ) ) ;
#20719=EDGE_CURVE ( 'NONE', #26093, #14015, #30956, .T. ) ;
#20720=CARTESIAN_POINT ( 'NONE',  ( 10.81189881249999729, 6.242252689847867408, -32.90625000204835970 ) ) ;
#20721=CARTESIAN_POINT ( 'NONE',  ( 9.999999999999996447, -5.773502691896262640, -158.1250000000000284 ) ) ;
#20722=CARTESIAN_POINT ( 'NONE',  ( -10.00000000000102496, 5.773502691895664007, -34.75000000409671941 ) ) ;
#20724=( BOUNDED_CURVE ( )  B_SPLINE_CURVE ( 2, ( #18790, #17924, #31121, #5429, #2196, #31552, #27875 ),
 .UNSPECIFIED., .F., .F. ) 
 B_SPLINE_CURVE_WITH_KNOTS ( ( 3, 2, 2, 3 ),
 ( 0.03731343283582092690, 0.03855721393034829136, 0.03980099502487565583, 0.04104477611940302029 ),
 .UNSPECIFIED. ) 
 CURVE ( )  GEOMETRIC_REPRESENTATION_ITEM ( )  RATIONAL_B_SPLINE_CURVE ( ( 0.9999999999999963363, 0.8660254037844424824, 1.000000000000000000, 0.8660254037844387076, 1.000000000000000000, 0.8660254037844349329, 1.000000000000003775 ) ) 
 REPRESENTATION_ITEM ( '' )  );
#20726=CARTESIAN_POINT ( 'NONE',  ( 10.81189881249999551, -6.242252689847874514, -135.1562500020484094 ) ) ;
#20727=VECTOR ( 'NONE', #30563, 1000.000000000000000 ) ;
#20728=CARTESIAN_POINT ( 'NONE',  ( 9.999999999999998224, 0.000000000000000000, -162.8750000040967905 ) ) ;
#20729=EDGE_LOOP ( 'NONE', ( #2892, #27580, #11968, #25064 ) ) ;
#20730=( BOUNDED_CURVE ( )  B_SPLINE_CURVE ( 2, ( #9259, #25260, #22427, #11852, #8638, #21793, #34973 ),
 .UNSPECIFIED., .F., .F. ) 
 B_SPLINE_CURVE_WITH_KNOTS ( ( 3, 2, 2, 3 ),
 ( 0.8432835820895525636, 0.8445273631840799489, 0.8457711442786073341, 0.8470149253731346084 ),
 .UNSPECIFIED. ) 
 CURVE ( )  GEOMETRIC_REPRESENTATION_ITEM ( )  RATIONAL_B_SPLINE_CURVE ( ( 0.9999999999999641398, 0.8660254037844745678, 1.000000000000000000, 0.8660254037844387076, 1.000000000000000000, 0.8660254037844028474, 1.000000000000035971 ) ) 
 REPRESENTATION_ITEM ( '' )  );
#20731=ORIENTED_EDGE ( 'NONE', *, *, #30729, .F. ) ;
#20732=ORIENTED_EDGE ( 'NONE', *, *, #26583, .T. ) ;
#20734=CARTESIAN_POINT ( 'NONE',  ( -9.999999999999998224, 1.224646799147353059E-15, -155.7500000000000000 ) ) ;
#20735=CARTESIAN_POINT ( 'NONE',  ( 7.644554776091147741E-16, 12.48450537969573659, -165.9687500020483810 ) ) ;
#20737=CARTESIAN_POINT ( 'NONE',  ( 10.81189881249999729, 0.000000000000000000, -13.34375000204834905 ) ) ;
#20738=DIRECTION ( 'NONE',  ( -0.000000000000000000, -0.000000000000000000, 1.000000000000000000 ) ) ;
#20739=CARTESIAN_POINT ( 'NONE',  ( -10.81189881249999729, -6.242252689847864744, -150.4687500020484094 ) ) ;
#20740=CARTESIAN_POINT ( 'NONE',  ( 10.81189881249999551, -6.242252689847874514, -134.9687500020483810 ) ) ;
#20741=CARTESIAN_POINT ( 'NONE',  ( -10.81189881249999729, 1.324075727343319199E-15, -110.2812500020483810 ) ) ;
#20745=B_SPLINE_CURVE_WITH_KNOTS ( 'NONE', 3,
 ( #1165, #3973, #27703, #30946, #40841, #34192, #7419, #4820, #21003, #17967, #27270, #31167, #34400, #4610, #30313, #37186, #1379, #40409, #37626, #1597, #24475, #10854, #20569, #14725, #7634, #13870, #33975, #14509, #27917, #17534, #36983, #10433 ),
 .UNSPECIFIED., .F., .F.,
 ( 4, 2, 2, 2, 2, 2, 2, 2, 2, 2, 2, 2, 2, 2, 2, 4 ),
 ( 0.002038875896278021741, 0.004610120927203064864, 0.005895743442665587510, 0.007181365958128110155, 0.008466988473590628464, 0.009752610989053148507, 0.01103823350451566855, 0.01232385601997818859, 0.01360947853544071037, 0.01489510105090322868, 0.01618072356636575046, 0.01746634608182826703, 0.01875196859729078708, 0.02003759111275331059, 0.02132321362821582716, 0.02260883614367834721 ),
 .UNSPECIFIED. ) ;
#20746=CARTESIAN_POINT ( 'NONE',  ( -10.81189881249999729, 6.242252689847871849, -8.218750002048354375 ) ) ;
#20748=CARTESIAN_POINT ( 'NONE',  ( -9.999999999999998224, 1.224646799147353059E-15, -200.0000000000000000 ) ) ;
#20749=CARTESIAN_POINT ( 'NONE',  ( -9.999999999999998224, 1.224646799147353059E-15, -196.6250000040967905 ) ) ;
#20753=CARTESIAN_POINT ( 'NONE',  ( -10.81189881249999729, 1.324075727343319199E-15, -72.59375000204838102 ) ) ;
#20754=CARTESIAN_POINT ( 'NONE',  ( -10.81189881249999907, -6.242252689847864744, -61.96875000204838813 ) ) ;
#20755=CARTESIAN_POINT ( 'NONE',  ( 5.405949406249992428, -9.363379034771808662, -37.78125000204838102 ) ) ;
#20757=DIRECTION ( 'NONE',  ( -0.000000000000000000, -0.000000000000000000, 1.000000000000000000 ) ) ;
#20759=CARTESIAN_POINT ( 'NONE',  ( 7.070501591499377789E-16, 11.54700538379251284, -118.6250000000000142 ) ) ;
#20760=CARTESIAN_POINT ( 'NONE',  ( -10.81189881249999729, -6.242252689847864744, -134.1562500020483810 ) ) ;
#20761=CARTESIAN_POINT ( 'NONE',  ( -9.999999999998969713, -5.773502691896847949, -67.50000000409676204 ) ) ;
#20763=CARTESIAN_POINT ( 'NONE',  ( 5.405949406249992428, -9.363379034771808662, -19.78125000204836326 ) ) ;
#20764=ORIENTED_EDGE ( 'NONE', *, *, #33818, .F. ) ;
#20767=CARTESIAN_POINT ( 'NONE',  ( 9.999999999999998224, 0.000000000000000000, -9.499999999999953815 ) ) ;
#20769=CARTESIAN_POINT ( 'NONE',  ( 9.999999999999996447, -5.773502691896262640, -32.50000000409675494 ) ) ;
#20772=CARTESIAN_POINT ( 'NONE',  ( -9.999999999999998224, 1.224646799147353059E-15, -146.7500000000000000 ) ) ;
#20773=CARTESIAN_POINT ( 'NONE',  ( 7.644554776091147741E-16, 12.48450537969573659, -155.6562500020484094 ) ) ;
#20774=CARTESIAN_POINT ( 'NONE',  ( -5.405949406250003975, -9.363379034771801557, -135.3437500020484094 ) ) ;
#20775=ORIENTED_EDGE ( 'NONE', *, *, #39145, .F. ) ;
#20780=ORIENTED_EDGE ( 'NONE', *, *, #17738, .T. ) ;
#20781=CARTESIAN_POINT ( 'NONE',  ( -2.293366432827344421E-15, -12.48450537969573659, -114.2187500020483668 ) ) ;
#20782=ORIENTED_EDGE ( 'NONE', *, *, #15145, .F. ) ;
#20783=CARTESIAN_POINT ( 'NONE',  ( -9.999999999999998224, 1.224646799147353059E-15, -52.24999999999996447 ) ) ;
#20784=CARTESIAN_POINT ( 'NONE',  ( 5.405949406249992428, -9.363379034771808662, -187.5937500020483810 ) ) ;
#20785=VECTOR ( 'NONE', #25116, 1000.000000000000000 ) ;
#20786=CARTESIAN_POINT ( 'NONE',  ( -10.81189881249999729, 1.324075727343319199E-15, -41.09375000204837391 ) ) ;
#20787=CARTESIAN_POINT ( 'NONE',  ( -2.293366432827344421E-15, -12.48450537969573659, -175.7187500020483810 ) ) ;
#20788=CARTESIAN_POINT ( 'NONE',  ( 5.405949406249992428, -9.363379034771808662, -165.0937500020484094 ) ) ;
#20790=CARTESIAN_POINT ( 'NONE',  ( 10.00000000000102318, -5.773502691895667560, -65.50000000409674783 ) ) ;
#20794=CARTESIAN_POINT ( 'NONE',  ( -10.00000000000154188, 5.773502691895366468, -66.25000000409673362 ) ) ;
#20796=CARTESIAN_POINT ( 'NONE',  ( 10.81189881249999907, 6.242252689847868297, -91.21875000204838102 ) ) ;
#20797=CARTESIAN_POINT ( 'NONE',  ( -9.999999999999998224, 1.224646799147353059E-15, -198.1250000040967905 ) ) ;
#20798=CARTESIAN_POINT ( 'NONE',  ( 5.405949406249992428, -9.363379034771808662, -55.78125000204836681 ) ) ;
#20799=CARTESIAN_POINT ( 'NONE',  ( 5.000000000000000000, 8.660254037844385522, -87.62500000409677625 ) ) ;
#20801=CARTESIAN_POINT ( 'NONE',  ( -10.81189881249999907, -6.242252689847864744, -120.6562500020483810 ) ) ;
#20802=CARTESIAN_POINT ( 'NONE',  ( 7.644554776091147741E-16, 12.48450537969573659, -151.1562500020484094 ) ) ;
#20805=CARTESIAN_POINT ( 'NONE',  ( -10.00000000000000000, -5.773502691896251982, -133.5000000040967905 ) ) ;
#20809=ORIENTED_EDGE ( 'NONE', *, *, #42227, .T. ) ;
#20813=CARTESIAN_POINT ( 'NONE',  ( -5.405949406249996869, 9.363379034771805109, -190.0312500020484094 ) ) ;
#20814=ORIENTED_EDGE ( 'NONE', *, *, #15002, .T. ) ;
#20815=CARTESIAN_POINT ( 'NONE',  ( -9.999999999999998224, 5.773502691896259087, -49.37499999999997868 ) ) ;
#20817=CARTESIAN_POINT ( 'NONE',  ( -9.999999999999998224, 5.773502691896259087, -58.75000000409676915 ) ) ;
#20818=CARTESIAN_POINT ( 'NONE',  ( 9.999999999999998224, 0.000000000000000000, -179.0000000000000000 ) ) ;
#20819=CARTESIAN_POINT ( 'NONE',  ( -5.000000000000003553, -8.660254037844383745, -166.0000000000000000 ) ) ;
#20821=CARTESIAN_POINT ( 'NONE',  ( -10.81189881249999729, 1.324075727343319199E-15, -48.78125000204838813 ) ) ;
#20824=DIRECTION ( 'NONE',  ( -0.000000000000000000, -0.000000000000000000, 1.000000000000000000 ) ) ;
#20825=CARTESIAN_POINT ( 'NONE',  ( -2.293366432827344421E-15, -12.48450537969573659, -177.4062500020483810 ) ) ;
#20830=CARTESIAN_POINT ( 'NONE',  ( 9.999999999999998224, 0.000000000000000000, -70.99999999999998579 ) ) ;
#20832=CARTESIAN_POINT ( 'NONE',  ( -9.999999999999998224, 1.224646799147353059E-15, -195.1250000040967905 ) ) ;
#20833=CARTESIAN_POINT ( 'NONE',  ( -10.81189881249999907, -6.242252689847864744, -83.15625000204836681 ) ) ;
#20834=VERTEX_POINT ( 'NONE', #28087 ) ;
#20835=EDGE_CURVE ( 'NONE', #35094, #38971, #14405, .T. ) ;
#20836=CARTESIAN_POINT ( 'NONE',  ( 9.999999999999998224, 0.000000000000000000, -69.49999999999997158 ) ) ;
#20838=ORIENTED_EDGE ( 'NONE', *, *, #33336, .F. ) ;
#20839=VECTOR ( 'NONE', #23866, 1000.000000000000000 ) ;
#20840=( BOUNDED_CURVE ( )  B_SPLINE_CURVE ( 2, ( #37540, #40759, #11201, #34962, #2156, #27836, #4736 ),
 .UNSPECIFIED., .F., .F. ) 
 B_SPLINE_CURVE_WITH_KNOTS ( ( 3, 2, 2, 3 ),
 ( 0.02611940298507465369, 0.02736318407960201815, 0.02860696517412938261, 0.02985074626865674360 ),
 .UNSPECIFIED. ) 
 CURVE ( )  GEOMETRIC_REPRESENTATION_ITEM ( )  RATIONAL_B_SPLINE_CURVE ( ( 0.9999999999999970024, 0.8660254037844417052, 1.000000000000000000, 0.8660254037844387076, 1.000000000000000000, 0.8660254037844357100, 1.000000000000003109 ) ) 
 REPRESENTATION_ITEM ( '' )  );
#20841=CARTESIAN_POINT ( 'NONE',  ( -5.405949406249996869, 9.363379034771805109, -38.34375000204837391 ) ) ;
#20842=CARTESIAN_POINT ( 'NONE',  ( 10.81189881249999729, 0.000000000000000000, -28.34375000204836326 ) ) ;
#20843=CARTESIAN_POINT ( 'NONE',  ( -10.81189881249999729, 6.242252689847871849, -12.90625000204835970 ) ) ;
#20844=CARTESIAN_POINT ( 'NONE',  ( 10.81189881249999907, 6.242252689847868297, -65.71875000204836681 ) ) ;
#20845=CARTESIAN_POINT ( 'NONE',  ( 9.999999999999998224, 0.000000000000000000, -131.0000000000000000 ) ) ;
#20847=CARTESIAN_POINT ( 'NONE',  ( 10.81189881249999729, 0.000000000000000000, -185.8437500020483810 ) ) ;
#20854=CARTESIAN_POINT ( 'NONE',  ( 5.405949406249999534, 9.363379034771803333, -110.5937500020483810 ) ) ;
#20855=CARTESIAN_POINT ( 'NONE',  ( 5.000000000000000000, 8.660254037844385522, -109.7499999999999858 ) ) ;
#20856=CARTESIAN_POINT ( 'NONE',  ( -10.81189881249999907, -6.242252689847864744, -92.15625000204839523 ) ) ;
#20857=CARTESIAN_POINT ( 'NONE',  ( -2.293366432827344421E-15, -12.48450537969573659, -97.71875000204838102 ) ) ;
#20860=CARTESIAN_POINT ( 'NONE',  ( 7.070501591499377789E-16, 11.54700538379251284, -155.0000000040968189 ) ) ;
#20864=CARTESIAN_POINT ( 'NONE',  ( 5.000000000000000000, 8.660254037844385522, -153.6250000040967905 ) ) ;
#20865=CARTESIAN_POINT ( 'NONE',  ( -9.999999999999998224, 1.224646799147353059E-15, -38.74999999999997868 ) ) ;
#20867=CARTESIAN_POINT ( 'NONE',  ( -9.999999999999998224, 1.224646799147353059E-15, -120.1250000040967905 ) ) ;
#20868=CARTESIAN_POINT ( 'NONE',  ( 9.999999999999996447, -5.773502691896262640, -77.12499999999998579 ) ) ;
#20870=CARTESIAN_POINT ( 'NONE',  ( -4.999999999999996447, 8.660254037844387298, -79.87500000409677625 ) ) ;
#20872=CARTESIAN_POINT ( 'NONE',  ( 10.81189881249999729, 6.242252689847867408, -80.90625000204839523 ) ) ;
#20874=CARTESIAN_POINT ( 'NONE',  ( -5.000000000000003553, -8.660254037844383745, -59.49999999999997158 ) ) ;
#20877=CARTESIAN_POINT ( 'NONE',  ( -10.00000000000000000, -5.773502691896251982, -4.124999999999955591 ) ) ;
#20879=CARTESIAN_POINT ( 'NONE',  ( 5.405949406249999534, 9.363379034771803333, -16.09375000204835260 ) ) ;
#20882=CARTESIAN_POINT ( 'NONE',  ( -5.405949406249996869, 9.363379034771805109, -131.5312500020484094 ) ) ;
#20883=CARTESIAN_POINT ( 'NONE',  ( -2.121150477449813534E-15, -11.54700538379251284, -179.3750000000000284 ) ) ;
#20885=CARTESIAN_POINT ( 'NONE',  ( 10.81189881249999729, 0.000000000000000000, -109.5312500020483810 ) ) ;
#20886=VERTEX_POINT ( 'NONE', #17694 ) ;
#20888=EDGE_CURVE ( 'NONE', #30784, #38354, #18850, .T. ) ;
#20889=ORIENTED_EDGE ( 'NONE', *, *, #6146, .F. ) ;
#20891=ORIENTED_EDGE ( 'NONE', *, *, #24376, .T. ) ;
#20892=CARTESIAN_POINT ( 'NONE',  ( -10.81189881249999907, -6.242252689847864744, -36.65625000204835970 ) ) ;
#20894=CARTESIAN_POINT ( 'NONE',  ( 10.81189881249999907, 6.242252689847868297, -86.71875000204836681 ) ) ;
#20895=DIRECTION ( 'NONE',  ( 0.000000000000000000, 0.000000000000000000, -1.000000000000000000 ) ) ;
#20897=CARTESIAN_POINT ( 'NONE',  ( -9.999999999999998224, 1.224646799147353059E-15, -33.12500000409676915 ) ) ;
#20901=CARTESIAN_POINT ( 'NONE',  ( -5.405949406249996869, 9.363379034771805109, -122.3437500020483952 ) ) ;
#20903=CARTESIAN_POINT ( 'NONE',  ( 10.81189881249999551, -6.242252689847874514, -3.156250002048347270 ) ) ;
#20906=CARTESIAN_POINT ( 'NONE',  ( -5.000000000000003553, -8.660254037844383745, -181.3750000040967905 ) ) ;
#20908=CARTESIAN_POINT ( 'NONE',  ( -10.81189881249999729, -6.242252689847864744, -182.1562500020483810 ) ) ;
#20912=CARTESIAN_POINT ( 'NONE',  ( 5.405949406249999534, 9.363379034771803333, -49.09375000204838102 ) ) ;
#20913=CARTESIAN_POINT ( 'NONE',  ( 5.405949406249999534, 9.363379034771803333, -44.59375000204837391 ) ) ;
#20915=CARTESIAN_POINT ( 'NONE',  ( 10.81189881249999729, 0.000000000000000000, -9.031250002048352599 ) ) ;
#20917=CARTESIAN_POINT ( 'NONE',  ( -10.00000000000051337, 5.773502691895962435, -145.3750000000000000 ) ) ;
#20919=CARTESIAN_POINT ( 'NONE',  ( 5.000000000000000000, 8.660254037844385522, -97.74999999999998579 ) ) ;
#20921=CARTESIAN_POINT ( 'NONE',  ( -10.00000000000000000, -5.773502691896251982, -114.0000000040967905 ) ) ;
#20926=CARTESIAN_POINT ( 'NONE',  ( 10.81189881249999729, 0.000000000000000000, -111.0312500020483810 ) ) ;
#20927=ORIENTED_EDGE ( 'NONE', *, *, #9831, .T. ) ;
#20931=CARTESIAN_POINT ( 'NONE',  ( 10.81189881249999729, 0.000000000000000000, -163.5312500020484094 ) ) ;
#20933=ORIENTED_EDGE ( 'NONE', *, *, #18864, .F. ) ;
#20934=CARTESIAN_POINT ( 'NONE',  ( 7.070501591499377789E-16, 11.54700538379251284, -25.62499999999997513 ) ) ;
#20935=CARTESIAN_POINT ( 'NONE',  ( 5.405949406249999534, 9.363379034771803333, -37.28125000204837391 ) ) ;
#20936=CARTESIAN_POINT ( 'NONE',  ( 10.00000000000000000, 5.773502691896255534, -160.8750000000000000 ) ) ;
#20937=CARTESIAN_POINT ( 'NONE',  ( -2.121150477449813534E-15, -11.54700538379251284, -92.37500000000000000 ) ) ;
#20938=( BOUNDED_CURVE ( )  B_SPLINE_CURVE ( 2, ( #9574, #9787, #29651, #93, #23169, #37610, #33535 ),
 .UNSPECIFIED., .F., .F. ) 
 B_SPLINE_CURVE_WITH_KNOTS ( ( 3, 2, 2, 3 ),
 ( 0.4850746268656717652, 0.4863184079601990950, 0.4875621890547264248, 0.4888059701492538101 ),
 .UNSPECIFIED. ) 
 CURVE ( )  GEOMETRIC_REPRESENTATION_ITEM ( )  RATIONAL_B_SPLINE_CURVE ( ( 0.9999999999999880096, 0.8660254037844506980, 1.000000000000000000, 0.8660254037844387076, 1.000000000000000000, 0.8660254037844327124, 1.000000000000005995 ) ) 
 REPRESENTATION_ITEM ( '' )  );
#20940=DIRECTION ( 'NONE',  ( -0.000000000000000000, -0.000000000000000000, 1.000000000000000000 ) ) ;
#20941=CARTESIAN_POINT ( 'NONE',  ( -10.81189881249999907, -6.242252689847864744, -137.1562500020483810 ) ) ;
#20942=CARTESIAN_POINT ( 'NONE',  ( 3.989097665506361245, 9.623024927554942209, -1.486633740873807397E-14 ) ) ;
#20944=CARTESIAN_POINT ( 'NONE',  ( -9.999999999999998224, 1.224646799147353059E-15, -166.6250000040967905 ) ) ;
#20946=EDGE_CURVE ( 'NONE', #37673, #38469, #11229, .T. ) ;
#20951=CARTESIAN_POINT ( 'NONE',  ( -2.121150477449813534E-15, -11.54700538379251284, -134.3750000000000000 ) ) ;
#20952=CARTESIAN_POINT ( 'NONE',  ( -10.81189881249999729, 1.324075727343319199E-15, -162.5937500020484094 ) ) ;
#20954=CARTESIAN_POINT ( 'NONE',  ( 10.81189881249999551, -6.242252689847874514, -14.96875000204837036 ) ) ;
#20955=CARTESIAN_POINT ( 'NONE',  ( -9.999999999999996447, 5.773502691896259975, -170.8750000000000000 ) ) ;
#20956=CARTESIAN_POINT ( 'NONE',  ( 10.81189881249999729, 6.242252689847867408, -146.7187500020484094 ) ) ;
#20957=CARTESIAN_POINT ( 'NONE',  ( 7.644554776091147741E-16, 12.48450537969573659, -137.4687500020483810 ) ) ;
#20958=CARTESIAN_POINT ( 'NONE',  ( 10.81189881249999907, 6.242252689847868297, -103.4062500020483952 ) ) ;
#20962=CARTESIAN_POINT ( 'NONE',  ( 7.070501591499377789E-16, 11.54700538379251284, -198.5000000040968189 ) ) ;
#20964=ADVANCED_FACE ( 'NONE', ( #22241 ), #8868, .T. ) ;
#20965=CARTESIAN_POINT ( 'NONE',  ( -9.999999999999998224, 1.224646799147353059E-15, -200.0000000000000000 ) ) ;
#20968=CARTESIAN_POINT ( 'NONE',  ( 5.405949406249992428, -9.363379034771808662, -79.59375000204838102 ) ) ;
#20969=CARTESIAN_POINT ( 'NONE',  ( -2.293366432827344421E-15, -12.48450537969573659, -66.21875000204836681 ) ) ;
#20971=CARTESIAN_POINT ( 'NONE',  ( -2.293366432827344421E-15, -12.48450537969573659, -36.40625000204835970 ) ) ;
#20975=CARTESIAN_POINT ( 'NONE',  ( 9.999999999999996447, -5.773502691896262640, -122.1250000000000000 ) ) ;
#20976=CARTESIAN_POINT ( 'NONE',  ( 5.405949406249999534, 9.363379034771803333, -130.2812500020483810 ) ) ;
#20977=CARTESIAN_POINT ( 'NONE',  ( 9.999999999999479527, 5.773502691896553074, -94.87499999999997158 ) ) ;
#20979=CARTESIAN_POINT ( 'NONE',  ( -5.405949406249996869, 9.363379034771805109, -14.53125000204835615 ) ) ;
#20981=( BOUNDED_CURVE ( )  B_SPLINE_CURVE ( 2, ( #17877, #13568, #7335, #10342, #34313, #10767, #23956 ),
 .UNSPECIFIED., .F., .F. ) 
 B_SPLINE_CURVE_WITH_KNOTS ( ( 3, 2, 2, 3 ),
 ( 0.08955223880597024122, 0.09079601990049755711, 0.09203980099502487300, 0.09328358208955218889 ),
 .UNSPECIFIED. ) 
 CURVE ( )  GEOMETRIC_REPRESENTATION_ITEM ( )  RATIONAL_B_SPLINE_CURVE ( ( 0.9999999999999895639, 0.8660254037844491437, 1.000000000000000000, 0.8660254037844387076, 1.000000000000000000, 0.8660254037844447028, 0.9999999999999940048 ) ) 
 REPRESENTATION_ITEM ( '' )  );
#20984=CARTESIAN_POINT ( 'NONE',  ( -9.999999999999998224, 1.224646799147353059E-15, -180.1250000040968189 ) ) ;
#20985=CARTESIAN_POINT ( 'NONE',  ( 7.070501591499377789E-16, 11.54700538379251284, -32.00000000409674783 ) ) ;
#20986=CARTESIAN_POINT ( 'NONE',  ( -4.999999999999996447, 8.660254037844387298, -148.5000000000000000 ) ) ;
#20988=( BOUNDED_CURVE ( )  B_SPLINE_CURVE ( 2, ( #7581, #4992, #33704, #24642, #7803, #17695, #37786 ),
 .UNSPECIFIED., .F., .F. ) 
 B_SPLINE_CURVE_WITH_KNOTS ( ( 3, 2, 2, 3 ),
 ( 0.7126865671641793298, 0.7139303482587067151, 0.7151741293532342114, 0.7164179104477614857 ),
 .UNSPECIFIED. ) 
 CURVE ( )  GEOMETRIC_REPRESENTATION_ITEM ( )  RATIONAL_B_SPLINE_CURVE ( ( 0.9999999999999761302, 0.8660254037844625774, 1.000000000000000000, 0.8660254037844387076, 1.000000000000000000, 0.8660254037844028474, 1.000000000000035971 ) ) 
 REPRESENTATION_ITEM ( '' )  );
#20989=CARTESIAN_POINT ( 'NONE',  ( 4.999999999999992006, -8.660254037844389075, -40.12500000409676915 ) ) ;
#20990=CARTESIAN_POINT ( 'NONE',  ( -10.81189881249999729, 1.324075727343319199E-15, -153.7812500020484094 ) ) ;
#20991=CARTESIAN_POINT ( 'NONE',  ( 10.81189881249999551, -6.242252689847874514, -130.4687500020483810 ) ) ;
#20993=ORIENTED_EDGE ( 'NONE', *, *, #15632, .T. ) ;
#20997=CARTESIAN_POINT ( 'NONE',  ( 10.81189881249999729, 0.000000000000000000, -110.8437500020483810 ) ) ;
#20998=ORIENTED_EDGE ( 'NONE', *, *, #32021, .F. ) ;
#20999=CARTESIAN_POINT ( 'NONE',  ( 9.999999999999998224, 0.000000000000000000, -200.0000000000000000 ) ) ;
#21000=CARTESIAN_POINT ( 'NONE',  ( 10.81189881249999551, -6.242252689847874514, -190.4687500020484094 ) ) ;
#21001=CARTESIAN_POINT ( 'NONE',  ( 5.405949406249992428, -9.363379034771808662, -40.59375000204837391 ) ) ;
#21002=ADVANCED_FACE ( 'NONE', ( #32179 ), #2398, .T. ) ;
#21003=CARTESIAN_POINT ( 'NONE',  ( 3.768369288276942619, -9.903100897459154339, -1.167351363741238987E-15 ) ) ;
#21004=CARTESIAN_POINT ( 'NONE',  ( 9.999999999999998224, 0.000000000000000000, -30.87500000409676559 ) ) ;
#21005=CARTESIAN_POINT ( 'NONE',  ( 5.405949406249999534, 9.363379034771803333, -169.0937500020484094 ) ) ;
#21006=CARTESIAN_POINT ( 'NONE',  ( -10.81189881249999729, 6.242252689847871849, -161.2187500020483526 ) ) ;
#21007=CARTESIAN_POINT ( 'NONE',  ( -9.999999999999998224, 1.224646799147353059E-15, -93.12500000409677625 ) ) ;
#21013=CARTESIAN_POINT ( 'NONE',  ( 10.81189881249999551, -6.242252689847874514, -85.46875000204836681 ) ) ;
#21015=CARTESIAN_POINT ( 'NONE',  ( -2.293366432827344421E-15, -12.48450537969573659, -60.40625000204839523 ) ) ;
#21018=CARTESIAN_POINT ( 'NONE',  ( 5.405949406249999534, 9.363379034771803333, -115.2812500020483952 ) ) ;
#21019=CARTESIAN_POINT ( 'NONE',  ( 10.81189881249999729, 6.242252689847867408, -151.4062500020484094 ) ) ;
#21021=CARTESIAN_POINT ( 'NONE',  ( 9.999999999999996447, -5.773502691896262640, -128.5000000040967905 ) ) ;
#21023=ORIENTED_EDGE ( 'NONE', *, *, #11679, .F. ) ;
#21028=CARTESIAN_POINT ( 'NONE',  ( -10.81189881249999729, 1.324075727343319199E-15, -179.2812500020484094 ) ) ;
#21029=ORIENTED_EDGE ( 'NONE', *, *, #2242, .F. ) ;
#21030=CARTESIAN_POINT ( 'NONE',  ( -2.121150477449813534E-15, -11.54700538379251284, -53.37499999999997868 ) ) ;
#21032=CARTESIAN_POINT ( 'NONE',  ( 5.000000000000000000, 8.660254037844385522, -56.12500000409676204 ) ) ;
#21033=CARTESIAN_POINT ( 'NONE',  ( -5.000000000000003553, -8.660254037844383745, -18.99999999999996092 ) ) ;
#21036=CARTESIAN_POINT ( 'NONE',  ( -10.81189881249999729, -6.242252689847864744, -48.65625000204837391 ) ) ;
#21039=CARTESIAN_POINT ( 'NONE',  ( 10.00000000000051159, -5.773502691895965988, -35.12499999999995026 ) ) ;
#21040=CARTESIAN_POINT ( 'NONE',  ( 5.405949406249999534, 9.363379034771803333, -178.2812500020484094 ) ) ;
#21043=CARTESIAN_POINT ( 'NONE',  ( 7.070501591499376803E-16, 11.54700538379251284, -117.1249999999999858 ) ) ;
#21045=CARTESIAN_POINT ( 'NONE',  ( -5.000000000000003553, -8.660254037844383745, -163.3750000040967905 ) ) ;
#21046=CARTESIAN_POINT ( 'NONE',  ( -2.293366432827344421E-15, -12.48450537969573659, -87.40625000204838102 ) ) ;
#21047=ORIENTED_EDGE ( 'NONE', *, *, #41656, .F. ) ;
#21049=CARTESIAN_POINT ( 'NONE',  ( -10.00000000000051337, 5.773502691895962435, -91.75000000409676204 ) ) ;
#21050=ORIENTED_EDGE ( 'NONE', *, *, #19327, .T. ) ;
#21053=CARTESIAN_POINT ( 'NONE',  ( 5.405949406249999534, 9.363379034771803333, -37.09375000204836681 ) ) ;
#21054=CARTESIAN_POINT ( 'NONE',  ( -10.81189881249999729, 6.242252689847871849, -29.21875000204835615 ) ) ;
#21055=CARTESIAN_POINT ( 'NONE',  ( 10.81189881249999729, 0.000000000000000000, -12.03125000204835438 ) ) ;
#21056=CARTESIAN_POINT ( 'NONE',  ( -10.81189881249999729, 1.324075727343319199E-15, -63.59375000204836681 ) ) ;
#21057=CARTESIAN_POINT ( 'NONE',  ( 5.000000000000000000, 8.660254037844385522, -93.24999999999998579 ) ) ;
#21059=CARTESIAN_POINT ( 'NONE',  ( -5.405949406250003975, -9.363379034771801557, -184.8437500020483810 ) ) ;
#21061=LINE ( 'NONE', #31230, #16455 ) ;
#21065=FACE_OUTER_BOUND ( 'NONE', #6769, .T. ) ;
#21066=CARTESIAN_POINT ( 'NONE',  ( 5.405949406249992428, -9.363379034771808662, -111.0937500020483810 ) ) ;
#21067=FACE_OUTER_BOUND ( 'NONE', #42073, .T. ) ;
#21068=CARTESIAN_POINT ( 'NONE',  ( 10.81189881249999729, 0.000000000000000000, -81.03125000204839523 ) ) ;
#21069=CARTESIAN_POINT ( 'NONE',  ( 5.405949406249992428, -9.363379034771808662, -100.5937500020483810 ) ) ;
#21070=ADVANCED_FACE ( 'NONE', ( #15527 ), #15322, .T. ) ;
#21074=CARTESIAN_POINT ( 'NONE',  ( -2.121150477449813534E-15, -11.54700538379251284, -155.7500000040967620 ) ) ;
#21080=CARTESIAN_POINT ( 'NONE',  ( -9.999999999999998224, 1.224646799147353059E-15, -197.7500000000000000 ) ) ;
#21082=DIRECTION ( 'NONE',  ( -0.000000000000000000, -0.000000000000000000, 1.000000000000000000 ) ) ;
#21083=CARTESIAN_POINT ( 'NONE',  ( 4.999999999999992006, -8.660254037844389075, -69.74999999999997158 ) ) ;
#21085=CARTESIAN_POINT ( 'NONE',  ( -9.999999999999998224, 5.773502691896259087, -84.25000000409677625 ) ) ;
#21088=CARTESIAN_POINT ( 'NONE',  ( 10.81189881249999729, 6.242252689847867408, -74.90625000204836681 ) ) ;
#21092=ORIENTED_EDGE ( 'NONE', *, *, #40401, .F. ) ;
#21093=CARTESIAN_POINT ( 'NONE',  ( 9.999999999999996447, -5.773502691896262640, -5.124999999999960032 ) ) ;
#21095=CARTESIAN_POINT ( 'NONE',  ( 10.81189881249999729, 0.000000000000000000, -16.34375000204835260 ) ) ;
#21096=CARTESIAN_POINT ( 'NONE',  ( 10.00000000000051159, -5.773502691895965988, -94.00000000409677625 ) ) ;
#21098=CARTESIAN_POINT ( 'NONE',  ( -5.405949406249996869, 9.363379034771805109, -130.0312500020484094 ) ) ;
#21100=CARTESIAN_POINT ( 'NONE',  ( -2.121150477449813534E-15, -11.54700538379251284, -182.3750000000000000 ) ) ;
#21101=LINE ( 'NONE', #21316, #37196 ) ;
#21102=CARTESIAN_POINT ( 'NONE',  ( -10.81189881249999907, -6.242252689847864744, -107.1562500020483952 ) ) ;
#21103=ORIENTED_EDGE ( 'NONE', *, *, #23720, .F. ) ;
#21104=LINE ( 'NONE', #17856, #8331 ) ;
#21106=VERTEX_POINT ( 'NONE', #2608 ) ;
#21107=CARTESIAN_POINT ( 'NONE',  ( 10.81189881249999729, 0.000000000000000000, -37.53125000204838102 ) ) ;
#21109=CARTESIAN_POINT ( 'NONE',  ( 7.644554776091147741E-16, 12.48450537969573659, -84.96875000204835260 ) ) ;
#21111=CARTESIAN_POINT ( 'NONE',  ( 0.000000000000000000, 0.000000000000000000, -200.0000000000000000 ) ) ;
#21112=CARTESIAN_POINT ( 'NONE',  ( -10.00000000000025580, 5.773502691896109873, -122.8750000000000000 ) ) ;
#21114=DIRECTION ( 'NONE',  ( -0.000000000000000000, -0.000000000000000000, 1.000000000000000000 ) ) ;
#21115=CARTESIAN_POINT ( 'NONE',  ( 5.405949406249999534, 9.363379034771803333, -127.0937500020483668 ) ) ;
#21117=CARTESIAN_POINT ( 'NONE',  ( 10.81189881249999729, 0.000000000000000000, -0.03125000204837191653 ) ) ;
#21120=CARTESIAN_POINT ( 'NONE',  ( -10.00000000000000000, -5.773502691896251982, -178.5000000040967905 ) ) ;
#21122=CARTESIAN_POINT ( 'NONE',  ( -10.81189881249999729, 6.242252689847871849, -174.9062500020484094 ) ) ;
#21123=CARTESIAN_POINT ( 'NONE',  ( -9.999999999999998224, 1.224646799147353059E-15, -109.6250000040967763 ) ) ;
#21124=CARTESIAN_POINT ( 'NONE',  ( -10.00000000000025580, 5.773502691896109873, -121.7500000040967905 ) ) ;
#21126=CARTESIAN_POINT ( 'NONE',  ( -5.405949406250003975, -9.363379034771801557, -48.34375000204838102 ) ) ;
#21128=CARTESIAN_POINT ( 'NONE',  ( 7.644554776091147741E-16, 12.48450537969573659, -13.15625000204836148 ) ) ;
#21130=DIRECTION ( 'NONE',  ( -0.000000000000000000, -0.000000000000000000, 1.000000000000000000 ) ) ;
#21132=ADVANCED_FACE ( 'NONE', ( #19201 ), #16151, .T. ) ;
#21133=CARTESIAN_POINT ( 'NONE',  ( -9.999999999999998224, 5.773502691896259087, -94.37499999999998579 ) ) ;
#21135=CARTESIAN_POINT ( 'NONE',  ( 9.999999999999998224, 0.000000000000000000, -104.3750000040967763 ) ) ;
#21136=CARTESIAN_POINT ( 'NONE',  ( 9.999999999999998224, 0.000000000000000000, -168.5000000000000000 ) ) ;
#21140=CARTESIAN_POINT ( 'NONE',  ( 7.644554776091147741E-16, 12.48450537969573659, -97.15625000204839523 ) ) ;
#21141=ORIENTED_EDGE ( 'NONE', *, *, #33499, .T. ) ;
#21144=CARTESIAN_POINT ( 'NONE',  ( -10.81189881249999907, -6.242252689847864744, -161.1562500020484094 ) ) ;
#21147=CARTESIAN_POINT ( 'NONE',  ( 9.999999999999998224, 0.000000000000000000, -22.99999999999996447 ) ) ;
#21148=CARTESIAN_POINT ( 'NONE',  ( 5.405949406249992428, -9.363379034771808662, -33.28125000204837391 ) ) ;
#21149=CARTESIAN_POINT ( 'NONE',  ( -5.000000000000003553, -8.660254037844383745, -160.0000000000000000 ) ) ;
#21153=CARTESIAN_POINT ( 'NONE',  ( 10.81189881249999907, 6.242252689847868297, -133.4062500020483810 ) ) ;
#21154=CARTESIAN_POINT ( 'NONE',  ( 0.000000000000000000, 0.000000000000000000, -200.0000000000000000 ) ) ;
#21155=CARTESIAN_POINT ( 'NONE',  ( 7.070501591499376803E-16, 11.54700538379251284, -174.5000000040967905 ) ) ;
#21156=ORIENTED_EDGE ( 'NONE', *, *, #16390, .F. ) ;
#21157=CARTESIAN_POINT ( 'NONE',  ( -10.81189881249999907, -6.242252689847864744, -59.15625000204838813 ) ) ;
#21158=VERTEX_POINT ( 'NONE', #32391 ) ;
#21159=ORIENTED_EDGE ( 'NONE', *, *, #40949, .T. ) ;
#21160=CARTESIAN_POINT ( 'NONE',  ( -9.999999999999998224, 1.224646799147353059E-15, -121.2500000000000000 ) ) ;
#21161=FACE_OUTER_BOUND ( 'NONE', #7577, .T. ) ;
#21162=CARTESIAN_POINT ( 'NONE',  ( -5.405949406249996869, 9.363379034771805109, -164.3437500020484094 ) ) ;
#21164=CARTESIAN_POINT ( 'NONE',  ( 10.81189881249999907, 6.242252689847868297, -11.71875000204837214 ) ) ;
#21165=CARTESIAN_POINT ( 'NONE',  ( -11.54700538379251817, 20.00000000000000355, 0.000000000000000000 ) ) ;
#21166=CARTESIAN_POINT ( 'NONE',  ( 5.405949406249999534, 9.363379034771803333, -148.0937500020483810 ) ) ;
#21167=CARTESIAN_POINT ( 'NONE',  ( 5.405949406249999534, 9.363379034771803333, -131.5937500020483810 ) ) ;
#21168=CARTESIAN_POINT ( 'NONE',  ( -10.81189881249999907, -6.242252689847864744, -108.6562500020483952 ) ) ;
#21172=CARTESIAN_POINT ( 'NONE',  ( 10.81189881249999729, 0.000000000000000000, -1.343750002048366143 ) ) ;
#21175=CARTESIAN_POINT ( 'NONE',  ( -9.999999999999998224, 1.224646799147353059E-15, -114.1250000040967763 ) ) ;
#21178=CARTESIAN_POINT ( 'NONE',  ( -5.405949406250003975, -9.363379034771801557, -72.34375000204836681 ) ) ;
#21179=CARTESIAN_POINT ( 'NONE',  ( 5.405949406249992428, -9.363379034771808662, -69.09375000204836681 ) ) ;
#21181=CARTESIAN_POINT ( 'NONE',  ( 5.405949406249999534, 9.363379034771803333, -32.78125000204837391 ) ) ;
#21183=CARTESIAN_POINT ( 'NONE',  ( 9.999999999998969713, 5.773502691896851502, -32.25000000409673362 ) ) ;
#21186=CARTESIAN_POINT ( 'NONE',  ( -5.000000000000003553, -8.660254037844383745, -122.5000000000000000 ) ) ;
#21187=CARTESIAN_POINT ( 'NONE',  ( -5.405949406250003975, -9.363379034771801557, -132.5312500020484094 ) ) ;
#21188=( BOUNDED_CURVE ( )  B_SPLINE_CURVE ( 2, ( #20136, #19496, #33323, #39770, #26198, #22749, #10204 ),
 .UNSPECIFIED., .F., .F. ) 
 B_SPLINE_CURVE_WITH_KNOTS ( ( 3, 2, 2, 3 ),
 ( 0.6753731343283584376, 0.6766169154228858229, 0.6778606965174133192, 0.6791044776119405935 ),
 .UNSPECIFIED. ) 
 CURVE ( )  GEOMETRIC_REPRESENTATION_ITEM ( )  RATIONAL_B_SPLINE_CURVE ( ( 0.9999999999999761302, 0.8660254037844625774, 1.000000000000000000, 0.8660254037844387076, 1.000000000000000000, 0.8660254037844028474, 1.000000000000035971 ) ) 
 REPRESENTATION_ITEM ( '' )  );
#21189=CARTESIAN_POINT ( 'NONE',  ( 9.999999999999998224, 0.000000000000000000, -66.87500000409676204 ) ) ;
#21191=CARTESIAN_POINT ( 'NONE',  ( 7.644554776091147741E-16, 12.48450537969573659, -19.15625000204837391 ) ) ;
#21193=ORIENTED_EDGE ( 'NONE', *, *, #29446, .T. ) ;
#21196=CARTESIAN_POINT ( 'NONE',  ( -5.000000000000003553, -8.660254037844383745, -179.8750000040967905 ) ) ;
#21197=CARTESIAN_POINT ( 'NONE',  ( 4.999999999999992006, -8.660254037844389075, -35.62500000409676915 ) ) ;
#21198=CARTESIAN_POINT ( 'NONE',  ( -9.999999999998969713, -5.773502691896847949, -14.62499999999995026 ) ) ;
#21201=CARTESIAN_POINT ( 'NONE',  ( -2.121150477449813534E-15, -11.54700538379251284, -191.3750000000000284 ) ) ;
#21202=CARTESIAN_POINT ( 'NONE',  ( 7.644554776091147741E-16, 12.48450537969573659, -154.1562500020484094 ) ) ;
#21203=CARTESIAN_POINT ( 'NONE',  ( -5.405949406249996869, 9.363379034771805109, -129.8437500020484094 ) ) ;
#21206=CARTESIAN_POINT ( 'NONE',  ( 9.999999999999998224, 0.000000000000000000, -185.3750000040967905 ) ) ;
#21207=ORIENTED_EDGE ( 'NONE', *, *, #9126, .T. ) ;
#21208=EDGE_CURVE ( 'NONE', #12734, #31643, #1468, .T. ) ;
#21210=VECTOR ( 'NONE', #16320, 1000.000000000000000 ) ;
#21211=ORIENTED_EDGE ( 'NONE', *, *, #382, .T. ) ;
#21212=( BOUNDED_CURVE ( )  B_SPLINE_CURVE ( 2, ( #22818, #7050, #20201, #16947, #584, #27967, #33807 ),
 .UNSPECIFIED., .F., .F. ) 
 B_SPLINE_CURVE_WITH_KNOTS ( ( 3, 2, 2, 3 ),
 ( 0.8656716417910450545, 0.8669154228855724398, 0.8681592039800998251, 0.8694029850746272103 ),
 .UNSPECIFIED. ) 
 CURVE ( )  GEOMETRIC_REPRESENTATION_ITEM ( )  RATIONAL_B_SPLINE_CURVE ( ( 0.9999999999999641398, 0.8660254037844745678, 1.000000000000000000, 0.8660254037844387076, 1.000000000000000000, 0.8660254037844028474, 1.000000000000035971 ) ) 
 REPRESENTATION_ITEM ( '' )  );
#21213=CARTESIAN_POINT ( 'NONE',  ( 10.00000000000051159, -5.773502691895965988, -145.0000000040967620 ) ) ;
#21214=CARTESIAN_POINT ( 'NONE',  ( -5.405949406250003975, -9.363379034771801557, -187.8437500020483810 ) ) ;
#21215=CARTESIAN_POINT ( 'NONE',  ( 10.81189881249999551, -6.242252689847874514, -40.46875000204835260 ) ) ;
#21217=CARTESIAN_POINT ( 'NONE',  ( 0.000000000000000000, 0.000000000000000000, -200.0000000000000000 ) ) ;
#21218=CARTESIAN_POINT ( 'NONE',  ( 10.81189881249999729, 0.000000000000000000, -173.8437500020484094 ) ) ;
#21219=CARTESIAN_POINT ( 'NONE',  ( 7.644554776091147741E-16, 12.48450537969573659, -161.4687500020484094 ) ) ;
#21220=LINE ( 'NONE', #24479, #10042 ) ;
#21224=CARTESIAN_POINT ( 'NONE',  ( -11.54700538379251817, 20.00000000000000355, 45.00000000000009237 ) ) ;
#21226=LINE ( 'NONE', #14519, #3877 ) ;
#21228=CARTESIAN_POINT ( 'NONE',  ( -10.81189881249999729, 1.324075727343319199E-15, -87.59375000204836681 ) ) ;
#21229=CARTESIAN_POINT ( 'NONE',  ( -9.999999999998456346, -5.773502691897145489, -82.50000000409673362 ) ) ;
#21230=CARTESIAN_POINT ( 'NONE',  ( -2.293366432827344421E-15, -12.48450537969573659, -55.90625000204837391 ) ) ;
#21233=CARTESIAN_POINT ( 'NONE',  ( 10.81189881249999729, 0.000000000000000000, -112.5312500020483952 ) ) ;
#21234=CARTESIAN_POINT ( 'NONE',  ( -5.405949406250003975, -9.363379034771801557, -158.0312500020484094 ) ) ;
#21235=DIRECTION ( 'NONE',  ( -0.000000000000000000, -0.000000000000000000, 1.000000000000000000 ) ) ;
#21237=CARTESIAN_POINT ( 'NONE',  ( -9.999999999999998224, 5.773502691896259087, -127.7500000040967905 ) ) ;
#21239=ORIENTED_EDGE ( 'NONE', *, *, #18864, .T. ) ;
#21240=( BOUNDED_CURVE ( )  B_SPLINE_CURVE ( 2, ( #22530, #35703, #15606, #25355, #28808, #32471, #12793 ),
 .UNSPECIFIED., .F., .F. ) 
 B_SPLINE_CURVE_WITH_KNOTS ( ( 3, 2, 2, 3 ),
 ( 0.7313432835820897759, 0.7325870646766171612, 0.7338308457711446575, 0.7350746268656719318 ),
 .UNSPECIFIED. ) 
 CURVE ( )  GEOMETRIC_REPRESENTATION_ITEM ( )  RATIONAL_B_SPLINE_CURVE ( ( 0.9999999999999761302, 0.8660254037844625774, 1.000000000000000000, 0.8660254037844387076, 1.000000000000000000, 0.8660254037844028474, 1.000000000000035971 ) ) 
 REPRESENTATION_ITEM ( '' )  );
#21244=CARTESIAN_POINT ( 'NONE',  ( -10.81189881249999729, 1.324075727343319199E-15, -180.7812500020484094 ) ) ;
#21245=ORIENTED_EDGE ( 'NONE', *, *, #40425, .T. ) ;
#21247=CARTESIAN_POINT ( 'NONE',  ( -9.999999999999998224, 1.224646799147353059E-15, -60.12500000409676204 ) ) ;
#21248=CARTESIAN_POINT ( 'NONE',  ( 9.999999999999998224, 0.000000000000000000, -18.49999999999996092 ) ) ;
#21249=CARTESIAN_POINT ( 'NONE',  ( 7.070501591499376803E-16, 11.54700538379251284, -135.5000000040967905 ) ) ;
#21251=CARTESIAN_POINT ( 'NONE',  ( 5.405949406249992428, -9.363379034771808662, -49.78125000204838813 ) ) ;
#21254=LINE ( 'NONE', #34442, #20727 ) ;
#21255=CARTESIAN_POINT ( 'NONE',  ( 10.81189881249999551, -6.242252689847874514, -178.6562500020484094 ) ) ;
#21256=EDGE_CURVE ( 'NONE', #7028, #318, #29143, .T. ) ;
#21257=CARTESIAN_POINT ( 'NONE',  ( -9.999999999999998224, 1.224646799147353059E-15, -159.1250000040967905 ) ) ;
#21260=ORIENTED_EDGE ( 'NONE', *, *, #42062, .F. ) ;
#21261=CARTESIAN_POINT ( 'NONE',  ( -4.999999999999996447, 8.660254037844387298, -117.0000000000000000 ) ) ;
#21262=CARTESIAN_POINT ( 'NONE',  ( 9.999999999999998224, 0.000000000000000000, -59.37500000409676204 ) ) ;
#21264=CARTESIAN_POINT ( 'NONE',  ( -10.81189881249999729, 1.324075727343319199E-15, -86.28125000204838102 ) ) ;
#21266=CARTESIAN_POINT ( 'NONE',  ( -23.09401076758503280, 0.000000000000000000, 49.99999999999998579 ) ) ;
#21267=VERTEX_POINT ( 'NONE', #38426 ) ;
#21268=EDGE_LOOP ( 'NONE', ( #31542, #16069, #4337, #38987 ) ) ;
#21269=CARTESIAN_POINT ( 'NONE',  ( -10.81189881249999729, 6.242252689847871849, -41.21875000204834549 ) ) ;
#21270=CARTESIAN_POINT ( 'NONE',  ( 10.81189881249999551, -6.242252689847874514, -23.96875000204836681 ) ) ;
#21271=CARTESIAN_POINT ( 'NONE',  ( 5.405949406249992428, -9.363379034771808662, -10.78125000204835438 ) ) ;
#21272=CARTESIAN_POINT ( 'NONE',  ( 7.644554776091147741E-16, 12.48450537969573659, -63.96875000204837391 ) ) ;
#21273=ORIENTED_EDGE ( 'NONE', *, *, #27256, .T. ) ;
#21274=DIRECTION ( 'NONE',  ( 1.000000000000000000, 0.000000000000000000, 0.000000000000000000 ) ) ;
#21277=CARTESIAN_POINT ( 'NONE',  ( 10.81189881249999551, -6.242252689847874514, -188.9687500020484094 ) ) ;
#21279=CARTESIAN_POINT ( 'NONE',  ( 9.999999999999998224, 0.000000000000000000, -59.37500000409676204 ) ) ;
#21282=CARTESIAN_POINT ( 'NONE',  ( -9.999999999999998224, 1.224646799147353059E-15, -60.12500000409676204 ) ) ;
#21283=CARTESIAN_POINT ( 'NONE',  ( 10.81189881249999907, 6.242252689847868297, -113.7187500020483810 ) ) ;
#21285=CARTESIAN_POINT ( 'NONE',  ( 5.405949406249999534, 9.363379034771803333, -85.28125000204838102 ) ) ;
#21286=CARTESIAN_POINT ( 'NONE',  ( -10.81189881249999729, 1.324075727343319199E-15, -104.0937500020483810 ) ) ;
#21289=CARTESIAN_POINT ( 'NONE',  ( 5.000000000000000000, 8.660254037844385522, -153.6250000040967905 ) ) ;
#21293=CARTESIAN_POINT ( 'NONE',  ( 4.999999999999992006, -8.660254037844389075, -174.7500000000000284 ) ) ;
#21294=DIRECTION ( 'NONE',  ( -0.000000000000000000, -0.000000000000000000, 1.000000000000000000 ) ) ;
#21296=CARTESIAN_POINT ( 'NONE',  ( 7.070501591499376803E-16, 11.54700538379251284, -120.5000000040967905 ) ) ;
#21297=CARTESIAN_POINT ( 'NONE',  ( 5.000000000000000000, 8.660254037844385522, -75.24999999999998579 ) ) ;
#21299=CARTESIAN_POINT ( 'NONE',  ( 10.00000000000000000, 5.773502691896255534, -83.25000000409677625 ) ) ;
#21302=CARTESIAN_POINT ( 'NONE',  ( 10.81189881249999729, 0.000000000000000000, -78.03125000204838102 ) ) ;
#21304=CARTESIAN_POINT ( 'NONE',  ( -2.121150477449813534E-15, -11.54700538379251284, -59.37500000000001421 ) ) ;
#21307=CARTESIAN_POINT ( 'NONE',  ( 4.999999999999992006, -8.660254037844389075, -5.249999999999976907 ) ) ;
#21309=CARTESIAN_POINT ( 'NONE',  ( 10.81189881249999551, -6.242252689847874514, -14.96875000204837214 ) ) ;
#21310=CARTESIAN_POINT ( 'NONE',  ( -9.999999999999998224, 1.224646799147353059E-15, -149.7500000000000000 ) ) ;
#21311=( BOUNDED_CURVE ( )  B_SPLINE_CURVE ( 2, ( #10227, #3561, #19944, #23414, #22775, #36563, #16479 ),
 .UNSPECIFIED., .F., .F. ) 
 B_SPLINE_CURVE_WITH_KNOTS ( ( 3, 2, 2, 3 ),
 ( 0.02238805970149256030, 0.02363184079601992477, 0.02487562189054729270, 0.02611940298507465369 ),
 .UNSPECIFIED. ) 
 CURVE ( )  GEOMETRIC_REPRESENTATION_ITEM ( )  RATIONAL_B_SPLINE_CURVE ( ( 0.9999999999999973355, 0.8660254037844413721, 1.000000000000000000, 0.8660254037844387076, 1.000000000000000000, 0.8660254037844357100, 1.000000000000003109 ) ) 
 REPRESENTATION_ITEM ( '' )  );
#21314=CARTESIAN_POINT ( 'NONE',  ( -10.81189881249999729, 6.242252689847871849, -128.4062500020484094 ) ) ;
#21315=CARTESIAN_POINT ( 'NONE',  ( 9.999999999999998224, 0.000000000000000000, -183.5000000000000000 ) ) ;
#21316=CARTESIAN_POINT ( 'NONE',  ( -9.999999999999998224, 1.224646799147353059E-15, -200.0000000000000000 ) ) ;
#21317=CARTESIAN_POINT ( 'NONE',  ( -2.293366432827344421E-15, -12.48450537969573659, -108.4062500020483810 ) ) ;
#21320=VERTEX_POINT ( 'NONE', #12705 ) ;
#21321=ADVANCED_FACE ( 'NONE', ( #25902 ), #39054, .T. ) ;
#21323=CARTESIAN_POINT ( 'NONE',  ( 10.81189881249999551, -6.242252689847874514, -36.15625000204835970 ) ) ;
#21325=CARTESIAN_POINT ( 'NONE',  ( -5.405949406249996869, 9.363379034771805109, -89.34375000204838102 ) ) ;
#21326=FACE_OUTER_BOUND ( 'NONE', #15364, .T. ) ;
#21330=DIRECTION ( 'NONE',  ( -0.5000000000000008882, 0.8660254037844382635, 0.000000000000000000 ) ) ;
#21331=CARTESIAN_POINT ( 'NONE',  ( 10.81189881249999551, -6.242252689847874514, -121.4687500020484237 ) ) ;
#21333=CARTESIAN_POINT ( 'NONE',  ( -5.405949406250003975, -9.363379034771801557, -0.5312500020483723606 ) ) ;
#21336=CARTESIAN_POINT ( 'NONE',  ( 10.00000000000000000, 5.773502691896255534, -176.2500000040968189 ) ) ;
#21337=CARTESIAN_POINT ( 'NONE',  ( -2.293366432827344421E-15, -12.48450537969573659, -169.9062500020484379 ) ) ;
#21338=DIRECTION ( 'NONE',  ( -0.000000000000000000, -0.000000000000000000, 1.000000000000000000 ) ) ;
#21341=CARTESIAN_POINT ( 'NONE',  ( -10.81189881249999729, 1.324075727343319199E-15, -56.09375000204835970 ) ) ;
#21343=EDGE_CURVE ( 'NONE', #12803, #17345, #5880, .T. ) ;
#21345=CARTESIAN_POINT ( 'NONE',  ( -10.81189881249999729, 6.242252689847871849, -9.906250002048379244 ) ) ;
#21349=CARTESIAN_POINT ( 'NONE',  ( -10.00000000000000000, -5.773502691896251982, -100.1249999999999858 ) ) ;
#21351=CARTESIAN_POINT ( 'NONE',  ( 9.999999999999996447, -5.773502691896262640, -104.5000000040967763 ) ) ;
#21352=CARTESIAN_POINT ( 'NONE',  ( -9.999999999999998224, 1.224646799147353059E-15, -115.2499999999999858 ) ) ;
#21355=CARTESIAN_POINT ( 'NONE',  ( 10.81189881249999551, -6.242252689847874514, -96.15625000204838102 ) ) ;
#21358=ADVANCED_FACE ( 'NONE', ( #23726 ), #19618, .T. ) ;
#21360=CARTESIAN_POINT ( 'NONE',  ( -9.999999999999998224, 1.224646799147353059E-15, -139.6250000040967905 ) ) ;
#21361=CARTESIAN_POINT ( 'NONE',  ( -10.81189881249999907, -6.242252689847864744, -162.6562500020483810 ) ) ;
#21363=ORIENTED_EDGE ( 'NONE', *, *, #11142, .T. ) ;
#21364=CARTESIAN_POINT ( 'NONE',  ( -2.121150477449813534E-15, -11.54700538379251284, -21.87499999999997513 ) ) ;
#21365=CARTESIAN_POINT ( 'NONE',  ( -10.81189881249999729, -6.242252689847864744, -27.65625000204838102 ) ) ;
#21366=CARTESIAN_POINT ( 'NONE',  ( 7.070501591499377789E-16, 11.54700538379251284, -157.6250000000000000 ) ) ;
#21367=DIRECTION ( 'NONE',  ( 1.000000000000000000, 0.000000000000000000, 0.000000000000000000 ) ) ;
#21370=CARTESIAN_POINT ( 'NONE',  ( -5.405949406249996869, 9.363379034771805109, -134.5312500020484094 ) ) ;
#21371=CARTESIAN_POINT ( 'NONE',  ( 5.504483976897049047, 8.886403137384359496, -8.678191841965556968E-15 ) ) ;
#21372=ORIENTED_EDGE ( 'NONE', *, *, #32223, .T. ) ;
#21373=CARTESIAN_POINT ( 'NONE',  ( 5.405949406249999534, 9.363379034771803333, -62.78125000204837391 ) ) ;
#21375=VECTOR ( 'NONE', #1267, 1000.000000000000000 ) ;
#21376=EDGE_CURVE ( 'NONE', #23028, #33859, #6129, .T. ) ;
#21377=ORIENTED_EDGE ( 'NONE', *, *, #19093, .F. ) ;
#21378=ORIENTED_EDGE ( 'NONE', *, *, #11028, .F. ) ;
#21380=CARTESIAN_POINT ( 'NONE',  ( -7.071067811865477282, -7.071067811865471064, -200.0000000000000000 ) ) ;
#21381=CARTESIAN_POINT ( 'NONE',  ( 10.81189881249999551, -6.242252689847874514, -160.4687500020484094 ) ) ;
#21383=CARTESIAN_POINT ( 'NONE',  ( -10.81189881249999729, 6.242252689847871849, -14.21875000204836681 ) ) ;
#21385=CARTESIAN_POINT ( 'NONE',  ( -10.81189881249999729, 6.242252689847871849, -150.7187500020483810 ) ) ;
#21386=CARTESIAN_POINT ( 'NONE',  ( -5.405949406249996869, 9.363379034771805109, -106.0312500020483810 ) ) ;
#21388=DIRECTION ( 'NONE',  ( 1.000000000000000000, 0.000000000000000000, 0.000000000000000000 ) ) ;
#21390=CARTESIAN_POINT ( 'NONE',  ( -2.293366432827344421E-15, -12.48450537969573659, -6.218750002048345493 ) ) ;
#21392=CARTESIAN_POINT ( 'NONE',  ( 7.644554776091147741E-16, 12.48450537969573659, -191.6562500020484094 ) ) ;
#21393=DIRECTION ( 'NONE',  ( -0.000000000000000000, -0.000000000000000000, 1.000000000000000000 ) ) ;
#21396=CARTESIAN_POINT ( 'NONE',  ( 7.644554776091147741E-16, 12.48450537969573659, -75.96875000204838102 ) ) ;
#21397=CARTESIAN_POINT ( 'NONE',  ( 10.81189881249999907, 6.242252689847868297, -55.21875000204836681 ) ) ;
#21399=CARTESIAN_POINT ( 'NONE',  ( -2.293366432827344421E-15, -12.48450537969573659, -34.90625000204836681 ) ) ;
#21402=CARTESIAN_POINT ( 'NONE',  ( -4.999999999999996447, 8.660254037844387298, -121.5000000000000000 ) ) ;
#21405=CARTESIAN_POINT ( 'NONE',  ( 5.405949406249999534, 9.363379034771803333, -7.281250002048378356 ) ) ;
#21406=VERTEX_POINT ( 'NONE', #36666 ) ;
#21409=CARTESIAN_POINT ( 'NONE',  ( -10.00000000000025757, -5.773502691896102768, -180.0000000040968189 ) ) ;
#21411=AXIS2_PLACEMENT_3D ( 'NONE', #34932, #38573, #5996 ) ;
#21412=CARTESIAN_POINT ( 'NONE',  ( -9.999999999999998224, 5.773502691896259087, -31.75000000409675138 ) ) ;
#21414=CARTESIAN_POINT ( 'NONE',  ( -9.999999999999998224, 1.224646799147353059E-15, -3.125000004096767370 ) ) ;
#21417=CARTESIAN_POINT ( 'NONE',  ( -5.405949406250003975, -9.363379034771801557, -141.5312500020483810 ) ) ;
#21418=CARTESIAN_POINT ( 'NONE',  ( -10.81189881249999729, 6.242252689847871849, -123.7187500020483952 ) ) ;
#21419=CARTESIAN_POINT ( 'NONE',  ( 9.999999999999479527, 5.773502691896553074, -144.3750000000000000 ) ) ;
#21421=ORIENTED_EDGE ( 'NONE', *, *, #14872, .F. ) ;
#21422=EDGE_CURVE ( 'NONE', #19092, #40867, #10517, .T. ) ;
#21423=ORIENTED_EDGE ( 'NONE', *, *, #33597, .T. ) ;
#21426=EDGE_CURVE ( 'NONE', #23854, #11337, #10264, .T. ) ;
#21427=LINE ( 'NONE', #1376, #23774 ) ;
#21428=CARTESIAN_POINT ( 'NONE',  ( -10.81189881249999907, -6.242252689847864744, -180.4687500020484094 ) ) ;
#21430=CARTESIAN_POINT ( 'NONE',  ( -5.405949406250003975, -9.363379034771801557, -36.34375000204836681 ) ) ;
#21431=CARTESIAN_POINT ( 'NONE',  ( -5.000000000000003553, -8.660254037844383745, -41.49999999999997868 ) ) ;
#21432=CARTESIAN_POINT ( 'NONE',  ( -10.81189881249999729, -6.242252689847864744, -171.4687500020483526 ) ) ;
#21433=CARTESIAN_POINT ( 'NONE',  ( 5.405949406249992428, -9.363379034771808662, -156.0937500020483810 ) ) ;
#21434=CARTESIAN_POINT ( 'NONE',  ( 0.000000000000000000, 0.000000000000000000, -200.0000000000000000 ) ) ;
#21438=CARTESIAN_POINT ( 'NONE',  ( 10.00000000000025402, -5.773502691896113426, -155.1250000000000000 ) ) ;
#21439=CARTESIAN_POINT ( 'NONE',  ( 5.000000000000000000, 8.660254037844385522, -11.12500000409674605 ) ) ;
#21441=CARTESIAN_POINT ( 'NONE',  ( 7.644554776091147741E-16, 12.48450537969573659, -80.46875000204838102 ) ) ;
#21442=FACE_OUTER_BOUND ( 'NONE', #37406, .T. ) ;
#21443=CARTESIAN_POINT ( 'NONE',  ( -5.405949406250003975, -9.363379034771801557, -56.03125000204836681 ) ) ;
#21446=EDGE_CURVE ( 'NONE', #4273, #40023, #14674, .T. ) ;
#21447=CARTESIAN_POINT ( 'NONE',  ( 5.405949406249999534, 9.363379034771803333, -116.7812500020483952 ) ) ;
#21448=CARTESIAN_POINT ( 'NONE',  ( -2.293366432827344421E-15, -12.48450537969573659, -157.9062500020483810 ) ) ;
#21449=CARTESIAN_POINT ( 'NONE',  ( 10.00000000000102318, -5.773502691895667560, -11.12499999999993072 ) ) ;
#21451=CARTESIAN_POINT ( 'NONE',  ( 9.999999999999996447, -5.773502691896262640, -127.0000000040967763 ) ) ;
#21457=CARTESIAN_POINT ( 'NONE',  ( 10.81189881249999907, 6.242252689847868297, -184.4062500020484094 ) ) ;
#21458=VERTEX_POINT ( 'NONE', #30211 ) ;
#21460=CARTESIAN_POINT ( 'NONE',  ( 4.999999999999992006, -8.660254037844389075, -59.62500000409676204 ) ) ;
#21464=CARTESIAN_POINT ( 'NONE',  ( -10.81189881249999729, -6.242252689847864744, -51.65625000204838102 ) ) ;
#21465=VECTOR ( 'NONE', #12376, 1000.000000000000000 ) ;
#21468=CARTESIAN_POINT ( 'NONE',  ( -9.999999999999998224, 1.224646799147353059E-15, -9.125000004096744277 ) ) ;
#21469=CARTESIAN_POINT ( 'NONE',  ( 7.644554776091147741E-16, 12.48450537969573659, -181.1562500020484094 ) ) ;
#21472=CARTESIAN_POINT ( 'NONE',  ( 9.999999999999998224, 0.000000000000000000, -137.0000000000000000 ) ) ;
#21473=ORIENTED_EDGE ( 'NONE', *, *, #20639, .T. ) ;
#21475=CARTESIAN_POINT ( 'NONE',  ( -9.999999999999998224, 1.224646799147353059E-15, -105.1250000040967763 ) ) ;
#21477=CARTESIAN_POINT ( 'NONE',  ( 7.070501591499376803E-16, 11.54700538379251284, -195.5000000040968189 ) ) ;
#21478=AXIS2_PLACEMENT_3D ( 'NONE', #19670, #9541, #30257 ) ;
#21479=CARTESIAN_POINT ( 'NONE',  ( 5.405949406249992428, -9.363379034771808662, -75.28125000204838102 ) ) ;
#21481=CARTESIAN_POINT ( 'NONE',  ( 0.000000000000000000, 0.000000000000000000, -200.0000000000000000 ) ) ;
#21482=CARTESIAN_POINT ( 'NONE',  ( -7.423074889580956182, -12.85714285714295890, 52.14285714285716011 ) ) ;
#21483=ORIENTED_EDGE ( 'NONE', *, *, #11704, .T. ) ;
#21484=VERTEX_POINT ( 'NONE', #19830 ) ;
#21485=EDGE_CURVE ( 'NONE', #38772, #25832, #13557, .T. ) ;
#21486=CARTESIAN_POINT ( 'NONE',  ( 10.81189881249999551, -6.242252689847874514, -38.96875000204835970 ) ) ;
#21488=CARTESIAN_POINT ( 'NONE',  ( 5.000000000000000000, 8.660254037844385522, -74.12500000409677625 ) ) ;
#21489=CARTESIAN_POINT ( 'NONE',  ( 10.81189881249999907, 6.242252689847868297, -17.90625000204837036 ) ) ;
#21490=CARTESIAN_POINT ( 'NONE',  ( -5.405949406250003975, -9.363379034771801557, -60.34375000204835970 ) ) ;
#21491=ORIENTED_EDGE ( 'NONE', *, *, #25736, .T. ) ;
#21492=EDGE_CURVE ( 'NONE', #31836, #3056, #14927, .T. ) ;
#21495=CARTESIAN_POINT ( 'NONE',  ( 10.81189881249999729, 6.242252689847867408, -193.2187500020484094 ) ) ;
#21496=CARTESIAN_POINT ( 'NONE',  ( -10.81189881249999729, 6.242252689847871849, -179.2187500020483810 ) ) ;
#21500=CARTESIAN_POINT ( 'NONE',  ( 10.00000000000015632, -5.773502691896169381, -192.6250000000000568 ) ) ;
#21501=DIRECTION ( 'NONE',  ( -0.000000000000000000, -0.000000000000000000, 1.000000000000000000 ) ) ;
#21503=CARTESIAN_POINT ( 'NONE',  ( 5.405949406249992428, -9.363379034771808662, -115.5937500020483810 ) ) ;
#21504=DIRECTION ( 'NONE',  ( 1.000000000000000000, 0.000000000000000000, 0.000000000000000000 ) ) ;
#21505=CARTESIAN_POINT ( 'NONE',  ( 5.405949406249999534, 9.363379034771803333, -82.28125000204838102 ) ) ;
#21506=CARTESIAN_POINT ( 'NONE',  ( 5.405949406249992428, -9.363379034771808662, -93.09375000204838102 ) ) ;
#21509=CARTESIAN_POINT ( 'NONE',  ( 5.000000000000000000, 8.660254037844385522, -156.6250000040967905 ) ) ;
#21511=EDGE_CURVE ( 'NONE', #10167, #2239, #24588, .T. ) ;
#21514=CARTESIAN_POINT ( 'NONE',  ( 4.999999999999992006, -8.660254037844389075, -13.12500000409674783 ) ) ;
#21518=CARTESIAN_POINT ( 'NONE',  ( 9.999999999999996447, -5.773502691896262640, -68.12500000000000000 ) ) ;
#21520=CARTESIAN_POINT ( 'NONE',  ( 9.999999999999998224, 0.000000000000000000, -83.37500000409677625 ) ) ;
#21523=CARTESIAN_POINT ( 'NONE',  ( -10.81189881249999729, -6.242252689847864744, -74.15625000204836681 ) ) ;
#21525=CARTESIAN_POINT ( 'NONE',  ( 0.000000000000000000, 0.000000000000000000, -200.0000000000000000 ) ) ;
#21527=ORIENTED_EDGE ( 'NONE', *, *, #9863, .F. ) ;
#21528=CARTESIAN_POINT ( 'NONE',  ( 7.644554776091147741E-16, 12.48450537969573659, -199.1562500020484094 ) ) ;
#21530=CARTESIAN_POINT ( 'NONE',  ( -2.293366432827344421E-15, -12.48450537969573659, -10.71875000204836503 ) ) ;
#21532=CARTESIAN_POINT ( 'NONE',  ( -2.293366432827344421E-15, -12.48450537969573659, -142.7187500020484094 ) ) ;
#21533=CARTESIAN_POINT ( 'NONE',  ( 9.999999999999998224, 0.000000000000000000, -49.99999999999998579 ) ) ;
#21534=CARTESIAN_POINT ( 'NONE',  ( 7.071067811865472841, -7.071067811865472841, -200.0000000000000000 ) ) ;
#21535=CARTESIAN_POINT ( 'NONE',  ( 5.405949406249999534, 9.363379034771803333, -128.7812500020483810 ) ) ;
#21537=CARTESIAN_POINT ( 'NONE',  ( -9.999999999999998224, 1.224646799147353059E-15, -182.7500000000000000 ) ) ;
#21539=CARTESIAN_POINT ( 'NONE',  ( -10.81189881249999729, 1.324075727343319199E-15, -108.7812500020483810 ) ) ;
#21540=EDGE_LOOP ( 'NONE', ( #24073, #39988, #976, #5247 ) ) ;
#21541=CARTESIAN_POINT ( 'NONE',  ( 10.00000000000025402, -5.773502691896113426, -154.0000000040967905 ) ) ;
#21542=ORIENTED_EDGE ( 'NONE', *, *, #30976, .T. ) ;
#21543=ORIENTED_EDGE ( 'NONE', *, *, #42108, .F. ) ;
#21544=CARTESIAN_POINT ( 'NONE',  ( 7.644554776091147741E-16, 12.48450537969573659, -37.15625000204836681 ) ) ;
#21547=CARTESIAN_POINT ( 'NONE',  ( 5.405949406249992428, -9.363379034771808662, -90.09375000204838102 ) ) ;
#21550=CARTESIAN_POINT ( 'NONE',  ( -4.999999999999996447, 8.660254037844387298, -123.0000000000000000 ) ) ;
#21552=CARTESIAN_POINT ( 'NONE',  ( -2.121150477449813534E-15, -11.54700538379251284, -77.37500000000000000 ) ) ;
#21553=ADVANCED_FACE ( 'NONE', ( #24161 ), #34080, .T. ) ;
#21554=CARTESIAN_POINT ( 'NONE',  ( -5.405949406249996869, 9.363379034771805109, -117.8437500020483810 ) ) ;
#21556=CARTESIAN_POINT ( 'NONE',  ( 5.405949406249992428, -9.363379034771808662, -0.2812500020483721386 ) ) ;
#21559=CARTESIAN_POINT ( 'NONE',  ( 10.00000000000000000, 5.773502691896255534, -177.7500000040967905 ) ) ;
#21560=CARTESIAN_POINT ( 'NONE',  ( 10.81189881249999729, 6.242252689847867408, -173.9062500020483810 ) ) ;
#21561=CARTESIAN_POINT ( 'NONE',  ( -9.999999999999479527, -5.773502691896549521, -70.50000000409677625 ) ) ;
#21564=CARTESIAN_POINT ( 'NONE',  ( -5.405949406249996869, 9.363379034771805109, -54.84375000204835970 ) ) ;
#21566=CARTESIAN_POINT ( 'NONE',  ( 10.81189881249999551, -6.242252689847874514, -0.1562500020483646446 ) ) ;
#21568=FACE_OUTER_BOUND ( 'NONE', #32335, .T. ) ;
#21570=CARTESIAN_POINT ( 'NONE',  ( -9.999999999999998224, 5.773502691896259087, -95.87499999999998579 ) ) ;
#21572=CARTESIAN_POINT ( 'NONE',  ( -4.999999999999996447, 8.660254037844387298, -102.3750000040967905 ) ) ;
#21573=( BOUNDED_CURVE ( )  B_SPLINE_CURVE ( 2, ( #23581, #36729, #17499, #7167, #20319, #30272, #33720 ),
 .UNSPECIFIED., .F., .F. ) 
 B_SPLINE_CURVE_WITH_KNOTS ( ( 3, 2, 2, 3 ),
 ( 0.3656716417910448325, 0.3669154228855722177, 0.3681592039800996030, 0.3694029850746269883 ),
 .UNSPECIFIED. ) 
 CURVE ( )  GEOMETRIC_REPRESENTATION_ITEM ( )  RATIONAL_B_SPLINE_CURVE ( ( 0.9999999999999940048, 0.8660254037844447028, 1.000000000000000000, 0.8660254037844387076, 1.000000000000000000, 0.8660254037844267172, 1.000000000000011990 ) ) 
 REPRESENTATION_ITEM ( '' )  );
#21574=CARTESIAN_POINT ( 'NONE',  ( 9.999999999999998224, 0.000000000000000000, -149.3750000040967905 ) ) ;
#21577=CARTESIAN_POINT ( 'NONE',  ( -10.81189881249999729, -6.242252689847864744, -98.15625000204840944 ) ) ;
#21578=EDGE_CURVE ( 'NONE', #10744, #900, #7749, .T. ) ;
#21582=CARTESIAN_POINT ( 'NONE',  ( 5.405949406249999534, 9.363379034771803333, -155.7812500020484094 ) ) ;
#21584=ORIENTED_EDGE ( 'NONE', *, *, #37047, .F. ) ;
#21585=CARTESIAN_POINT ( 'NONE',  ( -9.999999999999998224, 5.773502691896259087, -25.37499999999997868 ) ) ;
#21586=CARTESIAN_POINT ( 'NONE',  ( -2.293366432827344421E-15, -12.48450537969573659, -28.90625000204835615 ) ) ;
#21587=CARTESIAN_POINT ( 'NONE',  ( 10.00000000000000000, 5.773502691896255534, -162.3750000000000000 ) ) ;
#21588=CARTESIAN_POINT ( 'NONE',  ( 0.000000000000000000, 0.000000000000000000, -200.0000000000000000 ) ) ;
#21590=DIRECTION ( 'NONE',  ( 1.000000000000000000, 0.000000000000000000, 0.000000000000000000 ) ) ;
#21591=CARTESIAN_POINT ( 'NONE',  ( 10.81189881249999551, -6.242252689847874514, -136.6562500020484094 ) ) ;
#21592=CARTESIAN_POINT ( 'NONE',  ( 6.569145736382243861, 8.192416893213705364, -5.257032284683799044E-15 ) ) ;
#21593=DIRECTION ( 'NONE',  ( -0.000000000000000000, -0.000000000000000000, 1.000000000000000000 ) ) ;
#21594=ORIENTED_EDGE ( 'NONE', *, *, #7221, .T. ) ;
#21595=CARTESIAN_POINT ( 'NONE',  ( 10.81189881249999551, -6.242252689847874514, -58.65625000204838813 ) ) ;
#21598=ORIENTED_EDGE ( 'NONE', *, *, #24376, .F. ) ;
#21600=CARTESIAN_POINT ( 'NONE',  ( -5.000000000000003553, -8.660254037844383745, -197.8750000040967905 ) ) ;
#21601=CARTESIAN_POINT ( 'NONE',  ( -5.405949406249996869, 9.363379034771805109, -155.3437500020483810 ) ) ;
#21604=CARTESIAN_POINT ( 'NONE',  ( -5.405949406250003975, -9.363379034771801557, -3.343750002048367698 ) ) ;
#21605=CARTESIAN_POINT ( 'NONE',  ( -2.293366432827344421E-15, -12.48450537969573659, -136.7187500020483810 ) ) ;
#21606=CARTESIAN_POINT ( 'NONE',  ( -5.405949406250003975, -9.363379034771801557, -99.53125000204839523 ) ) ;
#21608=CARTESIAN_POINT ( 'NONE',  ( 9.999999999999998224, 0.000000000000000000, -161.0000000000000000 ) ) ;
#21610=CARTESIAN_POINT ( 'NONE',  ( -5.405949406249996869, 9.363379034771805109, -5.343750002048369474 ) ) ;
#21612=CARTESIAN_POINT ( 'NONE',  ( 10.81189881249999551, -6.242252689847874514, -196.6562500020484094 ) ) ;
#21613=( BOUNDED_CURVE ( )  B_SPLINE_CURVE ( 2, ( #34731, #492, #14629, #1494, #24589, #25022, #18087 ),
 .UNSPECIFIED., .F., .F. ) 
 B_SPLINE_CURVE_WITH_KNOTS ( ( 3, 2, 2, 3 ),
 ( 0.1417910447761193959, 0.1430348258706467535, 0.1442786069651741387, 0.1455223880597014963 ),
 .UNSPECIFIED. ) 
 CURVE ( )  GEOMETRIC_REPRESENTATION_ITEM ( )  RATIONAL_B_SPLINE_CURVE ( ( 1.000000000000000000, 0.8660254037844387076, 1.000000000000000000, 0.8660254037844387076, 1.000000000000000000, 0.8660254037844387076, 1.000000000000000000 ) ) 
 REPRESENTATION_ITEM ( '' )  );
#21617=CARTESIAN_POINT ( 'NONE',  ( 5.405949406249992428, -9.363379034771808662, -78.09375000204838102 ) ) ;
#21618=CARTESIAN_POINT ( 'NONE',  ( -10.81189881249999729, 1.324075727343319199E-15, -57.59375000204835970 ) ) ;
#21620=CARTESIAN_POINT ( 'NONE',  ( 10.81189881249999907, 6.242252689847868297, -34.40625000204836681 ) ) ;
#21622=DIRECTION ( 'NONE',  ( -0.000000000000000000, -0.000000000000000000, 1.000000000000000000 ) ) ;
#21624=CARTESIAN_POINT ( 'NONE',  ( -2.121150477449813534E-15, -11.54700538379251284, -120.8749999999999858 ) ) ;
#21629=CARTESIAN_POINT ( 'NONE',  ( -2.293366432827344421E-15, -12.48450537969573659, -6.406250002048362369 ) ) ;
#21633=CARTESIAN_POINT ( 'NONE',  ( 9.999999999999998224, 0.000000000000000000, -55.99999999999996447 ) ) ;
#21635=CARTESIAN_POINT ( 'NONE',  ( -4.999999999999996447, 8.660254037844387298, -24.37500000409675849 ) ) ;
#21637=CARTESIAN_POINT ( 'NONE',  ( 0.000000000000000000, 0.000000000000000000, -200.0000000000000000 ) ) ;
#21638=CARTESIAN_POINT ( 'NONE',  ( 7.644554776091147741E-16, 12.48450537969573659, -145.1562500020484094 ) ) ;
#21639=CARTESIAN_POINT ( 'NONE',  ( 10.81189881249999551, -6.242252689847874514, -127.4687500020483810 ) ) ;
#21641=FACE_OUTER_BOUND ( 'NONE', #5682, .T. ) ;
#21642=ORIENTED_EDGE ( 'NONE', *, *, #38786, .T. ) ;
#21645=CARTESIAN_POINT ( 'NONE',  ( 9.999999999999998224, 0.000000000000000000, -200.0000000000000000 ) ) ;
#21646=CARTESIAN_POINT ( 'NONE',  ( -5.405949406250003975, -9.363379034771801557, -180.3437500020483810 ) ) ;
#21647=CARTESIAN_POINT ( 'NONE',  ( 7.644554776091147741E-16, 12.48450537969573659, -33.96875000204834549 ) ) ;
#21649=CARTESIAN_POINT ( 'NONE',  ( 5.405949406249992428, -9.363379034771808662, -172.5937500020484094 ) ) ;
#21650=CARTESIAN_POINT ( 'NONE',  ( -2.293366432827344421E-15, -12.48450537969573659, -151.7187500020483810 ) ) ;
#21651=CARTESIAN_POINT ( 'NONE',  ( -4.999999999999996447, 8.660254037844387298, -178.5000000000000000 ) ) ;
#21656=CARTESIAN_POINT ( 'NONE',  ( -9.999999999999998224, 1.224646799147353059E-15, -33.12500000409676915 ) ) ;
#21659=CARTESIAN_POINT ( 'NONE',  ( -2.293366432827344421E-15, -12.48450537969573659, -82.71875000204838102 ) ) ;
#21660=CARTESIAN_POINT ( 'NONE',  ( -2.121150477449813534E-15, -11.54700538379251284, -82.25000000409676204 ) ) ;
#21661=CARTESIAN_POINT ( 'NONE',  ( -10.81189881249999729, 6.242252689847871849, -56.40625000204837391 ) ) ;
#21664=CARTESIAN_POINT ( 'NONE',  ( 7.644554776091147741E-16, 12.48450537969573659, -116.6562500020483952 ) ) ;
#21665=CARTESIAN_POINT ( 'NONE',  ( -5.405949406250003975, -9.363379034771801557, -146.0312500020483810 ) ) ;
#21667=CARTESIAN_POINT ( 'NONE',  ( 4.999999999999992006, -8.660254037844389075, -118.1250000040967905 ) ) ;
#21669=VERTEX_POINT ( 'NONE', #40310 ) ;
#21672=CARTESIAN_POINT ( 'NONE',  ( 7.070501591499376803E-16, 11.54700538379251284, -192.5000000040968189 ) ) ;
#21673=CARTESIAN_POINT ( 'NONE',  ( -2.293366432827344421E-15, -12.48450537969573659, -178.9062500020484379 ) ) ;
#21674=EDGE_LOOP ( 'NONE', ( #1855, #23816, #18661, #15019 ) ) ;
#21676=CARTESIAN_POINT ( 'NONE',  ( -9.999999999999998224, 5.773502691896259087, -57.25000000409677625 ) ) ;
#21680=ADVANCED_FACE ( 'NONE', ( #8179 ), #4714, .T. ) ;
#21684=CARTESIAN_POINT ( 'NONE',  ( 10.00000000000051159, -5.773502691895965988, -148.0000000040967905 ) ) ;
#21685=CARTESIAN_POINT ( 'NONE',  ( 5.405949406249992428, -9.363379034771808662, -168.2812500020484094 ) ) ;
#21686=DIRECTION ( 'NONE',  ( -0.000000000000000000, -0.000000000000000000, 1.000000000000000000 ) ) ;
#21689=CARTESIAN_POINT ( 'NONE',  ( -9.999999999999998224, 1.224646799147353059E-15, -13.24999999999995559 ) ) ;
#21690=CARTESIAN_POINT ( 'NONE',  ( 9.999999999999998224, 0.000000000000000000, -194.0000000000000000 ) ) ;
#21691=DIRECTION ( 'NONE',  ( 1.000000000000000000, 0.000000000000000000, 0.000000000000000000 ) ) ;
#21692=CARTESIAN_POINT ( 'NONE',  ( -10.81189881249999729, 1.324075727343319199E-15, -80.28125000204838102 ) ) ;
#21695=CARTESIAN_POINT ( 'NONE',  ( 4.999999999999992006, -8.660254037844389075, -119.2500000000000000 ) ) ;
#21698=CARTESIAN_POINT ( 'NONE',  ( -5.405949406249996869, 9.363379034771805109, -35.34375000204836681 ) ) ;
#21700=CARTESIAN_POINT ( 'NONE',  ( 5.405949406249992428, -9.363379034771808662, -9.281250002048352599 ) ) ;
#21701=CARTESIAN_POINT ( 'NONE',  ( -5.405949406249996869, 9.363379034771805109, -59.34375000204835970 ) ) ;
#21702=VERTEX_POINT ( 'NONE', #40520 ) ;
#21705=CARTESIAN_POINT ( 'NONE',  ( -10.81189881249999729, 1.324075727343319199E-15, -198.5937500020484094 ) ) ;
#21706=CARTESIAN_POINT ( 'NONE',  ( -5.405949406250003975, -9.363379034771801557, -175.8437500020483810 ) ) ;
#21708=CARTESIAN_POINT ( 'NONE',  ( 5.000000000000000000, 8.660254037844385522, -43.74999999999998579 ) ) ;
#21709=CARTESIAN_POINT ( 'NONE',  ( 9.999999999999998224, 0.000000000000000000, -75.49999999999998579 ) ) ;
#21713=CARTESIAN_POINT ( 'NONE',  ( -5.405949406250003975, -9.363379034771801557, -103.8437500020483810 ) ) ;
#21715=CARTESIAN_POINT ( 'NONE',  ( 10.81189881249999551, -6.242252689847874514, -82.65625000204836681 ) ) ;
#21716=CARTESIAN_POINT ( 'NONE',  ( 10.81189881249999551, -6.242252689847874514, -94.46875000204838102 ) ) ;
#21718=CARTESIAN_POINT ( 'NONE',  ( 5.000000000000000000, 8.660254037844385522, -147.6250000040967905 ) ) ;
#21723=CARTESIAN_POINT ( 'NONE',  ( 10.00000000000006040, -5.773502691896226224, -197.1250000000000284 ) ) ;
#21725=ORIENTED_EDGE ( 'NONE', *, *, #836, .T. ) ;
#21726=CARTESIAN_POINT ( 'NONE',  ( -5.000000000000003553, -8.660254037844383745, -65.49999999999997158 ) ) ;
#21728=CARTESIAN_POINT ( 'NONE',  ( 7.070501591499377789E-16, 11.54700538379251284, -86.00000000409676204 ) ) ;
#21731=FACE_OUTER_BOUND ( 'NONE', #35280, .T. ) ;
#21734=CARTESIAN_POINT ( 'NONE',  ( -2.293366432827344421E-15, -12.48450537969573659, -75.40625000204838102 ) ) ;
#21735=( BOUNDED_CURVE ( )  B_SPLINE_CURVE ( 2, ( #27255, #8273, #17737, #31155, #37830, #40395, #14931 ),
 .UNSPECIFIED., .F., .F. ) 
 B_SPLINE_CURVE_WITH_KNOTS ( ( 3, 2, 2, 3 ),
 ( 0.9701492537313435305, 0.9713930348258709158, 0.9726368159203981900, 0.9738805970149255753 ),
 .UNSPECIFIED. ) 
 CURVE ( )  GEOMETRIC_REPRESENTATION_ITEM ( )  RATIONAL_B_SPLINE_CURVE ( ( 0.9999999999999761302, 0.8660254037844625774, 1.000000000000000000, 0.8660254037844387076, 1.000000000000000000, 0.8660254037844148378, 1.000000000000023981 ) ) 
 REPRESENTATION_ITEM ( '' )  );
#21736=EDGE_CURVE ( 'NONE', #6545, #5513, #14016, .T. ) ;
#21738=CYLINDRICAL_SURFACE ( 'NONE', #8001, 9.999999999999998224 ) ;
#21740=CARTESIAN_POINT ( 'NONE',  ( -5.405949406249996869, 9.363379034771805109, -194.5312500020484094 ) ) ;
#21743=CARTESIAN_POINT ( 'NONE',  ( 10.81189881249999551, -6.242252689847874514, -7.468750002048351710 ) ) ;
#21745=CARTESIAN_POINT ( 'NONE',  ( -10.81189881249999729, 1.324075727343319199E-15, -144.5937500020483810 ) ) ;
#21746=CARTESIAN_POINT ( 'NONE',  ( 10.00000000000051159, -5.773502691895965988, -50.12499999999997158 ) ) ;
#21748=CARTESIAN_POINT ( 'NONE',  ( 9.999999999999998224, 0.000000000000000000, -111.8750000040967763 ) ) ;
#21750=CARTESIAN_POINT ( 'NONE',  ( -10.00000000000000000, -5.773502691896251982, -175.1249999999999716 ) ) ;
#21751=CARTESIAN_POINT ( 'NONE',  ( -5.405949406250003975, -9.363379034771801557, -98.03125000204839523 ) ) ;
#21754=EDGE_CURVE ( 'NONE', #5836, #2425, #12647, .T. ) ;
#21755=EDGE_LOOP ( 'NONE', ( #15655, #29540, #32370, #36130 ) ) ;
#21756=VERTEX_POINT ( 'NONE', #2767 ) ;
#21757=CARTESIAN_POINT ( 'NONE',  ( -10.81189881249999729, 1.324075727343319199E-15, -30.78125000204837036 ) ) ;
#21760=CARTESIAN_POINT ( 'NONE',  ( 5.405949406249999534, 9.363379034771803333, -89.59375000204838102 ) ) ;
#21761=CARTESIAN_POINT ( 'NONE',  ( 0.000000000000000000, 0.000000000000000000, -200.0000000000000000 ) ) ;
#21765=CARTESIAN_POINT ( 'NONE',  ( 10.00000000000000000, 5.773502691896255534, -9.750000004096756712 ) ) ;
#21766=CARTESIAN_POINT ( 'NONE',  ( 9.999999999999998224, 0.000000000000000000, -198.5000000000000000 ) ) ;
#21767=CARTESIAN_POINT ( 'NONE',  ( -5.405949406250003975, -9.363379034771801557, -115.8437500020483810 ) ) ;
#21770=CARTESIAN_POINT ( 'NONE',  ( -10.81189881249999729, -6.242252689847864744, -5.156250002048356151 ) ) ;
#21773=CARTESIAN_POINT ( 'NONE',  ( -4.999999999999996447, 8.660254037844387298, -175.8750000040967905 ) ) ;
#21774=CARTESIAN_POINT ( 'NONE',  ( -5.405949406250003975, -9.363379034771801557, -173.0312500020484094 ) ) ;
#21775=CARTESIAN_POINT ( 'NONE',  ( 9.999999999998969713, 5.773502691896851502, -102.7500000040967620 ) ) ;
#21778=CARTESIAN_POINT ( 'NONE',  ( 5.405949406249999534, 9.363379034771803333, -43.09375000204837391 ) ) ;
#21780=CARTESIAN_POINT ( 'NONE',  ( 5.405949406249992428, -9.363379034771808662, -4.781250002048375691 ) ) ;
#21782=CARTESIAN_POINT ( 'NONE',  ( 5.000000000000000000, 8.660254037844385522, -54.24999999999996447 ) ) ;
#21784=CARTESIAN_POINT ( 'NONE',  ( -5.000000000000003553, -8.660254037844383745, -89.49999999999998579 ) ) ;
#21786=CARTESIAN_POINT ( 'NONE',  ( 4.999999999999992006, -8.660254037844389075, -106.1250000040967763 ) ) ;
#21787=CARTESIAN_POINT ( 'NONE',  ( 4.999999999999992006, -8.660254037844389075, -149.6250000040967905 ) ) ;
#21790=CARTESIAN_POINT ( 'NONE',  ( 10.81189881249999729, 6.242252689847867408, -98.90625000204839523 ) ) ;
#21791=VERTEX_POINT ( 'NONE', #12035 ) ;
#21793=CARTESIAN_POINT ( 'NONE',  ( -10.00000000000154188, 5.773502691895366468, -28.75000000409670520 ) ) ;
#21794=CARTESIAN_POINT ( 'NONE',  ( -5.405949406250003975, -9.363379034771801557, -155.0312500020484094 ) ) ;
#21796=ORIENTED_EDGE ( 'NONE', *, *, #36841, .F. ) ;
#21797=CARTESIAN_POINT ( 'NONE',  ( -9.999999999999998224, 1.224646799147353059E-15, -23.74999999999996447 ) ) ;
#21798=CARTESIAN_POINT ( 'NONE',  ( 10.81189881249999729, 0.000000000000000000, -25.53125000204836681 ) ) ;
#21799=CARTESIAN_POINT ( 'NONE',  ( -9.999999999999998224, 5.773502691896259087, -151.3750000000000000 ) ) ;
#21801=AXIS2_PLACEMENT_3D ( 'NONE', #9493, #2189, #22660 ) ;
#21802=CARTESIAN_POINT ( 'NONE',  ( 9.999999999999998224, 0.000000000000000000, -80.37500000409677625 ) ) ;
#21803=ADVANCED_FACE ( 'NONE', ( #9229 ), #25228, .T. ) ;
#21804=CARTESIAN_POINT ( 'NONE',  ( -10.81189881249999729, 1.324075727343319199E-15, -126.7812500020483668 ) ) ;
#21805=CARTESIAN_POINT ( 'NONE',  ( -4.999999999999996447, 8.660254037844387298, -75.37500000409677625 ) ) ;
#21807=CARTESIAN_POINT ( 'NONE',  ( -5.405949406249996869, 9.363379034771805109, -62.53125000204837391 ) ) ;
#21809=CARTESIAN_POINT ( 'NONE',  ( 5.405949406249999534, 9.363379034771803333, -107.5937500020483810 ) ) ;
#21810=EDGE_LOOP ( 'NONE', ( #32585, #19195, #15574, #25474 ) ) ;
#21812=CARTESIAN_POINT ( 'NONE',  ( -9.999999999998969713, -5.773502691896847949, -85.50000000409674783 ) ) ;
#21813=CARTESIAN_POINT ( 'NONE',  ( -9.999999999999998224, 1.224646799147353059E-15, -116.7499999999999858 ) ) ;
#21814=CARTESIAN_POINT ( 'NONE',  ( 5.405949406249992428, -9.363379034771808662, -157.5937500020483810 ) ) ;
#21816=CARTESIAN_POINT ( 'NONE',  ( 5.405949406249999534, 9.363379034771803333, -10.09375000204834549 ) ) ;
#21817=CARTESIAN_POINT ( 'NONE',  ( -10.81189881249999729, 6.242252689847871849, -140.2187500020483810 ) ) ;
#21818=( BOUNDED_CURVE ( )  B_SPLINE_CURVE ( 2, ( #20728, #27431, #8007, #40354, #23985, #30252, #7363 ),
 .UNSPECIFIED., .F., .F. ) 
 B_SPLINE_CURVE_WITH_KNOTS ( ( 3, 2, 2, 3 ),
 ( 0.1791044776119403437, 0.1803482587064677289, 0.1815920398009950587, 0.1828358208955224162 ),
 .UNSPECIFIED. ) 
 CURVE ( )  GEOMETRIC_REPRESENTATION_ITEM ( )  RATIONAL_B_SPLINE_CURVE ( ( 0.9999999999999940048, 0.8660254037844447028, 1.000000000000000000, 0.8660254037844387076, 1.000000000000000000, 0.8660254037844357100, 1.000000000000003109 ) ) 
 REPRESENTATION_ITEM ( '' )  );
#21822=CARTESIAN_POINT ( 'NONE',  ( 10.00000000000000000, 5.773502691896255534, -198.7500000040968189 ) ) ;
#21824=CARTESIAN_POINT ( 'NONE',  ( 10.81189881249999729, 0.000000000000000000, -190.5312500020484094 ) ) ;
#21829=CARTESIAN_POINT ( 'NONE',  ( 7.644554776091147741E-16, 12.48450537969573659, -68.46875000204838102 ) ) ;
#21830=CARTESIAN_POINT ( 'NONE',  ( -5.405949406249996869, 9.363379034771805109, -60.84375000204836681 ) ) ;
#21832=CARTESIAN_POINT ( 'NONE',  ( -10.81189881249999729, 1.324075727343319199E-15, -27.78125000204837036 ) ) ;
#21834=CARTESIAN_POINT ( 'NONE',  ( 7.070501591499376803E-16, 11.54700538379251284, -95.00000000409677625 ) ) ;
#21836=CARTESIAN_POINT ( 'NONE',  ( -9.999999999999998224, 1.224646799147353059E-15, -112.2499999999999858 ) ) ;
#21840=CARTESIAN_POINT ( 'NONE',  ( -10.81189881249999729, -6.242252689847864744, -11.15625000204838457 ) ) ;
#21846=CARTESIAN_POINT ( 'NONE',  ( 10.00000000000000000, 5.773502691896255534, -52.87499999999997868 ) ) ;
#21847=CARTESIAN_POINT ( 'NONE',  ( 10.00000000000000000, 5.773502691896255534, -27.75000000409677980 ) ) ;
#21849=CARTESIAN_POINT ( 'NONE',  ( -4.999999999999996447, 8.660254037844387298, -61.49999999999997158 ) ) ;
#21851=LINE ( 'NONE', #24893, #29003 ) ;
#21852=CARTESIAN_POINT ( 'NONE',  ( -10.81189881249999729, 1.324075727343319199E-15, -144.7812500020483810 ) ) ;
#21853=CARTESIAN_POINT ( 'NONE',  ( 10.81189881249999729, 0.000000000000000000, -130.3437500020484094 ) ) ;
#21854=CARTESIAN_POINT ( 'NONE',  ( 4.999999999999992006, -8.660254037844389075, -65.24999999999997158 ) ) ;
#21855=CARTESIAN_POINT ( 'NONE',  ( -5.000000000000003553, -8.660254037844383745, -127.3750000040967905 ) ) ;
#21856=ORIENTED_EDGE ( 'NONE', *, *, #8284, .F. ) ;
#21857=VERTEX_POINT ( 'NONE', #15689 ) ;
#21858=ORIENTED_EDGE ( 'NONE', *, *, #23848, .F. ) ;
#21860=CARTESIAN_POINT ( 'NONE',  ( -2.121150477449813534E-15, -11.54700538379251284, -7.250000004096746054 ) ) ;
#21862=CARTESIAN_POINT ( 'NONE',  ( 7.644554776091147741E-16, 12.48450537969573659, -182.4687500020484094 ) ) ;
#21863=CARTESIAN_POINT ( 'NONE',  ( 10.81189881249999551, -6.242252689847874514, -34.46875000204835260 ) ) ;
#21864=DIRECTION ( 'NONE',  ( -0.000000000000000000, -0.000000000000000000, 1.000000000000000000 ) ) ;
#21865=CARTESIAN_POINT ( 'NONE',  ( -10.81189881249999729, -6.242252689847864744, -166.9687500020484094 ) ) ;
#21866=CARTESIAN_POINT ( 'NONE',  ( 10.81189881249999729, 0.000000000000000000, -154.3437500020483810 ) ) ;
#21871=CARTESIAN_POINT ( 'NONE',  ( 0.000000000000000000, 0.000000000000000000, -200.0000000000000000 ) ) ;
#21872=( BOUNDED_CURVE ( )  B_SPLINE_CURVE ( 2, ( #38104, #9171, #28829, #5304, #12393, #18457, #22342 ),
 .UNSPECIFIED., .F., .F. ) 
 B_SPLINE_CURVE_WITH_KNOTS ( ( 3, 2, 2, 3 ),
 ( 0.1380597014925373234, 0.1393034825870646809, 0.1405472636815920384, 0.1417910447761193959 ),
 .UNSPECIFIED. ) 
 CURVE ( )  GEOMETRIC_REPRESENTATION_ITEM ( )  RATIONAL_B_SPLINE_CURVE ( ( 1.000000000000000000, 0.8660254037844387076, 1.000000000000000000, 0.8660254037844387076, 1.000000000000000000, 0.8660254037844387076, 1.000000000000000000 ) ) 
 REPRESENTATION_ITEM ( '' )  );
#21873=CARTESIAN_POINT ( 'NONE',  ( 9.999999999999872102, 5.773502691896329253, -169.8750000000000000 ) ) ;
#21875=CARTESIAN_POINT ( 'NONE',  ( -2.293366432827344421E-15, -12.48450537969573659, -78.21875000204838102 ) ) ;
#21876=DIRECTION ( 'NONE',  ( -0.000000000000000000, -0.000000000000000000, 1.000000000000000000 ) ) ;
#21877=CARTESIAN_POINT ( 'NONE',  ( 5.405949406249992428, -9.363379034771808662, -46.78125000204838813 ) ) ;
#21878=CARTESIAN_POINT ( 'NONE',  ( 0.000000000000000000, 0.000000000000000000, -200.0000000000000000 ) ) ;
#21880=CARTESIAN_POINT ( 'NONE',  ( -10.81189881249999907, -6.242252689847864744, -113.1562500020483952 ) ) ;
#21881=CARTESIAN_POINT ( 'NONE',  ( 5.405949406249992428, -9.363379034771808662, -147.2812500020483810 ) ) ;
#21882=CARTESIAN_POINT ( 'NONE',  ( 10.00000000000102318, -5.773502691895667560, -29.12499999999995381 ) ) ;
#21884=CARTESIAN_POINT ( 'NONE',  ( -9.999999999999998224, 1.224646799147353059E-15, -124.6250000040967763 ) ) ;
#21886=ORIENTED_EDGE ( 'NONE', *, *, #23947, .F. ) ;
#21889=ADVANCED_FACE ( 'NONE', ( #42022 ), #4985, .F. ) ;
#21890=CARTESIAN_POINT ( 'NONE',  ( -10.81189881249999729, 1.324075727343319199E-15, -183.7812500020484094 ) ) ;
#21893=CARTESIAN_POINT ( 'NONE',  ( 7.070501591499377789E-16, 11.54700538379251284, -53.00000000409676915 ) ) ;
#21896=CARTESIAN_POINT ( 'NONE',  ( 9.999999999998969713, 5.773502691896851502, -9.750000004096735395 ) ) ;
#21897=CARTESIAN_POINT ( 'NONE',  ( 5.405949406249992428, -9.363379034771808662, -166.7812500020484094 ) ) ;
#21899=CARTESIAN_POINT ( 'NONE',  ( 7.070501591499376803E-16, 11.54700538379251284, -64.62499999999998579 ) ) ;
#21903=CARTESIAN_POINT ( 'NONE',  ( -9.999999999999998224, 1.224646799147353059E-15, -52.62500000409675494 ) ) ;
#21905=CARTESIAN_POINT ( 'NONE',  ( 10.81189881249999551, -6.242252689847874514, -81.15625000204839523 ) ) ;
#21908=ORIENTED_EDGE ( 'NONE', *, *, #27480, .F. ) ;
#21910=CARTESIAN_POINT ( 'NONE',  ( 10.81189881249999729, 6.242252689847867408, -29.71875000204834549 ) ) ;
#21912=CARTESIAN_POINT ( 'NONE',  ( -10.81189881249999729, 1.324075727343319199E-15, -3.781250002048375247 ) ) ;
#21913=CARTESIAN_POINT ( 'NONE',  ( -5.405949406249996869, 9.363379034771805109, -53.34375000204835970 ) ) ;
#21914=ORIENTED_EDGE ( 'NONE', *, *, #38889, .T. ) ;
#21915=CARTESIAN_POINT ( 'NONE',  ( 9.999999999999998224, 0.000000000000000000, -51.49999999999996447 ) ) ;
#21916=EDGE_CURVE ( 'NONE', #24037, #10798, #31718, .T. ) ;
#21918=CARTESIAN_POINT ( 'NONE',  ( 5.405949406249992428, -9.363379034771808662, -184.5937500020483810 ) ) ;
#21919=CARTESIAN_POINT ( 'NONE',  ( -5.405949406250003975, -9.363379034771801557, -177.3437500020483810 ) ) ;
#21922=CARTESIAN_POINT ( 'NONE',  ( 9.999999999999998224, 0.000000000000000000, -200.0000000000000000 ) ) ;
#21925=CARTESIAN_POINT ( 'NONE',  ( -2.293366432827344421E-15, -12.48450537969573659, -102.2187500020483952 ) ) ;
#21926=CARTESIAN_POINT ( 'NONE',  ( 0.000000000000000000, 0.000000000000000000, -200.0000000000000000 ) ) ;
#21928=CARTESIAN_POINT ( 'NONE',  ( 5.405949406249999534, 9.363379034771803333, -79.28125000204838102 ) ) ;
#21929=CARTESIAN_POINT ( 'NONE',  ( 10.81189881249999729, 0.000000000000000000, -94.34375000204838102 ) ) ;
#21930=AXIS2_PLACEMENT_3D ( 'NONE', #24483, #34410, #30319 ) ;
#21932=CARTESIAN_POINT ( 'NONE',  ( -9.999999999999998224, 5.773502691896259087, -148.7500000040967905 ) ) ;
#21937=CARTESIAN_POINT ( 'NONE',  ( 7.070501591499376803E-16, 11.54700538379251284, -98.00000000409677625 ) ) ;
#21938=LINE ( 'NONE', #25402, #1330 ) ;
#21940=ORIENTED_EDGE ( 'NONE', *, *, #41105, .T. ) ;
#21941=CARTESIAN_POINT ( 'NONE',  ( -9.999999999999998224, 5.773502691896259087, -62.87499999999996447 ) ) ;
#21943=CARTESIAN_POINT ( 'NONE',  ( 4.999999999999992006, -8.660254037844389075, -74.62500000409677625 ) ) ;
#21944=CARTESIAN_POINT ( 'NONE',  ( -9.999999999999998224, 1.224646799147353059E-15, -85.62500000409677625 ) ) ;
#21947=CARTESIAN_POINT ( 'NONE',  ( -10.81189881249999729, 1.324075727343319199E-15, -77.28125000204838102 ) ) ;
#21949=CARTESIAN_POINT ( 'NONE',  ( -11.54700538379251817, 20.00000000000000355, 45.00000000000009237 ) ) ;
#21951=EDGE_LOOP ( 'NONE', ( #10956, #27895, #32795, #14442 ) ) ;
#21952=CARTESIAN_POINT ( 'NONE',  ( -5.405949406249996869, 9.363379034771805109, -196.0312500020484094 ) ) ;
#21954=CARTESIAN_POINT ( 'NONE',  ( 10.81189881249999551, -6.242252689847874514, -2.968750002048361925 ) ) ;
#21955=CARTESIAN_POINT ( 'NONE',  ( 9.999999999999742428, 5.773502691896404748, -186.7500000040967905 ) ) ;
#21956=CARTESIAN_POINT ( 'NONE',  ( 7.070501591499376803E-16, 11.54700538379251284, -192.1250000000000284 ) ) ;
#21957=LINE ( 'NONE', #35772, #39679 ) ;
#21958=CARTESIAN_POINT ( 'NONE',  ( -4.999999999999996447, 8.660254037844387298, -177.0000000000000000 ) ) ;
#21959=CARTESIAN_POINT ( 'NONE',  ( 9.999999999999998224, 0.000000000000000000, -106.9999999999999858 ) ) ;
#21960=CARTESIAN_POINT ( 'NONE',  ( -10.81189881249999729, 6.242252689847871849, -105.9062500020483810 ) ) ;
#21961=VERTEX_POINT ( 'NONE', #34255 ) ;
#21962=CARTESIAN_POINT ( 'NONE',  ( -9.999999999999872102, -5.773502691896326589, -162.0000000040967620 ) ) ;
#21964=VERTEX_POINT ( 'NONE', #38482 ) ;
#21965=CARTESIAN_POINT ( 'NONE',  ( -10.81189881249999729, 1.324075727343319199E-15, -32.28125000204837391 ) ) ;
#21967=CARTESIAN_POINT ( 'NONE',  ( 5.405949406249992428, -9.363379034771808662, -78.09375000204838102 ) ) ;
#21968=DIRECTION ( 'NONE',  ( -0.000000000000000000, -0.000000000000000000, 1.000000000000000000 ) ) ;
#21971=ADVANCED_FACE ( 'NONE', ( #4668 ), #8131, .T. ) ;
#21972=EDGE_CURVE ( 'NONE', #34874, #16149, #36112, .T. ) ;
#21973=CARTESIAN_POINT ( 'NONE',  ( 9.999999999999998224, 0.000000000000000000, -156.8750000040967905 ) ) ;
#21975=CARTESIAN_POINT ( 'NONE',  ( 9.999999999999996447, -5.773502691896262640, -13.00000000409675849 ) ) ;
#21977=CARTESIAN_POINT ( 'NONE',  ( -5.405949406249996869, 9.363379034771805109, -126.8437500020483952 ) ) ;
#21978=CARTESIAN_POINT ( 'NONE',  ( 5.405949406249992428, -9.363379034771808662, -117.0937500020483810 ) ) ;
#21983=CARTESIAN_POINT ( 'NONE',  ( -5.000000000000003553, -8.660254037844383745, -172.3750000040968189 ) ) ;
#21984=CARTESIAN_POINT ( 'NONE',  ( -2.293366432827344421E-15, -12.48450537969573659, -168.4062500020484379 ) ) ;
#21985=( BOUNDED_CURVE ( )  B_SPLINE_CURVE ( 2, ( #8802, #11808, #1910, #5350, #41592, #14391, #28459 ),
 .UNSPECIFIED., .F., .F. ) 
 B_SPLINE_CURVE_WITH_KNOTS ( ( 3, 2, 2, 3 ),
 ( 0.1119402985074627876, 0.1131840796019901035, 0.1144278606965174333, 0.1156716417910447492 ),
 .UNSPECIFIED. ) 
 CURVE ( )  GEOMETRIC_REPRESENTATION_ITEM ( )  RATIONAL_B_SPLINE_CURVE ( ( 0.9999999999999894529, 0.8660254037844491437, 1.000000000000000000, 0.8660254037844387076, 1.000000000000000000, 0.8660254037844417052, 0.9999999999999970024 ) ) 
 REPRESENTATION_ITEM ( '' )  );
#21989=CARTESIAN_POINT ( 'NONE',  ( 5.405949406249999534, 9.363379034771803333, -41.59375000204837391 ) ) ;
#21991=CARTESIAN_POINT ( 'NONE',  ( -5.405949406249996869, 9.363379034771805109, -1.031250002048372805 ) ) ;
#21995=CARTESIAN_POINT ( 'NONE',  ( -2.121150477449813534E-15, -11.54700538379251284, -86.37499999999997158 ) ) ;
#21997=CARTESIAN_POINT ( 'NONE',  ( -9.999999999999998224, 1.224646799147353059E-15, -103.6250000040967763 ) ) ;
#21999=AXIS2_PLACEMENT_3D ( 'NONE', #21878, #41712, #14740 ) ;
#22000=CARTESIAN_POINT ( 'NONE',  ( 9.999999999999998224, 0.000000000000000000, -200.0000000000000000 ) ) ;
#22002=CARTESIAN_POINT ( 'NONE',  ( 10.81189881249999729, 0.000000000000000000, -97.53125000204839523 ) ) ;
#22003=ORIENTED_EDGE ( 'NONE', *, *, #948, .F. ) ;
#22006=CARTESIAN_POINT ( 'NONE',  ( 7.644554776091147741E-16, 12.48450537969573659, -154.1562500020484094 ) ) ;
#22008=VERTEX_POINT ( 'NONE', #11129 ) ;
#22010=CARTESIAN_POINT ( 'NONE',  ( -4.999999999999996447, 8.660254037844387298, -14.99999999999995737 ) ) ;
#22011=VECTOR ( 'NONE', #37919, 1000.000000000000000 ) ;
#22012=CARTESIAN_POINT ( 'NONE',  ( -10.81189881249999729, 6.242252689847871849, -27.90625000204838102 ) ) ;
#22013=CARTESIAN_POINT ( 'NONE',  ( 4.999999999999992006, -8.660254037844389075, -152.2500000000000000 ) ) ;
#22016=VECTOR ( 'NONE', #26598, 1000.000000000000000 ) ;
#22017=CARTESIAN_POINT ( 'NONE',  ( -9.999999999999998224, 1.224646799147353059E-15, -199.2500000000000000 ) ) ;
#22018=CARTESIAN_POINT ( 'NONE',  ( -10.81189881249999907, -6.242252689847864744, -129.6562500020483810 ) ) ;
#22020=PLANE ( 'NONE',  #15167 ) ;
#22023=EDGE_CURVE ( 'NONE', #30574, #39730, #12145, .T. ) ;
#22024=ORIENTED_EDGE ( 'NONE', *, *, #21208, .F. ) ;
#22025=CARTESIAN_POINT ( 'NONE',  ( -5.405949406250003975, -9.363379034771801557, -54.53125000204836681 ) ) ;
#22027=CARTESIAN_POINT ( 'NONE',  ( 10.81189881249999551, -6.242252689847874514, -112.4687500020483810 ) ) ;
#22028=ORIENTED_EDGE ( 'NONE', *, *, #8296, .T. ) ;
#22029=ORIENTED_EDGE ( 'NONE', *, *, #8605, .T. ) ;
#22031=CARTESIAN_POINT ( 'NONE',  ( 11.54700538379250396, 20.00000000000000711, 45.00000000000009237 ) ) ;
#22032=CARTESIAN_POINT ( 'NONE',  ( 7.644554776091147741E-16, 12.48450537969573659, -161.4687500020484094 ) ) ;
#22034=CARTESIAN_POINT ( 'NONE',  ( -10.81189881249999907, -6.242252689847864744, -7.968750002048352599 ) ) ;
#22036=AXIS2_PLACEMENT_3D ( 'NONE', #10742, #33857, #843 ) ;
#22037=CARTESIAN_POINT ( 'NONE',  ( 5.405949406249999534, 9.363379034771803333, -140.5937500020483810 ) ) ;
#22041=CARTESIAN_POINT ( 'NONE',  ( -10.00000000000000000, -5.773502691896251982, -196.5000000040967905 ) ) ;
#22043=CARTESIAN_POINT ( 'NONE',  ( 10.81189881249999729, 0.000000000000000000, -193.5312500020484094 ) ) ;
#22044=CARTESIAN_POINT ( 'NONE',  ( -4.999999999999996447, 8.660254037844387298, -165.3750000040967905 ) ) ;
#22047=CARTESIAN_POINT ( 'NONE',  ( -10.81189881249999729, 1.324075727343319199E-15, -69.59375000204836681 ) ) ;
#22048=CARTESIAN_POINT ( 'NONE',  ( -5.405949406249996869, 9.363379034771805109, -54.84375000204835970 ) ) ;
#22050=CARTESIAN_POINT ( 'NONE',  ( 10.81189881249999729, 0.000000000000000000, -30.03125000204837036 ) ) ;
#22052=CARTESIAN_POINT ( 'NONE',  ( -4.999999999999996447, 8.660254037844387298, -52.87500000409675494 ) ) ;
#22054=CARTESIAN_POINT ( 'NONE',  ( -4.999999999999996447, 8.660254037844387298, -115.4999999999999858 ) ) ;
#22055=DIRECTION ( 'NONE',  ( -0.000000000000000000, -0.000000000000000000, 1.000000000000000000 ) ) ;
#22058=CARTESIAN_POINT ( 'NONE',  ( 7.644554776091147741E-16, 12.48450537969573659, -10.15625000204837924 ) ) ;
#22059=EDGE_CURVE ( 'NONE', #41040, #25114, #39853, .T. ) ;
#22060=VERTEX_POINT ( 'NONE', #13304 ) ;
#22061=CARTESIAN_POINT ( 'NONE',  ( 0.000000000000000000, 0.000000000000000000, -200.0000000000000000 ) ) ;
#22063=CARTESIAN_POINT ( 'NONE',  ( -9.999999999999479527, -5.773502691896549521, -39.00000000409675494 ) ) ;
#22065=CARTESIAN_POINT ( 'NONE',  ( -2.121150477449813534E-15, -11.54700538379251284, -38.37499999999995737 ) ) ;
#22066=CARTESIAN_POINT ( 'NONE',  ( -4.999999999999996447, 8.660254037844387298, -22.87500000409675849 ) ) ;
#22067=FACE_OUTER_BOUND ( 'NONE', #23070, .T. ) ;
#22069=DIRECTION ( 'NONE',  ( -1.000000000000000000, 0.000000000000000000, 0.000000000000000000 ) ) ;
#22070=CARTESIAN_POINT ( 'NONE',  ( -2.293366432827344421E-15, -12.48450537969573659, -144.4062500020484094 ) ) ;
#22072=CARTESIAN_POINT ( 'NONE',  ( -5.405949406250003975, -9.363379034771801557, -150.5312500020483810 ) ) ;
#22073=CARTESIAN_POINT ( 'NONE',  ( -9.999999999999998224, 1.224646799147353059E-15, -65.74999999999997158 ) ) ;
#22074=CYLINDRICAL_SURFACE ( 'NONE', #7293, 9.999999999999998224 ) ;
#22078=( BOUNDED_CURVE ( )  B_SPLINE_CURVE ( 2, ( #34051, #7289, #31248, #27354, #7498, #37706, #10935 ),
 .UNSPECIFIED., .F., .F. ) 
 B_SPLINE_CURVE_WITH_KNOTS ( ( 3, 2, 2, 3 ),
 ( 0.6791044776119405935, 0.6803482587064679787, 0.6815920398009952530, 0.6828358208955226383 ),
 .UNSPECIFIED. ) 
 CURVE ( )  GEOMETRIC_REPRESENTATION_ITEM ( )  RATIONAL_B_SPLINE_CURVE ( ( 0.9999999999999641398, 0.8660254037844745678, 1.000000000000000000, 0.8660254037844387076, 1.000000000000000000, 0.8660254037844148378, 1.000000000000023981 ) ) 
 REPRESENTATION_ITEM ( '' )  );
#22079=FACE_OUTER_BOUND ( 'NONE', #24140, .T. ) ;
#22080=CARTESIAN_POINT ( 'NONE',  ( -10.81189881249999729, 1.324075727343319199E-15, -183.5937500020483810 ) ) ;
#22081=CARTESIAN_POINT ( 'NONE',  ( 10.81189881249999551, -6.242252689847874514, -31.46875000204835260 ) ) ;
#22082=CARTESIAN_POINT ( 'NONE',  ( -10.00000000000076916, 5.773502691895813221, -109.7500000040967620 ) ) ;
#22083=CARTESIAN_POINT ( 'NONE',  ( 5.405949406249992428, -9.363379034771808662, -163.5937500020484094 ) ) ;
#22084=CARTESIAN_POINT ( 'NONE',  ( 10.81189881249999729, 0.000000000000000000, -155.8437500020483810 ) ) ;
#22085=CYLINDRICAL_SURFACE ( 'NONE', #27264, 9.999999999999998224 ) ;
#22090=CARTESIAN_POINT ( 'NONE',  ( -9.999999999999998224, 1.224646799147353059E-15, -152.7500000000000000 ) ) ;
#22091=CARTESIAN_POINT ( 'NONE',  ( 9.999999999999998224, 0.000000000000000000, -33.87500000409676915 ) ) ;
#22093=VECTOR ( 'NONE', #27377, 1000.000000000000000 ) ;
#22094=EDGE_CURVE ( 'NONE', #6996, #8228, #40270, .T. ) ;
#22095=CARTESIAN_POINT ( 'NONE',  ( -5.405949406249996869, 9.363379034771805109, -77.34375000204838102 ) ) ;
#22097=CARTESIAN_POINT ( 'NONE',  ( -5.405949406249996869, 9.363379034771805109, -50.53125000204835970 ) ) ;
#22100=CARTESIAN_POINT ( 'NONE',  ( 7.070501591499377789E-16, 11.54700538379251284, -138.1250000000000000 ) ) ;
#22101=CARTESIAN_POINT ( 'NONE',  ( 10.81189881249999729, 6.242252689847867408, -145.4062500020484094 ) ) ;
#22102=DIRECTION ( 'NONE',  ( 1.000000000000000000, 0.000000000000000000, 0.000000000000000000 ) ) ;
#22104=CARTESIAN_POINT ( 'NONE',  ( -9.999999999999998224, 1.224646799147353059E-15, -121.6250000040967905 ) ) ;
#22109=CARTESIAN_POINT ( 'NONE',  ( 9.999999999999998224, 0.000000000000000000, -140.3750000040967905 ) ) ;
#22110=CARTESIAN_POINT ( 'NONE',  ( -5.405949406249996869, 9.363379034771805109, -175.0312500020484094 ) ) ;
#22111=CARTESIAN_POINT ( 'NONE',  ( 7.070501591499377789E-16, 11.54700538379251284, -51.50000000409676204 ) ) ;
#22112=CARTESIAN_POINT ( 'NONE',  ( 5.000000000000000000, 8.660254037844385522, -48.62500000409678336 ) ) ;
#22115=DIRECTION ( 'NONE',  ( 1.000000000000000000, 0.000000000000000000, 0.000000000000000000 ) ) ;
#22116=CARTESIAN_POINT ( 'NONE',  ( -10.81189881249999729, 6.242252689847871849, -165.9062500020483810 ) ) ;
#22117=CARTESIAN_POINT ( 'NONE',  ( 0.000000000000000000, 0.000000000000000000, -200.0000000000000000 ) ) ;
#22118=DIRECTION ( 'NONE',  ( -0.000000000000000000, -0.000000000000000000, 1.000000000000000000 ) ) ;
#22119=VERTEX_POINT ( 'NONE', #26493 ) ;
#22120=CYLINDRICAL_SURFACE ( 'NONE', #13215, 9.999999999999998224 ) ;
#22121=DIRECTION ( 'NONE',  ( -0.000000000000000000, -0.000000000000000000, 1.000000000000000000 ) ) ;
#22122=( BOUNDED_CURVE ( )  B_SPLINE_CURVE ( 2, ( #31636, #5726, #41091, #18447, #34447, #31418, #18011 ),
 .UNSPECIFIED., .F., .F. ) 
 B_SPLINE_CURVE_WITH_KNOTS ( ( 3, 2, 2, 3 ),
 ( 0.9888059701492539766, 0.9900497512437813619, 0.9912935323383086361, 0.9925373134328360214 ),
 .UNSPECIFIED. ) 
 CURVE ( )  GEOMETRIC_REPRESENTATION_ITEM ( )  RATIONAL_B_SPLINE_CURVE ( ( 0.9999999999999761302, 0.8660254037844625774, 1.000000000000000000, 0.8660254037844387076, 1.000000000000000000, 0.8660254037844148378, 1.000000000000023981 ) ) 
 REPRESENTATION_ITEM ( '' )  );
#22123=CARTESIAN_POINT ( 'NONE',  ( -9.999999999999998224, 1.224646799147353059E-15, -71.74999999999998579 ) ) ;
#22124=CARTESIAN_POINT ( 'NONE',  ( -10.81189881249999907, -6.242252689847864744, -81.65625000204839523 ) ) ;
#22125=VERTEX_POINT ( 'NONE', #27127 ) ;
#22129=CARTESIAN_POINT ( 'NONE',  ( -5.405949406250003975, -9.363379034771801557, -33.34375000204836681 ) ) ;
#22130=CARTESIAN_POINT ( 'NONE',  ( 4.999999999999992006, -8.660254037844389075, -53.24999999999996447 ) ) ;
#22131=CARTESIAN_POINT ( 'NONE',  ( -10.81189881249999729, 6.242252689847871849, -2.406250002048375247 ) ) ;
#22132=( BOUNDED_CURVE ( )  B_SPLINE_CURVE ( 2, ( #34881, #18239, #35305, #31429, #41324, #41546, #24748 ),
 .UNSPECIFIED., .F., .F. ) 
 B_SPLINE_CURVE_WITH_KNOTS ( ( 3, 2, 2, 3 ),
 ( 0.06343283582089558059, 0.06467661691542293811, 0.06592039800995032339, 0.06716417910447768091 ),
 .UNSPECIFIED. ) 
 CURVE ( )  GEOMETRIC_REPRESENTATION_ITEM ( )  RATIONAL_B_SPLINE_CURVE ( ( 0.9999999999999940048, 0.8660254037844447028, 1.000000000000000000, 0.8660254037844387076, 1.000000000000000000, 0.8660254037844312691, 1.000000000000007550 ) ) 
 REPRESENTATION_ITEM ( '' )  );
#22133=CARTESIAN_POINT ( 'NONE',  ( 5.405949406249999534, 9.363379034771803333, -53.59375000204835970 ) ) ;
#22137=CARTESIAN_POINT ( 'NONE',  ( 5.405949406249992428, -9.363379034771808662, -189.0937500020483810 ) ) ;
#22138=CARTESIAN_POINT ( 'NONE',  ( 10.81189881249999551, -6.242252689847874514, -176.9687500020483810 ) ) ;
#22142=DIRECTION ( 'NONE',  ( -0.000000000000000000, -0.000000000000000000, 1.000000000000000000 ) ) ;
#22145=CARTESIAN_POINT ( 'NONE',  ( -2.293366432827344421E-15, -12.48450537969573659, -106.7187500020483668 ) ) ;
#22146=CARTESIAN_POINT ( 'NONE',  ( -9.999999999999998224, 1.224646799147353059E-15, -17.74999999999996092 ) ) ;
#22147=CARTESIAN_POINT ( 'NONE',  ( 10.81189881249999907, 6.242252689847868297, -77.90625000204836681 ) ) ;
#22148=CARTESIAN_POINT ( 'NONE',  ( -5.405949406250003975, -9.363379034771801557, -93.34375000204838102 ) ) ;
#22150=CARTESIAN_POINT ( 'NONE',  ( -5.000000000000003553, -8.660254037844383745, -146.8750000040967905 ) ) ;
#22152=VECTOR ( 'NONE', #18342, 1000.000000000000000 ) ;
#22153=VERTEX_POINT ( 'NONE', #7486 ) ;
#22160=CARTESIAN_POINT ( 'NONE',  ( 5.000000000000000000, 8.660254037844385522, -61.74999999999997158 ) ) ;
#22162=CARTESIAN_POINT ( 'NONE',  ( -9.999999999999998224, 1.224646799147353059E-15, -72.12500000409677625 ) ) ;
#22164=CARTESIAN_POINT ( 'NONE',  ( -9.999999999999998224, 1.224646799147353059E-15, -200.0000000000000000 ) ) ;
#22166=CARTESIAN_POINT ( 'NONE',  ( -5.405949406250003975, -9.363379034771801557, -68.03125000204838102 ) ) ;
#22170=ORIENTED_EDGE ( 'NONE', *, *, #20888, .T. ) ;
#22171=CARTESIAN_POINT ( 'NONE',  ( 5.405949406249992428, -9.363379034771808662, -196.7812500020484094 ) ) ;
#22172=VECTOR ( 'NONE', #34994, 1000.000000000000000 ) ;
#22174=EDGE_CURVE ( 'NONE', #317, #14499, #20637, .T. ) ;
#22175=CARTESIAN_POINT ( 'NONE',  ( 10.81189881249999729, 6.242252689847867408, -8.718750002048357928 ) ) ;
#22176=DIRECTION ( 'NONE',  ( -0.000000000000000000, -0.000000000000000000, 1.000000000000000000 ) ) ;
#22177=CARTESIAN_POINT ( 'NONE',  ( -9.999999999998969713, -5.773502691896847949, -63.00000000409676915 ) ) ;
#22178=LINE ( 'NONE', #42429, #10044 ) ;
#22179=CARTESIAN_POINT ( 'NONE',  ( -10.00000000000000000, -5.773502691896251982, -178.1250000000000284 ) ) ;
#22180=CARTESIAN_POINT ( 'NONE',  ( 0.000000000000000000, 0.000000000000000000, -200.0000000000000000 ) ) ;
#22181=CARTESIAN_POINT ( 'NONE',  ( -5.405949406250003975, -9.363379034771801557, -102.5312500020483952 ) ) ;
#22182=VERTEX_POINT ( 'NONE', #10923 ) ;
#22184=VERTEX_POINT ( 'NONE', #17392 ) ;
#22185=CARTESIAN_POINT ( 'NONE',  ( -2.293366432827344421E-15, -12.48450537969573659, -27.40625000204838102 ) ) ;
#22188=CARTESIAN_POINT ( 'NONE',  ( -10.81189881249999907, -6.242252689847864744, -79.96875000204836681 ) ) ;
#22191=CARTESIAN_POINT ( 'NONE',  ( 9.999999999999998224, 0.000000000000000000, -200.0000000000000000 ) ) ;
#22192=FACE_OUTER_BOUND ( 'NONE', #846, .T. ) ;
#22194=CARTESIAN_POINT ( 'NONE',  ( 9.999999999999996447, -5.773502691896262640, -8.500000004096751383 ) ) ;
#22195=CARTESIAN_POINT ( 'NONE',  ( 10.81189881249999729, 0.000000000000000000, -131.8437500020484094 ) ) ;
#22196=CARTESIAN_POINT ( 'NONE',  ( -10.81189881249999729, 6.242252689847871849, -119.2187500020483810 ) ) ;
#22197=( BOUNDED_CURVE ( )  B_SPLINE_CURVE ( 2, ( #20234, #40493, #13736, #26926, #13949, #26717, #10727 ),
 .UNSPECIFIED., .F., .F. ) 
 B_SPLINE_CURVE_WITH_KNOTS ( ( 3, 2, 2, 3 ),
 ( 0.1492537313432835966, 0.1504975124378109819, 0.1517412935323383116, 0.1529850746268656692 ),
 .UNSPECIFIED. ) 
 CURVE ( )  GEOMETRIC_REPRESENTATION_ITEM ( )  RATIONAL_B_SPLINE_CURVE ( ( 0.9999999999999970024, 0.8660254037844417052, 1.000000000000000000, 0.8660254037844387076, 1.000000000000000000, 0.8660254037844387076, 1.000000000000000000 ) ) 
 REPRESENTATION_ITEM ( '' )  );
#22200=CARTESIAN_POINT ( 'NONE',  ( 9.999999999999996447, -5.773502691896262640, -170.5000000040967905 ) ) ;
#22201=CARTESIAN_POINT ( 'NONE',  ( 7.644554776091147741E-16, 12.48450537969573659, -167.6562500020484094 ) ) ;
#22202=CARTESIAN_POINT ( 'NONE',  ( 9.999999999999998224, 0.000000000000000000, -155.0000000000000000 ) ) ;
#22205=CARTESIAN_POINT ( 'NONE',  ( 10.81189881249999729, 6.242252689847867408, -43.21875000204835970 ) ) ;
#22207=CARTESIAN_POINT ( 'NONE',  ( 5.405949406249999534, 9.363379034771803333, -5.781250002048377468 ) ) ;
#22211=CARTESIAN_POINT ( 'NONE',  ( 9.999999999999998224, 0.000000000000000000, -93.49999999999998579 ) ) ;
#22213=CARTESIAN_POINT ( 'NONE',  ( 7.070501591499377789E-16, 11.54700538379251284, -101.0000000040967905 ) ) ;
#22216=CARTESIAN_POINT ( 'NONE',  ( 5.405949406249992428, -9.363379034771808662, -91.78125000204838102 ) ) ;
#22217=VERTEX_POINT ( 'NONE', #30589 ) ;
#22221=CARTESIAN_POINT ( 'NONE',  ( -10.81189881249999729, 6.242252689847871849, -158.4062500020483810 ) ) ;
#22223=ORIENTED_EDGE ( 'NONE', *, *, #24858, .T. ) ;
#22224=CARTESIAN_POINT ( 'NONE',  ( -10.00000000000000000, -5.773502691896251982, -20.62499999999997158 ) ) ;
#22225=ADVANCED_FACE ( 'NONE', ( #36622 ), #40067, .T. ) ;
#22226=CARTESIAN_POINT ( 'NONE',  ( 7.644554776091147741E-16, 12.48450537969573659, -28.15625000204838813 ) ) ;
#22227=CARTESIAN_POINT ( 'NONE',  ( -2.121150477449813534E-15, -11.54700538379251284, -156.8750000000000000 ) ) ;
#22229=EDGE_CURVE ( 'NONE', #26657, #39297, #9384, .T. ) ;
#22231=CARTESIAN_POINT ( 'NONE',  ( 9.999999999999998224, 0.000000000000000000, -198.5000000000000000 ) ) ;
#22232=CARTESIAN_POINT ( 'NONE',  ( -5.405949406250003975, -9.363379034771801557, -126.5312500020483952 ) ) ;
#22233=ORIENTED_EDGE ( 'NONE', *, *, #41110, .F. ) ;
#22234=CARTESIAN_POINT ( 'NONE',  ( -10.00000000000025580, 5.773502691896109873, -117.2500000040968047 ) ) ;
#22235=ORIENTED_EDGE ( 'NONE', *, *, #29704, .F. ) ;
#22236=CARTESIAN_POINT ( 'NONE',  ( 5.405949406249992428, -9.363379034771808662, -51.28125000204835970 ) ) ;
#22238=CARTESIAN_POINT ( 'NONE',  ( 10.81189881249999729, 0.000000000000000000, -106.3437500020483810 ) ) ;
#22239=EDGE_LOOP ( 'NONE', ( #35516, #8942, #7318, #21886 ) ) ;
#22240=ORIENTED_EDGE ( 'NONE', *, *, #30325, .F. ) ;
#22241=FACE_OUTER_BOUND ( 'NONE', #14622, .T. ) ;
#22243=( BOUNDED_CURVE ( )  B_SPLINE_CURVE ( 2, ( #29964, #7496, #404, #16552, #13731, #20013, #26920 ),
 .UNSPECIFIED., .F., .F. ) 
 B_SPLINE_CURVE_WITH_KNOTS ( ( 3, 2, 2, 3 ),
 ( 0.4514925373134329734, 0.4527363184079603031, 0.4539800995024877439, 0.4552238805970150737 ),
 .UNSPECIFIED. ) 
 CURVE ( )  GEOMETRIC_REPRESENTATION_ITEM ( )  RATIONAL_B_SPLINE_CURVE ( ( 0.9999999999999880096, 0.8660254037844506980, 1.000000000000000000, 0.8660254037844387076, 1.000000000000000000, 0.8660254037844207220, 1.000000000000017986 ) ) 
 REPRESENTATION_ITEM ( '' )  );
#22244=CARTESIAN_POINT ( 'NONE',  ( -5.405949406249996869, 9.363379034771805109, -156.8437500020483810 ) ) ;
#22246=CARTESIAN_POINT ( 'NONE',  ( 10.81189881249999551, -6.242252689847874514, -10.46875000204836503 ) ) ;
#22247=CARTESIAN_POINT ( 'NONE',  ( -4.999999999999996447, 8.660254037844387298, -139.5000000000000000 ) ) ;
#22249=CARTESIAN_POINT ( 'NONE',  ( 5.405949406249992428, -9.363379034771808662, -144.0937500020483810 ) ) ;
#22251=CARTESIAN_POINT ( 'NONE',  ( -7.071067811865472841, -7.071067811865472841, -200.0000000000000000 ) ) ;
#22253=CARTESIAN_POINT ( 'NONE',  ( -5.000000000000003553, -8.660254037844383745, -197.8750000040967905 ) ) ;
#22255=CARTESIAN_POINT ( 'NONE',  ( -10.81189881249999729, 1.324075727343319199E-15, -194.2812500020484094 ) ) ;
#22259=VECTOR ( 'NONE', #34917, 1000.000000000000114 ) ;
#22260=CARTESIAN_POINT ( 'NONE',  ( 5.405949406249992428, -9.363379034771808662, -72.09375000204836681 ) ) ;
#22261=CARTESIAN_POINT ( 'NONE',  ( -5.405949406249996869, 9.363379034771805109, -53.34375000204835970 ) ) ;
#22263=CARTESIAN_POINT ( 'NONE',  ( -5.405949406250003975, -9.363379034771801557, -24.53125000204836681 ) ) ;
#22267=CARTESIAN_POINT ( 'NONE',  ( 4.999999999999992006, -8.660254037844389075, -114.7499999999999858 ) ) ;
#22271=CARTESIAN_POINT ( 'NONE',  ( -2.293366432827344421E-15, -12.48450537969573659, -7.906250002048370362 ) ) ;
#22272=VERTEX_POINT ( 'NONE', #29953 ) ;
#22273=LINE ( 'NONE', #32000, #12079 ) ;
#22275=CARTESIAN_POINT ( 'NONE',  ( 9.999999999999998224, 0.000000000000000000, -38.37500000409676915 ) ) ;
#22277=CARTESIAN_POINT ( 'NONE',  ( 4.999999999999992006, -8.660254037844389075, -42.74999999999998579 ) ) ;
#22278=CARTESIAN_POINT ( 'NONE',  ( 9.999999999999998224, 0.000000000000000000, -23.37500000409675849 ) ) ;
#22279=EDGE_CURVE ( 'NONE', #21961, #36222, #4459, .T. ) ;
#22280=CARTESIAN_POINT ( 'NONE',  ( 10.81189881249999729, 6.242252689847867408, -52.40625000204838813 ) ) ;
#22281=CARTESIAN_POINT ( 'NONE',  ( -9.999999999999998224, 1.224646799147353059E-15, -121.2500000000000000 ) ) ;
#22284=CYLINDRICAL_SURFACE ( 'NONE', #749, 9.999999999999998224 ) ;
#22285=CARTESIAN_POINT ( 'NONE',  ( 5.405949406249999534, 9.363379034771803333, -148.2812500020483810 ) ) ;
#22286=ADVANCED_FACE ( 'NONE', ( #21067 ), #37476, .T. ) ;
#22287=CARTESIAN_POINT ( 'NONE',  ( -10.81189881249999729, 1.324075727343319199E-15, -150.7812500020483810 ) ) ;
#22289=DIRECTION ( 'NONE',  ( -0.000000000000000000, -0.000000000000000000, 1.000000000000000000 ) ) ;
#22290=ORIENTED_EDGE ( 'NONE', *, *, #3804, .T. ) ;
#22292=EDGE_LOOP ( 'NONE', ( #29553, #31699, #5302, #38878, #32600, #35955 ) ) ;
#22293=EDGE_CURVE ( 'NONE', #10615, #3056, #31444, .T. ) ;
#22295=CARTESIAN_POINT ( 'NONE',  ( 5.405949406249999534, 9.363379034771803333, -184.0937500020483810 ) ) ;
#22296=CARTESIAN_POINT ( 'NONE',  ( -10.81189881249999729, 6.242252689847871849, -32.21875000204835970 ) ) ;
#22297=CARTESIAN_POINT ( 'NONE',  ( -9.999999999998969713, -5.773502691896847949, -41.62499999999995737 ) ) ;
#22298=CARTESIAN_POINT ( 'NONE',  ( 10.81189881249999729, 0.000000000000000000, -161.8437500020484094 ) ) ;
#22299=CARTESIAN_POINT ( 'NONE',  ( 10.81189881249999729, 0.000000000000000000, -151.3437500020483810 ) ) ;
#22300=DIRECTION ( 'NONE',  ( 1.000000000000000000, 0.000000000000000000, 0.000000000000000000 ) ) ;
#22303=CARTESIAN_POINT ( 'NONE',  ( 7.644554776091147741E-16, 12.48450537969573659, -20.46875000204836326 ) ) ;
#22307=CARTESIAN_POINT ( 'NONE',  ( -10.81189881249999729, 6.242252689847871849, -83.21875000204838102 ) ) ;
#22309=CARTESIAN_POINT ( 'NONE',  ( -10.81189881249999729, 1.324075727343319199E-15, -47.28125000204838813 ) ) ;
#22311=CARTESIAN_POINT ( 'NONE',  ( -9.999999999999998224, 1.224646799147353059E-15, -77.74999999999998579 ) ) ;
#22313=CARTESIAN_POINT ( 'NONE',  ( 5.000000000000000000, 8.660254037844385522, -136.7499999999999716 ) ) ;
#22314=CARTESIAN_POINT ( 'NONE',  ( 5.405949406249992428, -9.363379034771808662, -142.7812500020483810 ) ) ;
#22315=CARTESIAN_POINT ( 'NONE',  ( 0.000000000000000000, 0.000000000000000000, -200.0000000000000000 ) ) ;
#22317=CARTESIAN_POINT ( 'NONE',  ( 5.000000000000000000, 8.660254037844385522, -120.6250000040967905 ) ) ;
#22319=EDGE_LOOP ( 'NONE', ( #7956, #11921, #25586, #38050 ) ) ;
#22323=CARTESIAN_POINT ( 'NONE',  ( -5.405949406249996869, 9.363379034771805109, -170.5312500020484094 ) ) ;
#22324=CARTESIAN_POINT ( 'NONE',  ( 4.999999999999992006, -8.660254037844389075, -53.62500000409675494 ) ) ;
#22327=CARTESIAN_POINT ( 'NONE',  ( 4.999999999999992006, -8.660254037844389075, -134.6250000040967620 ) ) ;
#22328=CARTESIAN_POINT ( 'NONE',  ( -10.81189881249999907, -6.242252689847864744, -171.6562500020484094 ) ) ;
#22329=CARTESIAN_POINT ( 'NONE',  ( 9.999999999999678479, 5.773502691896442940, -183.7500000040967905 ) ) ;
#22330=CARTESIAN_POINT ( 'NONE',  ( -10.00000000000102496, 5.773502691895664007, -64.37499999999994316 ) ) ;
#22331=VERTEX_POINT ( 'NONE', #31017 ) ;
#22332=CARTESIAN_POINT ( 'NONE',  ( 9.999999999999998224, 0.000000000000000000, -105.4999999999999858 ) ) ;
#22334=ADVANCED_FACE ( 'NONE', ( #1879 ), #34258, .T. ) ;
#22335=CARTESIAN_POINT ( 'NONE',  ( -2.293366432827344421E-15, -12.48450537969573659, -79.90625000204839523 ) ) ;
#22336=ORIENTED_EDGE ( 'NONE', *, *, #24629, .F. ) ;
#22339=ORIENTED_EDGE ( 'NONE', *, *, #6671, .F. ) ;
#22340=VERTEX_POINT ( 'NONE', #31660 ) ;
#22341=CARTESIAN_POINT ( 'NONE',  ( -5.405949406250003975, -9.363379034771801557, -28.84375000204836326 ) ) ;
#22342=CARTESIAN_POINT ( 'NONE',  ( 9.999999999999998224, 0.000000000000000000, -170.3750000040968189 ) ) ;
#22343=CARTESIAN_POINT ( 'NONE',  ( -10.81189881249999729, 1.324075727343319199E-15, -9.781250002048352599 ) ) ;
#22344=CARTESIAN_POINT ( 'NONE',  ( 7.644554776091147741E-16, 12.48450537969573659, -53.46875000204837391 ) ) ;
#22348=CARTESIAN_POINT ( 'NONE',  ( 10.81189881249999551, -6.242252689847874514, -185.9687500020484094 ) ) ;
#22349=CARTESIAN_POINT ( 'NONE',  ( 7.644554776091147741E-16, 12.48450537969573659, -179.4687500020483810 ) ) ;
#22352=CARTESIAN_POINT ( 'NONE',  ( 7.070501591499376803E-16, 11.54700538379251284, -41.00000000409676204 ) ) ;
#22353=DIRECTION ( 'NONE',  ( 1.000000000000000000, 0.000000000000000000, 0.000000000000000000 ) ) ;
#22355=CARTESIAN_POINT ( 'NONE',  ( 5.405949406249992428, -9.363379034771808662, -103.5937500020483668 ) ) ;
#22356=CARTESIAN_POINT ( 'NONE',  ( 10.00000000000102318, -5.773502691895667560, -84.62499999999995737 ) ) ;
#22357=CARTESIAN_POINT ( 'NONE',  ( -5.405949406250003975, -9.363379034771801557, -72.53125000204838102 ) ) ;
#22358=CARTESIAN_POINT ( 'NONE',  ( 7.644554776091147741E-16, 12.48450537969573659, -80.46875000204838102 ) ) ;
#22360=CARTESIAN_POINT ( 'NONE',  ( 4.999999999999992006, -8.660254037844389075, -149.6250000040967905 ) ) ;
#22362=ORIENTED_EDGE ( 'NONE', *, *, #15152, .F. ) ;
#22365=CARTESIAN_POINT ( 'NONE',  ( -10.81189881249999729, 1.324075727343319199E-15, -194.2812500020484094 ) ) ;
#22368=CARTESIAN_POINT ( 'NONE',  ( 9.999999999999996447, -5.773502691896262640, -65.12499999999998579 ) ) ;
#22370=CARTESIAN_POINT ( 'NONE',  ( 4.999999999999992006, -8.660254037844389075, -73.12500000409677625 ) ) ;
#22372=PLANE ( 'NONE',  #33751 ) ;
#22374=CARTESIAN_POINT ( 'NONE',  ( -2.293366432827344421E-15, -12.48450537969573659, -64.90625000204838102 ) ) ;
#22379=CARTESIAN_POINT ( 'NONE',  ( -9.999999999999998224, 1.224646799147353059E-15, -0.1250000040967647053 ) ) ;
#22380=CARTESIAN_POINT ( 'NONE',  ( -10.81189881249999907, -6.242252689847864744, -192.6562500020484094 ) ) ;
#22382=CARTESIAN_POINT ( 'NONE',  ( -10.81189881249999729, -6.242252689847864744, -1.968750002048357262 ) ) ;
#22384=CARTESIAN_POINT ( 'NONE',  ( -5.000000000000003553, -8.660254037844383745, -107.8750000040967763 ) ) ;
#22385=( BOUNDED_CURVE ( )  B_SPLINE_CURVE ( 2, ( #42284, #7108, #32392, #2816, #15948, #29351, #29144 ),
 .UNSPECIFIED., .F., .F. ) 
 B_SPLINE_CURVE_WITH_KNOTS ( ( 3, 2, 2, 3 ),
 ( 0.8283582089552240513, 0.8296019900497514366, 0.8308457711442787108, 0.8320895522388060961 ),
 .UNSPECIFIED. ) 
 CURVE ( )  GEOMETRIC_REPRESENTATION_ITEM ( )  RATIONAL_B_SPLINE_CURVE ( ( 0.9999999999999761302, 0.8660254037844625774, 1.000000000000000000, 0.8660254037844387076, 1.000000000000000000, 0.8660254037844267172, 1.000000000000011990 ) ) 
 REPRESENTATION_ITEM ( '' )  );
#22386=CARTESIAN_POINT ( 'NONE',  ( -10.00000000000000000, -5.773502691896251982, -173.6249999999999716 ) ) ;
#22387=CARTESIAN_POINT ( 'NONE',  ( 7.070501591499376803E-16, 11.54700538379251284, -166.6250000000000000 ) ) ;
#22388=CARTESIAN_POINT ( 'NONE',  ( -10.81189881249999907, -6.242252689847864744, -102.6562500020483952 ) ) ;
#22389=VERTEX_POINT ( 'NONE', #35107 ) ;
#22390=CARTESIAN_POINT ( 'NONE',  ( 7.070501591499376803E-16, 11.54700538379251284, -37.62499999999995737 ) ) ;
#22392=ORIENTED_EDGE ( 'NONE', *, *, #8605, .F. ) ;
#22393=VECTOR ( 'NONE', #2951, 1000.000000000000000 ) ;
#22394=CARTESIAN_POINT ( 'NONE',  ( -10.81189881249999907, -6.242252689847864744, -26.15625000204837391 ) ) ;
#22396=CARTESIAN_POINT ( 'NONE',  ( 5.405949406249999534, 9.363379034771803333, -77.59375000204838102 ) ) ;
#22398=ADVANCED_FACE ( 'NONE', ( #41559 ), #7920, .T. ) ;
#22400=CARTESIAN_POINT ( 'NONE',  ( 5.000000000000000000, 8.660254037844385522, -30.62500000409676559 ) ) ;
#22402=CARTESIAN_POINT ( 'NONE',  ( 9.999999999999998224, 0.000000000000000000, -14.37500000409674961 ) ) ;
#22403=CARTESIAN_POINT ( 'NONE',  ( -9.999999999999998224, 1.224646799147353059E-15, -125.7499999999999716 ) ) ;
#22404=CARTESIAN_POINT ( 'NONE',  ( 5.405949406249999534, 9.363379034771803333, -130.0937500020483810 ) ) ;
#22405=CARTESIAN_POINT ( 'NONE',  ( -10.81189881249999729, 1.324075727343319199E-15, -96.78125000204839523 ) ) ;
#22406=CARTESIAN_POINT ( 'NONE',  ( 7.644554776091147741E-16, 12.48450537969573659, -119.4687500020483668 ) ) ;
#22409=CARTESIAN_POINT ( 'NONE',  ( 10.00000000000000000, 5.773502691896255534, -168.7500000040967905 ) ) ;
#22410=LINE ( 'NONE', #29526, #14399 ) ;
#22413=CARTESIAN_POINT ( 'NONE',  ( -10.81189881249999729, 1.324075727343319199E-15, -47.09375000204838102 ) ) ;
#22415=CARTESIAN_POINT ( 'NONE',  ( -5.405949406250003975, -9.363379034771801557, -0.5312500020483723606 ) ) ;
#22417=CARTESIAN_POINT ( 'NONE',  ( 5.000000000000000000, 8.660254037844385522, -6.249999999999977796 ) ) ;
#22419=CARTESIAN_POINT ( 'NONE',  ( -4.999999999999996447, 8.660254037844387298, -91.49999999999998579 ) ) ;
#22421=CARTESIAN_POINT ( 'NONE',  ( -10.00000000000000000, -5.773502691896251982, -100.5000000040967905 ) ) ;
#22422=CARTESIAN_POINT ( 'NONE',  ( -4.999999999999996447, 8.660254037844387298, -150.3750000040967905 ) ) ;
#22424=CARTESIAN_POINT ( 'NONE',  ( -10.81189881249999729, 6.242252689847871849, -89.40625000204838102 ) ) ;
#22427=CARTESIAN_POINT ( 'NONE',  ( 5.000000000000000000, 8.660254037844385522, -29.12500000409676204 ) ) ;
#22429=EDGE_LOOP ( 'NONE', ( #33484, #726, #20407, #32789 ) ) ;
#22430=CARTESIAN_POINT ( 'NONE',  ( 10.00000000000000000, 5.773502691896255534, -15.37499999999997691 ) ) ;
#22431=CARTESIAN_POINT ( 'NONE',  ( 7.644554776091147741E-16, 12.48450537969573659, -23.65625000204837747 ) ) ;
#22432=CARTESIAN_POINT ( 'NONE',  ( 7.070501591499377789E-16, 11.54700538379251284, -156.1250000000000000 ) ) ;
#22434=CARTESIAN_POINT ( 'NONE',  ( 4.999999999999992006, -8.660254037844389075, -197.2500000000000000 ) ) ;
#22435=CARTESIAN_POINT ( 'NONE',  ( -2.293366432827344421E-15, -12.48450537969573659, -123.4062500020484094 ) ) ;
#22439=EDGE_LOOP ( 'NONE', ( #34280, #8446, #20559, #24155 ) ) ;
#22440=CARTESIAN_POINT ( 'NONE',  ( 5.405949406249999534, 9.363379034771803333, -50.78125000204835970 ) ) ;
#22442=CARTESIAN_POINT ( 'NONE',  ( -2.293366432827344421E-15, -12.48450537969573659, -100.7187500020483952 ) ) ;
#22443=EDGE_LOOP ( 'NONE', ( #42264, #39564, #14504, #20562 ) ) ;
#22447=DIRECTION ( 'NONE',  ( 1.000000000000000000, 0.000000000000000000, 0.000000000000000000 ) ) ;
#22448=CARTESIAN_POINT ( 'NONE',  ( -2.121150477449813534E-15, -11.54700538379251284, -197.7500000040967905 ) ) ;
#22449=CARTESIAN_POINT ( 'NONE',  ( -10.81189881249999907, -6.242252689847864744, -150.4687500020484094 ) ) ;
#22451=CARTESIAN_POINT ( 'NONE',  ( -2.293366432827344421E-15, -12.48450537969573659, -6.218750002048345493 ) ) ;
#22454=CARTESIAN_POINT ( 'NONE',  ( -5.405949406250003975, -9.363379034771801557, -138.3437500020484094 ) ) ;
#22456=CARTESIAN_POINT ( 'NONE',  ( 9.999999999999998224, 0.000000000000000000, -200.0000000000000000 ) ) ;
#22458=CARTESIAN_POINT ( 'NONE',  ( 4.999999999999992006, -8.660254037844389075, -190.1250000040967905 ) ) ;
#22460=CARTESIAN_POINT ( 'NONE',  ( -5.405949406250003975, -9.363379034771801557, -186.5312500020484094 ) ) ;
#22461=CARTESIAN_POINT ( 'NONE',  ( 4.999999999999992006, -8.660254037844389075, -95.24999999999998579 ) ) ;
#22464=CARTESIAN_POINT ( 'NONE',  ( 5.405949406249992428, -9.363379034771808662, -66.09375000204836681 ) ) ;
#22465=CARTESIAN_POINT ( 'NONE',  ( 5.405949406249992428, -9.363379034771808662, -52.59375000204835260 ) ) ;
#22467=CARTESIAN_POINT ( 'NONE',  ( 5.405949406249992428, -9.363379034771808662, -25.78125000204836681 ) ) ;
#22471=CARTESIAN_POINT ( 'NONE',  ( -2.121150477449813534E-15, -11.54700538379251284, -111.8749999999999858 ) ) ;
#22472=CARTESIAN_POINT ( 'NONE',  ( 0.000000000000000000, 0.000000000000000000, -200.0000000000000000 ) ) ;
#22476=CARTESIAN_POINT ( 'NONE',  ( 10.81189881249999729, 0.000000000000000000, -114.0312500020483952 ) ) ;
#22478=CARTESIAN_POINT ( 'NONE',  ( -10.00000000000012790, -5.773502691896177375, -176.6250000000000284 ) ) ;
#22482=CARTESIAN_POINT ( 'NONE',  ( -2.121150477449813534E-15, -11.54700538379251284, -41.37499999999997158 ) ) ;
#22483=CARTESIAN_POINT ( 'NONE',  ( -10.00000000000000000, -5.773502691896251982, -28.50000000409675138 ) ) ;
#22484=CARTESIAN_POINT ( 'NONE',  ( 10.81189881249999729, 6.242252689847867408, -46.40625000204835970 ) ) ;
#22485=VECTOR ( 'NONE', #39058, 1000.000000000000114 ) ;
#22486=CARTESIAN_POINT ( 'NONE',  ( 9.999999999999998224, 0.000000000000000000, -141.5000000000000000 ) ) ;
#22489=CARTESIAN_POINT ( 'NONE',  ( 7.070501591499376803E-16, 11.54700538379251284, -156.5000000040968189 ) ) ;
#22490=CARTESIAN_POINT ( 'NONE',  ( -5.405949406249996869, 9.363379034771805109, -137.5312500020484094 ) ) ;
#22491=CARTESIAN_POINT ( 'NONE',  ( -10.81189881249999907, -6.242252689847864744, -150.6562500020484094 ) ) ;
#22493=DIRECTION ( 'NONE',  ( 0.000000000000000000, 1.000000000000000000, 0.000000000000000000 ) ) ;
#22494=VERTEX_POINT ( 'NONE', #4671 ) ;
#22495=( BOUNDED_CURVE ( )  B_SPLINE_CURVE ( 2, ( #20065, #7774, #29804, #24180, #37327, #20917, #3466 ),
 .UNSPECIFIED., .F., .F. ) 
 B_SPLINE_CURVE_WITH_KNOTS ( ( 3, 2, 2, 3 ),
 ( 0.2686567164179105571, 0.2699004975124379424, 0.2711442786069652722, 0.2723880597014926574 ),
 .UNSPECIFIED. ) 
 CURVE ( )  GEOMETRIC_REPRESENTATION_ITEM ( )  RATIONAL_B_SPLINE_CURVE ( ( 0.9999999999999880096, 0.8660254037844506980, 1.000000000000000000, 0.8660254037844387076, 1.000000000000000000, 0.8660254037844267172, 1.000000000000011990 ) ) 
 REPRESENTATION_ITEM ( '' )  );
#22497=EDGE_LOOP ( 'NONE', ( #6562, #42012, #2076, #30402 ) ) ;
#22498=AXIS2_PLACEMENT_3D ( 'NONE', #21926, #24978, #11349 ) ;
#22499=CYLINDRICAL_SURFACE ( 'NONE', #28401, 9.999999999999998224 ) ;
#22500=CARTESIAN_POINT ( 'NONE',  ( -5.405949406250003975, -9.363379034771801557, -177.3437500020483810 ) ) ;
#22501=CARTESIAN_POINT ( 'NONE',  ( -2.293366432827344421E-15, -12.48450537969573659, -31.71875000204834905 ) ) ;
#22503=ADVANCED_FACE ( 'NONE', ( #18040 ), #31236, .T. ) ;
#22504=CARTESIAN_POINT ( 'NONE',  ( -10.81189881249999729, 6.242252689847871849, -164.2187500020483810 ) ) ;
#22505=CARTESIAN_POINT ( 'NONE',  ( -10.81189881249999729, 6.242252689847871849, -146.2187500020483810 ) ) ;
#22510=CARTESIAN_POINT ( 'NONE',  ( 5.405949406249999534, 9.363379034771803333, -19.09375000204835260 ) ) ;
#22514=DIRECTION ( 'NONE',  ( -0.000000000000000000, -0.000000000000000000, 1.000000000000000000 ) ) ;
#22516=CARTESIAN_POINT ( 'NONE',  ( 10.81189881249999551, -6.242252689847874514, -76.46875000204838102 ) ) ;
#22517=CARTESIAN_POINT ( 'NONE',  ( 5.405949406249992428, -9.363379034771808662, -54.28125000204836681 ) ) ;
#22521=CARTESIAN_POINT ( 'NONE',  ( -4.999999999999996447, 8.660254037844387298, -136.5000000000000000 ) ) ;
#22522=CARTESIAN_POINT ( 'NONE',  ( 5.405949406249999534, 9.363379034771803333, -149.7812500020483810 ) ) ;
#22524=CARTESIAN_POINT ( 'NONE',  ( 7.070501591499376803E-16, 11.54700538379251284, -15.50000000409676915 ) ) ;
#22525=CARTESIAN_POINT ( 'NONE',  ( -5.000000000000003553, -8.660254037844383745, -122.8750000040967905 ) ) ;
#22527=ORIENTED_EDGE ( 'NONE', *, *, #18315, .T. ) ;
#22530=CARTESIAN_POINT ( 'NONE',  ( 9.999999999999998224, 0.000000000000000000, -52.99999999999996447 ) ) ;
#22531=CARTESIAN_POINT ( 'NONE',  ( -10.81189881249999729, 6.242252689847871849, -174.9062500020483810 ) ) ;
#22532=CARTESIAN_POINT ( 'NONE',  ( 9.999999999999996447, -5.773502691896262640, -49.00000000409676915 ) ) ;
#22535=CARTESIAN_POINT ( 'NONE',  ( -9.999999999999998224, 1.224646799147353059E-15, -44.74999999999998579 ) ) ;
#22536=CARTESIAN_POINT ( 'NONE',  ( 10.81189881249999551, -6.242252689847874514, -169.6562500020484094 ) ) ;
#22538=CARTESIAN_POINT ( 'NONE',  ( -10.81189881249999907, -6.242252689847864744, -141.4687500020484094 ) ) ;
#22539=CARTESIAN_POINT ( 'NONE',  ( 0.000000000000000000, 0.000000000000000000, -200.0000000000000000 ) ) ;
#22540=CARTESIAN_POINT ( 'NONE',  ( 5.000000000000000000, 8.660254037844385522, -80.12500000409677625 ) ) ;
#22541=EDGE_LOOP ( 'NONE', ( #9198, #28882, #15940, #41991 ) ) ;
#22543=CARTESIAN_POINT ( 'NONE',  ( 10.81189881249999551, -6.242252689847874514, -72.15625000204836681 ) ) ;
#22544=ORIENTED_EDGE ( 'NONE', *, *, #12569, .F. ) ;
#22546=ORIENTED_EDGE ( 'NONE', *, *, #26483, .F. ) ;
#22547=EDGE_CURVE ( 'NONE', #5178, #21158, #41116, .T. ) ;
#22549=CARTESIAN_POINT ( 'NONE',  ( 5.405949406249992428, -9.363379034771808662, -30.09375000204836326 ) ) ;
#22551=CARTESIAN_POINT ( 'NONE',  ( 5.405949406249999534, 9.363379034771803333, -2.781250002048374359 ) ) ;
#22552=CARTESIAN_POINT ( 'NONE',  ( 5.405949406249992428, -9.363379034771808662, -58.59375000204835970 ) ) ;
#22555=CARTESIAN_POINT ( 'NONE',  ( 5.405949406249999534, 9.363379034771803333, -188.5937500020483810 ) ) ;
#22556=CARTESIAN_POINT ( 'NONE',  ( -5.405949406250003975, -9.363379034771801557, -169.8437500020484094 ) ) ;
#22559=LINE ( 'NONE', #25183, #19822 ) ;
#22562=CARTESIAN_POINT ( 'NONE',  ( 10.81189881249999551, -6.242252689847874514, -104.9687500020483810 ) ) ;
#22563=CARTESIAN_POINT ( 'NONE',  ( 10.00000000000102318, -5.773502691895667560, -47.50000000409674783 ) ) ;
#22564=CARTESIAN_POINT ( 'NONE',  ( -5.405949406249996869, 9.363379034771805109, -74.53125000204838102 ) ) ;
#22566=CARTESIAN_POINT ( 'NONE',  ( 10.81189881249999551, -6.242252689847874514, -83.96875000204838102 ) ) ;
#22568=CARTESIAN_POINT ( 'NONE',  ( 5.000000000000000000, 8.660254037844385522, -143.1250000040967905 ) ) ;
#22570=ORIENTED_EDGE ( 'NONE', *, *, #23848, .T. ) ;
#22573=EDGE_CURVE ( 'NONE', #5984, #26792, #27769, .T. ) ;
#22574=CARTESIAN_POINT ( 'NONE',  ( 5.405949406249992428, -9.363379034771808662, -193.7812500020484094 ) ) ;
#22577=VECTOR ( 'NONE', #1549, 1000.000000000000000 ) ;
#22579=CARTESIAN_POINT ( 'NONE',  ( -2.121150477449813534E-15, -11.54700538379251284, -56.37499999999997868 ) ) ;
#22581=CARTESIAN_POINT ( 'NONE',  ( 10.00000000000000000, 5.773502691896255534, -75.75000000409679046 ) ) ;
#22583=( BOUNDED_CURVE ( )  B_SPLINE_CURVE ( 2, ( #16621, #29825, #23127, #22489, #25946, #35664, #39095 ),
 .UNSPECIFIED., .F., .F. ) 
 B_SPLINE_CURVE_WITH_KNOTS ( ( 3, 2, 2, 3 ),
 ( 0.2089552238805970630, 0.2101990049751244205, 0.2114427860696518058, 0.2126865671641791633 ),
 .UNSPECIFIED. ) 
 CURVE ( )  GEOMETRIC_REPRESENTATION_ITEM ( )  RATIONAL_B_SPLINE_CURVE ( ( 0.9999999999999940048, 0.8660254037844447028, 1.000000000000000000, 0.8660254037844387076, 1.000000000000000000, 0.8660254037844327124, 1.000000000000005995 ) ) 
 REPRESENTATION_ITEM ( '' )  );
#22584=CARTESIAN_POINT ( 'NONE',  ( 9.999999999998456346, 5.773502691897149042, -12.75000000409671941 ) ) ;
#22586=CARTESIAN_POINT ( 'NONE',  ( 7.644554776091147741E-16, 12.48450537969573659, -70.15625000204839523 ) ) ;
#22590=CARTESIAN_POINT ( 'NONE',  ( -2.293366432827344421E-15, -12.48450537969573659, -193.9062500020484094 ) ) ;
#22592=CARTESIAN_POINT ( 'NONE',  ( 5.405949406249992428, -9.363379034771808662, -3.093750002048367698 ) ) ;
#22595=CARTESIAN_POINT ( 'NONE',  ( -9.999999999999998224, 1.224646799147353059E-15, -173.7500000000000284 ) ) ;
#22596=CARTESIAN_POINT ( 'NONE',  ( 9.999999999999998224, 0.000000000000000000, -171.5000000000000000 ) ) ;
#22597=CARTESIAN_POINT ( 'NONE',  ( 7.070501591499376803E-16, 11.54700538379251284, -97.62499999999997158 ) ) ;
#22598=CARTESIAN_POINT ( 'NONE',  ( -10.81189881249999729, 6.242252689847871849, -98.40625000204838102 ) ) ;
#22599=ORIENTED_EDGE ( 'NONE', *, *, #10123, .T. ) ;
#22600=CARTESIAN_POINT ( 'NONE',  ( -9.999999999999998224, 1.224646799147353059E-15, -200.0000000000000000 ) ) ;
#22602=VERTEX_POINT ( 'NONE', #37909 ) ;
#22604=CARTESIAN_POINT ( 'NONE',  ( -5.405949406250003975, -9.363379034771801557, -37.84375000204837391 ) ) ;
#22605=CARTESIAN_POINT ( 'NONE',  ( -10.81189881249999729, 6.242252689847871849, -30.90625000204834905 ) ) ;
#22607=CARTESIAN_POINT ( 'NONE',  ( 7.644554776091147741E-16, 12.48450537969573659, -81.96875000204839523 ) ) ;
#22610=VECTOR ( 'NONE', #39738, 1000.000000000000000 ) ;
#22611=CARTESIAN_POINT ( 'NONE',  ( 10.81189881249999729, 0.000000000000000000, -197.8437500020484094 ) ) ;
#22613=CARTESIAN_POINT ( 'NONE',  ( -11.54700538379250396, -20.00000000000000355, 0.000000000000000000 ) ) ;
#22614=CARTESIAN_POINT ( 'NONE',  ( 7.070501591499376803E-16, 11.54700538379251284, -49.62499999999997868 ) ) ;
#22616=CARTESIAN_POINT ( 'NONE',  ( -10.00000000000000000, -5.773502691896251982, -9.000000004096754935 ) ) ;
#22617=CARTESIAN_POINT ( 'NONE',  ( 9.999999999999998224, 0.000000000000000000, -99.87500000409679046 ) ) ;
#22618=CARTESIAN_POINT ( 'NONE',  ( 5.405949406249999534, 9.363379034771803333, -125.5937500020483668 ) ) ;
#22619=CARTESIAN_POINT ( 'NONE',  ( 10.81189881249999729, 0.000000000000000000, -94.53125000204838102 ) ) ;
#22620=CARTESIAN_POINT ( 'NONE',  ( 7.644554776091147741E-16, 12.48450537969573659, -108.9687500020483668 ) ) ;
#22623=CARTESIAN_POINT ( 'NONE',  ( 7.070501591499377789E-16, 11.54700538379251284, -167.0000000040967905 ) ) ;
#22625=CARTESIAN_POINT ( 'NONE',  ( 9.999999999999998224, 0.000000000000000000, -66.49999999999997158 ) ) ;
#22630=DIRECTION ( 'NONE',  ( -0.7559289460184526188, -8.392497208503125347E-17, 0.6546536707079791961 ) ) ;
#22632=CARTESIAN_POINT ( 'NONE',  ( -2.121150477449813534E-15, -11.54700538379251284, -59.75000000409676915 ) ) ;
#22634=CARTESIAN_POINT ( 'NONE',  ( -2.121150477449813534E-15, -11.54700538379251284, -87.87499999999997158 ) ) ;
#22636=CARTESIAN_POINT ( 'NONE',  ( 5.000000000000000000, 8.660254037844385522, -95.12500000409677625 ) ) ;
#22639=CARTESIAN_POINT ( 'NONE',  ( -2.293366432827344421E-15, -12.48450537969573659, -90.40625000204838102 ) ) ;
#22640=ORIENTED_EDGE ( 'NONE', *, *, #22059, .F. ) ;
#22641=( BOUNDED_SURFACE ( )  B_SPLINE_SURFACE ( 1, 2, ( 
 ( #32590, #19607, #15312, #25480, #18982, #5619, #22017, #16138, #29338, #12906, #18770, #36027, #22231, #15515, #38414, #28720, #35403, #26102, #38626, #5828, #39256, #32169, #22434, #42063, #9689, #22865, #6465, #42269, #32787, #28508, #41639, #2804, #12074, #12493, #25269, #8858, #25685, #38838, #35613, #6041, #19191, #32380, #15936, #16781, #39466, #40097, #424, #10318, #36865, #10108, #29982, #13117, #17208, #13546, #26730, #33226, #9900, #36234, #10529, #39736, #20670, #26940, #23504, #7307, #13749, #23712, #20457, #16349, #39883, #23284, #13333, #16999, #26316, #33645, #29770, #23932, #36654, #23076, #7519, #30198, #6666, #36446, #26523, #33437, #19817, #214, #16570, #3655, #20248, #634, #4068, #30410, #33005, #842, #7096, #3226, #27157, #6880, #3863, #29549, #10741, #13962, #20032, #3434, #40298, #37076, #39672, #30828, #34717, #31269, #4280, #8167, #34504, #11378, #40508, #37941, #14390, #24576, #40935, #11168, #18074, #1696, #4924, #27587, #37724, #37507, #14822, #17634, #28020, #28236, #14615, #18289, #21315, #1048, #17851, #27804, #31048, #15039, #21537, #37290, #40726, #21100, #31476, #4701, #34070, #1909, #41150, #11588, #4491, #24795, #8386, #5141, #14172, #24150, #41371, #1266, #10953, #11807, #25010, #27373, #1479, #24365, #38152, #7736, #8595, #20883, #33856, #17422, #30619, #7950, #34287, #38995, #12859, #18933, #35564, #22179, #32328, #5564, #29285, #15880, #2337, #12648, #31910, #26053, #21958, #19349, #25839, #39204, #19142, #32536, #25219, #9431, #42430, #12024, #35350, #28876, #42009, #35138, #15466, #21750, #38363, #29082, #18716, #5779, #2754, #5992, #28667, #9217, #12233, #12438, #28458, #22386, #25425, #2964, #16091, #38568, #8801, #42219, #41796, #9011, #2548, #15258, #25633, #32117, #34928, #15675, #31693, #5349, #22596, #2126, #38791, #35773, #6203, #18504, #41591, #42640, #6616, #26469, #23234, #39618, #36394, #16302, #6825, #3381, #13492, #19981, #29716, #33170, #6413, #3176, #3602, #39414, #29929, #16517, #16731, #370, #29498, #26680, #19553, #160, #23450, #13067, #10055, #32738, #26263, #39832, #9640, #10265, #9848, #22813, #23025, #35976, #36177, #19768, #32951, #13282, #4753, #4975, #11859, #7568, #17682, #11218, #40560, #14224, #18121, #31316, #1748, #27425, #28285, #14445, #11004, #30669, #24198, #1312, #14875, #34119, #37347, #41199, #4540, #1531, #7794, #21587, #28072, #8434, #34549, #11639, #37990, #25057, #37773, #1959, #34335, #33912, #24843, #20936, #30878, #34766, #5187, #4332, #31531, #27637, #21149, #1097, #18341, #17900, #14664, #15088, #40777, #31098, #17471, #41422, #27853, #40987, #37558, #24418, #7997, #20721, #11429, #24626, #8217, #21366, #42266, #6038, #32377, #12692, #8644, #22227, #2385, #5613, #9264, #18556, #25888, #22432, #19187, #12072, #2801, #35401, #19395, #29131, #2595, #15930, #31746, #41636, #39042, #31956, #22647, #32165, #9479, #35820, #25266, #6252, #2174, #5825, #12904, #38412, #35611, #15309, #18767, #32587, #38200, #3012, #28506, #16136, #22013, #29335, #18980, #8853, #15512, #42476, #15724, #21799, #34979, #5405, #28717, #41843, #35186, #12281, #25477, #38623, #9059, #28923, #42059, #12488, #25682, #38835, #29546, #19814, #23501, #9897, #41804, #16996, #23072, #20029, #16347, #40093, #3860, #26936, #10315, #30193, #13746, #837, #13541, #20453, #10104, #9687, #629, #13114, #26313, #36650, #7094, #22861, #7303, #32785, #39668, #19604, #20244, #23281, #33220, #10525, #33001, #36441, #36024, #23709, #6877, #3651, #13330, #3223, #39463, #33433, #6462, #26100, #36860, #16778, #33641, #4062, #17204, #30405, #39251, #29978, #3430, #36229, #39879, #6663, #16567, #29764, #210, #421, #26520, #26726, #6123, #25976, #12988, #22735, #41931, #19481, #36106, #42144, #16017, #2674, #9352, #39127, #38492, #5707, #12784, #38711, #29424, #38921, #32667, #35901, #32038, #9561, #8936, #12575, #19693, #2468, #29213, #22100, #12362, #6338, #2266, #3096, #25346, #16224, #28799, #42565, #25768, #15597, #22313, #9772, #22521, #42352, #6540, #15387, #25560, #5913, #35274, #18858, #26185, #39333, #22952, #9145, #28586, #35486, #19066, #32247, #15808, #29004, #41714, #35694, #19268, #12153, #32462, #2887, #23156, #4153, #10610, #33730, #17083, #23797, #20541, #7605, #20328, #27239, #16866, #16437, #36952, #6750, #33089, #721, #30282, #29635, #14044, #39546, #3736, #26395, #27034, #30069, #39971, #7394, #39756, #511, #79, #17296, #13626, #26819, #20123, #9977, #36319, #40179, #13202, #32877, #13840, #10401, #30501, #927, #40382, #10824, #3308, #23592, #10191, #292, #3945, #19904, #24017, #16653, #37158, #36738, #3516, #29854, #13413, #33311, #26606, #7176, #23376, #36526, #6967, #33522, #8041, #37812, #18159, #34588, #1784, #37385, #14914, #17939, #2000, #11680, #4581, #31354, #15126, #1571, #5223, #8256, #30705, #4791, #14701, #31138, #28322, #8472, #24234, #1351, #21186, #18379, #34375, #20975, #31568, #5018, #27890, #34160, #21402, #41023, #38029, #1136, #11040, #21624, #17721, #40597, #41462, #34803, #14259, #11467, #30916, #41241, #7828, #24668, #27462, #28114, #24879, #11897, #25092, #14481, #38237, #20759, #33948, #4370, #17509, #27676, #40814, #11254, #24451, #37597, #42307, #18807, #12940, #8891, #6289, #12729, #26136, #6078, #19433, #12109, #25927, #16177, #41674, #9099, #15762, #28960, #22054, #31994, #8682, #25304, #15971, #35227, #22267, #19225, #35648, #5658, #38872, #41881, #42096, #15344, #9302, #12317, #32624, #3049, #25515, #38448, #29167, #2420, #15552, #32203, #2214, #12530, #21836, #29372, #28754, #22471, #35016, #42514, #39078, #38663, #31783, #25723, #2837, #5445, #35437, #9517, #32415, #18596, #22687, #35855, #28542, #5864, #19018, #2630, #30015, #3688, #16603, #23540, #36689, #10351, #19855, #16816, #246, #7129, #20283, #30232, #26973, #13994, #26768, #33678, #23324, #22905, #672, #13153, #39500, #33472, #3898, #36061, #20493, #3259, #10144, #32828, #17033, #36479, #461, #13790, #36272, #4105, #40132, #30, #33040, #26560, #36900, #6914, #9931, #7344, #10561, #33262, #23110, #39921, #13577, #23747, #19644, #29587, #17246, #6703, #16387, #30446, #877, #26347, #20067, #3468, #39288, #29806, #9722, #13368, #6495, #39707, #37975, #4959, #24182, #1733, #18325, #24401, #40970, #27621, #37756, #10987, #34751, #21349, #7776, #18106, #37329, #31514, #27407, #24829, #31301, #1944, #24607, #8419, #30652, #14859, #5171, #17455, #40761, #34321, #4738, #40543, #20919, #27190, #1082, #34535, #34101, #11203, #8200, #11413, #4524, #14649, #17667, #17884, #33894, #27838, #30861, #21570, #40334, #1297, #14208, #28056, #14428, #37542, #7982, #20706, #31082, #10776, #23965, #21133, #41182, #37109, #7553, #11622, #1515, #4316, #22211, #9250, #6239, #12056, #15917, #12472, #28271, #32151, #15710, #35387, #2370, #2581, #25667, #28909, #38821, #31729, #22419, #12266, #39030, #6025, #5811, #35597, #8628, #18538, #19175, #8839, #42254, #9046, #2788, #32364, #2159, #29118, #21784, #25462, #32573, #15293, #42046, #34964, #25252, #12679, #15069, #25876, #38184, #9465, #41622, #22634, #38607, #28490, #35173, #35807, #18964, #19383, #41407, #11841, #38397, #18752, #5387, #21995, #25042, #5598, #31942, #15496, #28702, #41829, #6448, #26087, #19590, #39450, #406, #29534, #32773, #36635, #42676, #39654, #36011, #16981, #23487, #3846, #29966, #7081, #33420, #20442, #33208, #40080, #29752, #29321, #20231, #3209, #16336, #13527, #26714, #42465, #26922, #9676, #16554, #39238, #39866, #197, #10091, #19801, #13102, #23269, #13318, #30179, #26507, #36428, #32989, #22849, #26301, #10300, #12893, #2999, #617, #6864, #13733, #10511, #23698, #36847, #16124, #20015, #9885, #23059, #16766, #36215, #7290, #6651, #3417, #3639, #825, #37922, #4686, #20868, #11362, #14374, #24557, #30392, #17405, #4264, #27785, #37707, #4049, #17616, #40490, #1032, #17835, #13946, #21297, #30603, #11571, #30811, #27139, #8368, #31030, #34052, #8149, #27571, #34485, #40282, #14155, #27355, #4474, #7933, #1462, #14595, #40919, #7499, #4907, #1250, #14805, #18054, #40706, #31249, #10723, #37060, #1677, #10936, #28001, #11149, #41131, #24777, #20651, #33627, #23916, #24348, #17193, #33838, #24129, #37271, #7720, #37489, #21083, #34271, #1891, #38773, #5331, #32098, #31893, #34909, #41573, #29065, #18697, #18915, #25823, #21518, #31674, #25201, #11789, #28219, #2531, #15656, #28856, #41352, #42203, #28437, #24991, #15020, #38133, #15239, #41992, #18486, #8576, #12421, #2108, #15450, #21726, #35545, #25615, #22368, #5762, #9199, #5975, #38978, #8992, #15864, #5545, #5119, #19126, #12006, #38342, #32311, #2734, #18268, #12629, #8784, #35121, #21941, #34699, #2321, #28648, #41778, #12212, #25405, #38551, #31457, #22160, #35335, #39395, #2948, #42413, #16716, #6185, #26874, #33152, #29697, #13472, #19966, #26036, #9622, #3582, #6811, #35757, #33371, #16076, #23009, #29269, #29911, #6596, #16499, #26246, #12844, #143, #19752, #23434, #36163, #32934, #9827, #39188, #22794, #350, #19324, #9414, #26664, #13264, #39814, #10246, #36582, #7029, #22579, #3366, #16284, #19538, #23218, #32519, #20181, #35956, #30126, #26450, #6397, #13683, #36376, #39602, #3791, #10036, #16925, #32722, #3155, #29482, #563, #42622, #13052, #11092, #21030, #13897, #34220, #37215, #21846, #30979, #4422, #4636, #33575, #771, #7882, #33786, #24502, #34001, #27732, #17782, #27090, #1408, #3998, #7662, #15354, #40233, #24295, #17141, #7446, #14538, #40029, #40868, #20384, #11309, #23862, #38248, #20815, #10668, #17352, #5455, #17562, #37439, #2227, #10459, #20599, #983, #30342, #37010, #8693, #35025, #18605, #4209, #31793, #30556, #14100, #27302, #40438, #10882, #23650, #24074, #30762, #36796, #1195, #14319, #27518, #7234, #40650, #29384, #12740, #19443, #16187, #3270, #15981, #22916, #12541, #12122, #32635, #2848, #29178, #6089, #35237, #3062, #9109, #19236, #35658, #5875, #25940, #39089, #42317, #22277, #32424, #32213, #9528, #12327, #22698, #36071, #9314, #12952, #35867, #38459, #22482, #19029, #25525, #6507, #42527, #32004, #35449, #15772, #26147, #42106, #28765, #39298, #6300, #9735, #41893, #19657, #32842, #28552, #8900, #18820, #41684, #38674, #5667, #25314, #22065, #2429, #25733, #2641, #15564, #28969, #38883, #23121, #20294, #40145, #27202, #36912, #13380, #33692, #7566, #13589, #30245, #16829, #26986, #259, #23978, #10573, #39721, #7358, #26572, #20718, #16615, #14007, #20505, #33909, #13802, #40346, #19868, #4118, #37122, #6716, #30028, #23553, #36701, #29818, #10157, #16400, #33054, #23759, #23338, #474, #17258, #685, #36490, #3911, #6927, #7141, #36286, #17045, #20080, #10789, #29600, #33274, #3480, #30461, #3700, #26782, #39934, #9942, #33485, #43, #13166, #10361, #888, #26360, #39513, #37988, #11215, #27422, #11427, #41195, #38198, #1310, #5185, #1746, #17468, #14873, #14662, #17680, #24416, #11856, #1529, #28069, #8642, #4330, #14443, #7994, #37344, #11002, #11636, #24841, #8432, #24196, #25055, #37556, #7791, #40558, #20934, #40774, #21585, #30875, #34116, #34763, #27635, #40985, #4538, #18339, #31529, #1957, #31314, #15083, #28283, #21797, #34547, #41420, #31096, #30667, #1095, #21147, #34333, #14222, #4751, #17897, #27851, #24622, #37770, #8215, #21364, #4973, #18119, #9057, #38409, #42057, #2593, #6251, #5823, #18978, #22224, #28504, #25264, #42265, #31743, #9686, #15929, #12486, #39041, #2799, #29130, #9478, #5402, #32163, #41841, #2383, #6036, #15307, #22646, #18765, #12903, #15722, #2172, #39249, #19186, #35399, #12690, #28920, #25887, #41634, #31954, #5610, #25680, #9262, #32375, #35818, #19394, #8851, #32586, #38832, #16135, #3011, #22430, #29333, #12070, #22010, #42475, #28715, #26099, #35609, #34977, #18553, #35184, #15510, #12279, #25475, #38621, #23071, #7092, #42688, #33000, #26933, #40292, #3858, #3221, #40091, #6662, #10522, #36023, #6875, #29763, #3428, #36647, #16346, #23707, #19812, #834, #20027, #32784, #27149, #20242, #10103, #627, #3650, #13743, #19603, #16566, #36227, #23280, #39878, #33431, #16993, #30191, #39462, #36858, #33219, #4060, #7301, #29977, #20451, #29545, #26312, #33638, #209, #17202, #16777, #30403, #13956, #9896, #22860, #13113, #420, #6461, #13329, #26519, #39667, #36439, #13540, #26725, #10311, #23499, #28013, #37282, #21307, #21093, #24141, #30822, #18278, #7942, #8159, #15030, #10734, #20877, #14384, #1041, #17415, #34495, #4917, #18065, #30613, #31468, #17627, #14166, #33850, #27365, #4485, #31261, #7729, #40501, #1687, #34063, #4696, #10946, #24788, #14816, #11580, #37717, #41141, #37932, #28229, #40928, #5131, #37500, #37070, #8378, #1260 ),
 ( #11371, #31041, #27581, #21528, #40718, #1473, #17845, #11159, #34710, #1901, #24568, #24358, #14607, #34281, #23926, #27797, #7512, #20662, #4274, #25833, #15668, #8588, #22171, #31903, #38355, #35767, #29075, #2119, #21952, #28660, #38988, #12225, #41584, #9424, #12431, #35345, #12016, #42003, #5773, #15873, #21740, #31685, #42213, #25212, #18497, #22590, #12640, #34920, #38562, #8794, #19136, #15249, #18926, #5342, #2542, #22380, #6195, #32321, #35133, #19339, #32529, #9003, #25627, #41790, #9209, #5556, #2958, #35557, #18709, #2747, #2332, #16085, #15461, #41363, #11800, #25003, #38784, #38145, #28449, #25417, #32110, #28869, #5985, #36388, #6821, #29493, #9841, #4008, #3168, #36592, #13062, #153, #26674, #13485, #42632, #16726, #19762, #19975, #35969, #29921, #32945, #26884, #40039, #3375, #16295, #7039, #26256, #23019, #10048, #22804, #33162, #33587, #10469, #23659, #32732, #33381, #36807, #19548, #29708, #3594, #363, #39405, #36172, #29280, #6608, #20192, #16510, #13273, #39825, #10258, #26463, #23444, #39612, #3800, #6407, #16939, #23228, #7245, #20395, #30136, #574, #13692, #42424, #12854, #26046, #39198, #9633, #21469, #41087, #37225, #4646, #17151, #24733, #8104, #24086, #40242, #24305, #11319, #8324, #14111, #18004, #14551, #30352, #34230, #17794, #37449, #23872, #21255, #40449, #7893, #21040, #7673, #1419, #27742, #30991, #10893, #40878, #20825, #24512, #993, #37665, #11530, #40662, #1634, #34443, #27100, #11102, #34012, #27314, #37880, #4862, #20610, #4433, #17572, #14762, #30773, #17363, #27958, #31206, #34651, #30564, #782, #13907, #10679, #37020, #7460, #33796, #1206, #4221, #14331, #27527, #41309, #2283, #2065, #25574, #38090, #41732, #11747, #8953, #28817, #15823, #38729, #15194, #22328, #38936, #15404, #18874, #5503, #15612, #31632, #12590, #41947, #28391, #9159, #41531, #9367, #5289, #2690, #35504, #22536, #2484, #5929, #25783, #8530, #18652, #12171, #25361, #18441, #11961, #5079, #21685, #12379, #25151, #31848, #19081, #32054, #38299, #35290, #8744, #38509, #24947, #5722, #21897, #29020, #42158, #35077, #34866, #32261, #28602, #22116, #18225, #31414, #1851, #14977, #28175, #13004, #23170, #35709, #524, #26623, #42581, #16032, #94, #29866, #26831, #32682, #36541, #33109, #6139, #9991, #36333, #13217, #42367, #39771, #16239, #26411, #39560, #26199, #19919, #3532, #6764, #29440, #16669, #39346, #307, #19497, #13426, #30085, #16454, #20137, #10205, #2903, #29652, #9788, #3112, #13640, #23391, #39144, #22967, #36123, #33324, #6554, #35916, #3748, #6982, #16882, #6352, #39984, #10415, #19283, #29228, #25994, #32477, #19710, #12799, #9575, #22750, #32891, #3321, #20555, #1364, #13854, #17522, #30296, #27474, #4596, #34388, #14496, #33745, #40826, #14714, #20773, #37399, #24033, #34177, #7408, #31153, #17735, #4166, #27688, #17311, #27903, #23812, #21202, #11268, #41037, #20990, #4805, #27051, #30723, #30929, #23608, #30515, #24464, #37611, #36753, #40609, #24249, #1150, #734, #8055, #941, #14273, #11052, #14060, #7842, #17954, #1585, #27253, #7189, #40393, #20344, #10838, #33536, #3958, #4383, #17097, #40195, #10625, #36965, #37171, #7620, #33962, #41900, #14929, #34817, #41479, #9115, #25106, #11698, #22285, #25319, #5460, #24894, #12128, #18609, #28771, #34602, #1801, #12333, #38043, #31367, #38681, #25532, #5033, #8699, #8485, #32010, #28127, #31802, #18174, #15359, #35245, #35457, #2435, #21638, #5882, #2646, #21852, #38465, #11912, #22070, #5241, #19036, #5676, #18394, #15570, #31582, #15778, #2014, #32220, #28975, #11480, #8907, #24681, #41257, #37828, #8270, #15143, #38253, #2234, #28557, #28341, #35031, #21417, #41689, #18826, #25947, #12959, #39520, #26367, #42325, #29605, #32642, #19663, #6096, #49, #3069, #40296, #10739, #16195, #29186, #7306, #12750, #22705, #22923, #35665, #6514, #4279, #23931, #19451, #13173, #42114, #7518, #33644, #6306, #22490, #35874, #32851, #3278, #29394, #9948, #23128, #36292, #42535, #16406, #26155, #20456, #39096, #4066, #37075, #36077, #27154, #17207, #9321, #30409, #39305, #9534, #20668, #840, #2857, #9742, #13961, #33855, #17421, #12548, #25740, #38892, #19243, #32432, #15989, #1478, #28019, #40506, #7734, #41149, #17632, #37288, #24793, #37940, #10952, #4700, #30827, #31268, #20882, #14613, #24148, #11376, #4923, #8385, #1694, #1265, #11587, #18287, #17850, #8165, #21098, #34502, #14389, #5140, #18071, #27586, #14821, #40725, #31474, #4490, #21535, #34716, #1908, #21314, #30618, #34069, #1046, #14171, #11165, #31047, #24575, #37723, #24364, #37505, #27371, #40934, #7948, #34285, #27802, #23849, #10656, #26652, #13883, #16912, #3986, #33140, #27079, #30114, #24060, #37203, #551, #13458, #33774, #39802, #7016, #7222, #19952, #33562, #30750, #7650, #3778, #40222, #26438, #33989, #17340, #33358, #6796, #17127, #20585, #17549, #23421, #27289, #36998, #39589, #760, #7433, #30330, #3568, #30543, #1183, #4196, #971, #14088, #40426, #10869, #20801, #10024, #10447, #13670, #36570, #4410, #16702, #23204, #10234, #36363, #23639, #29899, #337, #20168, #26863, #40017, #20373, #36785, #11080, #40856, #27720, #1613, #31394, #11727, #28154, #38070, #30965, #8510, #11509, #38279, #5268, #21447, #21664, #7870, #17770, #24925, #8082, #41509, #8301, #2042, #34845, #1396, #18420, #21018, #24711, #31830, #14526, #41288, #34208, #24490, #31610, #14305, #15173, #37427, #28370, #11296, #11942, #37857, #37643, #34419, #21880, #34630, #25133, #18636, #27504, #21233, #17983, #4624, #4838, #8726, #35058, #5486, #31183, #40639, #14742, #27935, #41064, #5056, #18204, #24282, #1828, #14956, #14685, #20741, #30482, #36934, #40796, #24436, #1334, #911, #27873, #4352, #14465, #30899, #1118, #8024, #21168, #37579, #17493, #27655, #27445, #34358, #7588, #4774, #18141, #4562, #8238, #11237, #33711, #17704, #14242, #33929, #31337, #11450, #27222, #30686, #11022, #21386, #37367, #24000, #34569, #17922, #5000, #40581, #10807, #31119, #37140, #24216, #1552, #17277, #41006, #28096, #1768, #7810, #24650, #23780, #14897, #37793, #20958, #4136, #41224, #7377, #34144, #20523, #14026, #40366, #24862, #29306, #12879, #32557, #18361, #16322, #35582, #2986, #19370, #32350, #39225, #9663, #26074, #6011, #16110, #15900, #22836, #38220, #35998, #6638, #35794, #39437, #42452, #21606, #6225, #2774, #9236, #19788, #42663, #15109, #19160, #42241, #9870, #25861, #11879, #23043, #6432, #19576, #25075, #32759, #3196, #29521, #34785, #1983, #13087, #22405, #31550, #36201, #26287, #5206, #9453, #29105, #32975, #28304, #3404, #41443, #16539, #29738, #11661, #38010, #12666, #8455, #39016, #22619, #13934, #606, #10708, #26702, #7706, #37050, #23475, #33827, #10288, #4460, #394, #40476, #4251, #17603, #40271, #10924, #3626, #17393, #20856, #33195, #13721, #7277, #20431, #13513, #36623, #185, #16753, #7487, #39854, #26911, #23905, #27128, #7070, #30380, #33409, #33616, #6850, #812, #3834, #24118, #40068, #20638, #20219, #34040, #30590, #16970, #1021, #30165, #13305, #10499, #37254, #14141, #26494, #27342, #39639, #29954, #10080, #23256, #23687, #36834, #4035, #17182, #36416, #20003, #5533, #4673, #38120, #14583, #1661, #28206, #15008, #31018, #18254, #21285, #8354, #37477, #31445, #34471, #28424, #41560, #4893, #17823, #8565, #1448, #11350, #11557, #24336, #37910, #35108, #11993, #8136, #1880, #30799, #38329, #21715, #37694, #11134, #21505, #24979, #24543, #34896, #27770, #7921, #1236, #5107, #41340, #34687, #21068, #5320, #18041, #11777, #18474, #31237, #31661, #2095, #15225, #14793, #25188, #27988, #8771, #40908, #21928, #14361, #24766, #27559, #40693, #34259, #41118, #9186, #15643, #13036, #6381, #22147, #41977, #5961, #16268, #32295, #18903, #29467, #32503, #12616, #32084, #19311, #25809, #35940, #41766, #8980, #19524, #2518, #38539, #3141, #32708, #12200, #15850, #28843, #39172, #35321, #38965, #25391, #22564, #42398, #42609, #9606, #12409, #26230, #9814, #29050, #2933, #26020, #25602, #2719, #16062, #29254, #38760, #6170, #22357, #9400, #5750, #12829, #35533, #39378, #22992, #19112, #42189, #22779, #35742, #36149, #18682, #31880, #2310, #15437, #28635, #26649, #36782, #6582, #14085, #40219, #13454, #29683, #13667, #758, #29895, #10653, #3565, #13248, #19738, #23636, #7218, #26860, #26435, #23845, #334, #40014, #10444, #39799, #33559, #3982, #20370, #10231, #17124, #23419, #30327, #33137, #13880, #968, #30110, #33771, #27076, #16484, #548, #36567, #16699, #27286, #36995, #10022, #7013, #20165, #4193, #33355, #6793, #17338, #7430, #20581, #19949, #30541, #40422, #10866, #127, #39586, #24057, #3775, #23201, #32918, #3351, #36360, #16909, #34205, #14953, #27501, #31180, #1180, #41061, #18200, #5265, #28151, #4621, #11724, #28367, #34416, #8299, #37640, #5053, #21015, #2039, #31391, #17767, #41285, #30961, #41506, #37424, #34841, #24922, #11938, #34627, #18417, #40636, #38066, #15170, #11076, #8079, #1609, #14739, #7867, #1393, #37199, #24279, #14523, #27932, #14301, #11506, #1825, #31607, #8507, #27716, #21661, #7647, #4834, #21443, #21230, #20798, #40854, #33986, #4407, #11293, #17546, #24487, #30748, #17980, #24708, #37854, #29420, #22517, #22731, #28582, #29209, #32663, #15384, #25556, #32243, #2670, #25342, #5704, #42560, #41711, #32457, #8933, #38707, #35690, #9348, #38489, #12571, #15593, #15803, #31827, #25764, #28795, #35897, #6334, #41926, #12150, #2883, #22097, #18855, #5909, #18633, #28999, #25130, #19477, #2463, #38917, #38276, #3093, #16013, #32035, #5483, #42140, #19264, #12358, #42348, #35271, #2263, #8722, #6119, #12780, #25972, #9141, #39123, #22309, #9557, #16220, #35482, #21877, #35055, #19062, #36315, #20119, #16649, #23587, #39542, #36734, #7390, #36522, #40174, #30065, #22948, #6962, #3512, #9973, #20537, #717, #16432, #6747, #288, #10606, #26602, #13198, #23793, #26815, #33307, #26391, #13623, #3732, #30278, #36102, #3304, #13836, #23153, #32873, #36948, #27030, #6536, #10187, #19900, #33518, #33084, #29850, #13409, #507, #10397, #39967, #7172, #29631, #20324, #23372, #33726, #3941, #16862, #17079, #19689, #74, #4149, #39752, #17293, #30497, #12984, #26181, #39328, #9768, #7601, #11250, #18375, #1132, #27886, #20755, #11036, #5014, #923, #24664, #24013, #18155, #27458, #11463, #24448, #14255, #20971, #8469, #40810, #41019, #5219, #14039, #24230, #4575, #33944, #4366, #37806, #8252, #21399, #17505, #31134, #27235, #21620, #34584, #7824, #37154, #8037, #31350, #37381, #1780, #40594, #30700, #40378, #17935, #1567, #21181, #34157, #14910, #17717, #34371, #4787, #30912, #28109, #41237, #14697, #1348, #11675, #14477, #24875, #27672, #38025, #34799, #37593, #10820, #5860, #41458, #12313, #22050, #28538, #25922, #19221, #35011, #12105, #18802, #29163, #2416, #31779, #42303, #2626, #25511, #2209, #32199, #38659, #6073, #11893, #21832, #32411, #15341, #8678, #15967, #2833, #25088, #28750, #41670, #9297, #5441, #9096, #38233, #35432, #12526, #12725, #22467, #25300, #18593, #39074, #38443, #42093, #41876, #8887, #35223, #9512, #22263, #28956, #35851, #31564, #5654, #31990, #15548, #19014, #25719, #22683, #15758, #35644, #38868, #6285, #1997, #15122, #28317, #13149, #16812, #3255, #22901, #33035, #36057, #26344, #6492, #33468, #39917, #20280, #3684, #10347, #7125, #36896, #6909, #13786, #3464, #3045, #23535, #19640, #32824, #30011, #457, #16173, #668, #26132, #16599, #12935, #13573, #29802, #26556, #36268, #16381, #39704, #242, #3894, #13364, #10140, #6699, #39285, #9718, #26764, #29368, #19430, #36685, #23320, #17029, #30228, #26969, #40127, #32620, #36475, #39496, #29583, #33258, #42509, #10557, #26, #23743, #20063, #9927, #23106, #19850, #37325, #27834, #30857, #40966, #4101, #33890, #20702, #7772, #24397, #4734, #21128, #31078, #23961, #1511, #4519, #31297, #11409, #14424, #14645, #873, #10772, #17881, #1078, #34531, #1294, #37752, #24603, #37105, #8196, #13989, #17663, #24825, #7549, #34317, #27186, #17451, #21345, #7340, #4955, #18102, #17242, #4312, #30647, #20915, #37538, #1729, #14855, #28052, #14204, #41178, #27617, #11617, #20489, #40757, #33675, #40330, #27403, #30442, #40539, #10983, #11199, #24178, #34098, #7978, #18960, #1940, #5594, #12675, #38180, #22207, #15066, #5383, #42042, #37971, #32147, #18321, #12469, #21780, #5807, #18747, #8624, #15289, #2784, #35169, #35382, #42250, #8415, #18534, #41618, #28266, #41403, #2577, #35593, #12262, #28905, #31725, #2154, #11837, #31510, #25038, #28486, #15706, #34960, #12052, #8835, #25248, #38393, #21991, #9245, #25663, #38818, #22415, #6021, #19171, #21566, #25458, #32360, #31939, #34747, #15913 ) ),
 .UNSPECIFIED., .F., .F., .F. ) 
 B_SPLINE_SURFACE_WITH_KNOTS ( ( 2, 2 ),
 ( 3, 2, 2, 2, 2, 2, 2, 2, 2, 2, 2, 2, 2, 2, 2, 2, 2, 2, 2, 2, 2, 2, 2, 2, 2, 2, 2, 2, 2, 2, 2, 2, 2, 2, 2, 2, 2, 2, 2, 2, 2, 2, 2, 2, 2, 2, 2, 2, 2, 2, 2, 2, 2, 2, 2, 2, 2, 2, 2, 2, 2, 2, 2, 2, 2, 2, 2, 2, 2, 2, 2, 2, 2, 2, 2, 2, 2, 2, 2, 2, 2, 2, 2, 2, 2, 2, 2, 2, 2, 2, 2, 2, 2, 2, 2, 2, 2, 2, 2, 2, 2, 2, 2, 2, 2, 2, 2, 2, 2, 2, 2, 2, 2, 2, 2, 2, 2, 2, 2, 2, 2, 2, 2, 2, 2, 2, 2, 2, 2, 2, 2, 2, 2, 2, 2, 2, 2, 2, 2, 2, 2, 2, 2, 2, 2, 2, 2, 2, 2, 2, 2, 2, 2, 2, 2, 2, 2, 2, 2, 2, 2, 2, 2, 2, 2, 2, 2, 2, 2, 2, 2, 2, 2, 2, 2, 2, 2, 2, 2, 2, 2, 2, 2, 2, 2, 2, 2, 2, 2, 2, 2, 2, 2, 2, 2, 2, 2, 2, 2, 2, 2, 2, 2, 2, 2, 2, 2, 2, 2, 2, 2, 2, 2, 2, 2, 2, 2, 2, 2, 2, 2, 2, 2, 2, 2, 2, 2, 2, 2, 2, 2, 2, 2, 2, 2, 2, 2, 2, 2, 2, 2, 2, 2, 2, 2, 2, 2, 2, 2, 2, 2, 2, 2, 2, 2, 2, 2, 2, 2, 2, 2, 2, 2, 2, 2, 2, 2, 2, 2, 2, 2, 2, 2, 2, 2, 2, 2, 2, 2, 2, 2, 2, 2, 2, 2, 2, 2, 2, 2, 2, 2, 2, 2, 2, 2, 2, 2, 2, 2, 2, 2, 2, 2, 2, 2, 2, 2, 2, 2, 2, 2, 2, 2, 2, 2, 2, 2, 2, 2, 2, 2, 2, 2, 2, 2, 2, 2, 2, 2, 2, 2, 2, 2, 2, 2, 2, 2, 2, 2, 2, 2, 2, 2, 2, 2, 2, 2, 2, 2, 2, 2, 2, 2, 2, 2, 2, 2, 2, 2, 2, 2, 2, 2, 2, 2, 2, 2, 2, 2, 2, 2, 2, 2, 2, 2, 2, 2, 2, 2, 2, 2, 2, 2, 2, 2, 2, 2, 2, 2, 2, 2, 2, 2, 2, 2, 2, 2, 2, 2, 2, 2, 2, 2, 2, 2, 2, 2, 2, 2, 2, 2, 2, 2, 2, 2, 2, 2, 2, 2, 2, 2, 2, 2, 2, 2, 2, 2, 2, 2, 2, 2, 2, 2, 2, 2, 2, 2, 2, 2, 2, 2, 2, 2, 2, 2, 2, 2, 2, 2, 2, 2, 2, 2, 2, 2, 2, 2, 2, 2, 2, 2, 2, 2, 2, 2, 2, 2, 2, 2, 2, 2, 2, 2, 2, 2, 2, 2, 2, 2, 2, 2, 2, 2, 2, 2, 2, 2, 2, 2, 2, 2, 2, 2, 2, 2, 2, 2, 2, 2, 2, 2, 2, 2, 2, 2, 2, 2, 2, 2, 2, 2, 2, 2, 2, 2, 2, 2, 2, 2, 2, 2, 2, 2, 2, 2, 2, 2, 2, 2, 2, 2, 2, 2, 2, 2, 2, 2, 2, 2, 2, 2, 2, 2, 2, 2, 2, 2, 2, 2, 2, 2, 2, 2, 2, 2, 2, 2, 2, 2, 2, 2, 2, 2, 2, 2, 2, 2, 2, 2, 2, 2, 2, 2, 2, 2, 2, 2, 2, 2, 2, 2, 2, 2, 2, 2, 2, 2, 2, 2, 2, 2, 2, 2, 2, 2, 2, 2, 2, 2, 2, 2, 2, 2, 2, 2, 2, 2, 2, 2, 2, 2, 2, 2, 2, 2, 2, 2, 2, 2, 2, 2, 2, 2, 2, 2, 2, 2, 2, 2, 2, 2, 2, 2, 2, 2, 2, 2, 2, 2, 2, 2, 2, 2, 2, 2, 2, 2, 2, 2, 2, 2, 2, 2, 2, 2, 2, 2, 2, 2, 2, 2, 2, 2, 2, 2, 2, 2, 2, 2, 2, 2, 2, 2, 2, 2, 2, 2, 2, 2, 2, 2, 2, 2, 2, 2, 2, 2, 2, 2, 2, 2, 2, 2, 2, 2, 2, 2, 2, 2, 2, 2, 2, 2, 2, 2, 2, 2, 2, 2, 2, 2, 2, 2, 2, 2, 2, 2, 2, 2, 2, 2, 2, 2, 2, 2, 2, 2, 2, 2, 2, 2, 2, 2, 2, 2, 2, 2, 2, 2, 2, 2, 2, 2, 2, 2, 2, 2, 2, 2, 2, 2, 2, 2, 2, 2, 2, 2, 2, 2, 2, 2, 2, 2, 2, 2, 2, 2, 2, 2, 2, 2, 2, 2, 2, 2, 2, 2, 2, 2, 2, 2, 2, 2, 2, 2, 2, 2, 2, 2, 2, 2, 2, 2, 2, 2, 2, 2, 2, 2, 2, 3 ),
 ( 0.000000000000000000, 1.000000000000000000 ),
 ( 0.000000000000000000, 0.001243781094527363160, 0.002487562189054726321, 0.003731343283582089481, 0.004975124378109452641, 0.006218905472636816235, 0.007462686567164178962, 0.008706467661691542556, 0.009950248756218905283, 0.01119402985074626801, 0.01243781094527363247, 0.01368159203980099520, 0.01492537313432835792, 0.01616915422885572065, 0.01741293532338308511, 0.01865671641791044610, 0.01990049751243781057, 0.02114427860696517503, 0.02238805970149253602, 0.02363184079601990048, 0.02487562189054726494, 0.02611940298507462593, 0.02736318407960199039, 0.02860696517412935486, 0.02985074626865671585, 0.03109452736318408031, 0.03233830845771144130, 0.03358208955223880576, 0.03482587064676617022, 0.03606965174129353469, 0.03731343283582089221, 0.03855721393034825667, 0.03980099502487562113, 0.04104477611940298559, 0.04228855721393035005, 0.04353233830845771452, 0.04477611940298507204, 0.04601990049751243650, 0.04726368159203980096, 0.04850746268656716542, 0.04975124378109452988, 0.05099502487562188741, 0.05223880597014925187, 0.05348258706467661633, 0.05472636815920398079, 0.05597014925373134525, 0.05721393034825870971, 0.05845771144278606724, 0.05970149253731343170, 0.06094527363184079616, 0.06218905472636816062, 0.06343283582089552508, 0.06467661691542288260, 0.06592039800995025400, 0.06716417910447761153, 0.06840796019900496905, 0.06965174129353234045, 0.07089552238805969797, 0.07213930348258706937, 0.07338308457711442689, 0.07462686567164178442, 0.07587064676616915582, 0.07711442786069651334, 0.07835820895522388474, 0.07960199004975124226, 0.08084577114427861366, 0.08208955223880597118, 0.08333333333333332871, 0.08457711442786070011, 0.08582089552238805763, 0.08706467661691542903, 0.08830845771144278655, 0.08955223880597014408, 0.09079601990049751548, 0.09203980099502487300, 0.09328358208955224440, 0.09452736318407960192, 0.09577114427860695944, 0.09701492537313433084, 0.09825870646766168837, 0.09950248756218905977, 0.1007462686567164173, 0.1019900497512437748, 0.1032338308457711462, 0.1044776119402985037, 0.1057213930348258751, 0.1069651741293532327, 0.1082089552238805902, 0.1094527363184079616, 0.1106965174129353191, 0.1119402985074626905, 0.1131840796019900480, 0.1144278606965174194, 0.1156716417910447769, 0.1169154228855721345, 0.1181592039800995059, 0.1194029850746268634, 0.1206467661691542348, 0.1218905472636815923, 0.1231343283582089498, 0.1243781094527363212, 0.1256218905472636926, 0.1268656716417910502, 0.1281094527363184077, 0.1293532338308457652, 0.1305970149253731227, 0.1318407960199005080, 0.1330845771144278655, 0.1343283582089552231, 0.1355721393034825806, 0.1368159203980099381, 0.1380597014925373234, 0.1393034825870646809, 0.1405472636815920384, 0.1417910447761193959, 0.1430348258706467535, 0.1442786069651741387, 0.1455223880597014963, 0.1467661691542288538, 0.1480099502487562113, 0.1492537313432835688, 0.1504975124378109541, 0.1517412935323383116, 0.1529850746268656692, 0.1542288557213930267, 0.1554726368159203842, 0.1567164179104477695, 0.1579601990049751270, 0.1592039800995024845, 0.1604477611940298420, 0.1616915422885572273, 0.1629353233830845848, 0.1641791044776119424, 0.1654228855721392999, 0.1666666666666666574, 0.1679104477611940427, 0.1691542288557214002, 0.1703980099502487577, 0.1716417910447761153, 0.1728855721393034728, 0.1741293532338308581, 0.1753731343283582156, 0.1766169154228855731, 0.1778606965174129306, 0.1791044776119402882, 0.1803482587064676734, 0.1815920398009950310, 0.1828358208955223885, 0.1840796019900497460, 0.1853233830845771035, 0.1865671641791044888, 0.1878109452736318463, 0.1890547263681592038, 0.1902985074626865614, 0.1915422885572139189, 0.1927860696517413042, 0.1940298507462686617, 0.1952736318407960192, 0.1965174129353233767, 0.1977611940298507343, 0.1990049751243781195, 0.2002487562189054771, 0.2014925373134328346, 0.2027363184079601921, 0.2039800995024875496, 0.2052238805970149349, 0.2064676616915422924, 0.2077114427860696499, 0.2089552238805970075, 0.2101990049751243650, 0.2114427860696517503, 0.2126865671641791078, 0.2139303482587064653, 0.2151741293532338228, 0.2164179104477611804, 0.2176616915422885656, 0.2189054726368159232, 0.2201492537313432807, 0.2213930348258706382, 0.2226368159203980235, 0.2238805970149253810, 0.2251243781094527385, 0.2263681592039800961, 0.2276119402985074536, 0.2288557213930348389, 0.2300995024875621964, 0.2313432835820895539, 0.2325870646766169114, 0.2338308457711442689, 0.2350746268656716542, 0.2363184079601990117, 0.2375621890547263693, 0.2388059701492537268, 0.2400497512437810843, 0.2412935323383084696, 0.2425373134328358271, 0.2437810945273631846, 0.2450248756218905422, 0.2462686567164178997, 0.2475124378109452850, 0.2487562189054726425, 0.2500000000000000000, 0.2512437810945273853, 0.2524875621890547150, 0.2537313432835821003, 0.2549751243781094301, 0.2562189054726368154, 0.2574626865671642006, 0.2587064676616915304, 0.2599502487562189157, 0.2611940298507462455, 0.2624378109452736307, 0.2636815920398010160, 0.2649253731343283458, 0.2661691542288557311, 0.2674129353233830608, 0.2686567164179104461, 0.2699004975124378314, 0.2711442786069651611, 0.2723880597014925464, 0.2736318407960198762, 0.2748756218905472615, 0.2761194029850746468, 0.2773631840796019765, 0.2786069651741293618, 0.2798507462686566916, 0.2810945273631840768, 0.2823383084577114621, 0.2835820895522387919, 0.2848258706467661772, 0.2860696517412935069, 0.2873134328358208922, 0.2885572139303482775, 0.2898009950248756073, 0.2910447761194029925, 0.2922885572139303223, 0.2935323383084577076, 0.2947761194029850929, 0.2960199004975124226, 0.2972636815920398079, 0.2985074626865671377, 0.2997512437810945229, 0.3009950248756219082, 0.3022388059701492380, 0.3034825870646766233, 0.3047263681592039530, 0.3059701492537313383, 0.3072139303482587236, 0.3084577114427860534, 0.3097014925373134386, 0.3109452736318407684, 0.3121890547263681537, 0.3134328358208955390, 0.3146766169154228687, 0.3159203980099502540, 0.3171641791044776393, 0.3184079601990049690, 0.3196517412935323543, 0.3208955223880596841, 0.3221393034825870694, 0.3233830845771144546, 0.3246268656716417844, 0.3258706467661691697, 0.3271144278606964995, 0.3283582089552238847, 0.3296019900497512700, 0.3308457711442785998, 0.3320895522388059851, 0.3333333333333333148, 0.3345771144278607001, 0.3358208955223880854, 0.3370646766169154152, 0.3383084577114428004, 0.3395522388059701302, 0.3407960199004975155, 0.3420398009950249008, 0.3432835820895522305, 0.3445273631840796158, 0.3457711442786069456, 0.3470149253731343308, 0.3482587064676617161, 0.3495024875621890459, 0.3507462686567164312, 0.3519900497512437609, 0.3532338308457711462, 0.3544776119402985315, 0.3557213930348258613, 0.3569651741293532465, 0.3582089552238805763, 0.3594527363184079616, 0.3606965174129353469, 0.3619402985074626766, 0.3631840796019900619, 0.3644278606965173917, 0.3656716417910447769, 0.3669154228855721622, 0.3681592039800994920, 0.3694029850746268773, 0.3706467661691542070, 0.3718905472636815923, 0.3731343283582089776, 0.3743781094527363074, 0.3756218905472636926, 0.3768656716417910224, 0.3781094527363184077, 0.3793532338308457930, 0.3805970149253731227, 0.3818407960199005080, 0.3830845771144278378, 0.3843283582089552231, 0.3855721393034826083, 0.3868159203980099381, 0.3880597014925373234, 0.3893034825870646531, 0.3905472636815920384, 0.3917910447761194237, 0.3930348258706467535, 0.3942786069651741387, 0.3955223880597014685, 0.3967661691542288538, 0.3980099502487562391, 0.3992537313432835688, 0.4004975124378109541, 0.4017412935323382839, 0.4029850746268656692, 0.4042288557213930544, 0.4054726368159203842, 0.4067164179104477695, 0.4079601990049750992, 0.4092039800995024845, 0.4104477611940298698, 0.4116915422885571996, 0.4129353233830845848, 0.4141791044776119146, 0.4154228855721392999, 0.4166666666666666852, 0.4179104477611940149, 0.4191542288557214002, 0.4203980099502487300, 0.4216417910447761153, 0.4228855721393035005, 0.4241293532338308303, 0.4253731343283582156, 0.4266169154228855454, 0.4278606965174129306, 0.4291044776119403159, 0.4303482587064676457, 0.4315920398009950310, 0.4328358208955223607, 0.4340796019900497460, 0.4353233830845771313, 0.4365671641791044610, 0.4378109452736318463, 0.4390547263681592316, 0.4402985074626865614, 0.4415422885572139466, 0.4427860696517412764, 0.4440298507462686617, 0.4452736318407960470, 0.4465174129353233767, 0.4477611940298507620, 0.4490049751243780918, 0.4502487562189054771, 0.4514925373134328623, 0.4527363184079601921, 0.4539800995024875774, 0.4552238805970149071, 0.4564676616915422924, 0.4577114427860696777, 0.4589552238805970075, 0.4601990049751243927, 0.4614427860696517225, 0.4626865671641791078, 0.4639303482587064931, 0.4651741293532338228, 0.4664179104477612081, 0.4676616915422885379, 0.4689054726368159232, 0.4701492537313433084, 0.4713930348258706382, 0.4726368159203980235, 0.4738805970149253532, 0.4751243781094527385, 0.4763681592039801238, 0.4776119402985074536, 0.4788557213930348389, 0.4800995024875621686, 0.4813432835820895539, 0.4825870646766169392, 0.4838308457711442689, 0.4850746268656716542, 0.4863184079601989840, 0.4875621890547263693, 0.4888059701492537545, 0.4900497512437810843, 0.4912935323383084696, 0.4925373134328357994, 0.4937810945273631846, 0.4950248756218905699, 0.4962686567164178997, 0.4975124378109452850, 0.4987562189054726147, 0.5000000000000000000, 0.5012437810945273853, 0.5024875621890547706, 0.5037313432835820448, 0.5049751243781094301, 0.5062189054726368154, 0.5074626865671642006, 0.5087064676616915859, 0.5099502487562188602, 0.5111940298507462455, 0.5124378109452736307, 0.5136815920398010160, 0.5149253731343284013, 0.5161691542288556755, 0.5174129353233830608, 0.5186567164179104461, 0.5199004975124378314, 0.5211442786069652167, 0.5223880597014924909, 0.5236318407960198762, 0.5248756218905472615, 0.5261194029850746468, 0.5273631840796020320, 0.5286069651741293063, 0.5298507462686566916, 0.5310945273631840768, 0.5323383084577114621, 0.5335820895522388474, 0.5348258706467661217, 0.5360696517412935069, 0.5373134328358208922, 0.5385572139303482775, 0.5398009950248756628, 0.5410447761194029370, 0.5422885572139303223, 0.5435323383084577076, 0.5447761194029850929, 0.5460199004975124781, 0.5472636815920397524, 0.5485074626865671377, 0.5497512437810945229, 0.5509950248756219082, 0.5522388059701492935, 0.5534825870646765678, 0.5547263681592039530, 0.5559701492537313383, 0.5572139303482587236, 0.5584577114427861089, 0.5597014925373133831, 0.5609452736318407684, 0.5621890547263681537, 0.5634328358208955390, 0.5646766169154229242, 0.5659203980099501985, 0.5671641791044775838, 0.5684079601990049690, 0.5696517412935323543, 0.5708955223880597396, 0.5721393034825870139, 0.5733830845771143991, 0.5746268656716417844, 0.5758706467661691697, 0.5771144278606965550, 0.5783582089552238292, 0.5796019900497512145, 0.5808457711442785998, 0.5820895522388059851, 0.5833333333333333703, 0.5845771144278606446, 0.5858208955223880299, 0.5870646766169154152, 0.5883084577114428004, 0.5895522388059701857, 0.5907960199004974600, 0.5920398009950248452, 0.5932835820895522305, 0.5945273631840796158, 0.5957711442786070011, 0.5970149253731342753, 0.5982587064676616606, 0.5995024875621890459, 0.6007462686567164312, 0.6019900497512438164, 0.6032338308457710907, 0.6044776119402984760, 0.6057213930348258613, 0.6069651741293532465, 0.6082089552238806318, 0.6094527363184079061, 0.6106965174129352913, 0.6119402985074626766, 0.6131840796019900619, 0.6144278606965174472, 0.6156716417910447214, 0.6169154228855721067, 0.6181592039800994920, 0.6194029850746268773, 0.6206467661691542625, 0.6218905472636815368, 0.6231343283582089221, 0.6243781094527363074, 0.6256218905472636926, 0.6268656716417910779, 0.6281094527363184632, 0.6293532338308457375, 0.6305970149253731227, 0.6318407960199005080, 0.6330845771144278933, 0.6343283582089552786, 0.6355721393034825528, 0.6368159203980099381, 0.6380597014925373234, 0.6393034825870647087, 0.6405472636815920939, 0.6417910447761193682, 0.6430348258706467535, 0.6442786069651741387, 0.6455223880597015240, 0.6467661691542289093, 0.6480099502487561836, 0.6492537313432835688, 0.6504975124378109541, 0.6517412935323383394, 0.6529850746268657247, 0.6542288557213929989, 0.6554726368159203842, 0.6567164179104477695, 0.6579601990049751548, 0.6592039800995025400, 0.6604477611940298143, 0.6616915422885571996, 0.6629353233830845848, 0.6641791044776119701, 0.6654228855721393554, 0.6666666666666666297, 0.6679104477611940149, 0.6691542288557214002, 0.6703980099502487855, 0.6716417910447761708, 0.6728855721393034450, 0.6741293532338308303, 0.6753731343283582156, 0.6766169154228856009, 0.6778606965174129861, 0.6791044776119402604, 0.6803482587064676457, 0.6815920398009950310, 0.6828358208955224162, 0.6840796019900498015, 0.6853233830845770758, 0.6865671641791044610, 0.6878109452736318463, 0.6890547263681592316, 0.6902985074626866169, 0.6915422885572138911, 0.6927860696517412764, 0.6940298507462686617, 0.6952736318407960470, 0.6965174129353234322, 0.6977611940298507065, 0.6990049751243780918, 0.7002487562189054771, 0.7014925373134328623, 0.7027363184079602476, 0.7039800995024875219, 0.7052238805970149071, 0.7064676616915422924, 0.7077114427860696777, 0.7089552238805970630, 0.7101990049751243372, 0.7114427860696517225, 0.7126865671641791078, 0.7139303482587064931, 0.7151741293532338783, 0.7164179104477611526, 0.7176616915422885379, 0.7189054726368159232, 0.7201492537313433084, 0.7213930348258706937, 0.7226368159203979680, 0.7238805970149253532, 0.7251243781094527385, 0.7263681592039801238, 0.7276119402985075091, 0.7288557213930347833, 0.7300995024875621686, 0.7313432835820895539, 0.7325870646766169392, 0.7338308457711443245, 0.7350746268656715987, 0.7363184079601989840, 0.7375621890547263693, 0.7388059701492537545, 0.7400497512437811398, 0.7412935323383084141, 0.7425373134328357994, 0.7437810945273631846, 0.7450248756218905699, 0.7462686567164179552, 0.7475124378109452294, 0.7487562189054726147, 0.7500000000000000000, 0.7512437810945273853, 0.7524875621890547706, 0.7537313432835820448, 0.7549751243781094301, 0.7562189054726368154, 0.7574626865671642006, 0.7587064676616915859, 0.7599502487562188602, 0.7611940298507462455, 0.7624378109452736307, 0.7636815920398010160, 0.7649253731343284013, 0.7661691542288556755, 0.7674129353233830608, 0.7686567164179104461, 0.7699004975124378314, 0.7711442786069652167, 0.7723880597014924909, 0.7736318407960198762, 0.7748756218905472615, 0.7761194029850746468, 0.7773631840796020320, 0.7786069651741293063, 0.7798507462686566916, 0.7810945273631840768, 0.7823383084577114621, 0.7835820895522388474, 0.7848258706467661217, 0.7860696517412935069, 0.7873134328358208922, 0.7885572139303482775, 0.7898009950248756628, 0.7910447761194029370, 0.7922885572139303223, 0.7935323383084577076, 0.7947761194029850929, 0.7960199004975124781, 0.7972636815920397524, 0.7985074626865671377, 0.7997512437810945229, 0.8009950248756219082, 0.8022388059701492935, 0.8034825870646765678, 0.8047263681592039530, 0.8059701492537313383, 0.8072139303482587236, 0.8084577114427861089, 0.8097014925373133831, 0.8109452736318407684, 0.8121890547263681537, 0.8134328358208955390, 0.8146766169154229242, 0.8159203980099501985, 0.8171641791044775838, 0.8184079601990049690, 0.8196517412935323543, 0.8208955223880597396, 0.8221393034825870139, 0.8233830845771143991, 0.8246268656716417844, 0.8258706467661691697, 0.8271144278606965550, 0.8283582089552238292, 0.8296019900497512145, 0.8308457711442785998, 0.8320895522388059851, 0.8333333333333333703, 0.8345771144278606446, 0.8358208955223880299, 0.8370646766169154152, 0.8383084577114428004, 0.8395522388059701857, 0.8407960199004974600, 0.8420398009950248452, 0.8432835820895522305, 0.8445273631840796158, 0.8457711442786070011, 0.8470149253731342753, 0.8482587064676616606, 0.8495024875621890459, 0.8507462686567164312, 0.8519900497512438164, 0.8532338308457710907, 0.8544776119402984760, 0.8557213930348258613, 0.8569651741293532465, 0.8582089552238806318, 0.8594527363184079061, 0.8606965174129352913, 0.8619402985074626766, 0.8631840796019900619, 0.8644278606965174472, 0.8656716417910447214, 0.8669154228855721067, 0.8681592039800994920, 0.8694029850746268773, 0.8706467661691542625, 0.8718905472636815368, 0.8731343283582089221, 0.8743781094527363074, 0.8756218905472636926, 0.8768656716417910779, 0.8781094527363184632, 0.8793532338308457375, 0.8805970149253731227, 0.8818407960199005080, 0.8830845771144278933, 0.8843283582089552786, 0.8855721393034825528, 0.8868159203980099381, 0.8880597014925373234, 0.8893034825870647087, 0.8905472636815920939, 0.8917910447761193682, 0.8930348258706467535, 0.8942786069651741387, 0.8955223880597015240, 0.8967661691542289093, 0.8980099502487561836, 0.8992537313432835688, 0.9004975124378109541, 0.9017412935323383394, 0.9029850746268657247, 0.9042288557213929989, 0.9054726368159203842, 0.9067164179104477695, 0.9079601990049751548, 0.9092039800995025400, 0.9104477611940298143, 0.9116915422885571996, 0.9129353233830845848, 0.9141791044776119701, 0.9154228855721393554, 0.9166666666666666297, 0.9179104477611940149, 0.9191542288557214002, 0.9203980099502487855, 0.9216417910447761708, 0.9228855721393034450, 0.9241293532338308303, 0.9253731343283582156, 0.9266169154228856009, 0.9278606965174129861, 0.9291044776119402604, 0.9303482587064676457, 0.9315920398009950310, 0.9328358208955224162, 0.9340796019900498015, 0.9353233830845770758, 0.9365671641791044610, 0.9378109452736318463, 0.9390547263681592316, 0.9402985074626866169, 0.9415422885572138911, 0.9427860696517412764, 0.9440298507462686617, 0.9452736318407960470, 0.9465174129353234322, 0.9477611940298507065, 0.9490049751243780918, 0.9502487562189054771, 0.9514925373134328623, 0.9527363184079602476, 0.9539800995024875219, 0.9552238805970149071, 0.9564676616915422924, 0.9577114427860696777, 0.9589552238805970630, 0.9601990049751243372, 0.9614427860696517225, 0.9626865671641791078, 0.9639303482587064931, 0.9651741293532338783, 0.9664179104477611526, 0.9676616915422885379, 0.9689054726368159232, 0.9701492537313433084, 0.9713930348258706937, 0.9726368159203979680, 0.9738805970149253532, 0.9751243781094527385, 0.9763681592039801238, 0.9776119402985075091, 0.9788557213930347833, 0.9800995024875621686, 0.9813432835820895539, 0.9825870646766169392, 0.9838308457711443245, 0.9850746268656715987, 0.9863184079601989840, 0.9875621890547263693, 0.9888059701492537545, 0.9900497512437811398, 0.9912935323383084141, 0.9925373134328357994, 0.9937810945273631846, 0.9950248756218905699 ),
 .UNSPECIFIED. ) 
 GEOMETRIC_REPRESENTATION_ITEM ( )  RATIONAL_B_SPLINE_SURFACE ( (
 ( 1.000000000000000000, 0.8660254037844387076, 1.000000000000000000, 0.8660254037844387076, 1.000000000000000000, 0.8660254037844387076, 1.000000000000000000, 0.8660254037844387076, 1.000000000000000000, 0.8660254037844387076, 1.000000000000000000, 0.8660254037844387076, 1.000000000000000000, 0.8660254037844387076, 1.000000000000000000, 0.8660254037844387076, 1.000000000000000000, 0.8660254037844387076, 1.000000000000000000, 0.8660254037844387076, 1.000000000000000000, 0.8660254037844387076, 1.000000000000000000, 0.8660254037844387076, 1.000000000000000000, 0.8660254037844387076, 1.000000000000000000, 0.8660254037844387076, 1.000000000000000000, 0.8660254037844387076, 1.000000000000000000, 0.8660254037844387076, 1.000000000000000000, 0.8660254037844387076, 1.000000000000000000, 0.8660254037844387076, 1.000000000000000000, 0.8660254037844387076, 1.000000000000000000, 0.8660254037844387076, 1.000000000000000000, 0.8660254037844387076, 1.000000000000000000, 0.8660254037844387076, 1.000000000000000000, 0.8660254037844387076, 1.000000000000000000, 0.8660254037844387076, 1.000000000000000000, 0.8660254037844387076, 1.000000000000000000, 0.8660254037844387076, 1.000000000000000000, 0.8660254037844387076, 1.000000000000000000, 0.8660254037844387076, 1.000000000000000000, 0.8660254037844387076, 1.000000000000000000, 0.8660254037844387076, 1.000000000000000000, 0.8660254037844387076, 1.000000000000000000, 0.8660254037844387076, 1.000000000000000000, 0.8660254037844387076, 1.000000000000000000, 0.8660254037844387076, 1.000000000000000000, 0.8660254037844387076, 1.000000000000000000, 0.8660254037844387076, 1.000000000000000000, 0.8660254037844387076, 1.000000000000000000, 0.8660254037844387076, 1.000000000000000000, 0.8660254037844387076, 1.000000000000000000, 0.8660254037844387076, 1.000000000000000000, 0.8660254037844387076, 1.000000000000000000, 0.8660254037844387076, 1.000000000000000000, 0.8660254037844387076, 1.000000000000000000, 0.8660254037844387076, 1.000000000000000000, 0.8660254037844387076, 1.000000000000000000, 0.8660254037844387076, 1.000000000000000000, 0.8660254037844387076, 1.000000000000000000, 0.8660254037844387076, 1.000000000000000000, 0.8660254037844387076, 1.000000000000000000, 0.8660254037844387076, 1.000000000000000000, 0.8660254037844387076, 1.000000000000000000, 0.8660254037844387076, 1.000000000000000000, 0.8660254037844387076, 1.000000000000000000, 0.8660254037844387076, 1.000000000000000000, 0.8660254037844387076, 1.000000000000000000, 0.8660254037844387076, 1.000000000000000000, 0.8660254037844387076, 1.000000000000000000, 0.8660254037844387076, 1.000000000000000000, 0.8660254037844387076, 1.000000000000000000, 0.8660254037844387076, 1.000000000000000000, 0.8660254037844387076, 1.000000000000000000, 0.8660254037844387076, 1.000000000000000000, 0.8660254037844387076, 1.000000000000000000, 0.8660254037844387076, 1.000000000000000000, 0.8660254037844387076, 1.000000000000000000, 0.8660254037844387076, 1.000000000000000000, 0.8660254037844387076, 1.000000000000000000, 0.8660254037844387076, 1.000000000000000000, 0.8660254037844387076, 1.000000000000000000, 0.8660254037844387076, 1.000000000000000000, 0.8660254037844387076, 1.000000000000000000, 0.8660254037844387076, 1.000000000000000000, 0.8660254037844387076, 1.000000000000000000, 0.8660254037844387076, 1.000000000000000000, 0.8660254037844387076, 1.000000000000000000, 0.8660254037844387076, 1.000000000000000000, 0.8660254037844387076, 1.000000000000000000, 0.8660254037844387076, 1.000000000000000000, 0.8660254037844387076, 1.000000000000000000, 0.8660254037844387076, 1.000000000000000000, 0.8660254037844387076, 1.000000000000000000, 0.8660254037844387076, 1.000000000000000000, 0.8660254037844387076, 1.000000000000000000, 0.8660254037844387076, 1.000000000000000000, 0.8660254037844387076, 1.000000000000000000, 0.8660254037844387076, 1.000000000000000000, 0.8660254037844387076, 1.000000000000000000, 0.8660254037844387076, 1.000000000000000000, 0.8660254037844387076, 1.000000000000000000, 0.8660254037844387076, 1.000000000000000000, 0.8660254037844387076, 1.000000000000000000, 0.8660254037844387076, 1.000000000000000000, 0.8660254037844387076, 1.000000000000000000, 0.8660254037844387076, 1.000000000000000000, 0.8660254037844387076, 1.000000000000000000, 0.8660254037844387076, 1.000000000000000000, 0.8660254037844387076, 1.000000000000000000, 0.8660254037844387076, 1.000000000000000000, 0.8660254037844387076, 1.000000000000000000, 0.8660254037844387076, 1.000000000000000000, 0.8660254037844387076, 1.000000000000000000, 0.8660254037844387076, 1.000000000000000000, 0.8660254037844387076, 1.000000000000000000, 0.8660254037844387076, 1.000000000000000000, 0.8660254037844387076, 1.000000000000000000, 0.8660254037844387076, 1.000000000000000000, 0.8660254037844387076, 1.000000000000000000, 0.8660254037844387076, 1.000000000000000000, 0.8660254037844387076, 1.000000000000000000, 0.8660254037844387076, 1.000000000000000000, 0.8660254037844387076, 1.000000000000000000, 0.8660254037844387076, 1.000000000000000000, 0.8660254037844387076, 1.000000000000000000, 0.8660254037844387076, 1.000000000000000000, 0.8660254037844387076, 1.000000000000000000, 0.8660254037844387076, 1.000000000000000000, 0.8660254037844387076, 1.000000000000000000, 0.8660254037844387076, 1.000000000000000000, 0.8660254037844387076, 1.000000000000000000, 0.8660254037844387076, 1.000000000000000000, 0.8660254037844387076, 1.000000000000000000, 0.8660254037844387076, 1.000000000000000000, 0.8660254037844387076, 1.000000000000000000, 0.8660254037844387076, 1.000000000000000000, 0.8660254037844387076, 1.000000000000000000, 0.8660254037844387076, 1.000000000000000000, 0.8660254037844387076, 1.000000000000000000, 0.8660254037844387076, 1.000000000000000000, 0.8660254037844387076, 1.000000000000000000, 0.8660254037844387076, 1.000000000000000000, 0.8660254037844387076, 1.000000000000000000, 0.8660254037844387076, 1.000000000000000000, 0.8660254037844387076, 1.000000000000000000, 0.8660254037844387076, 1.000000000000000000, 0.8660254037844387076, 1.000000000000000000, 0.8660254037844387076, 1.000000000000000000, 0.8660254037844387076, 1.000000000000000000, 0.8660254037844387076, 1.000000000000000000, 0.8660254037844387076, 1.000000000000000000, 0.8660254037844387076, 1.000000000000000000, 0.8660254037844387076, 1.000000000000000000, 0.8660254037844387076, 1.000000000000000000, 0.8660254037844387076, 1.000000000000000000, 0.8660254037844387076, 1.000000000000000000, 0.8660254037844387076, 1.000000000000000000, 0.8660254037844387076, 1.000000000000000000, 0.8660254037844387076, 1.000000000000000000, 0.8660254037844387076, 1.000000000000000000, 0.8660254037844387076, 1.000000000000000000, 0.8660254037844387076, 1.000000000000000000, 0.8660254037844387076, 1.000000000000000000, 0.8660254037844387076, 1.000000000000000000, 0.8660254037844387076, 1.000000000000000000, 0.8660254037844387076, 1.000000000000000000, 0.8660254037844387076, 1.000000000000000000, 0.8660254037844387076, 1.000000000000000000, 0.8660254037844387076, 1.000000000000000000, 0.8660254037844387076, 1.000000000000000000, 0.8660254037844387076, 1.000000000000000000, 0.8660254037844387076, 1.000000000000000000, 0.8660254037844387076, 1.000000000000000000, 0.8660254037844387076, 1.000000000000000000, 0.8660254037844387076, 1.000000000000000000, 0.8660254037844387076, 1.000000000000000000, 0.8660254037844387076, 1.000000000000000000, 0.8660254037844387076, 1.000000000000000000, 0.8660254037844387076, 1.000000000000000000, 0.8660254037844387076, 1.000000000000000000, 0.8660254037844387076, 1.000000000000000000, 0.8660254037844387076, 1.000000000000000000, 0.8660254037844387076, 1.000000000000000000, 0.8660254037844387076, 1.000000000000000000, 0.8660254037844387076, 1.000000000000000000, 0.8660254037844387076, 1.000000000000000000, 0.8660254037844387076, 1.000000000000000000, 0.8660254037844387076, 1.000000000000000000, 0.8660254037844387076, 1.000000000000000000, 0.8660254037844387076, 1.000000000000000000, 0.8660254037844387076, 1.000000000000000000, 0.8660254037844387076, 1.000000000000000000, 0.8660254037844387076, 1.000000000000000000, 0.8660254037844387076, 1.000000000000000000, 0.8660254037844387076, 1.000000000000000000, 0.8660254037844387076, 1.000000000000000000, 0.8660254037844387076, 1.000000000000000000, 0.8660254037844387076, 1.000000000000000000, 0.8660254037844387076, 1.000000000000000000, 0.8660254037844387076, 1.000000000000000000, 0.8660254037844387076, 1.000000000000000000, 0.8660254037844387076, 1.000000000000000000, 0.8660254037844387076, 1.000000000000000000, 0.8660254037844387076, 1.000000000000000000, 0.8660254037844387076, 1.000000000000000000, 0.8660254037844387076, 1.000000000000000000, 0.8660254037844387076, 1.000000000000000000, 0.8660254037844387076, 1.000000000000000000, 0.8660254037844387076, 1.000000000000000000, 0.8660254037844387076, 1.000000000000000000, 0.8660254037844387076, 1.000000000000000000, 0.8660254037844387076, 1.000000000000000000, 0.8660254037844387076, 1.000000000000000000, 0.8660254037844387076, 1.000000000000000000, 0.8660254037844387076, 1.000000000000000000, 0.8660254037844387076, 1.000000000000000000, 0.8660254037844387076, 1.000000000000000000, 0.8660254037844387076, 1.000000000000000000, 0.8660254037844387076, 1.000000000000000000, 0.8660254037844387076, 1.000000000000000000, 0.8660254037844387076, 1.000000000000000000, 0.8660254037844387076, 1.000000000000000000, 0.8660254037844387076, 1.000000000000000000, 0.8660254037844387076, 1.000000000000000000, 0.8660254037844387076, 1.000000000000000000, 0.8660254037844387076, 1.000000000000000000, 0.8660254037844387076, 1.000000000000000000, 0.8660254037844387076, 1.000000000000000000, 0.8660254037844387076, 1.000000000000000000, 0.8660254037844387076, 1.000000000000000000, 0.8660254037844387076, 1.000000000000000000, 0.8660254037844387076, 1.000000000000000000, 0.8660254037844387076, 1.000000000000000000, 0.8660254037844387076, 1.000000000000000000, 0.8660254037844387076, 1.000000000000000000, 0.8660254037844387076, 1.000000000000000000, 0.8660254037844387076, 1.000000000000000000, 0.8660254037844387076, 1.000000000000000000, 0.8660254037844387076, 1.000000000000000000, 0.8660254037844387076, 1.000000000000000000, 0.8660254037844387076, 1.000000000000000000, 0.8660254037844387076, 1.000000000000000000, 0.8660254037844387076, 1.000000000000000000, 0.8660254037844387076, 1.000000000000000000, 0.8660254037844387076, 1.000000000000000000, 0.8660254037844387076, 1.000000000000000000, 0.8660254037844387076, 1.000000000000000000, 0.8660254037844387076, 1.000000000000000000, 0.8660254037844387076, 1.000000000000000000, 0.8660254037844387076, 1.000000000000000000, 0.8660254037844387076, 1.000000000000000000, 0.8660254037844387076, 1.000000000000000000, 0.8660254037844387076, 1.000000000000000000, 0.8660254037844387076, 1.000000000000000000, 0.8660254037844387076, 1.000000000000000000, 0.8660254037844387076, 1.000000000000000000, 0.8660254037844387076, 1.000000000000000000, 0.8660254037844387076, 1.000000000000000000, 0.8660254037844387076, 1.000000000000000000, 0.8660254037844387076, 1.000000000000000000, 0.8660254037844387076, 1.000000000000000000, 0.8660254037844387076, 1.000000000000000000, 0.8660254037844387076, 1.000000000000000000, 0.8660254037844387076, 1.000000000000000000, 0.8660254037844387076, 1.000000000000000000, 0.8660254037844387076, 1.000000000000000000, 0.8660254037844387076, 1.000000000000000000, 0.8660254037844387076, 1.000000000000000000, 0.8660254037844387076, 1.000000000000000000, 0.8660254037844387076, 1.000000000000000000, 0.8660254037844387076, 1.000000000000000000, 0.8660254037844387076, 1.000000000000000000, 0.8660254037844387076, 1.000000000000000000, 0.8660254037844387076, 1.000000000000000000, 0.8660254037844387076, 1.000000000000000000, 0.8660254037844387076, 1.000000000000000000, 0.8660254037844387076, 1.000000000000000000, 0.8660254037844387076, 1.000000000000000000, 0.8660254037844387076, 1.000000000000000000, 0.8660254037844387076, 1.000000000000000000, 0.8660254037844387076, 1.000000000000000000, 0.8660254037844387076, 1.000000000000000000, 0.8660254037844387076, 1.000000000000000000, 0.8660254037844387076, 1.000000000000000000, 0.8660254037844387076, 1.000000000000000000, 0.8660254037844387076, 1.000000000000000000, 0.8660254037844387076, 1.000000000000000000, 0.8660254037844387076, 1.000000000000000000, 0.8660254037844387076, 1.000000000000000000, 0.8660254037844387076, 1.000000000000000000, 0.8660254037844387076, 1.000000000000000000, 0.8660254037844387076, 1.000000000000000000, 0.8660254037844387076, 1.000000000000000000, 0.8660254037844387076, 1.000000000000000000, 0.8660254037844387076, 1.000000000000000000, 0.8660254037844387076, 1.000000000000000000, 0.8660254037844387076, 1.000000000000000000, 0.8660254037844387076, 1.000000000000000000, 0.8660254037844387076, 1.000000000000000000, 0.8660254037844387076, 1.000000000000000000, 0.8660254037844387076, 1.000000000000000000, 0.8660254037844387076, 1.000000000000000000, 0.8660254037844387076, 1.000000000000000000, 0.8660254037844387076, 1.000000000000000000, 0.8660254037844387076, 1.000000000000000000, 0.8660254037844387076, 1.000000000000000000, 0.8660254037844387076, 1.000000000000000000, 0.8660254037844387076, 1.000000000000000000, 0.8660254037844387076, 1.000000000000000000, 0.8660254037844387076, 1.000000000000000000, 0.8660254037844387076, 1.000000000000000000, 0.8660254037844387076, 1.000000000000000000, 0.8660254037844387076, 1.000000000000000000, 0.8660254037844387076, 1.000000000000000000, 0.8660254037844387076, 1.000000000000000000, 0.8660254037844387076, 1.000000000000000000, 0.8660254037844387076, 1.000000000000000000, 0.8660254037844387076, 1.000000000000000000, 0.8660254037844387076, 1.000000000000000000, 0.8660254037844387076, 1.000000000000000000, 0.8660254037844387076, 1.000000000000000000, 0.8660254037844387076, 1.000000000000000000, 0.8660254037844387076, 1.000000000000000000, 0.8660254037844387076, 1.000000000000000000, 0.8660254037844387076, 1.000000000000000000, 0.8660254037844387076, 1.000000000000000000, 0.8660254037844387076, 1.000000000000000000, 0.8660254037844387076, 1.000000000000000000, 0.8660254037844387076, 1.000000000000000000, 0.8660254037844387076, 1.000000000000000000, 0.8660254037844387076, 1.000000000000000000, 0.8660254037844387076, 1.000000000000000000, 0.8660254037844387076, 1.000000000000000000, 0.8660254037844387076, 1.000000000000000000, 0.8660254037844387076, 1.000000000000000000, 0.8660254037844387076, 1.000000000000000000, 0.8660254037844387076, 1.000000000000000000, 0.8660254037844387076, 1.000000000000000000, 0.8660254037844387076, 1.000000000000000000, 0.8660254037844387076, 1.000000000000000000, 0.8660254037844387076, 1.000000000000000000, 0.8660254037844387076, 1.000000000000000000, 0.8660254037844387076, 1.000000000000000000, 0.8660254037844387076, 1.000000000000000000, 0.8660254037844387076, 1.000000000000000000, 0.8660254037844387076, 1.000000000000000000, 0.8660254037844387076, 1.000000000000000000, 0.8660254037844387076, 1.000000000000000000, 0.8660254037844387076, 1.000000000000000000, 0.8660254037844387076, 1.000000000000000000, 0.8660254037844387076, 1.000000000000000000, 0.8660254037844387076, 1.000000000000000000, 0.8660254037844387076, 1.000000000000000000, 0.8660254037844387076, 1.000000000000000000, 0.8660254037844387076, 1.000000000000000000, 0.8660254037844387076, 1.000000000000000000, 0.8660254037844387076, 1.000000000000000000, 0.8660254037844387076, 1.000000000000000000, 0.8660254037844387076, 1.000000000000000000, 0.8660254037844387076, 1.000000000000000000, 0.8660254037844387076, 1.000000000000000000, 0.8660254037844387076, 1.000000000000000000, 0.8660254037844387076, 1.000000000000000000, 0.8660254037844387076, 1.000000000000000000, 0.8660254037844387076, 1.000000000000000000, 0.8660254037844387076, 1.000000000000000000, 0.8660254037844387076, 1.000000000000000000, 0.8660254037844387076, 1.000000000000000000, 0.8660254037844387076, 1.000000000000000000, 0.8660254037844387076, 1.000000000000000000, 0.8660254037844387076, 1.000000000000000000, 0.8660254037844387076, 1.000000000000000000, 0.8660254037844387076, 1.000000000000000000, 0.8660254037844387076, 1.000000000000000000, 0.8660254037844387076, 1.000000000000000000, 0.8660254037844387076, 1.000000000000000000, 0.8660254037844387076, 1.000000000000000000, 0.8660254037844387076, 1.000000000000000000, 0.8660254037844387076, 1.000000000000000000, 0.8660254037844387076, 1.000000000000000000, 0.8660254037844387076, 1.000000000000000000, 0.8660254037844387076, 1.000000000000000000, 0.8660254037844387076, 1.000000000000000000, 0.8660254037844387076, 1.000000000000000000, 0.8660254037844387076, 1.000000000000000000, 0.8660254037844387076, 1.000000000000000000, 0.8660254037844387076, 1.000000000000000000, 0.8660254037844387076, 1.000000000000000000, 0.8660254037844387076, 1.000000000000000000, 0.8660254037844387076, 1.000000000000000000, 0.8660254037844387076, 1.000000000000000000, 0.8660254037844387076, 1.000000000000000000, 0.8660254037844387076, 1.000000000000000000, 0.8660254037844387076, 1.000000000000000000, 0.8660254037844387076, 1.000000000000000000, 0.8660254037844387076, 1.000000000000000000, 0.8660254037844387076, 1.000000000000000000, 0.8660254037844387076, 1.000000000000000000, 0.8660254037844387076, 1.000000000000000000, 0.8660254037844387076, 1.000000000000000000, 0.8660254037844387076, 1.000000000000000000, 0.8660254037844387076, 1.000000000000000000, 0.8660254037844387076, 1.000000000000000000, 0.8660254037844387076, 1.000000000000000000, 0.8660254037844387076, 1.000000000000000000, 0.8660254037844387076, 1.000000000000000000, 0.8660254037844387076, 1.000000000000000000, 0.8660254037844387076, 1.000000000000000000, 0.8660254037844387076, 1.000000000000000000, 0.8660254037844387076, 1.000000000000000000, 0.8660254037844387076, 1.000000000000000000, 0.8660254037844387076, 1.000000000000000000, 0.8660254037844387076, 1.000000000000000000, 0.8660254037844387076, 1.000000000000000000, 0.8660254037844387076, 1.000000000000000000, 0.8660254037844387076, 1.000000000000000000, 0.8660254037844387076, 1.000000000000000000, 0.8660254037844387076, 1.000000000000000000, 0.8660254037844387076, 1.000000000000000000, 0.8660254037844387076, 1.000000000000000000, 0.8660254037844387076, 1.000000000000000000, 0.8660254037844387076, 1.000000000000000000, 0.8660254037844387076, 1.000000000000000000, 0.8660254037844387076, 1.000000000000000000, 0.8660254037844387076, 1.000000000000000000, 0.8660254037844387076, 1.000000000000000000, 0.8660254037844387076, 1.000000000000000000, 0.8660254037844387076, 1.000000000000000000, 0.8660254037844387076, 1.000000000000000000, 0.8660254037844387076, 1.000000000000000000, 0.8660254037844387076, 1.000000000000000000, 0.8660254037844387076, 1.000000000000000000, 0.8660254037844387076, 1.000000000000000000, 0.8660254037844387076, 1.000000000000000000, 0.8660254037844387076, 1.000000000000000000, 0.8660254037844387076, 1.000000000000000000, 0.8660254037844387076, 1.000000000000000000, 0.8660254037844387076, 1.000000000000000000, 0.8660254037844387076, 1.000000000000000000, 0.8660254037844387076, 1.000000000000000000, 0.8660254037844387076, 1.000000000000000000, 0.8660254037844387076, 1.000000000000000000, 0.8660254037844387076, 1.000000000000000000, 0.8660254037844387076, 1.000000000000000000, 0.8660254037844387076, 1.000000000000000000, 0.8660254037844387076, 1.000000000000000000, 0.8660254037844387076, 1.000000000000000000, 0.8660254037844387076, 1.000000000000000000, 0.8660254037844387076, 1.000000000000000000, 0.8660254037844387076, 1.000000000000000000, 0.8660254037844387076, 1.000000000000000000, 0.8660254037844387076, 1.000000000000000000, 0.8660254037844387076, 1.000000000000000000, 0.8660254037844387076, 1.000000000000000000, 0.8660254037844387076, 1.000000000000000000, 0.8660254037844387076, 1.000000000000000000, 0.8660254037844387076, 1.000000000000000000, 0.8660254037844387076, 1.000000000000000000, 0.8660254037844387076, 1.000000000000000000, 0.8660254037844387076, 1.000000000000000000, 0.8660254037844387076, 1.000000000000000000, 0.8660254037844387076, 1.000000000000000000, 0.8660254037844387076, 1.000000000000000000, 0.8660254037844387076, 1.000000000000000000, 0.8660254037844387076, 1.000000000000000000, 0.8660254037844387076, 1.000000000000000000, 0.8660254037844387076, 1.000000000000000000, 0.8660254037844387076, 1.000000000000000000, 0.8660254037844387076, 1.000000000000000000, 0.8660254037844387076, 1.000000000000000000, 0.8660254037844387076, 1.000000000000000000, 0.8660254037844387076, 1.000000000000000000, 0.8660254037844387076, 1.000000000000000000, 0.8660254037844387076, 1.000000000000000000, 0.8660254037844387076, 1.000000000000000000, 0.8660254037844387076, 1.000000000000000000, 0.8660254037844387076, 1.000000000000000000, 0.8660254037844387076, 1.000000000000000000, 0.8660254037844387076, 1.000000000000000000, 0.8660254037844387076, 1.000000000000000000, 0.8660254037844387076, 1.000000000000000000, 0.8660254037844387076, 1.000000000000000000, 0.8660254037844387076, 1.000000000000000000, 0.8660254037844387076, 1.000000000000000000, 0.8660254037844387076, 1.000000000000000000, 0.8660254037844387076, 1.000000000000000000, 0.8660254037844387076, 1.000000000000000000, 0.8660254037844387076, 1.000000000000000000, 0.8660254037844387076, 1.000000000000000000, 0.8660254037844387076, 1.000000000000000000, 0.8660254037844387076, 1.000000000000000000, 0.8660254037844387076, 1.000000000000000000, 0.8660254037844387076, 1.000000000000000000, 0.8660254037844387076, 1.000000000000000000, 0.8660254037844387076, 1.000000000000000000, 0.8660254037844387076, 1.000000000000000000, 0.8660254037844387076, 1.000000000000000000, 0.8660254037844387076, 1.000000000000000000, 0.8660254037844387076, 1.000000000000000000, 0.8660254037844387076, 1.000000000000000000, 0.8660254037844387076, 1.000000000000000000, 0.8660254037844387076, 1.000000000000000000, 0.8660254037844387076, 1.000000000000000000, 0.8660254037844387076, 1.000000000000000000, 0.8660254037844387076, 1.000000000000000000, 0.8660254037844387076, 1.000000000000000000, 0.8660254037844387076, 1.000000000000000000, 0.8660254037844387076, 1.000000000000000000, 0.8660254037844387076, 1.000000000000000000, 0.8660254037844387076, 1.000000000000000000, 0.8660254037844387076, 1.000000000000000000, 0.8660254037844387076, 1.000000000000000000, 0.8660254037844387076, 1.000000000000000000, 0.8660254037844387076, 1.000000000000000000, 0.8660254037844387076, 1.000000000000000000, 0.8660254037844387076, 1.000000000000000000, 0.8660254037844387076, 1.000000000000000000, 0.8660254037844387076, 1.000000000000000000, 0.8660254037844387076, 1.000000000000000000, 0.8660254037844387076, 1.000000000000000000, 0.8660254037844387076, 1.000000000000000000, 0.8660254037844387076, 1.000000000000000000, 0.8660254037844387076, 1.000000000000000000, 0.8660254037844387076, 1.000000000000000000, 0.8660254037844387076, 1.000000000000000000, 0.8660254037844387076, 1.000000000000000000, 0.8660254037844387076, 1.000000000000000000, 0.8660254037844387076, 1.000000000000000000, 0.8660254037844387076, 1.000000000000000000, 0.8660254037844387076, 1.000000000000000000, 0.8660254037844387076, 1.000000000000000000, 0.8660254037844387076, 1.000000000000000000, 0.8660254037844387076, 1.000000000000000000, 0.8660254037844387076, 1.000000000000000000, 0.8660254037844387076, 1.000000000000000000, 0.8660254037844387076, 1.000000000000000000, 0.8660254037844387076, 1.000000000000000000, 0.8660254037844387076, 1.000000000000000000, 0.8660254037844387076, 1.000000000000000000, 0.8660254037844387076, 1.000000000000000000, 0.8660254037844387076, 1.000000000000000000, 0.8660254037844387076, 1.000000000000000000, 0.8660254037844387076, 1.000000000000000000, 0.8660254037844387076, 1.000000000000000000, 0.8660254037844387076, 1.000000000000000000, 0.8660254037844387076, 1.000000000000000000, 0.8660254037844387076, 1.000000000000000000, 0.8660254037844387076, 1.000000000000000000, 0.8660254037844387076, 1.000000000000000000, 0.8660254037844387076, 1.000000000000000000, 0.8660254037844387076, 1.000000000000000000, 0.8660254037844387076, 1.000000000000000000, 0.8660254037844387076, 1.000000000000000000, 0.8660254037844387076, 1.000000000000000000, 0.8660254037844387076, 1.000000000000000000, 0.8660254037844387076, 1.000000000000000000, 0.8660254037844387076, 1.000000000000000000, 0.8660254037844387076, 1.000000000000000000, 0.8660254037844387076, 1.000000000000000000, 0.8660254037844387076, 1.000000000000000000, 0.8660254037844387076, 1.000000000000000000, 0.8660254037844387076, 1.000000000000000000, 0.8660254037844387076, 1.000000000000000000, 0.8660254037844387076, 1.000000000000000000, 0.8660254037844387076, 1.000000000000000000, 0.8660254037844387076, 1.000000000000000000, 0.8660254037844387076, 1.000000000000000000, 0.8660254037844387076, 1.000000000000000000, 0.8660254037844387076, 1.000000000000000000, 0.8660254037844387076, 1.000000000000000000, 0.8660254037844387076, 1.000000000000000000, 0.8660254037844387076, 1.000000000000000000, 0.8660254037844387076, 1.000000000000000000, 0.8660254037844387076, 1.000000000000000000, 0.8660254037844387076, 1.000000000000000000, 0.8660254037844387076, 1.000000000000000000, 0.8660254037844387076, 1.000000000000000000, 0.8660254037844387076, 1.000000000000000000, 0.8660254037844387076, 1.000000000000000000, 0.8660254037844387076, 1.000000000000000000, 0.8660254037844387076, 1.000000000000000000, 0.8660254037844387076, 1.000000000000000000, 0.8660254037844387076, 1.000000000000000000, 0.8660254037844387076, 1.000000000000000000, 0.8660254037844387076, 1.000000000000000000, 0.8660254037844387076, 1.000000000000000000, 0.8660254037844387076, 1.000000000000000000, 0.8660254037844387076, 1.000000000000000000, 0.8660254037844387076, 1.000000000000000000, 0.8660254037844387076, 1.000000000000000000, 0.8660254037844387076, 1.000000000000000000, 0.8660254037844387076, 1.000000000000000000, 0.8660254037844387076, 1.000000000000000000, 0.8660254037844387076, 1.000000000000000000, 0.8660254037844387076, 1.000000000000000000, 0.8660254037844387076, 1.000000000000000000, 0.8660254037844387076, 1.000000000000000000, 0.8660254037844387076, 1.000000000000000000, 0.8660254037844387076, 1.000000000000000000, 0.8660254037844387076, 1.000000000000000000, 0.8660254037844387076, 1.000000000000000000, 0.8660254037844387076, 1.000000000000000000, 0.8660254037844387076, 1.000000000000000000, 0.8660254037844387076, 1.000000000000000000, 0.8660254037844387076, 1.000000000000000000, 0.8660254037844387076, 1.000000000000000000, 0.8660254037844387076, 1.000000000000000000, 0.8660254037844387076, 1.000000000000000000, 0.8660254037844387076, 1.000000000000000000, 0.8660254037844387076, 1.000000000000000000, 0.8660254037844387076, 1.000000000000000000, 0.8660254037844387076, 1.000000000000000000, 0.8660254037844387076, 1.000000000000000000, 0.8660254037844387076, 1.000000000000000000, 0.8660254037844387076, 1.000000000000000000, 0.8660254037844387076, 1.000000000000000000, 0.8660254037844387076, 1.000000000000000000, 0.8660254037844387076, 1.000000000000000000, 0.8660254037844387076, 1.000000000000000000, 0.8660254037844387076, 1.000000000000000000, 0.8660254037844387076, 1.000000000000000000, 0.8660254037844387076, 1.000000000000000000, 0.8660254037844387076, 1.000000000000000000, 0.8660254037844387076, 1.000000000000000000, 0.8660254037844387076, 1.000000000000000000, 0.8660254037844387076, 1.000000000000000000, 0.8660254037844387076, 1.000000000000000000, 0.8660254037844387076, 1.000000000000000000, 0.8660254037844387076, 1.000000000000000000, 0.8660254037844387076, 1.000000000000000000, 0.8660254037844387076, 1.000000000000000000, 0.8660254037844387076, 1.000000000000000000, 0.8660254037844387076, 1.000000000000000000, 0.8660254037844387076, 1.000000000000000000, 0.8660254037844387076, 1.000000000000000000, 0.8660254037844387076, 1.000000000000000000, 0.8660254037844387076, 1.000000000000000000, 0.8660254037844387076, 1.000000000000000000, 0.8660254037844387076, 1.000000000000000000, 0.8660254037844387076, 1.000000000000000000, 0.8660254037844387076, 1.000000000000000000, 0.8660254037844387076, 1.000000000000000000, 0.8660254037844387076, 1.000000000000000000, 0.8660254037844387076, 1.000000000000000000, 0.8660254037844387076, 1.000000000000000000, 0.8660254037844387076, 1.000000000000000000, 0.8660254037844387076, 1.000000000000000000, 0.8660254037844387076, 1.000000000000000000, 0.8660254037844387076, 1.000000000000000000, 0.8660254037844387076, 1.000000000000000000, 0.8660254037844387076, 1.000000000000000000, 0.8660254037844387076, 1.000000000000000000, 0.8660254037844387076, 1.000000000000000000, 0.8660254037844387076, 1.000000000000000000, 0.8660254037844387076, 1.000000000000000000, 0.8660254037844387076, 1.000000000000000000, 0.8660254037844387076, 1.000000000000000000, 0.8660254037844387076, 1.000000000000000000, 0.8660254037844387076, 1.000000000000000000, 0.8660254037844387076, 1.000000000000000000, 0.8660254037844387076, 1.000000000000000000, 0.8660254037844387076, 1.000000000000000000, 0.8660254037844387076, 1.000000000000000000, 0.8660254037844387076, 1.000000000000000000, 0.8660254037844387076, 1.000000000000000000, 0.8660254037844387076, 1.000000000000000000, 0.8660254037844387076, 1.000000000000000000, 0.8660254037844387076, 1.000000000000000000, 0.8660254037844387076, 1.000000000000000000, 0.8660254037844387076, 1.000000000000000000, 0.8660254037844387076, 1.000000000000000000, 0.8660254037844387076, 1.000000000000000000, 0.8660254037844387076, 1.000000000000000000, 0.8660254037844387076, 1.000000000000000000, 0.8660254037844387076, 1.000000000000000000, 0.8660254037844387076, 1.000000000000000000, 0.8660254037844387076, 1.000000000000000000, 0.8660254037844387076, 1.000000000000000000, 0.8660254037844387076, 1.000000000000000000, 0.8660254037844387076, 1.000000000000000000, 0.8660254037844387076, 1.000000000000000000, 0.8660254037844387076, 1.000000000000000000, 0.8660254037844387076, 1.000000000000000000, 0.8660254037844387076, 1.000000000000000000, 0.8660254037844387076, 1.000000000000000000, 0.8660254037844387076, 1.000000000000000000, 0.8660254037844387076, 1.000000000000000000, 0.8660254037844387076, 1.000000000000000000, 0.8660254037844387076, 1.000000000000000000, 0.8660254037844387076, 1.000000000000000000, 0.8660254037844387076, 1.000000000000000000, 0.8660254037844387076, 1.000000000000000000, 0.8660254037844387076, 1.000000000000000000, 0.8660254037844387076, 1.000000000000000000, 0.8660254037844387076, 1.000000000000000000, 0.8660254037844387076, 1.000000000000000000, 0.8660254037844387076, 1.000000000000000000, 0.8660254037844387076, 1.000000000000000000, 0.8660254037844387076, 1.000000000000000000, 0.8660254037844387076, 1.000000000000000000, 0.8660254037844387076, 1.000000000000000000, 0.8660254037844387076, 1.000000000000000000, 0.8660254037844387076, 1.000000000000000000, 0.8660254037844387076, 1.000000000000000000, 0.8660254037844387076, 1.000000000000000000, 0.8660254037844387076, 1.000000000000000000, 0.8660254037844387076, 1.000000000000000000, 0.8660254037844387076, 1.000000000000000000, 0.8660254037844387076, 1.000000000000000000, 0.8660254037844387076, 1.000000000000000000, 0.8660254037844387076, 1.000000000000000000, 0.8660254037844387076, 1.000000000000000000, 0.8660254037844387076, 1.000000000000000000, 0.8660254037844387076, 1.000000000000000000, 0.8660254037844387076, 1.000000000000000000, 0.8660254037844387076, 1.000000000000000000, 0.8660254037844387076, 1.000000000000000000, 0.8660254037844387076, 1.000000000000000000, 0.8660254037844387076, 1.000000000000000000, 0.8660254037844387076, 1.000000000000000000, 0.8660254037844387076, 1.000000000000000000, 0.8660254037844387076, 1.000000000000000000, 0.8660254037844387076, 1.000000000000000000, 0.8660254037844387076, 1.000000000000000000, 0.8660254037844387076, 1.000000000000000000, 0.8660254037844387076, 1.000000000000000000, 0.8660254037844387076, 1.000000000000000000, 0.8660254037844387076, 1.000000000000000000, 0.8660254037844387076, 1.000000000000000000, 0.8660254037844387076, 1.000000000000000000, 0.8660254037844387076, 1.000000000000000000, 0.8660254037844387076, 1.000000000000000000, 0.8660254037844387076, 1.000000000000000000, 0.8660254037844387076, 1.000000000000000000, 0.8660254037844387076, 1.000000000000000000, 0.8660254037844387076, 1.000000000000000000, 0.8660254037844387076, 1.000000000000000000, 0.8660254037844387076, 1.000000000000000000, 0.8660254037844387076, 1.000000000000000000, 0.8660254037844387076, 1.000000000000000000, 0.8660254037844387076, 1.000000000000000000, 0.8660254037844387076, 1.000000000000000000, 0.8660254037844387076, 1.000000000000000000, 0.8660254037844387076, 1.000000000000000000, 0.8660254037844387076, 1.000000000000000000, 0.8660254037844387076, 1.000000000000000000, 0.8660254037844387076, 1.000000000000000000, 0.8660254037844387076, 1.000000000000000000, 0.8660254037844387076, 1.000000000000000000, 0.8660254037844387076, 1.000000000000000000, 0.8660254037844387076, 1.000000000000000000, 0.8660254037844387076, 1.000000000000000000, 0.8660254037844387076, 1.000000000000000000, 0.8660254037844387076, 1.000000000000000000, 0.8660254037844387076, 1.000000000000000000, 0.8660254037844387076, 1.000000000000000000, 0.8660254037844387076, 1.000000000000000000, 0.8660254037844387076, 1.000000000000000000, 0.8660254037844387076, 1.000000000000000000, 0.8660254037844387076, 1.000000000000000000, 0.8660254037844387076, 1.000000000000000000, 0.8660254037844387076, 1.000000000000000000, 0.8660254037844387076, 1.000000000000000000, 0.8660254037844387076, 1.000000000000000000, 0.8660254037844387076, 1.000000000000000000, 0.8660254037844387076, 1.000000000000000000, 0.8660254037844387076, 1.000000000000000000, 0.8660254037844387076, 1.000000000000000000, 0.8660254037844387076, 1.000000000000000000, 0.8660254037844387076, 1.000000000000000000, 0.8660254037844387076, 1.000000000000000000, 0.8660254037844387076, 1.000000000000000000, 0.8660254037844387076, 1.000000000000000000, 0.8660254037844387076, 1.000000000000000000, 0.8660254037844387076, 1.000000000000000000, 0.8660254037844387076, 1.000000000000000000, 0.8660254037844387076, 1.000000000000000000, 0.8660254037844387076, 1.000000000000000000, 0.8660254037844387076, 1.000000000000000000, 0.8660254037844387076, 1.000000000000000000, 0.8660254037844387076, 1.000000000000000000, 0.8660254037844387076, 1.000000000000000000, 0.8660254037844387076, 1.000000000000000000, 0.8660254037844387076, 1.000000000000000000, 0.8660254037844387076, 1.000000000000000000, 0.8660254037844387076, 1.000000000000000000, 0.8660254037844387076, 1.000000000000000000, 0.8660254037844387076, 1.000000000000000000, 0.8660254037844387076, 1.000000000000000000, 0.8660254037844387076, 1.000000000000000000, 0.8660254037844387076, 1.000000000000000000, 0.8660254037844387076, 1.000000000000000000, 0.8660254037844387076, 1.000000000000000000, 0.8660254037844387076, 1.000000000000000000, 0.8660254037844387076, 1.000000000000000000, 0.8660254037844387076, 1.000000000000000000, 0.8660254037844387076, 1.000000000000000000, 0.8660254037844387076, 1.000000000000000000, 0.8660254037844387076, 1.000000000000000000, 0.8660254037844387076, 1.000000000000000000, 0.8660254037844387076, 1.000000000000000000, 0.8660254037844387076, 1.000000000000000000, 0.8660254037844387076, 1.000000000000000000, 0.8660254037844387076, 1.000000000000000000, 0.8660254037844387076, 1.000000000000000000, 0.8660254037844387076, 1.000000000000000000, 0.8660254037844387076, 1.000000000000000000, 0.8660254037844387076, 1.000000000000000000, 0.8660254037844387076, 1.000000000000000000, 0.8660254037844387076, 1.000000000000000000, 0.8660254037844387076, 1.000000000000000000, 0.8660254037844387076, 1.000000000000000000),
 ( 1.000000000000000000, 0.8660254037844387076, 1.000000000000000000, 0.8660254037844387076, 1.000000000000000000, 0.8660254037844387076, 1.000000000000000000, 0.8660254037844387076, 1.000000000000000000, 0.8660254037844387076, 1.000000000000000000, 0.8660254037844387076, 1.000000000000000000, 0.8660254037844387076, 1.000000000000000000, 0.8660254037844387076, 1.000000000000000000, 0.8660254037844387076, 1.000000000000000000, 0.8660254037844387076, 1.000000000000000000, 0.8660254037844387076, 1.000000000000000000, 0.8660254037844387076, 1.000000000000000000, 0.8660254037844387076, 1.000000000000000000, 0.8660254037844387076, 1.000000000000000000, 0.8660254037844387076, 1.000000000000000000, 0.8660254037844387076, 1.000000000000000000, 0.8660254037844387076, 1.000000000000000000, 0.8660254037844387076, 1.000000000000000000, 0.8660254037844387076, 1.000000000000000000, 0.8660254037844387076, 1.000000000000000000, 0.8660254037844387076, 1.000000000000000000, 0.8660254037844387076, 1.000000000000000000, 0.8660254037844387076, 1.000000000000000000, 0.8660254037844387076, 1.000000000000000000, 0.8660254037844387076, 1.000000000000000000, 0.8660254037844387076, 1.000000000000000000, 0.8660254037844387076, 1.000000000000000000, 0.8660254037844387076, 1.000000000000000000, 0.8660254037844387076, 1.000000000000000000, 0.8660254037844387076, 1.000000000000000000, 0.8660254037844387076, 1.000000000000000000, 0.8660254037844387076, 1.000000000000000000, 0.8660254037844387076, 1.000000000000000000, 0.8660254037844387076, 1.000000000000000000, 0.8660254037844387076, 1.000000000000000000, 0.8660254037844387076, 1.000000000000000000, 0.8660254037844387076, 1.000000000000000000, 0.8660254037844387076, 1.000000000000000000, 0.8660254037844387076, 1.000000000000000000, 0.8660254037844387076, 1.000000000000000000, 0.8660254037844387076, 1.000000000000000000, 0.8660254037844387076, 1.000000000000000000, 0.8660254037844387076, 1.000000000000000000, 0.8660254037844387076, 1.000000000000000000, 0.8660254037844387076, 1.000000000000000000, 0.8660254037844387076, 1.000000000000000000, 0.8660254037844387076, 1.000000000000000000, 0.8660254037844387076, 1.000000000000000000, 0.8660254037844387076, 1.000000000000000000, 0.8660254037844387076, 1.000000000000000000, 0.8660254037844387076, 1.000000000000000000, 0.8660254037844387076, 1.000000000000000000, 0.8660254037844387076, 1.000000000000000000, 0.8660254037844387076, 1.000000000000000000, 0.8660254037844387076, 1.000000000000000000, 0.8660254037844387076, 1.000000000000000000, 0.8660254037844387076, 1.000000000000000000, 0.8660254037844387076, 1.000000000000000000, 0.8660254037844387076, 1.000000000000000000, 0.8660254037844387076, 1.000000000000000000, 0.8660254037844387076, 1.000000000000000000, 0.8660254037844387076, 1.000000000000000000, 0.8660254037844387076, 1.000000000000000000, 0.8660254037844387076, 1.000000000000000000, 0.8660254037844387076, 1.000000000000000000, 0.8660254037844387076, 1.000000000000000000, 0.8660254037844387076, 1.000000000000000000, 0.8660254037844387076, 1.000000000000000000, 0.8660254037844387076, 1.000000000000000000, 0.8660254037844387076, 1.000000000000000000, 0.8660254037844387076, 1.000000000000000000, 0.8660254037844387076, 1.000000000000000000, 0.8660254037844387076, 1.000000000000000000, 0.8660254037844387076, 1.000000000000000000, 0.8660254037844387076, 1.000000000000000000, 0.8660254037844387076, 1.000000000000000000, 0.8660254037844387076, 1.000000000000000000, 0.8660254037844387076, 1.000000000000000000, 0.8660254037844387076, 1.000000000000000000, 0.8660254037844387076, 1.000000000000000000, 0.8660254037844387076, 1.000000000000000000, 0.8660254037844387076, 1.000000000000000000, 0.8660254037844387076, 1.000000000000000000, 0.8660254037844387076, 1.000000000000000000, 0.8660254037844387076, 1.000000000000000000, 0.8660254037844387076, 1.000000000000000000, 0.8660254037844387076, 1.000000000000000000, 0.8660254037844387076, 1.000000000000000000, 0.8660254037844387076, 1.000000000000000000, 0.8660254037844387076, 1.000000000000000000, 0.8660254037844387076, 1.000000000000000000, 0.8660254037844387076, 1.000000000000000000, 0.8660254037844387076, 1.000000000000000000, 0.8660254037844387076, 1.000000000000000000, 0.8660254037844387076, 1.000000000000000000, 0.8660254037844387076, 1.000000000000000000, 0.8660254037844387076, 1.000000000000000000, 0.8660254037844387076, 1.000000000000000000, 0.8660254037844387076, 1.000000000000000000, 0.8660254037844387076, 1.000000000000000000, 0.8660254037844387076, 1.000000000000000000, 0.8660254037844387076, 1.000000000000000000, 0.8660254037844387076, 1.000000000000000000, 0.8660254037844387076, 1.000000000000000000, 0.8660254037844387076, 1.000000000000000000, 0.8660254037844387076, 1.000000000000000000, 0.8660254037844387076, 1.000000000000000000, 0.8660254037844387076, 1.000000000000000000, 0.8660254037844387076, 1.000000000000000000, 0.8660254037844387076, 1.000000000000000000, 0.8660254037844387076, 1.000000000000000000, 0.8660254037844387076, 1.000000000000000000, 0.8660254037844387076, 1.000000000000000000, 0.8660254037844387076, 1.000000000000000000, 0.8660254037844387076, 1.000000000000000000, 0.8660254037844387076, 1.000000000000000000, 0.8660254037844387076, 1.000000000000000000, 0.8660254037844387076, 1.000000000000000000, 0.8660254037844387076, 1.000000000000000000, 0.8660254037844387076, 1.000000000000000000, 0.8660254037844387076, 1.000000000000000000, 0.8660254037844387076, 1.000000000000000000, 0.8660254037844387076, 1.000000000000000000, 0.8660254037844387076, 1.000000000000000000, 0.8660254037844387076, 1.000000000000000000, 0.8660254037844387076, 1.000000000000000000, 0.8660254037844387076, 1.000000000000000000, 0.8660254037844387076, 1.000000000000000000, 0.8660254037844387076, 1.000000000000000000, 0.8660254037844387076, 1.000000000000000000, 0.8660254037844387076, 1.000000000000000000, 0.8660254037844387076, 1.000000000000000000, 0.8660254037844387076, 1.000000000000000000, 0.8660254037844387076, 1.000000000000000000, 0.8660254037844387076, 1.000000000000000000, 0.8660254037844387076, 1.000000000000000000, 0.8660254037844387076, 1.000000000000000000, 0.8660254037844387076, 1.000000000000000000, 0.8660254037844387076, 1.000000000000000000, 0.8660254037844387076, 1.000000000000000000, 0.8660254037844387076, 1.000000000000000000, 0.8660254037844387076, 1.000000000000000000, 0.8660254037844387076, 1.000000000000000000, 0.8660254037844387076, 1.000000000000000000, 0.8660254037844387076, 1.000000000000000000, 0.8660254037844387076, 1.000000000000000000, 0.8660254037844387076, 1.000000000000000000, 0.8660254037844387076, 1.000000000000000000, 0.8660254037844387076, 1.000000000000000000, 0.8660254037844387076, 1.000000000000000000, 0.8660254037844387076, 1.000000000000000000, 0.8660254037844387076, 1.000000000000000000, 0.8660254037844387076, 1.000000000000000000, 0.8660254037844387076, 1.000000000000000000, 0.8660254037844387076, 1.000000000000000000, 0.8660254037844387076, 1.000000000000000000, 0.8660254037844387076, 1.000000000000000000, 0.8660254037844387076, 1.000000000000000000, 0.8660254037844387076, 1.000000000000000000, 0.8660254037844387076, 1.000000000000000000, 0.8660254037844387076, 1.000000000000000000, 0.8660254037844387076, 1.000000000000000000, 0.8660254037844387076, 1.000000000000000000, 0.8660254037844387076, 1.000000000000000000, 0.8660254037844387076, 1.000000000000000000, 0.8660254037844387076, 1.000000000000000000, 0.8660254037844387076, 1.000000000000000000, 0.8660254037844387076, 1.000000000000000000, 0.8660254037844387076, 1.000000000000000000, 0.8660254037844387076, 1.000000000000000000, 0.8660254037844387076, 1.000000000000000000, 0.8660254037844387076, 1.000000000000000000, 0.8660254037844387076, 1.000000000000000000, 0.8660254037844387076, 1.000000000000000000, 0.8660254037844387076, 1.000000000000000000, 0.8660254037844387076, 1.000000000000000000, 0.8660254037844387076, 1.000000000000000000, 0.8660254037844387076, 1.000000000000000000, 0.8660254037844387076, 1.000000000000000000, 0.8660254037844387076, 1.000000000000000000, 0.8660254037844387076, 1.000000000000000000, 0.8660254037844387076, 1.000000000000000000, 0.8660254037844387076, 1.000000000000000000, 0.8660254037844387076, 1.000000000000000000, 0.8660254037844387076, 1.000000000000000000, 0.8660254037844387076, 1.000000000000000000, 0.8660254037844387076, 1.000000000000000000, 0.8660254037844387076, 1.000000000000000000, 0.8660254037844387076, 1.000000000000000000, 0.8660254037844387076, 1.000000000000000000, 0.8660254037844387076, 1.000000000000000000, 0.8660254037844387076, 1.000000000000000000, 0.8660254037844387076, 1.000000000000000000, 0.8660254037844387076, 1.000000000000000000, 0.8660254037844387076, 1.000000000000000000, 0.8660254037844387076, 1.000000000000000000, 0.8660254037844387076, 1.000000000000000000, 0.8660254037844387076, 1.000000000000000000, 0.8660254037844387076, 1.000000000000000000, 0.8660254037844387076, 1.000000000000000000, 0.8660254037844387076, 1.000000000000000000, 0.8660254037844387076, 1.000000000000000000, 0.8660254037844387076, 1.000000000000000000, 0.8660254037844387076, 1.000000000000000000, 0.8660254037844387076, 1.000000000000000000, 0.8660254037844387076, 1.000000000000000000, 0.8660254037844387076, 1.000000000000000000, 0.8660254037844387076, 1.000000000000000000, 0.8660254037844387076, 1.000000000000000000, 0.8660254037844387076, 1.000000000000000000, 0.8660254037844387076, 1.000000000000000000, 0.8660254037844387076, 1.000000000000000000, 0.8660254037844387076, 1.000000000000000000, 0.8660254037844387076, 1.000000000000000000, 0.8660254037844387076, 1.000000000000000000, 0.8660254037844387076, 1.000000000000000000, 0.8660254037844387076, 1.000000000000000000, 0.8660254037844387076, 1.000000000000000000, 0.8660254037844387076, 1.000000000000000000, 0.8660254037844387076, 1.000000000000000000, 0.8660254037844387076, 1.000000000000000000, 0.8660254037844387076, 1.000000000000000000, 0.8660254037844387076, 1.000000000000000000, 0.8660254037844387076, 1.000000000000000000, 0.8660254037844387076, 1.000000000000000000, 0.8660254037844387076, 1.000000000000000000, 0.8660254037844387076, 1.000000000000000000, 0.8660254037844387076, 1.000000000000000000, 0.8660254037844387076, 1.000000000000000000, 0.8660254037844387076, 1.000000000000000000, 0.8660254037844387076, 1.000000000000000000, 0.8660254037844387076, 1.000000000000000000, 0.8660254037844387076, 1.000000000000000000, 0.8660254037844387076, 1.000000000000000000, 0.8660254037844387076, 1.000000000000000000, 0.8660254037844387076, 1.000000000000000000, 0.8660254037844387076, 1.000000000000000000, 0.8660254037844387076, 1.000000000000000000, 0.8660254037844387076, 1.000000000000000000, 0.8660254037844387076, 1.000000000000000000, 0.8660254037844387076, 1.000000000000000000, 0.8660254037844387076, 1.000000000000000000, 0.8660254037844387076, 1.000000000000000000, 0.8660254037844387076, 1.000000000000000000, 0.8660254037844387076, 1.000000000000000000, 0.8660254037844387076, 1.000000000000000000, 0.8660254037844387076, 1.000000000000000000, 0.8660254037844387076, 1.000000000000000000, 0.8660254037844387076, 1.000000000000000000, 0.8660254037844387076, 1.000000000000000000, 0.8660254037844387076, 1.000000000000000000, 0.8660254037844387076, 1.000000000000000000, 0.8660254037844387076, 1.000000000000000000, 0.8660254037844387076, 1.000000000000000000, 0.8660254037844387076, 1.000000000000000000, 0.8660254037844387076, 1.000000000000000000, 0.8660254037844387076, 1.000000000000000000, 0.8660254037844387076, 1.000000000000000000, 0.8660254037844387076, 1.000000000000000000, 0.8660254037844387076, 1.000000000000000000, 0.8660254037844387076, 1.000000000000000000, 0.8660254037844387076, 1.000000000000000000, 0.8660254037844387076, 1.000000000000000000, 0.8660254037844387076, 1.000000000000000000, 0.8660254037844387076, 1.000000000000000000, 0.8660254037844387076, 1.000000000000000000, 0.8660254037844387076, 1.000000000000000000, 0.8660254037844387076, 1.000000000000000000, 0.8660254037844387076, 1.000000000000000000, 0.8660254037844387076, 1.000000000000000000, 0.8660254037844387076, 1.000000000000000000, 0.8660254037844387076, 1.000000000000000000, 0.8660254037844387076, 1.000000000000000000, 0.8660254037844387076, 1.000000000000000000, 0.8660254037844387076, 1.000000000000000000, 0.8660254037844387076, 1.000000000000000000, 0.8660254037844387076, 1.000000000000000000, 0.8660254037844387076, 1.000000000000000000, 0.8660254037844387076, 1.000000000000000000, 0.8660254037844387076, 1.000000000000000000, 0.8660254037844387076, 1.000000000000000000, 0.8660254037844387076, 1.000000000000000000, 0.8660254037844387076, 1.000000000000000000, 0.8660254037844387076, 1.000000000000000000, 0.8660254037844387076, 1.000000000000000000, 0.8660254037844387076, 1.000000000000000000, 0.8660254037844387076, 1.000000000000000000, 0.8660254037844387076, 1.000000000000000000, 0.8660254037844387076, 1.000000000000000000, 0.8660254037844387076, 1.000000000000000000, 0.8660254037844387076, 1.000000000000000000, 0.8660254037844387076, 1.000000000000000000, 0.8660254037844387076, 1.000000000000000000, 0.8660254037844387076, 1.000000000000000000, 0.8660254037844387076, 1.000000000000000000, 0.8660254037844387076, 1.000000000000000000, 0.8660254037844387076, 1.000000000000000000, 0.8660254037844387076, 1.000000000000000000, 0.8660254037844387076, 1.000000000000000000, 0.8660254037844387076, 1.000000000000000000, 0.8660254037844387076, 1.000000000000000000, 0.8660254037844387076, 1.000000000000000000, 0.8660254037844387076, 1.000000000000000000, 0.8660254037844387076, 1.000000000000000000, 0.8660254037844387076, 1.000000000000000000, 0.8660254037844387076, 1.000000000000000000, 0.8660254037844387076, 1.000000000000000000, 0.8660254037844387076, 1.000000000000000000, 0.8660254037844387076, 1.000000000000000000, 0.8660254037844387076, 1.000000000000000000, 0.8660254037844387076, 1.000000000000000000, 0.8660254037844387076, 1.000000000000000000, 0.8660254037844387076, 1.000000000000000000, 0.8660254037844387076, 1.000000000000000000, 0.8660254037844387076, 1.000000000000000000, 0.8660254037844387076, 1.000000000000000000, 0.8660254037844387076, 1.000000000000000000, 0.8660254037844387076, 1.000000000000000000, 0.8660254037844387076, 1.000000000000000000, 0.8660254037844387076, 1.000000000000000000, 0.8660254037844387076, 1.000000000000000000, 0.8660254037844387076, 1.000000000000000000, 0.8660254037844387076, 1.000000000000000000, 0.8660254037844387076, 1.000000000000000000, 0.8660254037844387076, 1.000000000000000000, 0.8660254037844387076, 1.000000000000000000, 0.8660254037844387076, 1.000000000000000000, 0.8660254037844387076, 1.000000000000000000, 0.8660254037844387076, 1.000000000000000000, 0.8660254037844387076, 1.000000000000000000, 0.8660254037844387076, 1.000000000000000000, 0.8660254037844387076, 1.000000000000000000, 0.8660254037844387076, 1.000000000000000000, 0.8660254037844387076, 1.000000000000000000, 0.8660254037844387076, 1.000000000000000000, 0.8660254037844387076, 1.000000000000000000, 0.8660254037844387076, 1.000000000000000000, 0.8660254037844387076, 1.000000000000000000, 0.8660254037844387076, 1.000000000000000000, 0.8660254037844387076, 1.000000000000000000, 0.8660254037844387076, 1.000000000000000000, 0.8660254037844387076, 1.000000000000000000, 0.8660254037844387076, 1.000000000000000000, 0.8660254037844387076, 1.000000000000000000, 0.8660254037844387076, 1.000000000000000000, 0.8660254037844387076, 1.000000000000000000, 0.8660254037844387076, 1.000000000000000000, 0.8660254037844387076, 1.000000000000000000, 0.8660254037844387076, 1.000000000000000000, 0.8660254037844387076, 1.000000000000000000, 0.8660254037844387076, 1.000000000000000000, 0.8660254037844387076, 1.000000000000000000, 0.8660254037844387076, 1.000000000000000000, 0.8660254037844387076, 1.000000000000000000, 0.8660254037844387076, 1.000000000000000000, 0.8660254037844387076, 1.000000000000000000, 0.8660254037844387076, 1.000000000000000000, 0.8660254037844387076, 1.000000000000000000, 0.8660254037844387076, 1.000000000000000000, 0.8660254037844387076, 1.000000000000000000, 0.8660254037844387076, 1.000000000000000000, 0.8660254037844387076, 1.000000000000000000, 0.8660254037844387076, 1.000000000000000000, 0.8660254037844387076, 1.000000000000000000, 0.8660254037844387076, 1.000000000000000000, 0.8660254037844387076, 1.000000000000000000, 0.8660254037844387076, 1.000000000000000000, 0.8660254037844387076, 1.000000000000000000, 0.8660254037844387076, 1.000000000000000000, 0.8660254037844387076, 1.000000000000000000, 0.8660254037844387076, 1.000000000000000000, 0.8660254037844387076, 1.000000000000000000, 0.8660254037844387076, 1.000000000000000000, 0.8660254037844387076, 1.000000000000000000, 0.8660254037844387076, 1.000000000000000000, 0.8660254037844387076, 1.000000000000000000, 0.8660254037844387076, 1.000000000000000000, 0.8660254037844387076, 1.000000000000000000, 0.8660254037844387076, 1.000000000000000000, 0.8660254037844387076, 1.000000000000000000, 0.8660254037844387076, 1.000000000000000000, 0.8660254037844387076, 1.000000000000000000, 0.8660254037844387076, 1.000000000000000000, 0.8660254037844387076, 1.000000000000000000, 0.8660254037844387076, 1.000000000000000000, 0.8660254037844387076, 1.000000000000000000, 0.8660254037844387076, 1.000000000000000000, 0.8660254037844387076, 1.000000000000000000, 0.8660254037844387076, 1.000000000000000000, 0.8660254037844387076, 1.000000000000000000, 0.8660254037844387076, 1.000000000000000000, 0.8660254037844387076, 1.000000000000000000, 0.8660254037844387076, 1.000000000000000000, 0.8660254037844387076, 1.000000000000000000, 0.8660254037844387076, 1.000000000000000000, 0.8660254037844387076, 1.000000000000000000, 0.8660254037844387076, 1.000000000000000000, 0.8660254037844387076, 1.000000000000000000, 0.8660254037844387076, 1.000000000000000000, 0.8660254037844387076, 1.000000000000000000, 0.8660254037844387076, 1.000000000000000000, 0.8660254037844387076, 1.000000000000000000, 0.8660254037844387076, 1.000000000000000000, 0.8660254037844387076, 1.000000000000000000, 0.8660254037844387076, 1.000000000000000000, 0.8660254037844387076, 1.000000000000000000, 0.8660254037844387076, 1.000000000000000000, 0.8660254037844387076, 1.000000000000000000, 0.8660254037844387076, 1.000000000000000000, 0.8660254037844387076, 1.000000000000000000, 0.8660254037844387076, 1.000000000000000000, 0.8660254037844387076, 1.000000000000000000, 0.8660254037844387076, 1.000000000000000000, 0.8660254037844387076, 1.000000000000000000, 0.8660254037844387076, 1.000000000000000000, 0.8660254037844387076, 1.000000000000000000, 0.8660254037844387076, 1.000000000000000000, 0.8660254037844387076, 1.000000000000000000, 0.8660254037844387076, 1.000000000000000000, 0.8660254037844387076, 1.000000000000000000, 0.8660254037844387076, 1.000000000000000000, 0.8660254037844387076, 1.000000000000000000, 0.8660254037844387076, 1.000000000000000000, 0.8660254037844387076, 1.000000000000000000, 0.8660254037844387076, 1.000000000000000000, 0.8660254037844387076, 1.000000000000000000, 0.8660254037844387076, 1.000000000000000000, 0.8660254037844387076, 1.000000000000000000, 0.8660254037844387076, 1.000000000000000000, 0.8660254037844387076, 1.000000000000000000, 0.8660254037844387076, 1.000000000000000000, 0.8660254037844387076, 1.000000000000000000, 0.8660254037844387076, 1.000000000000000000, 0.8660254037844387076, 1.000000000000000000, 0.8660254037844387076, 1.000000000000000000, 0.8660254037844387076, 1.000000000000000000, 0.8660254037844387076, 1.000000000000000000, 0.8660254037844387076, 1.000000000000000000, 0.8660254037844387076, 1.000000000000000000, 0.8660254037844387076, 1.000000000000000000, 0.8660254037844387076, 1.000000000000000000, 0.8660254037844387076, 1.000000000000000000, 0.8660254037844387076, 1.000000000000000000, 0.8660254037844387076, 1.000000000000000000, 0.8660254037844387076, 1.000000000000000000, 0.8660254037844387076, 1.000000000000000000, 0.8660254037844387076, 1.000000000000000000, 0.8660254037844387076, 1.000000000000000000, 0.8660254037844387076, 1.000000000000000000, 0.8660254037844387076, 1.000000000000000000, 0.8660254037844387076, 1.000000000000000000, 0.8660254037844387076, 1.000000000000000000, 0.8660254037844387076, 1.000000000000000000, 0.8660254037844387076, 1.000000000000000000, 0.8660254037844387076, 1.000000000000000000, 0.8660254037844387076, 1.000000000000000000, 0.8660254037844387076, 1.000000000000000000, 0.8660254037844387076, 1.000000000000000000, 0.8660254037844387076, 1.000000000000000000, 0.8660254037844387076, 1.000000000000000000, 0.8660254037844387076, 1.000000000000000000, 0.8660254037844387076, 1.000000000000000000, 0.8660254037844387076, 1.000000000000000000, 0.8660254037844387076, 1.000000000000000000, 0.8660254037844387076, 1.000000000000000000, 0.8660254037844387076, 1.000000000000000000, 0.8660254037844387076, 1.000000000000000000, 0.8660254037844387076, 1.000000000000000000, 0.8660254037844387076, 1.000000000000000000, 0.8660254037844387076, 1.000000000000000000, 0.8660254037844387076, 1.000000000000000000, 0.8660254037844387076, 1.000000000000000000, 0.8660254037844387076, 1.000000000000000000, 0.8660254037844387076, 1.000000000000000000, 0.8660254037844387076, 1.000000000000000000, 0.8660254037844387076, 1.000000000000000000, 0.8660254037844387076, 1.000000000000000000, 0.8660254037844387076, 1.000000000000000000, 0.8660254037844387076, 1.000000000000000000, 0.8660254037844387076, 1.000000000000000000, 0.8660254037844387076, 1.000000000000000000, 0.8660254037844387076, 1.000000000000000000, 0.8660254037844387076, 1.000000000000000000, 0.8660254037844387076, 1.000000000000000000, 0.8660254037844387076, 1.000000000000000000, 0.8660254037844387076, 1.000000000000000000, 0.8660254037844387076, 1.000000000000000000, 0.8660254037844387076, 1.000000000000000000, 0.8660254037844387076, 1.000000000000000000, 0.8660254037844387076, 1.000000000000000000, 0.8660254037844387076, 1.000000000000000000, 0.8660254037844387076, 1.000000000000000000, 0.8660254037844387076, 1.000000000000000000, 0.8660254037844387076, 1.000000000000000000, 0.8660254037844387076, 1.000000000000000000, 0.8660254037844387076, 1.000000000000000000, 0.8660254037844387076, 1.000000000000000000, 0.8660254037844387076, 1.000000000000000000, 0.8660254037844387076, 1.000000000000000000, 0.8660254037844387076, 1.000000000000000000, 0.8660254037844387076, 1.000000000000000000, 0.8660254037844387076, 1.000000000000000000, 0.8660254037844387076, 1.000000000000000000, 0.8660254037844387076, 1.000000000000000000, 0.8660254037844387076, 1.000000000000000000, 0.8660254037844387076, 1.000000000000000000, 0.8660254037844387076, 1.000000000000000000, 0.8660254037844387076, 1.000000000000000000, 0.8660254037844387076, 1.000000000000000000, 0.8660254037844387076, 1.000000000000000000, 0.8660254037844387076, 1.000000000000000000, 0.8660254037844387076, 1.000000000000000000, 0.8660254037844387076, 1.000000000000000000, 0.8660254037844387076, 1.000000000000000000, 0.8660254037844387076, 1.000000000000000000, 0.8660254037844387076, 1.000000000000000000, 0.8660254037844387076, 1.000000000000000000, 0.8660254037844387076, 1.000000000000000000, 0.8660254037844387076, 1.000000000000000000, 0.8660254037844387076, 1.000000000000000000, 0.8660254037844387076, 1.000000000000000000, 0.8660254037844387076, 1.000000000000000000, 0.8660254037844387076, 1.000000000000000000, 0.8660254037844387076, 1.000000000000000000, 0.8660254037844387076, 1.000000000000000000, 0.8660254037844387076, 1.000000000000000000, 0.8660254037844387076, 1.000000000000000000, 0.8660254037844387076, 1.000000000000000000, 0.8660254037844387076, 1.000000000000000000, 0.8660254037844387076, 1.000000000000000000, 0.8660254037844387076, 1.000000000000000000, 0.8660254037844387076, 1.000000000000000000, 0.8660254037844387076, 1.000000000000000000, 0.8660254037844387076, 1.000000000000000000, 0.8660254037844387076, 1.000000000000000000, 0.8660254037844387076, 1.000000000000000000, 0.8660254037844387076, 1.000000000000000000, 0.8660254037844387076, 1.000000000000000000, 0.8660254037844387076, 1.000000000000000000, 0.8660254037844387076, 1.000000000000000000, 0.8660254037844387076, 1.000000000000000000, 0.8660254037844387076, 1.000000000000000000, 0.8660254037844387076, 1.000000000000000000, 0.8660254037844387076, 1.000000000000000000, 0.8660254037844387076, 1.000000000000000000, 0.8660254037844387076, 1.000000000000000000, 0.8660254037844387076, 1.000000000000000000, 0.8660254037844387076, 1.000000000000000000, 0.8660254037844387076, 1.000000000000000000, 0.8660254037844387076, 1.000000000000000000, 0.8660254037844387076, 1.000000000000000000, 0.8660254037844387076, 1.000000000000000000, 0.8660254037844387076, 1.000000000000000000, 0.8660254037844387076, 1.000000000000000000, 0.8660254037844387076, 1.000000000000000000, 0.8660254037844387076, 1.000000000000000000, 0.8660254037844387076, 1.000000000000000000, 0.8660254037844387076, 1.000000000000000000, 0.8660254037844387076, 1.000000000000000000, 0.8660254037844387076, 1.000000000000000000, 0.8660254037844387076, 1.000000000000000000, 0.8660254037844387076, 1.000000000000000000, 0.8660254037844387076, 1.000000000000000000, 0.8660254037844387076, 1.000000000000000000, 0.8660254037844387076, 1.000000000000000000, 0.8660254037844387076, 1.000000000000000000, 0.8660254037844387076, 1.000000000000000000, 0.8660254037844387076, 1.000000000000000000, 0.8660254037844387076, 1.000000000000000000, 0.8660254037844387076, 1.000000000000000000, 0.8660254037844387076, 1.000000000000000000, 0.8660254037844387076, 1.000000000000000000, 0.8660254037844387076, 1.000000000000000000, 0.8660254037844387076, 1.000000000000000000, 0.8660254037844387076, 1.000000000000000000, 0.8660254037844387076, 1.000000000000000000, 0.8660254037844387076, 1.000000000000000000, 0.8660254037844387076, 1.000000000000000000, 0.8660254037844387076, 1.000000000000000000, 0.8660254037844387076, 1.000000000000000000, 0.8660254037844387076, 1.000000000000000000, 0.8660254037844387076, 1.000000000000000000, 0.8660254037844387076, 1.000000000000000000, 0.8660254037844387076, 1.000000000000000000, 0.8660254037844387076, 1.000000000000000000, 0.8660254037844387076, 1.000000000000000000, 0.8660254037844387076, 1.000000000000000000, 0.8660254037844387076, 1.000000000000000000, 0.8660254037844387076, 1.000000000000000000, 0.8660254037844387076, 1.000000000000000000, 0.8660254037844387076, 1.000000000000000000, 0.8660254037844387076, 1.000000000000000000, 0.8660254037844387076, 1.000000000000000000, 0.8660254037844387076, 1.000000000000000000, 0.8660254037844387076, 1.000000000000000000, 0.8660254037844387076, 1.000000000000000000, 0.8660254037844387076, 1.000000000000000000, 0.8660254037844387076, 1.000000000000000000, 0.8660254037844387076, 1.000000000000000000, 0.8660254037844387076, 1.000000000000000000, 0.8660254037844387076, 1.000000000000000000, 0.8660254037844387076, 1.000000000000000000, 0.8660254037844387076, 1.000000000000000000, 0.8660254037844387076, 1.000000000000000000, 0.8660254037844387076, 1.000000000000000000, 0.8660254037844387076, 1.000000000000000000, 0.8660254037844387076, 1.000000000000000000, 0.8660254037844387076, 1.000000000000000000, 0.8660254037844387076, 1.000000000000000000, 0.8660254037844387076, 1.000000000000000000, 0.8660254037844387076, 1.000000000000000000, 0.8660254037844387076, 1.000000000000000000, 0.8660254037844387076, 1.000000000000000000, 0.8660254037844387076, 1.000000000000000000, 0.8660254037844387076, 1.000000000000000000, 0.8660254037844387076, 1.000000000000000000, 0.8660254037844387076, 1.000000000000000000, 0.8660254037844387076, 1.000000000000000000, 0.8660254037844387076, 1.000000000000000000, 0.8660254037844387076, 1.000000000000000000, 0.8660254037844387076, 1.000000000000000000, 0.8660254037844387076, 1.000000000000000000, 0.8660254037844387076, 1.000000000000000000, 0.8660254037844387076, 1.000000000000000000, 0.8660254037844387076, 1.000000000000000000, 0.8660254037844387076, 1.000000000000000000, 0.8660254037844387076, 1.000000000000000000, 0.8660254037844387076, 1.000000000000000000, 0.8660254037844387076, 1.000000000000000000, 0.8660254037844387076, 1.000000000000000000, 0.8660254037844387076, 1.000000000000000000, 0.8660254037844387076, 1.000000000000000000, 0.8660254037844387076, 1.000000000000000000, 0.8660254037844387076, 1.000000000000000000, 0.8660254037844387076, 1.000000000000000000, 0.8660254037844387076, 1.000000000000000000, 0.8660254037844387076, 1.000000000000000000, 0.8660254037844387076, 1.000000000000000000, 0.8660254037844387076, 1.000000000000000000, 0.8660254037844387076, 1.000000000000000000, 0.8660254037844387076, 1.000000000000000000, 0.8660254037844387076, 1.000000000000000000, 0.8660254037844387076, 1.000000000000000000, 0.8660254037844387076, 1.000000000000000000, 0.8660254037844387076, 1.000000000000000000, 0.8660254037844387076, 1.000000000000000000, 0.8660254037844387076, 1.000000000000000000, 0.8660254037844387076, 1.000000000000000000, 0.8660254037844387076, 1.000000000000000000, 0.8660254037844387076, 1.000000000000000000, 0.8660254037844387076, 1.000000000000000000, 0.8660254037844387076, 1.000000000000000000, 0.8660254037844387076, 1.000000000000000000, 0.8660254037844387076, 1.000000000000000000, 0.8660254037844387076, 1.000000000000000000, 0.8660254037844387076, 1.000000000000000000, 0.8660254037844387076, 1.000000000000000000, 0.8660254037844387076, 1.000000000000000000, 0.8660254037844387076, 1.000000000000000000, 0.8660254037844387076, 1.000000000000000000, 0.8660254037844387076, 1.000000000000000000, 0.8660254037844387076, 1.000000000000000000, 0.8660254037844387076, 1.000000000000000000, 0.8660254037844387076, 1.000000000000000000, 0.8660254037844387076, 1.000000000000000000, 0.8660254037844387076, 1.000000000000000000, 0.8660254037844387076, 1.000000000000000000, 0.8660254037844387076, 1.000000000000000000, 0.8660254037844387076, 1.000000000000000000, 0.8660254037844387076, 1.000000000000000000, 0.8660254037844387076, 1.000000000000000000, 0.8660254037844387076, 1.000000000000000000, 0.8660254037844387076, 1.000000000000000000, 0.8660254037844387076, 1.000000000000000000, 0.8660254037844387076, 1.000000000000000000, 0.8660254037844387076, 1.000000000000000000, 0.8660254037844387076, 1.000000000000000000, 0.8660254037844387076, 1.000000000000000000, 0.8660254037844387076, 1.000000000000000000, 0.8660254037844387076, 1.000000000000000000, 0.8660254037844387076, 1.000000000000000000, 0.8660254037844387076, 1.000000000000000000, 0.8660254037844387076, 1.000000000000000000, 0.8660254037844387076, 1.000000000000000000, 0.8660254037844387076, 1.000000000000000000, 0.8660254037844387076, 1.000000000000000000, 0.8660254037844387076, 1.000000000000000000, 0.8660254037844387076, 1.000000000000000000, 0.8660254037844387076, 1.000000000000000000, 0.8660254037844387076, 1.000000000000000000, 0.8660254037844387076, 1.000000000000000000, 0.8660254037844387076, 1.000000000000000000, 0.8660254037844387076, 1.000000000000000000, 0.8660254037844387076, 1.000000000000000000, 0.8660254037844387076, 1.000000000000000000, 0.8660254037844387076, 1.000000000000000000, 0.8660254037844387076, 1.000000000000000000, 0.8660254037844387076, 1.000000000000000000, 0.8660254037844387076, 1.000000000000000000, 0.8660254037844387076, 1.000000000000000000, 0.8660254037844387076, 1.000000000000000000, 0.8660254037844387076, 1.000000000000000000, 0.8660254037844387076, 1.000000000000000000, 0.8660254037844387076, 1.000000000000000000, 0.8660254037844387076, 1.000000000000000000, 0.8660254037844387076, 1.000000000000000000, 0.8660254037844387076, 1.000000000000000000, 0.8660254037844387076, 1.000000000000000000, 0.8660254037844387076, 1.000000000000000000, 0.8660254037844387076, 1.000000000000000000, 0.8660254037844387076, 1.000000000000000000, 0.8660254037844387076, 1.000000000000000000, 0.8660254037844387076, 1.000000000000000000, 0.8660254037844387076, 1.000000000000000000, 0.8660254037844387076, 1.000000000000000000, 0.8660254037844387076, 1.000000000000000000, 0.8660254037844387076, 1.000000000000000000, 0.8660254037844387076, 1.000000000000000000, 0.8660254037844387076, 1.000000000000000000, 0.8660254037844387076, 1.000000000000000000, 0.8660254037844387076, 1.000000000000000000, 0.8660254037844387076, 1.000000000000000000, 0.8660254037844387076, 1.000000000000000000, 0.8660254037844387076, 1.000000000000000000, 0.8660254037844387076, 1.000000000000000000, 0.8660254037844387076, 1.000000000000000000, 0.8660254037844387076, 1.000000000000000000, 0.8660254037844387076, 1.000000000000000000, 0.8660254037844387076, 1.000000000000000000, 0.8660254037844387076, 1.000000000000000000, 0.8660254037844387076, 1.000000000000000000, 0.8660254037844387076, 1.000000000000000000, 0.8660254037844387076, 1.000000000000000000, 0.8660254037844387076, 1.000000000000000000, 0.8660254037844387076, 1.000000000000000000, 0.8660254037844387076, 1.000000000000000000, 0.8660254037844387076, 1.000000000000000000, 0.8660254037844387076, 1.000000000000000000, 0.8660254037844387076, 1.000000000000000000, 0.8660254037844387076, 1.000000000000000000, 0.8660254037844387076, 1.000000000000000000, 0.8660254037844387076, 1.000000000000000000, 0.8660254037844387076, 1.000000000000000000, 0.8660254037844387076, 1.000000000000000000, 0.8660254037844387076, 1.000000000000000000, 0.8660254037844387076, 1.000000000000000000, 0.8660254037844387076, 1.000000000000000000, 0.8660254037844387076, 1.000000000000000000, 0.8660254037844387076, 1.000000000000000000, 0.8660254037844387076, 1.000000000000000000, 0.8660254037844387076, 1.000000000000000000, 0.8660254037844387076, 1.000000000000000000, 0.8660254037844387076, 1.000000000000000000, 0.8660254037844387076, 1.000000000000000000, 0.8660254037844387076, 1.000000000000000000, 0.8660254037844387076, 1.000000000000000000, 0.8660254037844387076, 1.000000000000000000, 0.8660254037844387076, 1.000000000000000000, 0.8660254037844387076, 1.000000000000000000, 0.8660254037844387076, 1.000000000000000000, 0.8660254037844387076, 1.000000000000000000, 0.8660254037844387076, 1.000000000000000000, 0.8660254037844387076, 1.000000000000000000, 0.8660254037844387076, 1.000000000000000000, 0.8660254037844387076, 1.000000000000000000, 0.8660254037844387076, 1.000000000000000000, 0.8660254037844387076, 1.000000000000000000, 0.8660254037844387076, 1.000000000000000000, 0.8660254037844387076, 1.000000000000000000, 0.8660254037844387076, 1.000000000000000000, 0.8660254037844387076, 1.000000000000000000, 0.8660254037844387076, 1.000000000000000000, 0.8660254037844387076, 1.000000000000000000, 0.8660254037844387076, 1.000000000000000000, 0.8660254037844387076, 1.000000000000000000, 0.8660254037844387076, 1.000000000000000000, 0.8660254037844387076, 1.000000000000000000, 0.8660254037844387076, 1.000000000000000000, 0.8660254037844387076, 1.000000000000000000, 0.8660254037844387076, 1.000000000000000000, 0.8660254037844387076, 1.000000000000000000, 0.8660254037844387076, 1.000000000000000000, 0.8660254037844387076, 1.000000000000000000, 0.8660254037844387076, 1.000000000000000000, 0.8660254037844387076, 1.000000000000000000, 0.8660254037844387076, 1.000000000000000000, 0.8660254037844387076, 1.000000000000000000, 0.8660254037844387076, 1.000000000000000000, 0.8660254037844387076, 1.000000000000000000, 0.8660254037844387076, 1.000000000000000000, 0.8660254037844387076, 1.000000000000000000, 0.8660254037844387076, 1.000000000000000000, 0.8660254037844387076, 1.000000000000000000, 0.8660254037844387076, 1.000000000000000000, 0.8660254037844387076, 1.000000000000000000, 0.8660254037844387076, 1.000000000000000000, 0.8660254037844387076, 1.000000000000000000, 0.8660254037844387076, 1.000000000000000000, 0.8660254037844387076, 1.000000000000000000, 0.8660254037844387076, 1.000000000000000000) ) ) 
 REPRESENTATION_ITEM ( '' )  SURFACE ( )  );
#22645=ORIENTED_EDGE ( 'NONE', *, *, #15617, .F. ) ;
#22646=CARTESIAN_POINT ( 'NONE',  ( 10.00000000000000000, 5.773502691896255534, -18.37499999999997513 ) ) ;
#22647=CARTESIAN_POINT ( 'NONE',  ( -4.999999999999996447, 8.660254037844387298, -154.5000000000000000 ) ) ;
#22651=CARTESIAN_POINT ( 'NONE',  ( -10.81189881249999729, 1.324075727343319199E-15, -125.2812500020483668 ) ) ;
#22652=ORIENTED_EDGE ( 'NONE', *, *, #28347, .T. ) ;
#22653=CARTESIAN_POINT ( 'NONE',  ( 9.999999999999998224, 0.000000000000000000, -21.49999999999996447 ) ) ;
#22655=CARTESIAN_POINT ( 'NONE',  ( -5.405949406249996869, 9.363379034771805109, -56.53125000204836681 ) ) ;
#22657=CARTESIAN_POINT ( 'NONE',  ( 5.405949406249992428, -9.363379034771808662, -102.0937500020483810 ) ) ;
#22658=ORIENTED_EDGE ( 'NONE', *, *, #33578, .F. ) ;
#22659=VERTEX_POINT ( 'NONE', #28423 ) ;
#22660=DIRECTION ( 'NONE',  ( 1.000000000000000000, 0.000000000000000000, 0.000000000000000000 ) ) ;
#22661=CARTESIAN_POINT ( 'NONE',  ( -5.000000000000003553, -8.660254037844383745, -116.4999999999999858 ) ) ;
#22664=CARTESIAN_POINT ( 'NONE',  ( 9.999999999999998224, 0.000000000000000000, -50.37500000409675494 ) ) ;
#22665=EDGE_CURVE ( 'NONE', #42101, #39394, #13767, .T. ) ;
#22666=CARTESIAN_POINT ( 'NONE',  ( 10.81189881249999551, -6.242252689847874514, -128.9687500020483810 ) ) ;
#22667=VECTOR ( 'NONE', #33520, 1000.000000000000000 ) ;
#22669=CARTESIAN_POINT ( 'NONE',  ( 9.999999999999998224, 0.000000000000000000, -138.8750000040968189 ) ) ;
#22671=CARTESIAN_POINT ( 'NONE',  ( -5.000000000000003553, -8.660254037844383745, -191.8750000040967905 ) ) ;
#22673=CARTESIAN_POINT ( 'NONE',  ( 7.644554776091147741E-16, 12.48450537969573659, -184.1562500020484094 ) ) ;
#22674=EDGE_CURVE ( 'NONE', #14006, #36710, #9639, .T. ) ;
#22675=CARTESIAN_POINT ( 'NONE',  ( -5.000000000000003553, -8.660254037844383745, -47.49999999999998579 ) ) ;
#22678=CARTESIAN_POINT ( 'NONE',  ( 10.81189881249999729, 0.000000000000000000, -71.84375000204836681 ) ) ;
#22679=VECTOR ( 'NONE', #13261, 1000.000000000000000 ) ;
#22680=CARTESIAN_POINT ( 'NONE',  ( 5.405949406249999534, 9.363379034771803333, -50.59375000204835260 ) ) ;
#22683=CARTESIAN_POINT ( 'NONE',  ( -10.81189881249999729, 6.242252689847871849, -23.40625000204837747 ) ) ;
#22687=CARTESIAN_POINT ( 'NONE',  ( 4.999999999999992006, -8.660254037844389075, -110.2499999999999858 ) ) ;
#22691=CARTESIAN_POINT ( 'NONE',  ( 5.405949406249992428, -9.363379034771808662, -115.7812500020483952 ) ) ;
#22695=CARTESIAN_POINT ( 'NONE',  ( -9.999999999999998224, 1.224646799147353059E-15, -102.1250000040967905 ) ) ;
#22697=ORIENTED_EDGE ( 'NONE', *, *, #1146, .F. ) ;
#22698=CARTESIAN_POINT ( 'NONE',  ( 7.070501591499377789E-16, 11.54700538379251284, -42.12499999999997868 ) ) ;
#22699=CARTESIAN_POINT ( 'NONE',  ( -9.999999999999998224, 1.224646799147353059E-15, -21.12500000409675494 ) ) ;
#22700=CARTESIAN_POINT ( 'NONE',  ( -5.405949406249996869, 9.363379034771805109, -47.53125000204838813 ) ) ;
#22701=CARTESIAN_POINT ( 'NONE',  ( 9.999999999999998224, 0.000000000000000000, -24.87500000409675849 ) ) ;
#22705=CARTESIAN_POINT ( 'NONE',  ( -5.405949406249996869, 9.363379034771805109, -139.0312500020484094 ) ) ;
#22706=CARTESIAN_POINT ( 'NONE',  ( -2.293366432827344421E-15, -12.48450537969573659, -147.4062500020483810 ) ) ;
#22707=EDGE_CURVE ( 'NONE', #12159, #2188, #40496, .T. ) ;
#22710=ORIENTED_EDGE ( 'NONE', *, *, #24156, .T. ) ;
#22711=AXIS2_PLACEMENT_3D ( 'NONE', #39149, #25364, #28604 ) ;
#22712=ORIENTED_EDGE ( 'NONE', *, *, #27036, .F. ) ;
#22713=ORIENTED_EDGE ( 'NONE', *, *, #27856, .F. ) ;
#22714=DIRECTION ( 'NONE',  ( -0.000000000000000000, -0.000000000000000000, 1.000000000000000000 ) ) ;
#22715=CARTESIAN_POINT ( 'NONE',  ( 5.405949406249999534, 9.363379034771803333, -170.5937500020484094 ) ) ;
#22717=CARTESIAN_POINT ( 'NONE',  ( -2.293366432827344421E-15, -12.48450537969573659, -21.21875000204837036 ) ) ;
#22719=CARTESIAN_POINT ( 'NONE',  ( 7.644554776091147741E-16, 12.48450537969573659, -161.4687500020484094 ) ) ;
#22720=CARTESIAN_POINT ( 'NONE',  ( 5.405949406249992428, -9.363379034771808662, -142.5937500020483810 ) ) ;
#22724=CARTESIAN_POINT ( 'NONE',  ( 5.405949406249992428, -9.363379034771808662, -21.09375000204835615 ) ) ;
#22727=CARTESIAN_POINT ( 'NONE',  ( 0.000000000000000000, 0.000000000000000000, -200.0000000000000000 ) ) ;
#22729=CARTESIAN_POINT ( 'NONE',  ( -9.999999999999998224, 1.224646799147353059E-15, -168.1250000040967905 ) ) ;
#22730=CARTESIAN_POINT ( 'NONE',  ( -2.293366432827344421E-15, -12.48450537969573659, -76.71875000204838102 ) ) ;
#22731=CARTESIAN_POINT ( 'NONE',  ( 10.81189881249999551, -6.242252689847874514, -54.15625000204837391 ) ) ;
#22733=CARTESIAN_POINT ( 'NONE',  ( 9.999999999999998224, 0.000000000000000000, -15.87500000409675138 ) ) ;
#22735=CARTESIAN_POINT ( 'NONE',  ( 7.070501591499377789E-16, 11.54700538379251284, -141.1250000000000000 ) ) ;
#22736=CARTESIAN_POINT ( 'NONE',  ( 10.81189881249999729, 6.242252689847867408, -140.9062500020484094 ) ) ;
#22737=CARTESIAN_POINT ( 'NONE',  ( -5.000000000000003553, -8.660254037844383745, -151.0000000000000000 ) ) ;
#22738=CARTESIAN_POINT ( 'NONE',  ( -4.999999999999996447, 8.660254037844387298, -117.3750000040967905 ) ) ;
#22740=ORIENTED_EDGE ( 'NONE', *, *, #7944, .F. ) ;
#22744=CARTESIAN_POINT ( 'NONE',  ( -5.405949406250003975, -9.363379034771801557, -176.0312500020483810 ) ) ;
#22745=CARTESIAN_POINT ( 'NONE',  ( 9.999999999999996447, -5.773502691896262640, -53.50000000409677625 ) ) ;
#22748=( BOUNDED_CURVE ( )  B_SPLINE_CURVE ( 2, ( #37268, #15017, #41349, #18265, #38130, #34696, #7930 ),
 .UNSPECIFIED., .F., .F. ) 
 B_SPLINE_CURVE_WITH_KNOTS ( ( 3, 2, 2, 3 ),
 ( 0.08582089552238814090, 0.08706467661691551230, 0.08830845771144288370, 0.08955223880597024122 ),
 .UNSPECIFIED. ) 
 CURVE ( )  GEOMETRIC_REPRESENTATION_ITEM ( )  RATIONAL_B_SPLINE_CURVE ( ( 0.9999999999999910072, 0.8660254037844477004, 1.000000000000000000, 0.8660254037844387076, 1.000000000000000000, 0.8660254037844282715, 1.000000000000010436 ) ) 
 REPRESENTATION_ITEM ( '' )  );
#22749=CARTESIAN_POINT ( 'NONE',  ( 10.00000000000154010, -5.773502691895370020, -63.62499999999992895 ) ) ;
#22750=CARTESIAN_POINT ( 'NONE',  ( 10.81189881249999729, 0.000000000000000000, -157.5312500020484094 ) ) ;
#22751=CARTESIAN_POINT ( 'NONE',  ( 7.644554776091147741E-16, 12.48450537969573659, -140.4687500020483810 ) ) ;
#22752=CARTESIAN_POINT ( 'NONE',  ( -4.999999999999996447, 8.660254037844387298, -100.4999999999999858 ) ) ;
#22753=FACE_OUTER_BOUND ( 'NONE', #21540, .T. ) ;
#22754=EDGE_CURVE ( 'NONE', #15095, #16464, #25657, .T. ) ;
#22757=CARTESIAN_POINT ( 'NONE',  ( 9.999999999999998224, 0.000000000000000000, -114.8750000040967905 ) ) ;
#22758=CARTESIAN_POINT ( 'NONE',  ( 10.81189881249999729, 0.000000000000000000, -70.53125000204838102 ) ) ;
#22759=VERTEX_POINT ( 'NONE', #2718 ) ;
#22761=CARTESIAN_POINT ( 'NONE',  ( -5.405949406250003975, -9.363379034771801557, -118.8437500020483810 ) ) ;
#22762=ORIENTED_EDGE ( 'NONE', *, *, #28566, .F. ) ;
#22764=CARTESIAN_POINT ( 'NONE',  ( 5.405949406249992428, -9.363379034771808662, -27.09375000204835970 ) ) ;
#22765=CARTESIAN_POINT ( 'NONE',  ( -10.81189881249999907, -6.242252689847864744, -193.9687500020484094 ) ) ;
#22766=CARTESIAN_POINT ( 'NONE',  ( -10.81189881249999729, 6.242252689847871849, -59.21875000204837391 ) ) ;
#22767=CARTESIAN_POINT ( 'NONE',  ( -9.999999999999998224, 1.224646799147353059E-15, -127.2499999999999716 ) ) ;
#22769=EDGE_CURVE ( 'NONE', #22182, #27209, #16544, .T. ) ;
#22770=CARTESIAN_POINT ( 'NONE',  ( -5.405949406250003975, -9.363379034771801557, -190.8437500020484094 ) ) ;
#22771=CARTESIAN_POINT ( 'NONE',  ( 10.81189881249999551, -6.242252689847874514, -166.4687500020484094 ) ) ;
#22775=CARTESIAN_POINT ( 'NONE',  ( -4.999999999999996447, 8.660254037844387298, -193.8750000040967905 ) ) ;
#22777=CARTESIAN_POINT ( 'NONE',  ( 10.81189881249999907, 6.242252689847868297, -100.2187500020483810 ) ) ;
#22778=CARTESIAN_POINT ( 'NONE',  ( -4.999999999999996447, 8.660254037844387298, -108.3750000040967763 ) ) ;
#22779=CARTESIAN_POINT ( 'NONE',  ( -10.81189881249999729, 6.242252689847871849, -71.40625000204838102 ) ) ;
#22780=LINE ( 'NONE', #32709, #16416 ) ;
#22782=CARTESIAN_POINT ( 'NONE',  ( -5.405949406250003975, -9.363379034771801557, -82.84375000204836681 ) ) ;
#22783=ADVANCED_FACE ( 'NONE', ( #35320 ), #5749, .T. ) ;
#22785=CARTESIAN_POINT ( 'NONE',  ( -10.00000000000000000, -5.773502691896251982, -135.0000000040967905 ) ) ;
#22787=EDGE_LOOP ( 'NONE', ( #25745, #6150, #33967, #5230 ) ) ;
#22790=CARTESIAN_POINT ( 'NONE',  ( 5.405949406249992428, -9.363379034771808662, -198.2812500020484094 ) ) ;
#22791=CARTESIAN_POINT ( 'NONE',  ( 9.999999999999998224, 0.000000000000000000, -200.0000000000000000 ) ) ;
#22793=ORIENTED_EDGE ( 'NONE', *, *, #36252, .T. ) ;
#22794=CARTESIAN_POINT ( 'NONE',  ( 9.999999999999996447, -5.773502691896262640, -57.62499999999998579 ) ) ;
#22796=CARTESIAN_POINT ( 'NONE',  ( -2.121150477449813534E-15, -11.54700538379251284, -70.25000000409679046 ) ) ;
#22800=CARTESIAN_POINT ( 'NONE',  ( -10.81189881249999729, 1.324075727343319199E-15, -71.28125000204838102 ) ) ;
#22803=CARTESIAN_POINT ( 'NONE',  ( 9.999999999999998224, 0.000000000000000000, -200.0000000000000000 ) ) ;
#22804=CARTESIAN_POINT ( 'NONE',  ( 10.81189881249999907, 6.242252689847868297, -185.9062500020484094 ) ) ;
#22805=VECTOR ( 'NONE', #36658, 1000.000000000000000 ) ;
#22807=CARTESIAN_POINT ( 'NONE',  ( 5.000000000000000000, 8.660254037844385522, -79.74999999999998579 ) ) ;
#22808=FACE_OUTER_BOUND ( 'NONE', #1271, .T. ) ;
#22809=VECTOR ( 'NONE', #13906, 1000.000000000000000 ) ;
#22810=CARTESIAN_POINT ( 'NONE',  ( -10.00000000000000000, -0.8677423694974171209, 0.000000000000000000 ) ) ;
#22811=CARTESIAN_POINT ( 'NONE',  ( -1.040834085586084257E-14, -20.00000000000000355, 22.49999999999999289 ) ) ;
#22813=CARTESIAN_POINT ( 'NONE',  ( -9.999999999999998224, 5.773502691896259087, -166.3749999999999716 ) ) ;
#22814=CYLINDRICAL_SURFACE ( 'NONE', #40633, 9.999999999999998224 ) ;
#22815=EDGE_CURVE ( 'NONE', #42101, #12898, #39377, .T. ) ;
#22816=CARTESIAN_POINT ( 'NONE',  ( -5.405949406249996869, 9.363379034771805109, -97.03125000204839523 ) ) ;
#22818=CARTESIAN_POINT ( 'NONE',  ( 9.999999999999998224, 0.000000000000000000, -24.87500000409675849 ) ) ;
#22820=ORIENTED_EDGE ( 'NONE', *, *, #23564, .F. ) ;
#22821=VERTEX_POINT ( 'NONE', #9185 ) ;
#22822=CARTESIAN_POINT ( 'NONE',  ( -10.81189881249999729, 6.242252689847871849, -38.21875000204836681 ) ) ;
#22823=CARTESIAN_POINT ( 'NONE',  ( 7.644554776091147741E-16, 12.48450537969573659, -20.65625000204838102 ) ) ;
#22825=CARTESIAN_POINT ( 'NONE',  ( -5.405949406249996869, 9.363379034771805109, -75.84375000204838102 ) ) ;
#22826=DIRECTION ( 'NONE',  ( -0.000000000000000000, -0.000000000000000000, 1.000000000000000000 ) ) ;
#22827=CARTESIAN_POINT ( 'NONE',  ( -5.405949406250003975, -9.363379034771801557, -196.8437500020484094 ) ) ;
#22828=EDGE_CURVE ( 'NONE', #24456, #14015, #42188, .T. ) ;
#22832=CARTESIAN_POINT ( 'NONE',  ( -5.000000000000003553, -8.660254037844383745, 0.1249999959032355168 ) ) ;
#22835=CARTESIAN_POINT ( 'NONE',  ( -10.81189881249999907, -6.242252689847864744, -118.9687500020483810 ) ) ;
#22836=CARTESIAN_POINT ( 'NONE',  ( 10.81189881249999907, 6.242252689847868297, -100.4062500020483952 ) ) ;
#22837=CARTESIAN_POINT ( 'NONE',  ( 10.81189881249999729, 0.000000000000000000, -109.3437500020483810 ) ) ;
#22840=CARTESIAN_POINT ( 'NONE',  ( -2.121150477449813534E-15, -11.54700538379251284, -170.7500000040967620 ) ) ;
#22841=DIRECTION ( 'NONE',  ( 1.000000000000000000, 0.000000000000000000, 0.000000000000000000 ) ) ;
#22845=CARTESIAN_POINT ( 'NONE',  ( -9.999999999999998224, 1.224646799147353059E-15, -197.7500000000000000 ) ) ;
#22849=CARTESIAN_POINT ( 'NONE',  ( 9.999999999999996447, -5.773502691896262640, -80.12500000000000000 ) ) ;
#22851=CARTESIAN_POINT ( 'NONE',  ( 9.999999999999998224, 0.000000000000000000, -96.87500000409677625 ) ) ;
#22854=CARTESIAN_POINT ( 'NONE',  ( -5.405949406249996869, 9.363379034771805109, -95.53125000204838102 ) ) ;
#22855=ORIENTED_EDGE ( 'NONE', *, *, #34657, .T. ) ;
#22857=FACE_OUTER_BOUND ( 'NONE', #2807, .T. ) ;
#22859=ORIENTED_EDGE ( 'NONE', *, *, #8003, .T. ) ;
#22860=CARTESIAN_POINT ( 'NONE',  ( -5.000000000000003553, -8.660254037844383745, -6.999999999999978684 ) ) ;
#22861=CARTESIAN_POINT ( 'NONE',  ( -2.121150477449813534E-15, -11.54700538379251284, -146.3750000000000000 ) ) ;
#22865=CARTESIAN_POINT ( 'NONE',  ( 10.00000000000000000, 5.773502691896255534, -196.8750000000000284 ) ) ;
#22866=CARTESIAN_POINT ( 'NONE',  ( 10.81189881249999551, -6.242252689847874514, -117.1562500020483810 ) ) ;
#22867=ORIENTED_EDGE ( 'NONE', *, *, #30548, .T. ) ;
#22870=( BOUNDED_CURVE ( )  B_SPLINE_CURVE ( 2, ( #36230, #33221, #10737, #6664, #39669, #10316, #13331 ),
 .UNSPECIFIED., .F., .F. ) 
 B_SPLINE_CURVE_WITH_KNOTS ( ( 3, 2, 2, 3 ),
 ( 0.8320895522388060961, 0.8333333333333334814, 0.8345771144278608666, 0.8358208955223882519 ),
 .UNSPECIFIED. ) 
 CURVE ( )  GEOMETRIC_REPRESENTATION_ITEM ( )  RATIONAL_B_SPLINE_CURVE ( ( 0.9999999999999880096, 0.8660254037844506980, 1.000000000000000000, 0.8660254037844387076, 1.000000000000000000, 0.8660254037844148378, 1.000000000000023981 ) ) 
 REPRESENTATION_ITEM ( '' )  );
#22871=CARTESIAN_POINT ( 'NONE',  ( -5.405949406249996869, 9.363379034771805109, -52.03125000204835970 ) ) ;
#22874=EDGE_CURVE ( 'NONE', #40403, #30149, #28693, .T. ) ;
#22875=CARTESIAN_POINT ( 'NONE',  ( 10.81189881249999729, 0.000000000000000000, -104.8437500020483810 ) ) ;
#22876=CARTESIAN_POINT ( 'NONE',  ( -10.81189881249999729, 1.324075727343319199E-15, -122.2812500020483952 ) ) ;
#22877=EDGE_LOOP ( 'NONE', ( #37356, #13965, #23433, #27753 ) ) ;
#22878=CARTESIAN_POINT ( 'NONE',  ( 4.999999999999992006, -8.660254037844389075, -132.7499999999999716 ) ) ;
#22880=( BOUNDED_CURVE ( )  B_SPLINE_CURVE ( 2, ( #26142, #22478, #19232, #42102, #5664, #12323, #2223 ),
 .UNSPECIFIED., .F., .F. ) 
 B_SPLINE_CURVE_WITH_KNOTS ( ( 3, 2, 2, 3 ),
 ( 0.1156716417910447492, 0.1169154228855721483, 0.1181592039800995753, 0.1194029850746269744 ),
 .UNSPECIFIED. ) 
 CURVE ( )  GEOMETRIC_REPRESENTATION_ITEM ( )  RATIONAL_B_SPLINE_CURVE ( ( 1.000000000000003109, 0.8660254037844358210, 1.000000000000000000, 0.8660254037844387076, 1.000000000000000000, 0.8660254037844267172, 1.000000000000011990 ) ) 
 REPRESENTATION_ITEM ( '' )  );
#22882=CARTESIAN_POINT ( 'NONE',  ( 7.644554776091147741E-16, 12.48450537969573659, 0.5312499979516547288 ) ) ;
#22883=CARTESIAN_POINT ( 'NONE',  ( 9.999999999999998224, 0.000000000000000000, -8.375000004096744277 ) ) ;
#22884=CARTESIAN_POINT ( 'NONE',  ( -10.81189881249999729, 6.242252689847871849, -132.7187500020483810 ) ) ;
#22886=CARTESIAN_POINT ( 'NONE',  ( -9.999999999999998224, 1.224646799147353059E-15, -158.7500000000000000 ) ) ;
#22888=CARTESIAN_POINT ( 'NONE',  ( -2.121150477449813534E-15, -11.54700538379251284, -197.7500000040967905 ) ) ;
#22891=AXIS2_PLACEMENT_3D ( 'NONE', #12175, #15409, #25366 ) ;
#22892=CARTESIAN_POINT ( 'NONE',  ( -10.81189881249999729, -6.242252689847864744, -185.1562500020484094 ) ) ;
#22893=( BOUNDED_CURVE ( )  B_SPLINE_CURVE ( 2, ( #6346, #9780, #19489, #3105, #22960, #36115, #22109 ),
 .UNSPECIFIED., .F., .F. ) 
 B_SPLINE_CURVE_WITH_KNOTS ( ( 3, 2, 2, 3 ),
 ( 0.2873134328358210032, 0.2885572139303483885, 0.2898009950248757183, 0.2910447761194031036 ),
 .UNSPECIFIED. ) 
 CURVE ( )  GEOMETRIC_REPRESENTATION_ITEM ( )  RATIONAL_B_SPLINE_CURVE ( ( 0.9999999999999880096, 0.8660254037844506980, 1.000000000000000000, 0.8660254037844387076, 1.000000000000000000, 0.8660254037844267172, 1.000000000000011990 ) ) 
 REPRESENTATION_ITEM ( '' )  );
#22897=CARTESIAN_POINT ( 'NONE',  ( -5.405949406250003975, -9.363379034771801557, -63.34375000204836681 ) ) ;
#22898=CARTESIAN_POINT ( 'NONE',  ( -5.405949406250003975, -9.363379034771801557, -51.34375000204835260 ) ) ;
#22901=CARTESIAN_POINT ( 'NONE',  ( -5.405949406249996869, 9.363379034771805109, -22.03125000204836326 ) ) ;
#22905=CARTESIAN_POINT ( 'NONE',  ( -2.121150477449813534E-15, -11.54700538379251284, -107.3749999999999716 ) ) ;
#22906=CARTESIAN_POINT ( 'NONE',  ( -9.999999999999998224, 1.224646799147353059E-15, -115.2499999999999858 ) ) ;
#22909=CARTESIAN_POINT ( 'NONE',  ( 10.81189881249999551, -6.242252689847874514, -115.6562500020483810 ) ) ;
#22910=ORIENTED_EDGE ( 'NONE', *, *, #17051, .F. ) ;
#22915=ORIENTED_EDGE ( 'NONE', *, *, #6671, .T. ) ;
#22916=CARTESIAN_POINT ( 'NONE',  ( -9.999999999999998224, 1.224646799147353059E-15, -44.74999999999998579 ) ) ;
#22918=CARTESIAN_POINT ( 'NONE',  ( 9.999999999999998224, 0.000000000000000000, -15.87500000409675138 ) ) ;
#22919=CARTESIAN_POINT ( 'NONE',  ( 7.644554776091147741E-16, 12.48450537969573659, -41.65625000204836681 ) ) ;
#22922=CARTESIAN_POINT ( 'NONE',  ( 9.999999999999998224, 0.000000000000000000, -200.0000000000000000 ) ) ;
#22923=CARTESIAN_POINT ( 'NONE',  ( -10.81189881249999729, 6.242252689847871849, -138.9062500020484094 ) ) ;
#22924=CARTESIAN_POINT ( 'NONE',  ( 5.405949406249992428, -9.363379034771808662, -153.2812500020484094 ) ) ;
#22927=VECTOR ( 'NONE', #40655, 1000.000000000000000 ) ;
#22928=EDGE_CURVE ( 'NONE', #36134, #6564, #29824, .T. ) ;
#22929=ORIENTED_EDGE ( 'NONE', *, *, #14598, .F. ) ;
#22930=ORIENTED_EDGE ( 'NONE', *, *, #13755, .T. ) ;
#22931=LINE ( 'NONE', #16842, #2881 ) ;
#22932=CARTESIAN_POINT ( 'NONE',  ( -10.81189881249999729, 1.324075727343319199E-15, -174.5937500020484094 ) ) ;
#22934=CARTESIAN_POINT ( 'NONE',  ( -10.81189881249999907, -6.242252689847864744, -24.46875000204836681 ) ) ;
#22935=CARTESIAN_POINT ( 'NONE',  ( 9.999999999999998224, 0.000000000000000000, -128.3750000040967905 ) ) ;
#22936=CARTESIAN_POINT ( 'NONE',  ( 5.405949406249999534, 9.363379034771803333, -154.0937500020483810 ) ) ;
#22937=CARTESIAN_POINT ( 'NONE',  ( -10.81189881249999729, 6.242252689847871849, -143.2187500020484094 ) ) ;
#22941=CARTESIAN_POINT ( 'NONE',  ( -5.405949406249996869, 9.363379034771805109, -21.84375000204835615 ) ) ;
#22944=CARTESIAN_POINT ( 'NONE',  ( 9.999999999999998224, 0.000000000000000000, -25.99999999999996803 ) ) ;
#22946=CARTESIAN_POINT ( 'NONE',  ( 9.999999999999998224, 0.000000000000000000, -86.37500000409677625 ) ) ;
#22947=CARTESIAN_POINT ( 'NONE',  ( -2.293366432827344421E-15, -12.48450537969573659, -69.21875000204839523 ) ) ;
#22948=CARTESIAN_POINT ( 'NONE',  ( 10.81189881249999551, -6.242252689847874514, -45.15625000204836681 ) ) ;
#22952=CARTESIAN_POINT ( 'NONE',  ( 5.000000000000000000, 8.660254037844385522, -135.2499999999999716 ) ) ;
#22953=CARTESIAN_POINT ( 'NONE',  ( -10.81189881249999729, -6.242252689847864744, -140.1562500020484094 ) ) ;
#22954=CARTESIAN_POINT ( 'NONE',  ( -9.999999999999998224, 1.224646799147353059E-15, -99.12500000409677625 ) ) ;
#22955=CARTESIAN_POINT ( 'NONE',  ( -2.121150477449813534E-15, -11.54700538379251284, -112.2500000040967763 ) ) ;
#22957=ORIENTED_EDGE ( 'NONE', *, *, #42564, .F. ) ;
#22960=CARTESIAN_POINT ( 'NONE',  ( 4.999999999999992006, -8.660254037844389075, -140.6250000040967905 ) ) ;
#22961=CARTESIAN_POINT ( 'NONE',  ( 10.81189881249999729, 0.000000000000000000, -174.0312500020484094 ) ) ;
#22962=CARTESIAN_POINT ( 'NONE',  ( -10.00000000000000000, -5.773502691896251982, -40.50000000409675494 ) ) ;
#22963=( BOUNDED_CURVE ( )  B_SPLINE_CURVE ( 2, ( #9345, #16009, #9763, #39748, #23368, #29204, #12776 ),
 .UNSPECIFIED., .F., .F. ) 
 B_SPLINE_CURVE_WITH_KNOTS ( ( 3, 2, 2, 3 ),
 ( 0.7686567164179105571, 0.7699004975124379424, 0.7711442786069654387, 0.7723880597014927130 ),
 .UNSPECIFIED. ) 
 CURVE ( )  GEOMETRIC_REPRESENTATION_ITEM ( )  RATIONAL_B_SPLINE_CURVE ( ( 0.9999999999999880096, 0.8660254037844506980, 1.000000000000000000, 0.8660254037844387076, 1.000000000000000000, 0.8660254037844148378, 1.000000000000023981 ) ) 
 REPRESENTATION_ITEM ( '' )  );
#22964=CYLINDRICAL_SURFACE ( 'NONE', #33186, 9.999999999999998224 ) ;
#22966=CARTESIAN_POINT ( 'NONE',  ( 5.000000000000000000, 8.660254037844385522, -156.2500000000000000 ) ) ;
#22967=CARTESIAN_POINT ( 'NONE',  ( -10.81189881249999729, 1.324075727343319199E-15, -159.7812500020484094 ) ) ;
#22968=CARTESIAN_POINT ( 'NONE',  ( -10.81189881249999907, -6.242252689847864744, -139.9687500020483810 ) ) ;
#22969=CARTESIAN_POINT ( 'NONE',  ( 0.000000000000000000, 0.000000000000000000, -200.0000000000000000 ) ) ;
#22971=EDGE_LOOP ( 'NONE', ( #9746, #20732, #38847, #18564 ) ) ;
#22973=CARTESIAN_POINT ( 'NONE',  ( -10.81189881249999729, 6.242252689847871849, -68.40625000204840944 ) ) ;
#22976=CARTESIAN_POINT ( 'NONE',  ( 5.405949406249992428, -9.363379034771808662, -117.0937500020483810 ) ) ;
#22979=CARTESIAN_POINT ( 'NONE',  ( -2.293366432827344421E-15, -12.48450537969573659, -21.21875000204837036 ) ) ;
#22980=CARTESIAN_POINT ( 'NONE',  ( -5.405949406249996869, 9.363379034771805109, -198.8437500020484094 ) ) ;
#22981=CARTESIAN_POINT ( 'NONE',  ( -10.81189881249999907, -6.242252689847864744, -49.96875000204835970 ) ) ;
#22984=CARTESIAN_POINT ( 'NONE',  ( -5.405949406249996869, 9.363379034771805109, -177.8437500020483810 ) ) ;
#22985=CARTESIAN_POINT ( 'NONE',  ( -10.81189881249999729, 6.242252689847871849, -168.7187500020483810 ) ) ;
#22988=CARTESIAN_POINT ( 'NONE',  ( -4.999999999999996447, 8.660254037844387298, -187.8750000040967905 ) ) ;
#22990=CARTESIAN_POINT ( 'NONE',  ( -10.81189881249999729, 6.242252689847871849, -95.21875000204838102 ) ) ;
#22991=DIRECTION ( 'NONE',  ( -0.000000000000000000, -0.000000000000000000, 1.000000000000000000 ) ) ;
#22992=CARTESIAN_POINT ( 'NONE',  ( 5.405949406249999534, 9.363379034771803333, -71.78125000204838102 ) ) ;
#22993=CARTESIAN_POINT ( 'NONE',  ( 5.000000000000000000, 8.660254037844385522, -89.12500000409677625 ) ) ;
#22996=CARTESIAN_POINT ( 'NONE',  ( -2.293366432827344421E-15, -12.48450537969573659, -162.4062500020483810 ) ) ;
#22997=EDGE_CURVE ( 'NONE', #33637, #17527, #16698, .T. ) ;
#22999=CARTESIAN_POINT ( 'NONE',  ( 7.070501591499377789E-16, 11.54700538379251284, -141.5000000040967905 ) ) ;
#23001=( BOUNDED_CURVE ( )  B_SPLINE_CURVE ( 2, ( #14081, #7425, #14734, #1604, #23840, #27496, #27280 ),
 .UNSPECIFIED., .F., .F. ) 
 B_SPLINE_CURVE_WITH_KNOTS ( ( 3, 2, 2, 3 ),
 ( 0.3582089552238806873, 0.3594527363184080726, 0.3606965174129355134, 0.3619402985074628432 ),
 .UNSPECIFIED. ) 
 CURVE ( )  GEOMETRIC_REPRESENTATION_ITEM ( )  RATIONAL_B_SPLINE_CURVE ( ( 0.9999999999999880096, 0.8660254037844506980, 1.000000000000000000, 0.8660254037844387076, 1.000000000000000000, 0.8660254037844207220, 1.000000000000017986 ) ) 
 REPRESENTATION_ITEM ( '' )  );
#23002=ORIENTED_EDGE ( 'NONE', *, *, #38238, .F. ) ;
#23005=CARTESIAN_POINT ( 'NONE',  ( 7.644554776091147741E-16, 12.48450537969573659, -197.6562500020484379 ) ) ;
#23006=CARTESIAN_POINT ( 'NONE',  ( -2.121150477449813534E-15, -11.54700538379251284, -43.25000000409675494 ) ) ;
#23008=EDGE_LOOP ( 'NONE', ( #40568, #24581, #16399, #29141 ) ) ;
#23009=CARTESIAN_POINT ( 'NONE',  ( -2.121150477449813534E-15, -11.54700538379251284, -59.37500000000000000 ) ) ;
#23011=CARTESIAN_POINT ( 'NONE',  ( -9.999999999999998224, 5.773502691896259087, -69.25000000409677625 ) ) ;
#23013=CARTESIAN_POINT ( 'NONE',  ( -9.999999999999998224, 1.224646799147353059E-15, -145.2500000000000000 ) ) ;
#23015=CARTESIAN_POINT ( 'NONE',  ( -10.81189881249999729, 6.242252689847871849, -69.90625000204839523 ) ) ;
#23018=DIRECTION ( 'NONE',  ( 1.000000000000000000, 0.000000000000000000, 0.000000000000000000 ) ) ;
#23019=CARTESIAN_POINT ( 'NONE',  ( 10.81189881249999551, -6.242252689847874514, -186.1562500020484379 ) ) ;
#23022=CARTESIAN_POINT ( 'NONE',  ( -5.000000000000003553, -8.660254037844383745, -118.0000000000000000 ) ) ;
#23023=CARTESIAN_POINT ( 'NONE',  ( -8.675003188131697129, -4.974413003141672895, -0.0003472602639886801512 ) ) ;
#23025=CARTESIAN_POINT ( 'NONE',  ( -9.999999999999998224, 1.224646799147353059E-15, -166.2500000000000000 ) ) ;
#23026=CARTESIAN_POINT ( 'NONE',  ( 9.999999999999998224, 0.000000000000000000, -97.99999999999998579 ) ) ;
#23027=CARTESIAN_POINT ( 'NONE',  ( -5.405949406249996869, 9.363379034771805109, -92.53125000204838102 ) ) ;
#23028=VERTEX_POINT ( 'NONE', #26859 ) ;
#23033=CARTESIAN_POINT ( 'NONE',  ( 7.644554776091147741E-16, 12.48450537969573659, -30.96875000204835260 ) ) ;
#23034=CARTESIAN_POINT ( 'NONE',  ( 7.644554776091147741E-16, 12.48450537969573659, -23.65625000204838102 ) ) ;
#23035=CARTESIAN_POINT ( 'NONE',  ( 7.644554776091147741E-16, 12.48450537969573659, -74.46875000204838102 ) ) ;
#23036=FACE_OUTER_BOUND ( 'NONE', #18891, .T. ) ;
#23037=CARTESIAN_POINT ( 'NONE',  ( 7.644554776091147741E-16, 12.48450537969573659, -191.4687500020484094 ) ) ;
#23038=CARTESIAN_POINT ( 'NONE',  ( 0.000000000000000000, 0.000000000000000000, -200.0000000000000000 ) ) ;
#23040=CARTESIAN_POINT ( 'NONE',  ( -9.999999999999998224, 5.773502691896259087, -1.750000004096752049 ) ) ;
#23041=CARTESIAN_POINT ( 'NONE',  ( 5.000000000000000000, 8.660254037844385522, -50.12500000409675494 ) ) ;
#23042=CARTESIAN_POINT ( 'NONE',  ( 10.81189881249999729, 0.000000000000000000, -122.8437500020483952 ) ) ;
#23043=CARTESIAN_POINT ( 'NONE',  ( -5.405949406250003975, -9.363379034771801557, -98.03125000204839523 ) ) ;
#23044=EDGE_CURVE ( 'NONE', #29057, #5036, #34741, .T. ) ;
#23045=CARTESIAN_POINT ( 'NONE',  ( -5.405949406249996869, 9.363379034771805109, -108.8437500020483810 ) ) ;
#23048=CARTESIAN_POINT ( 'NONE',  ( -2.121150477449813534E-15, -11.54700538379251284, -163.2500000040967620 ) ) ;
#23050=CARTESIAN_POINT ( 'NONE',  ( -5.000000000000003553, -8.660254037844383745, -66.99999999999997158 ) ) ;
#23053=ADVANCED_FACE ( 'NONE', ( #40421 ), #30109, .T. ) ;
#23055=CYLINDRICAL_SURFACE ( 'NONE', #19444, 9.999999999999998224 ) ;
#23057=CARTESIAN_POINT ( 'NONE',  ( -5.000000000000003553, -8.660254037844383745, -149.5000000000000000 ) ) ;
#23059=CARTESIAN_POINT ( 'NONE',  ( 10.00000000000000000, 5.773502691896255534, -78.37499999999998579 ) ) ;
#23061=CARTESIAN_POINT ( 'NONE',  ( -2.121150477449813534E-15, -11.54700538379251284, -89.75000000409677625 ) ) ;
#23065=CARTESIAN_POINT ( 'NONE',  ( -5.405949406250003975, -9.363379034771801557, -95.03125000204838102 ) ) ;
#23066=VERTEX_POINT ( 'NONE', #10443 ) ;
#23068=CARTESIAN_POINT ( 'NONE',  ( -9.999999999999998224, 1.224646799147353059E-15, -200.0000000000000000 ) ) ;
#23070=EDGE_LOOP ( 'NONE', ( #18547, #40557, #31648, #22640 ) ) ;
#23071=CARTESIAN_POINT ( 'NONE',  ( -4.999999999999996447, 8.660254037844387298, -13.49999999999995737 ) ) ;
#23072=CARTESIAN_POINT ( 'NONE',  ( 5.000000000000000000, 8.660254037844385522, -148.7500000000000000 ) ) ;
#23075=EDGE_CURVE ( 'NONE', #19091, #11871, #6366, .T. ) ;
#23076=CARTESIAN_POINT ( 'NONE',  ( -9.999999999999998224, 5.773502691896259087, -190.3750000000000000 ) ) ;
#23077=CARTESIAN_POINT ( 'NONE',  ( -10.81189881249999729, 1.324075727343319199E-15, -120.7812500020483952 ) ) ;
#23079=CARTESIAN_POINT ( 'NONE',  ( 9.999999999999998224, 0.000000000000000000, -23.37500000409675849 ) ) ;
#23081=CARTESIAN_POINT ( 'NONE',  ( 7.644554776091147741E-16, 12.48450537969573659, -47.65625000204836681 ) ) ;
#23083=CARTESIAN_POINT ( 'NONE',  ( 5.405949406249992428, -9.363379034771808662, -94.59375000204838102 ) ) ;
#23084=CARTESIAN_POINT ( 'NONE',  ( 5.405949406249999534, 9.363379034771803333, -121.2812500020483952 ) ) ;
#23086=CARTESIAN_POINT ( 'NONE',  ( -9.999999999999998224, 1.224646799147353059E-15, -51.12500000409675494 ) ) ;
#23089=CARTESIAN_POINT ( 'NONE',  ( 4.999999999999992006, -8.660254037844389075, -26.24999999999996803 ) ) ;
#23090=CARTESIAN_POINT ( 'NONE',  ( -9.999999999999998224, 1.224646799147353059E-15, -13.62500000409674961 ) ) ;
#23091=CARTESIAN_POINT ( 'NONE',  ( 5.405949406249992428, -9.363379034771808662, -129.0937500020483810 ) ) ;
#23093=DIRECTION ( 'NONE',  ( -0.000000000000000000, -0.000000000000000000, 1.000000000000000000 ) ) ;
#23095=CARTESIAN_POINT ( 'NONE',  ( -2.121150477449813534E-15, -11.54700538379251284, -188.7500000040967905 ) ) ;
#23097=CARTESIAN_POINT ( 'NONE',  ( 5.405949406249999534, 9.363379034771803333, -190.2812500020484094 ) ) ;
#23099=CARTESIAN_POINT ( 'NONE',  ( 0.000000000000000000, 0.000000000000000000, -200.0000000000000000 ) ) ;
#23100=DIRECTION ( 'NONE',  ( -0.000000000000000000, -0.000000000000000000, 1.000000000000000000 ) ) ;
#23103=CARTESIAN_POINT ( 'NONE',  ( -10.81189881249999729, 6.242252689847871849, -57.71875000204836681 ) ) ;
#23104=CARTESIAN_POINT ( 'NONE',  ( -2.293366432827344421E-15, -12.48450537969573659, -46.71875000204835970 ) ) ;
#23106=CARTESIAN_POINT ( 'NONE',  ( 7.644554776091147741E-16, 12.48450537969573659, -14.65625000204836859 ) ) ;
#23110=CARTESIAN_POINT ( 'NONE',  ( 9.999999999999998224, 0.000000000000000000, -103.9999999999999858 ) ) ;
#23112=DIRECTION ( 'NONE',  ( -0.000000000000000000, -0.000000000000000000, 1.000000000000000000 ) ) ;
#23115=CARTESIAN_POINT ( 'NONE',  ( 10.81189881249999729, 0.000000000000000000, -117.0312500020483952 ) ) ;
#23118=CARTESIAN_POINT ( 'NONE',  ( 9.999999999999998224, 0.000000000000000000, -194.3750000040967905 ) ) ;
#23120=VERTEX_POINT ( 'NONE', #37423 ) ;
#23121=CARTESIAN_POINT ( 'NONE',  ( -4.999999999999996447, 8.660254037844387298, -37.49999999999997868 ) ) ;
#23123=CARTESIAN_POINT ( 'NONE',  ( 4.999999999999992006, -8.660254037844389075, -17.62500000409675138 ) ) ;
#23124=CARTESIAN_POINT ( 'NONE',  ( 7.644554776091147741E-16, 12.48450537969573659, -43.15625000204837391 ) ) ;
#23125=LINE ( 'NONE', #13804, #24943 ) ;
#23127=CARTESIAN_POINT ( 'NONE',  ( 5.000000000000000000, 8.660254037844385522, -156.6250000040967905 ) ) ;
#23128=CARTESIAN_POINT ( 'NONE',  ( 5.405949406249992428, -9.363379034771808662, -136.7812500020483810 ) ) ;
#23129=CARTESIAN_POINT ( 'NONE',  ( 10.81189881249999729, 0.000000000000000000, -139.5312500020484094 ) ) ;
#23131=CARTESIAN_POINT ( 'NONE',  ( 9.999999999999998224, 0.000000000000000000, -78.49999999999998579 ) ) ;
#23132=ORIENTED_EDGE ( 'NONE', *, *, #41755, .T. ) ;
#23133=EDGE_LOOP ( 'NONE', ( #25263, #31143, #18908, #22235 ) ) ;
#23135=CARTESIAN_POINT ( 'NONE',  ( 9.999999999999998224, 0.000000000000000000, -200.0000000000000000 ) ) ;
#23136=CARTESIAN_POINT ( 'NONE',  ( 5.405949406249992428, -9.363379034771808662, -172.5937500020484094 ) ) ;
#23137=CARTESIAN_POINT ( 'NONE',  ( 7.644554776091147741E-16, 12.48450537969573659, -21.96875000204837391 ) ) ;
#23139=CARTESIAN_POINT ( 'NONE',  ( 5.405949406249999534, 9.363379034771803333, -158.5937500020483810 ) ) ;
#23140=CARTESIAN_POINT ( 'NONE',  ( -5.405949406249996869, 9.363379034771805109, -147.8437500020483810 ) ) ;
#23141=CARTESIAN_POINT ( 'NONE',  ( 4.999999999999992006, -8.660254037844389075, -9.749999999999953815 ) ) ;
#23145=CARTESIAN_POINT ( 'NONE',  ( -10.81189881249999729, 6.242252689847871849, -15.71875000204835793 ) ) ;
#23148=AXIS2_PLACEMENT_3D ( 'NONE', #48, #35873, #32641 ) ;
#23151=CARTESIAN_POINT ( 'NONE',  ( 9.999999999999994671, -5.773502691896262640, -167.5000000040967905 ) ) ;
#23152=CARTESIAN_POINT ( 'NONE',  ( 5.405949406249992428, -9.363379034771808662, -72.09375000204836681 ) ) ;
#23153=CARTESIAN_POINT ( 'NONE',  ( -2.293366432827344421E-15, -12.48450537969573659, -42.40625000204837391 ) ) ;
#23156=CARTESIAN_POINT ( 'NONE',  ( -4.999999999999996447, 8.660254037844387298, -133.5000000000000000 ) ) ;
#23157=CARTESIAN_POINT ( 'NONE',  ( -10.81189881249999729, -6.242252689847864744, -135.6562500020484094 ) ) ;
#23159=CARTESIAN_POINT ( 'NONE',  ( 4.999999999999992006, -8.660254037844389075, -112.1250000040967763 ) ) ;
#23161=ORIENTED_EDGE ( 'NONE', *, *, #13888, .T. ) ;
#23164=CARTESIAN_POINT ( 'NONE',  ( 9.999999999999998224, 0.000000000000000000, -39.49999999999997868 ) ) ;
#23165=CARTESIAN_POINT ( 'NONE',  ( 7.644554776091147741E-16, 12.48450537969573659, -164.6562500020484094 ) ) ;
#23166=CARTESIAN_POINT ( 'NONE',  ( 10.00000000000000000, 5.773502691896255534, -45.75000000409676915 ) ) ;
#23169=CARTESIAN_POINT ( 'NONE',  ( -4.999999999999996447, 8.660254037844387298, -100.8750000040967905 ) ) ;
#23170=CARTESIAN_POINT ( 'NONE',  ( 10.81189881249999729, 0.000000000000000000, -165.0312500020484094 ) ) ;
#23171=CARTESIAN_POINT ( 'NONE',  ( 5.405949406249999534, 9.363379034771803333, -139.0937500020483810 ) ) ;
#23172=CARTESIAN_POINT ( 'NONE',  ( -2.121150477449813534E-15, -11.54700538379251284, -50.75000000409676204 ) ) ;
#23175=CARTESIAN_POINT ( 'NONE',  ( -5.000000000000003553, -8.660254037844383745, -78.99999999999998579 ) ) ;
#23176=VECTOR ( 'NONE', #42282, 1000.000000000000000 ) ;
#23177=EDGE_CURVE ( 'NONE', #28563, #4341, #1969, .T. ) ;
#23178=B_SPLINE_CURVE_WITH_KNOTS ( 'NONE', 3,
 ( #32447, #8923, #38696, #5897, #5256, #25962 ),
 .UNSPECIFIED., .F., .F.,
 ( 4, 2, 4 ),
 ( 0.000000000000000000, 0.004265001810245392516, 0.008530003620490783298 ),
 .UNSPECIFIED. ) ;
#23179=CARTESIAN_POINT ( 'NONE',  ( -2.293366432827344421E-15, -12.48450537969573659, -73.90625000204836681 ) ) ;
#23182=CARTESIAN_POINT ( 'NONE',  ( -2.293366432827344421E-15, -12.48450537969573659, -120.2187500020483952 ) ) ;
#23184=ORIENTED_EDGE ( 'NONE', *, *, #36231, .F. ) ;
#23185=CARTESIAN_POINT ( 'NONE',  ( 10.81189881249999729, 6.242252689847867408, -22.21875000204837747 ) ) ;
#23186=CARTESIAN_POINT ( 'NONE',  ( 10.81189881249999551, -6.242252689847874514, -196.4687500020484094 ) ) ;
#23187=CARTESIAN_POINT ( 'NONE',  ( -10.81189881249999729, 6.242252689847871849, -44.21875000204836681 ) ) ;
#23190=CARTESIAN_POINT ( 'NONE',  ( -5.405949406250003975, -9.363379034771801557, -178.8437500020483810 ) ) ;
#23191=CARTESIAN_POINT ( 'NONE',  ( -10.81189881249999907, -6.242252689847864744, -165.4687500020484094 ) ) ;
#23193=EDGE_CURVE ( 'NONE', #10633, #36222, #3337, .T. ) ;
#23198=CARTESIAN_POINT ( 'NONE',  ( 7.644554776091147741E-16, 12.48450537969573659, -99.96875000204839523 ) ) ;
#23199=EDGE_CURVE ( 'NONE', #26946, #21791, #2232, .T. ) ;
#23200=CARTESIAN_POINT ( 'NONE',  ( -2.121150477449813534E-15, -11.54700538379251284, -101.3750000000000000 ) ) ;
#23201=CARTESIAN_POINT ( 'NONE',  ( 10.81189881249999729, 0.000000000000000000, -63.03125000204837391 ) ) ;
#23204=CARTESIAN_POINT ( 'NONE',  ( 5.405949406249999534, 9.363379034771803333, -119.7812500020483952 ) ) ;
#23205=CARTESIAN_POINT ( 'NONE',  ( 10.81189881249999551, -6.242252689847874514, -163.6562500020484094 ) ) ;
#23206=( BOUNDED_CURVE ( )  B_SPLINE_CURVE ( 2, ( #27643, #40151, #33492, #21155, #898, #27860, #34128 ),
 .UNSPECIFIED., .F., .F. ) 
 B_SPLINE_CURVE_WITH_KNOTS ( ( 3, 2, 2, 3 ),
 ( 0.1194029850746269744, 0.1206467661691543042, 0.1218905472636816062, 0.1231343283582089221 ),
 .UNSPECIFIED. ) 
 CURVE ( )  GEOMETRIC_REPRESENTATION_ITEM ( )  RATIONAL_B_SPLINE_CURVE ( ( 0.9999999999999880096, 0.8660254037844506980, 1.000000000000000000, 0.8660254037844387076, 1.000000000000000000, 0.8660254037844417052, 0.9999999999999970024 ) ) 
 REPRESENTATION_ITEM ( '' )  );
#23208=CARTESIAN_POINT ( 'NONE',  ( -5.000000000000003553, -8.660254037844383745, -140.8750000040967905 ) ) ;
#23214=CARTESIAN_POINT ( 'NONE',  ( 5.405949406249999534, 9.363379034771803333, -199.2812500020484094 ) ) ;
#23215=CARTESIAN_POINT ( 'NONE',  ( 10.00000000000051159, -5.773502691895965988, -43.00000000409674072 ) ) ;
#23217=ORIENTED_EDGE ( 'NONE', *, *, #40022, .T. ) ;
#23218=CARTESIAN_POINT ( 'NONE',  ( 10.00000000000000000, 5.773502691896255534, -55.87499999999997158 ) ) ;
#23220=CARTESIAN_POINT ( 'NONE',  ( -4.999999999999996447, 8.660254037844387298, -66.37500000409676204 ) ) ;
#23221=FACE_OUTER_BOUND ( 'NONE', #8173, .T. ) ;
#23224=CARTESIAN_POINT ( 'NONE',  ( -10.81189881249999729, -6.242252689847864744, -59.15625000204838813 ) ) ;
#23227=CARTESIAN_POINT ( 'NONE',  ( 0.000000000000000000, 0.000000000000000000, -200.0000000000000000 ) ) ;
#23228=CARTESIAN_POINT ( 'NONE',  ( -5.405949406249996869, 9.363379034771805109, -182.5312500020484094 ) ) ;
#23230=CARTESIAN_POINT ( 'NONE',  ( 6.964452268037472749, 6.964452268037473637, -201.2186212422413689 ) ) ;
#23233=CARTESIAN_POINT ( 'NONE',  ( -6.454000741078234960, 7.688134883229009731, -0.000000000000000000 ) ) ;
#23234=CARTESIAN_POINT ( 'NONE',  ( 4.999999999999992006, -8.660254037844389075, -170.2500000000000000 ) ) ;
#23235=CARTESIAN_POINT ( 'NONE',  ( -5.000000000000003553, -8.660254037844383745, -137.8750000040967905 ) ) ;
#23236=CARTESIAN_POINT ( 'NONE',  ( -10.81189881249999907, -6.242252689847864744, -95.15625000204839523 ) ) ;
#23237=ORIENTED_EDGE ( 'NONE', *, *, #3528, .T. ) ;
#23238=ADVANCED_FACE ( 'NONE', ( #21442 ), #1608, .T. ) ;
#23240=ORIENTED_EDGE ( 'NONE', *, *, #32291, .F. ) ;
#23242=CARTESIAN_POINT ( 'NONE',  ( 7.644554776091147741E-16, 12.48450537969573659, -36.96875000204835970 ) ) ;
#23243=CARTESIAN_POINT ( 'NONE',  ( 10.81189881249999729, 0.000000000000000000, -25.53125000204836681 ) ) ;
#23245=CARTESIAN_POINT ( 'NONE',  ( 7.644554776091147741E-16, 12.48450537969573659, -69.96875000204838102 ) ) ;
#23247=CARTESIAN_POINT ( 'NONE',  ( -5.405949406249996869, 9.363379034771805109, -194.3437500020484094 ) ) ;
#23248=CARTESIAN_POINT ( 'NONE',  ( 10.81189881249999729, 0.000000000000000000, -152.8437500020483810 ) ) ;
#23253=CARTESIAN_POINT ( 'NONE',  ( -9.999999999999998224, 1.224646799147353059E-15, -6.125000004096770034 ) ) ;
#23254=CARTESIAN_POINT ( 'NONE',  ( 0.000000000000000000, 0.000000000000000000, -200.0000000000000000 ) ) ;
#23255=CARTESIAN_POINT ( 'NONE',  ( -10.81189881249999729, 1.324075727343319199E-15, -117.5937500020483810 ) ) ;
#23256=CARTESIAN_POINT ( 'NONE',  ( 5.405949406249992428, -9.363379034771808662, -87.28125000204838102 ) ) ;
#23257=CARTESIAN_POINT ( 'NONE',  ( 10.81189881249999729, 6.242252689847867408, -110.7187500020483810 ) ) ;
#23260=CARTESIAN_POINT ( 'NONE',  ( 5.000000000000000000, 8.660254037844385522, -161.1250000040967905 ) ) ;
#23261=( BOUNDED_CURVE ( )  B_SPLINE_CURVE ( 2, ( #30740, #30951, #8498, #14513, #21651, #14078, #27276 ),
 .UNSPECIFIED., .F., .F. ) 
 B_SPLINE_CURVE_WITH_KNOTS ( ( 3, 2, 2, 3 ),
 ( 0.1044776119402986148, 0.1057213930348259306, 0.1069651741293532465, 0.1082089552238805485 ),
 .UNSPECIFIED. ) 
 CURVE ( )  GEOMETRIC_REPRESENTATION_ITEM ( )  RATIONAL_B_SPLINE_CURVE ( ( 0.9999999999999880096, 0.8660254037844506980, 1.000000000000000000, 0.8660254037844387076, 1.000000000000000000, 0.8660254037844431485, 0.9999999999999955591 ) ) 
 REPRESENTATION_ITEM ( '' )  );
#23265=CARTESIAN_POINT ( 'NONE',  ( -9.999999999999998224, 1.224646799147353059E-15, -190.2500000000000000 ) ) ;
#23267=CARTESIAN_POINT ( 'NONE',  ( 4.999999999999992006, -8.660254037844389075, -149.2500000000000000 ) ) ;
#23269=CARTESIAN_POINT ( 'NONE',  ( -9.999999999999998224, 5.773502691896259087, -80.87499999999998579 ) ) ;
#23271=CARTESIAN_POINT ( 'NONE',  ( 7.070501591499377789E-16, 11.54700538379251284, -92.00000000409677625 ) ) ;
#23274=CARTESIAN_POINT ( 'NONE',  ( 10.81189881249999729, 0.000000000000000000, -84.03125000204838102 ) ) ;
#23275=ORIENTED_EDGE ( 'NONE', *, *, #1854, .F. ) ;
#23280=CARTESIAN_POINT ( 'NONE',  ( 9.999999999999996447, -5.773502691896262640, -9.624999999999982236 ) ) ;
#23281=CARTESIAN_POINT ( 'NONE',  ( 7.070501591499377789E-16, 11.54700538379251284, -145.6250000000000284 ) ) ;
#23282=CARTESIAN_POINT ( 'NONE',  ( 9.999999999999998224, 0.000000000000000000, -96.87500000409677625 ) ) ;
#23284=CARTESIAN_POINT ( 'NONE',  ( -2.121150477449813534E-15, -11.54700538379251284, -191.3750000000000284 ) ) ;
#23285=DIRECTION ( 'NONE',  ( 1.000000000000000000, 0.000000000000000000, 0.000000000000000000 ) ) ;
#23286=CARTESIAN_POINT ( 'NONE',  ( 5.405949406249999534, 9.363379034771803333, -115.2812500020483952 ) ) ;
#23290=AXIS2_PLACEMENT_3D ( 'NONE', #16687, #13236, #26637 ) ;
#23291=EDGE_CURVE ( 'NONE', #23881, #33268, #32849, .T. ) ;
#23294=CARTESIAN_POINT ( 'NONE',  ( 10.81189881249999551, -6.242252689847874514, -49.65625000204837391 ) ) ;
#23296=CARTESIAN_POINT ( 'NONE',  ( -10.81189881249999907, -6.242252689847864744, -93.46875000204836681 ) ) ;
#23297=CARTESIAN_POINT ( 'NONE',  ( 7.644554776091147741E-16, 12.48450537969573659, -122.6562500020483952 ) ) ;
#23298=ORIENTED_EDGE ( 'NONE', *, *, #42648, .F. ) ;
#23299=CARTESIAN_POINT ( 'NONE',  ( -5.000000000000003553, -8.660254037844383745, -111.9999999999999858 ) ) ;
#23305=CARTESIAN_POINT ( 'NONE',  ( 7.644554776091147741E-16, 12.48450537969573659, -132.9687500020483810 ) ) ;
#23307=CARTESIAN_POINT ( 'NONE',  ( 7.070501591499376803E-16, 11.54700538379251284, -116.0000000040967905 ) ) ;
#23309=CARTESIAN_POINT ( 'NONE',  ( 4.999999999999992006, -8.660254037844389075, -185.6250000040967905 ) ) ;
#23311=CARTESIAN_POINT ( 'NONE',  ( -10.81189881249999729, 1.324075727343319199E-15, -189.7812500020484094 ) ) ;
#23312=CARTESIAN_POINT ( 'NONE',  ( -9.999999999999998224, 1.224646799147353059E-15, -200.0000000000000000 ) ) ;
#23316=ADVANCED_FACE ( 'NONE', ( #26338 ), #20, .T. ) ;
#23317=CARTESIAN_POINT ( 'NONE',  ( -10.81189881249999729, 6.242252689847871849, -60.71875000204837391 ) ) ;
#23318=CARTESIAN_POINT ( 'NONE',  ( 7.644554776091147741E-16, 12.48450537969573659, -51.96875000204836681 ) ) ;
#23320=CARTESIAN_POINT ( 'NONE',  ( 10.81189881249999551, -6.242252689847874514, -16.65625000204837747 ) ) ;
#23324=CARTESIAN_POINT ( 'NONE',  ( -5.000000000000003553, -8.660254037844383745, -107.4999999999999858 ) ) ;
#23328=DIRECTION ( 'NONE',  ( 1.000000000000000000, 0.000000000000000000, 0.000000000000000000 ) ) ;
#23331=CARTESIAN_POINT ( 'NONE',  ( 7.644554776091147741E-16, 12.48450537969573659, -113.6562500020483952 ) ) ;
#23332=ORIENTED_EDGE ( 'NONE', *, *, #13919, .F. ) ;
#23335=CARTESIAN_POINT ( 'NONE',  ( -9.999999999999998224, 1.224646799147353059E-15, -200.0000000000000000 ) ) ;
#23338=CARTESIAN_POINT ( 'NONE',  ( -9.999999999999998224, 5.773502691896259087, -32.87499999999997158 ) ) ;
#23340=CARTESIAN_POINT ( 'NONE',  ( -2.121150477449813534E-15, -11.54700538379251284, -17.75000000409676559 ) ) ;
#23341=CARTESIAN_POINT ( 'NONE',  ( -2.293366432827344421E-15, -12.48450537969573659, -45.40625000204837391 ) ) ;
#23342=EDGE_CURVE ( 'NONE', #3545, #4655, #30075, .T. ) ;
#23343=CARTESIAN_POINT ( 'NONE',  ( -9.999999999999998224, 1.224646799147353059E-15, -2.749999999999974687 ) ) ;
#23346=CARTESIAN_POINT ( 'NONE',  ( -10.81189881249999729, 6.242252689847871849, -141.9062500020484094 ) ) ;
#23347=CARTESIAN_POINT ( 'NONE',  ( -9.999999999999227285, -5.773502691896698735, -110.6249999999999574 ) ) ;
#23348=EDGE_LOOP ( 'NONE', ( #28936, #31914, #3154, #22546 ) ) ;
#23351=ORIENTED_EDGE ( 'NONE', *, *, #38580, .T. ) ;
#23353=DIRECTION ( 'NONE',  ( -0.000000000000000000, -0.000000000000000000, 1.000000000000000000 ) ) ;
#23354=CARTESIAN_POINT ( 'NONE',  ( -9.999999999999998224, 1.224646799147353059E-15, -163.2500000000000000 ) ) ;
#23355=CARTESIAN_POINT ( 'NONE',  ( 10.81189881249999551, -6.242252689847874514, -172.4687500020484094 ) ) ;
#23356=CARTESIAN_POINT ( 'NONE',  ( 10.81189881249999551, -6.242252689847874514, -20.96875000204836681 ) ) ;
#23358=FACE_OUTER_BOUND ( 'NONE', #17692, .T. ) ;
#23359=CARTESIAN_POINT ( 'NONE',  ( -10.81189881249999729, -6.242252689847864744, -154.9687500020484094 ) ) ;
#23360=CARTESIAN_POINT ( 'NONE',  ( -10.81189881249999729, 6.242252689847871849, -144.7187500020483810 ) ) ;
#23364=CARTESIAN_POINT ( 'NONE',  ( -10.81189881249999729, 6.242252689847871849, -11.21875000204836859 ) ) ;
#23366=EDGE_CURVE ( 'NONE', #2600, #41098, #29575, .T. ) ;
#23368=CARTESIAN_POINT ( 'NONE',  ( -4.999999999999996447, 8.660254037844387298, -43.87500000409677625 ) ) ;
#23370=CARTESIAN_POINT ( 'NONE',  ( 7.070501591499376803E-16, 11.54700538379251284, -99.50000000409679046 ) ) ;
#23371=CARTESIAN_POINT ( 'NONE',  ( 5.405949406249992428, -9.363379034771808662, -75.09375000204838102 ) ) ;
#23372=CARTESIAN_POINT ( 'NONE',  ( 5.405949406249999534, 9.363379034771803333, -40.28125000204838102 ) ) ;
#23376=CARTESIAN_POINT ( 'NONE',  ( -4.999999999999996447, 8.660254037844387298, -126.0000000000000000 ) ) ;
#23377=CARTESIAN_POINT ( 'NONE',  ( -2.293366432827344421E-15, -12.48450537969573659, -136.9062500020484094 ) ) ;
#23378=CARTESIAN_POINT ( 'NONE',  ( 9.999999999999998224, 0.000000000000000000, -200.0000000000000000 ) ) ;
#23379=CARTESIAN_POINT ( 'NONE',  ( 9.999999999999996447, -5.773502691896262640, -116.5000000040967763 ) ) ;
#23386=CARTESIAN_POINT ( 'NONE',  ( -5.405949406249996869, 9.363379034771805109, -167.5312500020484094 ) ) ;
#23387=CARTESIAN_POINT ( 'NONE',  ( 5.000000000000000000, 8.660254037844385522, -39.62500000409676915 ) ) ;
#23388=CARTESIAN_POINT ( 'NONE',  ( -10.00000000000038547, 5.773502691896036154, -154.7500000040967905 ) ) ;
#23390=CARTESIAN_POINT ( 'NONE',  ( 9.999999999999998224, 0.000000000000000000, -73.99999999999998579 ) ) ;
#23391=CARTESIAN_POINT ( 'NONE',  ( -5.405949406249996869, 9.363379034771805109, -160.0312500020484094 ) ) ;
#23392=CARTESIAN_POINT ( 'NONE',  ( -10.81189881249999729, 6.242252689847871849, -134.2187500020483810 ) ) ;
#23393=CARTESIAN_POINT ( 'NONE',  ( 4.999999999999992006, -8.660254037844389075, -50.62500000409675494 ) ) ;
#23394=VERTEX_POINT ( 'NONE', #36262 ) ;
#23395=CARTESIAN_POINT ( 'NONE',  ( 9.999999999999998224, 0.000000000000000000, -189.5000000000000000 ) ) ;
#23397=CARTESIAN_POINT ( 'NONE',  ( 10.81189881249999729, 0.000000000000000000, -72.03125000204838102 ) ) ;
#23398=ORIENTED_EDGE ( 'NONE', *, *, #33406, .F. ) ;
#23400=CARTESIAN_POINT ( 'NONE',  ( 5.405949406249992428, -9.363379034771808662, -121.5937500020483952 ) ) ;
#23401=ORIENTED_EDGE ( 'NONE', *, *, #37566, .F. ) ;
#23402=CARTESIAN_POINT ( 'NONE',  ( 5.405949406249999534, 9.363379034771803333, -17.59375000204835260 ) ) ;
#23403=UNCERTAINTY_MEASURE_WITH_UNIT (LENGTH_MEASURE( 1.000000000000000082E-05 ), #11537, 'distance_accuracy_value', 'NONE');
#23404=CARTESIAN_POINT ( 'NONE',  ( -10.81189881249999907, -6.242252689847864744, -198.4687500020484379 ) ) ;
#23405=CARTESIAN_POINT ( 'NONE',  ( 10.81189881249999551, -6.242252689847874514, -43.46875000204836681 ) ) ;
#23407=CARTESIAN_POINT ( 'NONE',  ( 0.000000000000000000, 0.000000000000000000, -200.0000000000000000 ) ) ;
#23408=CARTESIAN_POINT ( 'NONE',  ( 10.00000000000102318, -5.773502691895667560, -10.00000000409673184 ) ) ;
#23409=CARTESIAN_POINT ( 'NONE',  ( 10.81189881249999729, 0.000000000000000000, -176.8437500020483810 ) ) ;
#23410=CARTESIAN_POINT ( 'NONE',  ( 5.405949406249999534, 9.363379034771803333, -172.0937500020484094 ) ) ;
#23414=CARTESIAN_POINT ( 'NONE',  ( 7.070501591499376803E-16, 11.54700538379251284, -194.0000000040968189 ) ) ;
#23416=VECTOR ( 'NONE', #25576, 1000.000000000000000 ) ;
#23417=CARTESIAN_POINT ( 'NONE',  ( -2.293366432827344421E-15, -12.48450537969573659, -100.7187500020483952 ) ) ;
#23419=CARTESIAN_POINT ( 'NONE',  ( -10.81189881249999729, 6.242252689847871849, -66.90625000204839523 ) ) ;
#23421=CARTESIAN_POINT ( 'NONE',  ( -5.405949406249996869, 9.363379034771805109, -122.5312500020483952 ) ) ;
#23422=CARTESIAN_POINT ( 'NONE',  ( 5.405949406249999534, 9.363379034771803333, -160.2812500020484094 ) ) ;
#23424=CARTESIAN_POINT ( 'NONE',  ( 10.00000000000000000, 5.773502691896255534, -141.7500000040967905 ) ) ;
#23426=ADVANCED_FACE ( 'NONE', ( #33252 ), #8721, .T. ) ;
#23427=ORIENTED_EDGE ( 'NONE', *, *, #929, .T. ) ;
#23430=CARTESIAN_POINT ( 'NONE',  ( 5.405949406249992428, -9.363379034771808662, -187.7812500020484094 ) ) ;
#23431=CARTESIAN_POINT ( 'NONE',  ( 17.32050807568890960, 1.173974112367310985E-14, 49.99999999999998579 ) ) ;
#23433=ORIENTED_EDGE ( 'NONE', *, *, #38294, .F. ) ;
#23434=CARTESIAN_POINT ( 'NONE',  ( -9.999999999999998224, 1.224646799147353059E-15, -58.24999999999997158 ) ) ;
#23436=CARTESIAN_POINT ( 'NONE',  ( 4.999999999999992006, -8.660254037844389075, -64.12500000409676204 ) ) ;
#23437=CARTESIAN_POINT ( 'NONE',  ( -9.999999999999227285, -5.773502691896698735, -109.5000000040967478 ) ) ;
#23438=CARTESIAN_POINT ( 'NONE',  ( 11.54700538379250396, 20.00000000000000711, 49.99999999999998579 ) ) ;
#23440=CARTESIAN_POINT ( 'NONE',  ( 5.405949406249992428, -9.363379034771808662, -60.28125000204836681 ) ) ;
#23444=CARTESIAN_POINT ( 'NONE',  ( 10.81189881249999551, -6.242252689847874514, -183.1562500020484094 ) ) ;
#23446=CARTESIAN_POINT ( 'NONE',  ( -10.00000000000102496, 5.773502691895664007, -85.37499999999994316 ) ) ;
#23447=CARTESIAN_POINT ( 'NONE',  ( -9.999999999999998224, 1.224646799147353059E-15, -200.0000000000000000 ) ) ;
#23448=CARTESIAN_POINT ( 'NONE',  ( 0.000000000000000000, 0.000000000000000000, -200.0000000000000000 ) ) ;
#23450=CARTESIAN_POINT ( 'NONE',  ( -5.000000000000003553, -8.660254037844383745, -167.5000000000000000 ) ) ;
#23451=CARTESIAN_POINT ( 'NONE',  ( -2.121150477449813534E-15, -11.54700538379251284, -62.37499999999997158 ) ) ;
#23453=CARTESIAN_POINT ( 'NONE',  ( -10.81189881249999729, 1.324075727343319199E-15, -95.28125000204838102 ) ) ;
#23455=CARTESIAN_POINT ( 'NONE',  ( -10.00000000000154188, 5.773502691895366468, -82.75000000409673362 ) ) ;
#23459=EDGE_CURVE ( 'NONE', #1402, #7087, #35054, .T. ) ;
#23460=CARTESIAN_POINT ( 'NONE',  ( 10.81189881249999729, 0.000000000000000000, -37.34375000204836681 ) ) ;
#23461=CARTESIAN_POINT ( 'NONE',  ( -5.405949406250003975, -9.363379034771801557, -24.53125000204836681 ) ) ;
#23462=CARTESIAN_POINT ( 'NONE',  ( 5.405949406249999534, 9.363379034771803333, -68.59375000204836681 ) ) ;
#23463=CARTESIAN_POINT ( 'NONE',  ( 9.999999999999998224, 0.000000000000000000, -73.99999999999998579 ) ) ;
#23465=CARTESIAN_POINT ( 'NONE',  ( -2.293366432827344421E-15, -12.48450537969573659, -195.2187500020484094 ) ) ;
#23466=CARTESIAN_POINT ( 'NONE',  ( 10.81189881249999907, 6.242252689847868297, -151.2187500020483810 ) ) ;
#23468=CARTESIAN_POINT ( 'NONE',  ( 10.00000000000000000, 5.773502691896255534, -132.7500000040967905 ) ) ;
#23471=CARTESIAN_POINT ( 'NONE',  ( -9.999999999999998224, 5.773502691896259087, -3.250000004096759376 ) ) ;
#23472=CARTESIAN_POINT ( 'NONE',  ( -4.999999999999996447, 8.660254037844387298, -49.87500000409675494 ) ) ;
#23473=CARTESIAN_POINT ( 'NONE',  ( 7.644554776091147741E-16, 12.48450537969573659, -122.4687500020483952 ) ) ;
#23475=CARTESIAN_POINT ( 'NONE',  ( -10.81189881249999907, -6.242252689847864744, -93.65625000204840944 ) ) ;
#23476=CARTESIAN_POINT ( 'NONE',  ( 7.644554776091147741E-16, 12.48450537969573659, -105.9687500020483668 ) ) ;
#23479=CARTESIAN_POINT ( 'NONE',  ( -2.121150477449813534E-15, -11.54700538379251284, -158.7500000040968189 ) ) ;
#23482=AXIS2_PLACEMENT_3D ( 'NONE', #21481, #17802, #11328 ) ;
#23487=CARTESIAN_POINT ( 'NONE',  ( -4.999999999999996447, 8.660254037844387298, -83.99999999999997158 ) ) ;
#23489=CARTESIAN_POINT ( 'NONE',  ( 10.00000000000000000, 5.773502691896255534, -86.25000000409677625 ) ) ;
#23490=VECTOR ( 'NONE', #35968, 1000.000000000000000 ) ;
#23491=CARTESIAN_POINT ( 'NONE',  ( 4.999999999999992006, -8.660254037844389075, -95.62500000409677625 ) ) ;
#23493=CARTESIAN_POINT ( 'NONE',  ( -10.81189881249999729, 1.324075727343319199E-15, -86.28125000204838102 ) ) ;
#23498=ORIENTED_EDGE ( 'NONE', *, *, #1806, .F. ) ;
#23499=CARTESIAN_POINT ( 'NONE',  ( -10.00000000000000000, -5.773502691896251982, -5.624999999999962697 ) ) ;
#23501=CARTESIAN_POINT ( 'NONE',  ( 4.999999999999992006, -8.660254037844389075, -149.2500000000000000 ) ) ;
#23502=CARTESIAN_POINT ( 'NONE',  ( -2.121150477449813534E-15, -11.54700538379251284, -14.75000000409676737 ) ) ;
#23504=CARTESIAN_POINT ( 'NONE',  ( 5.000000000000000000, 8.660254037844385522, -192.2500000000000000 ) ) ;
#23505=DIRECTION ( 'NONE',  ( 1.000000000000000000, -0.000000000000000000, -0.000000000000000000 ) ) ;
#23506=CARTESIAN_POINT ( 'NONE',  ( -10.81189881249999907, -6.242252689847864744, -117.6562500020483952 ) ) ;
#23507=ORIENTED_EDGE ( 'NONE', *, *, #3499, .T. ) ;
#23508=CARTESIAN_POINT ( 'NONE',  ( -9.999999999998969713, -5.773502691896847949, -75.00000000409674783 ) ) ;
#23509=ORIENTED_EDGE ( 'NONE', *, *, #22094, .F. ) ;
#23510=( BOUNDED_CURVE ( )  B_SPLINE_CURVE ( 2, ( #4121, #17260, #30464, #891, #26364, #41201, #11640 ),
 .UNSPECIFIED., .F., .F. ) 
 B_SPLINE_CURVE_WITH_KNOTS ( ( 3, 2, 2, 3 ),
 ( 0.5410447761194030480, 0.5422885572139304333, 0.5435323383084578186, 0.5447761194029852039 ),
 .UNSPECIFIED. ) 
 CURVE ( )  GEOMETRIC_REPRESENTATION_ITEM ( )  RATIONAL_B_SPLINE_CURVE ( ( 0.9999999999999880096, 0.8660254037844506980, 1.000000000000000000, 0.8660254037844387076, 1.000000000000000000, 0.8660254037844267172, 1.000000000000011990 ) ) 
 REPRESENTATION_ITEM ( '' )  );
#23511=CARTESIAN_POINT ( 'NONE',  ( 10.81189881249999551, -6.242252689847874514, -48.15625000204836681 ) ) ;
#23514=CARTESIAN_POINT ( 'NONE',  ( 10.81189881249999729, 0.000000000000000000, -95.84375000204838102 ) ) ;
#23515=CARTESIAN_POINT ( 'NONE',  ( 7.644554776091147741E-16, 12.48450537969573659, -121.1562500020483952 ) ) ;
#23516=ORIENTED_EDGE ( 'NONE', *, *, #1421, .F. ) ;
#23521=CARTESIAN_POINT ( 'NONE',  ( -9.999999999999998224, 1.224646799147353059E-15, -200.0000000000000000 ) ) ;
#23522=CARTESIAN_POINT ( 'NONE',  ( 5.405949406249999534, 9.363379034771803333, -131.5937500020483810 ) ) ;
#23526=CARTESIAN_POINT ( 'NONE',  ( 9.999999999999996447, -5.773502691896262640, -182.5000000040968189 ) ) ;
#23528=CARTESIAN_POINT ( 'NONE',  ( -10.81189881249999729, 6.242252689847871849, -179.4062500020484094 ) ) ;
#23532=CARTESIAN_POINT ( 'NONE',  ( -10.81189881249999729, 6.242252689847871849, -62.21875000204838813 ) ) ;
#23533=CARTESIAN_POINT ( 'NONE',  ( 10.81189881249999907, 6.242252689847868297, -44.71875000204837391 ) ) ;
#23535=CARTESIAN_POINT ( 'NONE',  ( -5.405949406250003975, -9.363379034771801557, -20.03125000204836326 ) ) ;
#23537=CYLINDRICAL_SURFACE ( 'NONE', #37131, 9.999999999999998224 ) ;
#23539=EDGE_CURVE ( 'NONE', #6043, #22060, #35270, .T. ) ;
#23540=CARTESIAN_POINT ( 'NONE',  ( -10.00000000000000000, -5.773502691896251982, -109.1249999999999858 ) ) ;
#23542=CARTESIAN_POINT ( 'NONE',  ( -9.999999999999998224, 1.224646799147353059E-15, -169.2500000000000000 ) ) ;
#23543=ADVANCED_FACE ( 'NONE', ( #18632 ), #18854, .T. ) ;
#23546=CARTESIAN_POINT ( 'NONE',  ( 5.405949406249992428, -9.363379034771808662, -111.2812500020483810 ) ) ;
#23547=ORIENTED_EDGE ( 'NONE', *, *, #39722, .F. ) ;
#23548=CARTESIAN_POINT ( 'NONE',  ( 9.999999999999872102, 5.773502691896329253, -160.8750000000000000 ) ) ;
#23550=CARTESIAN_POINT ( 'NONE',  ( -9.999999999999227285, -5.773502691896698735, -136.5000000040967620 ) ) ;
#23552=VERTEX_POINT ( 'NONE', #2462 ) ;
#23553=CARTESIAN_POINT ( 'NONE',  ( 4.999999999999992006, -8.660254037844389075, -33.74999999999997158 ) ) ;
#23555=CARTESIAN_POINT ( 'NONE',  ( -5.405949406249996869, 9.363379034771805109, -38.53125000204838102 ) ) ;
#23556=CARTESIAN_POINT ( 'NONE',  ( 9.999999999999998224, 0.000000000000000000, -111.8750000040967763 ) ) ;
#23559=VECTOR ( 'NONE', #34444, 1000.000000000000000 ) ;
#23560=CARTESIAN_POINT ( 'NONE',  ( 7.644554776091147741E-16, 12.48450537969573659, -145.1562500020484094 ) ) ;
#23561=CARTESIAN_POINT ( 'NONE',  ( -9.999999999999742428, -5.773502691896402084, -120.0000000040967905 ) ) ;
#23562=EDGE_LOOP ( 'NONE', ( #41695, #3918, #35353, #26098 ) ) ;
#23564=EDGE_CURVE ( 'NONE', #2600, #18939, #6615, .T. ) ;
#23565=DIRECTION ( 'NONE',  ( 1.000000000000000000, 0.000000000000000000, 0.000000000000000000 ) ) ;
#23566=LINE ( 'NONE', #3492, #8402 ) ;
#23567=CARTESIAN_POINT ( 'NONE',  ( -2.293366432827344421E-15, -12.48450537969573659, -162.2187500020483810 ) ) ;
#23569=CARTESIAN_POINT ( 'NONE',  ( -10.81189881249999729, 1.324075727343319199E-15, -20.09375000204835615 ) ) ;
#23570=CARTESIAN_POINT ( 'NONE',  ( -9.999999999999998224, 1.224646799147353059E-15, -200.0000000000000000 ) ) ;
#23571=CARTESIAN_POINT ( 'NONE',  ( 9.999999999999998224, 0.000000000000000000, -156.8750000040967905 ) ) ;
#23572=CARTESIAN_POINT ( 'NONE',  ( -10.81189881249999729, -6.242252689847864744, -159.4687500020484094 ) ) ;
#23573=CARTESIAN_POINT ( 'NONE',  ( -10.81189881249999729, 6.242252689847871849, -140.2187500020483810 ) ) ;
#23574=CARTESIAN_POINT ( 'NONE',  ( 9.999999999998969713, 5.773502691896851502, -67.87499999999998579 ) ) ;
#23578=CARTESIAN_POINT ( 'NONE',  ( -5.405949406250003975, -9.363379034771801557, -9.343750002048345493 ) ) ;
#23581=CARTESIAN_POINT ( 'NONE',  ( 9.999999999999998224, 0.000000000000000000, -125.3750000040967905 ) ) ;
#23583=CARTESIAN_POINT ( 'NONE',  ( -9.999999999999998224, 1.224646799147353059E-15, -17.74999999999996092 ) ) ;
#23585=CARTESIAN_POINT ( 'NONE',  ( 7.644554776091147741E-16, 12.48450537969573659, -86.46875000204838102 ) ) ;
#23586=CARTESIAN_POINT ( 'NONE',  ( 5.405949406249999534, 9.363379034771803333, -62.59375000204836681 ) ) ;
#23587=CARTESIAN_POINT ( 'NONE',  ( -5.405949406249996869, 9.363379034771805109, -46.03125000204838813 ) ) ;
#23589=CARTESIAN_POINT ( 'NONE',  ( 9.999999999999998224, 0.000000000000000000, -113.3750000040967763 ) ) ;
#23592=CARTESIAN_POINT ( 'NONE',  ( 10.00000000000000000, 5.773502691896255534, -127.8749999999999858 ) ) ;
#23593=CARTESIAN_POINT ( 'NONE',  ( -5.405949406249996869, 9.363379034771805109, -142.0312500020483810 ) ) ;
#23594=( BOUNDED_CURVE ( )  B_SPLINE_CURVE ( 2, ( #42097, #8257, #34589, #28115, #11682, #28323, #41463 ),
 .UNSPECIFIED., .F., .F. ) 
 B_SPLINE_CURVE_WITH_KNOTS ( ( 3, 2, 2, 3 ),
 ( 0.7835820895522389584, 0.7848258706467662327, 0.7860696517412937290, 0.7873134328358211143 ),
 .UNSPECIFIED. ) 
 CURVE ( )  GEOMETRIC_REPRESENTATION_ITEM ( )  RATIONAL_B_SPLINE_CURVE ( ( 0.9999999999999880096, 0.8660254037844506980, 1.000000000000000000, 0.8660254037844387076, 1.000000000000000000, 0.8660254037844148378, 1.000000000000023981 ) ) 
 REPRESENTATION_ITEM ( '' )  );
#23595=CARTESIAN_POINT ( 'NONE',  ( -9.999999999999998224, 1.224646799147353059E-15, -200.0000000000000000 ) ) ;
#23597=CARTESIAN_POINT ( 'NONE',  ( -2.293366432827344421E-15, -12.48450537969573659, -15.40625000204837391 ) ) ;
#23599=ORIENTED_EDGE ( 'NONE', *, *, #28324, .T. ) ;
#23602=CARTESIAN_POINT ( 'NONE',  ( -9.999999999999998224, 1.224646799147353059E-15, -56.74999999999996447 ) ) ;
#23604=CARTESIAN_POINT ( 'NONE',  ( -9.999999999999998224, 1.224646799147353059E-15, -42.12500000409677625 ) ) ;
#23605=CARTESIAN_POINT ( 'NONE',  ( 10.00000000000051159, -5.773502691895965988, -91.00000000409676204 ) ) ;
#23607=VECTOR ( 'NONE', #22826, 1000.000000000000000 ) ;
#23608=CARTESIAN_POINT ( 'NONE',  ( 10.81189881249999551, -6.242252689847874514, -153.1562500020484379 ) ) ;
#23609=CARTESIAN_POINT ( 'NONE',  ( -10.81189881249999729, 6.242252689847871849, -135.7187500020483810 ) ) ;
#23610=CARTESIAN_POINT ( 'NONE',  ( -5.000000000000003553, -8.660254037844383745, -33.99999999999997158 ) ) ;
#23613=CARTESIAN_POINT ( 'NONE',  ( 9.999999999999998224, 0.000000000000000000, -200.0000000000000000 ) ) ;
#23616=CARTESIAN_POINT ( 'NONE',  ( -10.81189881249999729, 6.242252689847871849, -63.90625000204836681 ) ) ;
#23617=ORIENTED_EDGE ( 'NONE', *, *, #29653, .F. ) ;
#23619=CARTESIAN_POINT ( 'NONE',  ( 10.81189881249999729, 0.000000000000000000, -115.3437500020483810 ) ) ;
#23620=VERTEX_POINT ( 'NONE', #40534 ) ;
#23621=CARTESIAN_POINT ( 'NONE',  ( -5.405949406249996869, 9.363379034771805109, -24.84375000204835970 ) ) ;
#23622=CARTESIAN_POINT ( 'NONE',  ( 10.81189881249999907, 6.242252689847868297, -194.7187500020484094 ) ) ;
#23623=CARTESIAN_POINT ( 'NONE',  ( -10.81189881249999729, 6.242252689847871849, -47.21875000204836681 ) ) ;
#23624=CARTESIAN_POINT ( 'NONE',  ( -9.999999999999998224, 1.224646799147353059E-15, -156.1250000040967905 ) ) ;
#23625=CARTESIAN_POINT ( 'NONE',  ( 5.000000000000000000, 8.660254037844385522, -152.1250000040967905 ) ) ;
#23626=CARTESIAN_POINT ( 'NONE',  ( 10.81189881249999729, 0.000000000000000000, -179.8437500020483810 ) ) ;
#23627=CARTESIAN_POINT ( 'NONE',  ( 7.644554776091147741E-16, 12.48450537969573659, -158.4687500020483810 ) ) ;
#23629=( BOUNDED_CURVE ( )  B_SPLINE_CURVE ( 2, ( #18482, #1887, #38129, #8572, #31670, #2104, #41569 ),
 .UNSPECIFIED., .F., .F. ) 
 B_SPLINE_CURVE_WITH_KNOTS ( ( 3, 2, 2, 3 ),
 ( 0.7947761194029852039, 0.7960199004975125892, 0.7972636815920399744, 0.7985074626865673597 ),
 .UNSPECIFIED. ) 
 CURVE ( )  GEOMETRIC_REPRESENTATION_ITEM ( )  RATIONAL_B_SPLINE_CURVE ( ( 0.9999999999999880096, 0.8660254037844506980, 1.000000000000000000, 0.8660254037844387076, 1.000000000000000000, 0.8660254037844148378, 1.000000000000023981 ) ) 
 REPRESENTATION_ITEM ( '' )  );
#23631=CARTESIAN_POINT ( 'NONE',  ( -9.999999999999479527, -5.773502691896549521, -118.5000000040967763 ) ) ;
#23634=CARTESIAN_POINT ( 'NONE',  ( 10.81189881249999729, 0.000000000000000000, -95.84375000204838102 ) ) ;
#23635=CARTESIAN_POINT ( 'NONE',  ( 4.999999999999992006, -8.660254037844389075, -72.74999999999998579 ) ) ;
#23636=CARTESIAN_POINT ( 'NONE',  ( 7.644554776091147741E-16, 12.48450537969573659, -68.65625000204840944 ) ) ;
#23637=CARTESIAN_POINT ( 'NONE',  ( 10.00000000000051159, -5.773502691895965988, -97.00000000409676204 ) ) ;
#23639=CARTESIAN_POINT ( 'NONE',  ( -10.81189881249999729, 6.242252689847871849, -119.4062500020483952 ) ) ;
#23640=CARTESIAN_POINT ( 'NONE',  ( 5.405949406249999534, 9.363379034771803333, -158.7812500020484094 ) ) ;
#23642=CARTESIAN_POINT ( 'NONE',  ( 10.00000000000000000, 5.773502691896255534, -140.2500000040967905 ) ) ;
#23647=CARTESIAN_POINT ( 'NONE',  ( 7.644554776091147741E-16, 12.48450537969573659, -187.1562500020484094 ) ) ;
#23650=CARTESIAN_POINT ( 'NONE',  ( 7.070501591499377789E-16, 11.54700538379251284, -46.62499999999996447 ) ) ;
#23652=CARTESIAN_POINT ( 'NONE',  ( 4.999999999999992006, -8.660254037844389075, -65.62500000409676204 ) ) ;
#23653=CARTESIAN_POINT ( 'NONE',  ( -4.999999999999996447, 8.660254037844387298, -153.0000000000000000 ) ) ;
#23655=CARTESIAN_POINT ( 'NONE',  ( 7.644554776091147741E-16, 12.48450537969573659, -61.15625000204838102 ) ) ;
#23658=CYLINDRICAL_SURFACE ( 'NONE', #39332, 9.999999999999998224 ) ;
#23659=CARTESIAN_POINT ( 'NONE',  ( -10.81189881249999729, 6.242252689847871849, -185.4062500020484094 ) ) ;
#23662=CARTESIAN_POINT ( 'NONE',  ( 5.000000000000000000, 8.660254037844385522, -40.74999999999997868 ) ) ;
#23666=DIRECTION ( 'NONE',  ( -0.000000000000000000, -0.000000000000000000, 1.000000000000000000 ) ) ;
#23667=CARTESIAN_POINT ( 'NONE',  ( 10.81189881249999551, -6.242252689847874514, -90.15625000204836681 ) ) ;
#23668=ORIENTED_EDGE ( 'NONE', *, *, #14285, .T. ) ;
#23669=CARTESIAN_POINT ( 'NONE',  ( -9.999999999999998224, 1.224646799147353059E-15, -82.62500000409676204 ) ) ;
#23672=VERTEX_POINT ( 'NONE', #33670 ) ;
#23673=CARTESIAN_POINT ( 'NONE',  ( 5.405949406249992428, -9.363379034771808662, -25.59375000204835970 ) ) ;
#23674=CARTESIAN_POINT ( 'NONE',  ( 7.644554776091147741E-16, 12.48450537969573659, -22.15625000204837391 ) ) ;
#23675=CARTESIAN_POINT ( 'NONE',  ( 5.405949406249992428, -9.363379034771808662, -73.59375000204838102 ) ) ;
#23676=DIRECTION ( 'NONE',  ( -0.000000000000000000, -0.000000000000000000, 1.000000000000000000 ) ) ;
#23678=CARTESIAN_POINT ( 'NONE',  ( 10.81189881249999729, 0.000000000000000000, -191.8437500020484094 ) ) ;
#23679=CARTESIAN_POINT ( 'NONE',  ( -10.81189881249999729, 1.324075727343319199E-15, -153.5937500020483810 ) ) ;
#23681=DIRECTION ( 'NONE',  ( 1.000000000000000000, 0.000000000000000000, 0.000000000000000000 ) ) ;
#23683=CARTESIAN_POINT ( 'NONE',  ( 9.999999999999998224, 0.000000000000000000, -2.375000004096766482 ) ) ;
#23684=CARTESIAN_POINT ( 'NONE',  ( 9.999999999999998224, 0.000000000000000000, -60.87500000409676204 ) ) ;
#23685=CARTESIAN_POINT ( 'NONE',  ( -2.293366432827344421E-15, -12.48450537969573659, -118.7187500020483952 ) ) ;
#23687=CARTESIAN_POINT ( 'NONE',  ( 10.81189881249999551, -6.242252689847874514, -87.15625000204838102 ) ) ;
#23688=CARTESIAN_POINT ( 'NONE',  ( 7.644554776091147741E-16, 12.48450537969573659, -99.96875000204836681 ) ) ;
#23691=CARTESIAN_POINT ( 'NONE',  ( 5.000000000000000000, 8.660254037844385522, -162.6250000040967905 ) ) ;
#23696=CARTESIAN_POINT ( 'NONE',  ( 9.999999999999998224, 0.000000000000000000, -200.0000000000000000 ) ) ;
#23698=CARTESIAN_POINT ( 'NONE',  ( -5.000000000000003553, -8.660254037844383745, -78.99999999999998579 ) ) ;
#23700=CARTESIAN_POINT ( 'NONE',  ( 9.999999999999996447, -5.773502691896262640, -86.50000000409676204 ) ) ;
#23701=DIRECTION ( 'NONE',  ( 1.000000000000000000, 0.000000000000000000, 0.000000000000000000 ) ) ;
#23703=CARTESIAN_POINT ( 'NONE',  ( -10.81189881249999729, 6.242252689847871849, -80.40625000204838102 ) ) ;
#23706=ORIENTED_EDGE ( 'NONE', *, *, #36218, .F. ) ;
#23707=CARTESIAN_POINT ( 'NONE',  ( -2.121150477449813534E-15, -11.54700538379251284, -11.37499999999995737 ) ) ;
#23709=CARTESIAN_POINT ( 'NONE',  ( -2.121150477449813534E-15, -11.54700538379251284, -144.8750000000000000 ) ) ;
#23710=CARTESIAN_POINT ( 'NONE',  ( 9.999999999998969713, 5.773502691896851502, -45.75000000409674783 ) ) ;
#23712=CARTESIAN_POINT ( 'NONE',  ( -9.999999999999998224, 5.773502691896259087, -191.8750000000000000 ) ) ;
#23713=LINE ( 'NONE', #33438, #14422 ) ;
#23714=CARTESIAN_POINT ( 'NONE',  ( 7.644554776091147741E-16, 12.48450537969573659, -115.1562500020483952 ) ) ;
#23716=CARTESIAN_POINT ( 'NONE',  ( -4.999999999999996447, 8.660254037844387298, -22.87500000409675849 ) ) ;
#23718=( BOUNDED_CURVE ( )  B_SPLINE_CURVE ( 2, ( #21903, #18657, #6147, #35508, #8959, #19289, #12383 ),
 .UNSPECIFIED., .F., .F. ) 
 B_SPLINE_CURVE_WITH_KNOTS ( ( 3, 2, 2, 3 ),
 ( 0.7276119402985077311, 0.7288557213930350054, 0.7300995024875623907, 0.7313432835820897759 ),
 .UNSPECIFIED. ) 
 CURVE ( )  GEOMETRIC_REPRESENTATION_ITEM ( )  RATIONAL_B_SPLINE_CURVE ( ( 0.9999999999999761302, 0.8660254037844625774, 1.000000000000000000, 0.8660254037844387076, 1.000000000000000000, 0.8660254037844148378, 1.000000000000023981 ) ) 
 REPRESENTATION_ITEM ( '' )  );
#23720=EDGE_CURVE ( 'NONE', #6, #30360, #20981, .T. ) ;
#23721=CARTESIAN_POINT ( 'NONE',  ( -10.81189881249999729, 1.324075727343319199E-15, -42.78125000204838102 ) ) ;
#23723=CARTESIAN_POINT ( 'NONE',  ( -10.81189881249999729, 6.242252689847871849, -92.21875000204838102 ) ) ;
#23724=CARTESIAN_POINT ( 'NONE',  ( -5.405949406250003975, -9.363379034771801557, -126.5312500020483952 ) ) ;
#23725=EDGE_LOOP ( 'NONE', ( #7260, #35817, #42474, #41153 ) ) ;
#23726=FACE_OUTER_BOUND ( 'NONE', #8062, .T. ) ;
#23727=CARTESIAN_POINT ( 'NONE',  ( 10.81189881249999729, 6.242252689847867408, -196.2187500020484094 ) ) ;
#23730=CARTESIAN_POINT ( 'NONE',  ( -10.81189881249999729, 1.324075727343319199E-15, -120.5937500020483952 ) ) ;
#23734=CARTESIAN_POINT ( 'NONE',  ( 9.999999999999998224, 0.000000000000000000, -188.3750000040967905 ) ) ;
#23736=CARTESIAN_POINT ( 'NONE',  ( 10.81189881249999729, 6.242252689847867408, -179.9062500020484094 ) ) ;
#23740=CARTESIAN_POINT ( 'NONE',  ( 10.81189881249999729, 0.000000000000000000, -58.34375000204835970 ) ) ;
#23741=CARTESIAN_POINT ( 'NONE',  ( -10.81189881249999907, -6.242252689847864744, -39.46875000204835970 ) ) ;
#23743=CARTESIAN_POINT ( 'NONE',  ( 10.81189881249999729, 0.000000000000000000, -15.03125000204835793 ) ) ;
#23747=CARTESIAN_POINT ( 'NONE',  ( 7.070501591499377789E-16, 11.54700538379251284, -103.6249999999999858 ) ) ;
#23749=CARTESIAN_POINT ( 'NONE',  ( -5.000000000000003553, -8.660254037844383745, -49.37500000409678336 ) ) ;
#23752=CARTESIAN_POINT ( 'NONE',  ( -2.293366432827344421E-15, -12.48450537969573659, -111.4062500020483952 ) ) ;
#23756=CARTESIAN_POINT ( 'NONE',  ( -9.999999999999998224, 1.224646799147353059E-15, -136.6250000040967620 ) ) ;
#23758=ORIENTED_EDGE ( 'NONE', *, *, #4523, .T. ) ;
#23759=CARTESIAN_POINT ( 'NONE',  ( -4.999999999999996447, 8.660254037844387298, -32.99999999999997158 ) ) ;
#23760=CARTESIAN_POINT ( 'NONE',  ( -5.405949406250003975, -9.363379034771801557, -38.03125000204838102 ) ) ;
#23761=CARTESIAN_POINT ( 'NONE',  ( 9.999999999999998224, 0.000000000000000000, -200.0000000000000000 ) ) ;
#23763=( BOUNDED_CURVE ( )  B_SPLINE_CURVE ( 2, ( #16451, #9572, #22112, #26408, #26196, #35286, #16236 ),
 .UNSPECIFIED., .F., .F. ) 
 B_SPLINE_CURVE_WITH_KNOTS ( ( 3, 2, 2, 3 ),
 ( 0.7462686567164180662, 0.7475124378109453405, 0.7487562189054727257, 0.7500000000000001110 ),
 .UNSPECIFIED. ) 
 CURVE ( )  GEOMETRIC_REPRESENTATION_ITEM ( )  RATIONAL_B_SPLINE_CURVE ( ( 0.9999999999999880096, 0.8660254037844506980, 1.000000000000000000, 0.8660254037844387076, 1.000000000000000000, 0.8660254037844267172, 1.000000000000011990 ) ) 
 REPRESENTATION_ITEM ( '' )  );
#23764=DIRECTION ( 'NONE',  ( -1.000000000000000000, 0.000000000000000000, 0.000000000000000000 ) ) ;
#23765=CARTESIAN_POINT ( 'NONE',  ( 10.81189881249999551, -6.242252689847874514, -145.6562500020484094 ) ) ;
#23769=EDGE_CURVE ( 'NONE', #15394, #25371, #26759, .T. ) ;
#23770=EDGE_LOOP ( 'NONE', ( #9952, #20450, #33538, #36602 ) ) ;
#23772=FACE_OUTER_BOUND ( 'NONE', #23972, .T. ) ;
#23773=CARTESIAN_POINT ( 'NONE',  ( 10.81189881249999729, 0.000000000000000000, -167.8437500020484094 ) ) ;
#23774=VECTOR ( 'NONE', #20566, 1000.000000000000000 ) ;
#23776=CARTESIAN_POINT ( 'NONE',  ( 10.81189881249999907, 6.242252689847868297, -19.21875000204837747 ) ) ;
#23777=CYLINDRICAL_SURFACE ( 'NONE', #12244, 9.999999999999998224 ) ;
#23778=CARTESIAN_POINT ( 'NONE',  ( -2.293366432827344421E-15, -12.48450537969573659, -154.7187500020483810 ) ) ;
#23779=CARTESIAN_POINT ( 'NONE',  ( -2.293366432827344421E-15, -12.48450537969573659, -136.7187500020483810 ) ) ;
#23780=CARTESIAN_POINT ( 'NONE',  ( 5.405949406249992428, -9.363379034771808662, -103.7812500020483810 ) ) ;
#23784=CARTESIAN_POINT ( 'NONE',  ( 10.81189881249999551, -6.242252689847874514, -7.468750002048351710 ) ) ;
#23786=CARTESIAN_POINT ( 'NONE',  ( -5.405949406249996869, 9.363379034771805109, -199.0312500020484094 ) ) ;
#23787=CARTESIAN_POINT ( 'NONE',  ( -9.999999999999479527, -5.773502691896549521, -97.12499999999997158 ) ) ;
#23790=CARTESIAN_POINT ( 'NONE',  ( 5.405949406249999534, 9.363379034771803333, -83.59375000204836681 ) ) ;
#23791=CARTESIAN_POINT ( 'NONE',  ( 10.81189881249999729, 0.000000000000000000, -65.84375000204836681 ) ) ;
#23793=CARTESIAN_POINT ( 'NONE',  ( 10.81189881249999551, -6.242252689847874514, -43.65625000204838102 ) ) ;
#23797=CARTESIAN_POINT ( 'NONE',  ( -2.121150477449813534E-15, -11.54700538379251284, -132.8750000000000000 ) ) ;
#23798=CARTESIAN_POINT ( 'NONE',  ( -2.293366432827344421E-15, -12.48450537969573659, -130.9062500020483810 ) ) ;
#23800=VECTOR ( 'NONE', #13453, 1000.000000000000000 ) ;
#23802=CARTESIAN_POINT ( 'NONE',  ( 10.81189881249999729, 0.000000000000000000, -18.03125000204835970 ) ) ;
#23803=ORIENTED_EDGE ( 'NONE', *, *, #36968, .T. ) ;
#23806=CARTESIAN_POINT ( 'NONE',  ( -5.000000000000003553, -8.660254037844383745, -185.5000000000000000 ) ) ;
#23807=CARTESIAN_POINT ( 'NONE',  ( 4.999999999999992006, -8.660254037844389075, -37.12500000409676915 ) ) ;
#23808=CARTESIAN_POINT ( 'NONE',  ( 9.999999999999998224, 0.000000000000000000, -102.5000000000000000 ) ) ;
#23810=AXIS2_PLACEMENT_3D ( 'NONE', #37546, #40134, #36902 ) ;
#23812=CARTESIAN_POINT ( 'NONE',  ( 5.405949406249999534, 9.363379034771803333, -154.2812500020484094 ) ) ;
#23813=CARTESIAN_POINT ( 'NONE',  ( -2.293366432827344421E-15, -12.48450537969573659, -138.2187500020483810 ) ) ;
#23814=ORIENTED_EDGE ( 'NONE', *, *, #36492, .F. ) ;
#23815=CARTESIAN_POINT ( 'NONE',  ( 9.999999999999998224, 0.000000000000000000, -200.0000000000000000 ) ) ;
#23816=ORIENTED_EDGE ( 'NONE', *, *, #39722, .T. ) ;
#23817=CARTESIAN_POINT ( 'NONE',  ( 5.405949406249992428, -9.363379034771808662, -60.28125000204836681 ) ) ;
#23818=VERTEX_POINT ( 'NONE', #14419 ) ;
#23821=CARTESIAN_POINT ( 'NONE',  ( 10.81189881249999907, 6.242252689847868297, -110.7187500020483810 ) ) ;
#23822=ORIENTED_EDGE ( 'NONE', *, *, #38083, .T. ) ;
#23823=EDGE_CURVE ( 'NONE', #18936, #40403, #4376, .T. ) ;
#23825=VECTOR ( 'NONE', #37631, 1000.000000000000000 ) ;
#23826=EDGE_CURVE ( 'NONE', #4273, #29829, #22273, .T. ) ;
#23827=CARTESIAN_POINT ( 'NONE',  ( -10.81189881249999729, -6.242252689847864744, -18.46875000204837036 ) ) ;
#23828=CARTESIAN_POINT ( 'NONE',  ( -5.405949406249996869, 9.363379034771805109, -192.8437500020484094 ) ) ;
#23830=CARTESIAN_POINT ( 'NONE',  ( 5.405949406249999534, 9.363379034771803333, -40.09375000204837391 ) ) ;
#23833=CARTESIAN_POINT ( 'NONE',  ( -10.81189881249999729, -6.242252689847864744, -178.9687500020484094 ) ) ;
#23834=AXIS2_PLACEMENT_3D ( 'NONE', #32482, #9372, #5508 ) ;
#23835=CARTESIAN_POINT ( 'NONE',  ( -5.405949406249996869, 9.363379034771805109, -162.8437500020484094 ) ) ;
#23840=CARTESIAN_POINT ( 'NONE',  ( -4.999999999999996447, 8.660254037844387298, -126.3750000040967905 ) ) ;
#23841=DIRECTION ( 'NONE',  ( 1.000000000000000000, 0.000000000000000000, 0.000000000000000000 ) ) ;
#23843=CARTESIAN_POINT ( 'NONE',  ( 5.405949406249992428, -9.363379034771808662, -91.59375000204838102 ) ) ;
#23845=CARTESIAN_POINT ( 'NONE',  ( -10.81189881249999907, -6.242252689847864744, -68.15625000204840944 ) ) ;
#23846=DIRECTION ( 'NONE',  ( -0.000000000000000000, -0.000000000000000000, 1.000000000000000000 ) ) ;
#23848=EDGE_CURVE ( 'NONE', #18780, #28714, #24023, .T. ) ;
#23849=CARTESIAN_POINT ( 'NONE',  ( -2.293366432827344421E-15, -12.48450537969573659, -126.4062500020483952 ) ) ;
#23850=CARTESIAN_POINT ( 'NONE',  ( -5.405949406249996869, 9.363379034771805109, -161.5312500020484094 ) ) ;
#23852=CARTESIAN_POINT ( 'NONE',  ( -9.999999999999998224, 1.224646799147353059E-15, -127.6250000040967620 ) ) ;
#23854=VERTEX_POINT ( 'NONE', #18816 ) ;
#23858=EDGE_CURVE ( 'NONE', #41098, #26093, #39134, .T. ) ;
#23859=CARTESIAN_POINT ( 'NONE',  ( 7.644554776091147741E-16, 12.48450537969573659, -185.6562500020484094 ) ) ;
#23861=ORIENTED_EDGE ( 'NONE', *, *, #28450, .F. ) ;
#23862=CARTESIAN_POINT ( 'NONE',  ( 7.070501591499377789E-16, 11.54700538379251284, -49.62499999999997868 ) ) ;
#23864=CARTESIAN_POINT ( 'NONE',  ( 10.00000000000000000, 5.773502691896255534, -63.75000000409679046 ) ) ;
#23865=CARTESIAN_POINT ( 'NONE',  ( 0.000000000000000000, 0.000000000000000000, -200.0000000000000000 ) ) ;
#23866=DIRECTION ( 'NONE',  ( -0.000000000000000000, -0.000000000000000000, 1.000000000000000000 ) ) ;
#23868=CARTESIAN_POINT ( 'NONE',  ( 5.405949406249992428, -9.363379034771808662, -63.28125000204837391 ) ) ;
#23871=CARTESIAN_POINT ( 'NONE',  ( 9.999999999999998224, 0.000000000000000000, -29.37500000409676204 ) ) ;
#23872=CARTESIAN_POINT ( 'NONE',  ( 5.405949406249992428, -9.363379034771808662, -178.7812500020484094 ) ) ;
#23874=CARTESIAN_POINT ( 'NONE',  ( 9.999999999999998224, 0.000000000000000000, -200.0000000000000000 ) ) ;
#23876=ADVANCED_FACE ( 'NONE', ( #32630 ), #16182, .T. ) ;
#23878=CARTESIAN_POINT ( 'NONE',  ( 9.999999999999998224, 0.000000000000000000, -153.5000000000000000 ) ) ;
#23879=CARTESIAN_POINT ( 'NONE',  ( 4.999999999999992006, -8.660254037844389075, -169.1250000040967905 ) ) ;
#23880=CARTESIAN_POINT ( 'NONE',  ( -2.293366432827344421E-15, -12.48450537969573659, -82.90625000204838102 ) ) ;
#23881=VERTEX_POINT ( 'NONE', #12947 ) ;
#23883=LINE ( 'NONE', #14561, #26159 ) ;
#23886=VERTEX_POINT ( 'NONE', #42313 ) ;
#23888=CARTESIAN_POINT ( 'NONE',  ( 5.405949406249999534, 9.363379034771803333, -25.09375000204835970 ) ) ;
#23889=CARTESIAN_POINT ( 'NONE',  ( 5.405949406249992428, -9.363379034771808662, -12.28125000204835438 ) ) ;
#23890=CARTESIAN_POINT ( 'NONE',  ( 10.81189881249999729, 0.000000000000000000, -73.34375000204838102 ) ) ;
#23891=CARTESIAN_POINT ( 'NONE',  ( 5.000000000000000000, 8.660254037844385522, -164.1250000040967905 ) ) ;
#23893=CARTESIAN_POINT ( 'NONE',  ( -2.293366432827344421E-15, -12.48450537969573659, -186.2187500020484094 ) ) ;
#23896=CARTESIAN_POINT ( 'NONE',  ( 5.405949406249999534, 9.363379034771803333, -2.593750002048367254 ) ) ;
#23897=DIRECTION ( 'NONE',  ( -0.000000000000000000, -0.000000000000000000, 1.000000000000000000 ) ) ;
#23901=CARTESIAN_POINT ( 'NONE',  ( -10.00000000000102496, 5.773502691895664007, -60.25000000409674783 ) ) ;
#23902=EDGE_CURVE ( 'NONE', #15830, #17639, #3057, .T. ) ;
#23903=CARTESIAN_POINT ( 'NONE',  ( 10.81189881249999551, -6.242252689847874514, -113.9687500020483810 ) ) ;
#23904=CARTESIAN_POINT ( 'NONE',  ( -9.999999999999998224, 1.224646799147353059E-15, -200.0000000000000000 ) ) ;
#23905=CARTESIAN_POINT ( 'NONE',  ( -10.81189881249999907, -6.242252689847864744, -90.65625000204836681 ) ) ;
#23906=CARTESIAN_POINT ( 'NONE',  ( 10.81189881249999729, 0.000000000000000000, -100.3437500020483810 ) ) ;
#23909=CARTESIAN_POINT ( 'NONE',  ( 9.999999999999996447, -5.773502691896262640, -160.0000000040968189 ) ) ;
#23913=CARTESIAN_POINT ( 'NONE',  ( -9.999999999999998224, 1.224646799147353059E-15, -200.0000000000000000 ) ) ;
#23915=CARTESIAN_POINT ( 'NONE',  ( -9.999999999999998224, 1.224646799147353059E-15, -76.62500000409677625 ) ) ;
#23916=CARTESIAN_POINT ( 'NONE',  ( 5.000000000000000000, 8.660254037844385522, -70.74999999999998579 ) ) ;
#23918=CARTESIAN_POINT ( 'NONE',  ( 9.999999999999996447, -5.773502691896262640, -92.50000000409677625 ) ) ;
#23919=CARTESIAN_POINT ( 'NONE',  ( 5.000000000000000000, 8.660254037844385522, -115.7499999999999858 ) ) ;
#23921=CARTESIAN_POINT ( 'NONE',  ( 10.81189881249999729, 6.242252689847867408, -82.40625000204836681 ) ) ;
#23926=CARTESIAN_POINT ( 'NONE',  ( 5.405949406249999534, 9.363379034771803333, -197.7812500020484094 ) ) ;
#23928=CARTESIAN_POINT ( 'NONE',  ( -5.405949406249996869, 9.363379034771805109, -15.84375000204835082 ) ) ;
#23929=CARTESIAN_POINT ( 'NONE',  ( -5.000000000000003553, -8.660254037844383745, -14.87500000409674961 ) ) ;
#23931=CARTESIAN_POINT ( 'NONE',  ( -2.293366432827344421E-15, -12.48450537969573659, -138.4062500020483810 ) ) ;
#23932=CARTESIAN_POINT ( 'NONE',  ( 7.070501591499377789E-16, 11.54700538379251284, -190.6250000000000000 ) ) ;
#23934=CARTESIAN_POINT ( 'NONE',  ( -10.81189881249999729, 6.242252689847871849, -111.9062500020483810 ) ) ;
#23935=VERTEX_POINT ( 'NONE', #38455 ) ;
#23939=CARTESIAN_POINT ( 'NONE',  ( -5.405949406250003975, -9.363379034771801557, -44.03125000204838102 ) ) ;
#23941=CARTESIAN_POINT ( 'NONE',  ( -10.81189881249999729, 6.242252689847871849, -98.21875000204838102 ) ) ;
#23942=CARTESIAN_POINT ( 'NONE',  ( 7.070501591499376803E-16, 11.54700538379251284, -128.0000000040967905 ) ) ;
#23944=CARTESIAN_POINT ( 'NONE',  ( -10.81189881249999729, 6.242252689847871849, -192.7187500020483810 ) ) ;
#23946=CARTESIAN_POINT ( 'NONE',  ( 10.00000000000000000, 5.773502691896255534, -138.3750000000000000 ) ) ;
#23947=EDGE_CURVE ( 'NONE', #32856, #4745, #22880, .T. ) ;
#23948=CARTESIAN_POINT ( 'NONE',  ( -2.293366432827344421E-15, -12.48450537969573659, -126.2187500020483952 ) ) ;
#23950=CARTESIAN_POINT ( 'NONE',  ( -9.999999999999998224, 1.224646799147353059E-15, -44.74999999999998579 ) ) ;
#23952=CARTESIAN_POINT ( 'NONE',  ( 10.00000000000000000, 5.773502691896255534, -189.7500000040968189 ) ) ;
#23954=CARTESIAN_POINT ( 'NONE',  ( -10.81189881249999729, 6.242252689847871849, -182.4062500020484094 ) ) ;
#23955=CARTESIAN_POINT ( 'NONE',  ( 7.070501591499376803E-16, 11.54700538379251284, -180.1250000000000000 ) ) ;
#23956=CARTESIAN_POINT ( 'NONE',  ( -9.999999999999998224, 1.224646799147353059E-15, -181.2500000000000284 ) ) ;
#23958=CARTESIAN_POINT ( 'NONE',  ( 5.405949406249992428, -9.363379034771808662, -51.09375000204835260 ) ) ;
#23959=CARTESIAN_POINT ( 'NONE',  ( 10.81189881249999729, 0.000000000000000000, -41.84375000204837391 ) ) ;
#23961=CARTESIAN_POINT ( 'NONE',  ( -10.81189881249999729, 6.242252689847871849, -12.90625000204835970 ) ) ;
#23965=CARTESIAN_POINT ( 'NONE',  ( -4.999999999999996447, 8.660254037844387298, -94.49999999999998579 ) ) ;
#23970=CARTESIAN_POINT ( 'NONE',  ( 7.644554776091147741E-16, 12.48450537969573659, -104.6562500020483810 ) ) ;
#23972=EDGE_LOOP ( 'NONE', ( #25886, #26840, #24899, #3760 ) ) ;
#23973=DIRECTION ( 'NONE',  ( 1.000000000000000000, 0.000000000000000000, 0.000000000000000000 ) ) ;
#23975=CARTESIAN_POINT ( 'NONE',  ( -9.999999999999998224, 1.224646799147353059E-15, -91.24999999999998579 ) ) ;
#23977=ORIENTED_EDGE ( 'NONE', *, *, #39591, .T. ) ;
#23978=CARTESIAN_POINT ( 'NONE',  ( -9.999999999999998224, 5.773502691896259087, -35.87499999999995737 ) ) ;
#23980=CARTESIAN_POINT ( 'NONE',  ( 10.81189881249999551, -6.242252689847874514, -33.15625000204835970 ) ) ;
#23981=CARTESIAN_POINT ( 'NONE',  ( 5.000000000000000000, 8.660254037844385522, -35.12500000409676915 ) ) ;
#23982=( BOUNDED_CURVE ( )  B_SPLINE_CURVE ( 2, ( #9632, #26045, #16938, #39197, #39611, #30135, #26462 ),
 .UNSPECIFIED., .F., .F. ) 
 B_SPLINE_CURVE_WITH_KNOTS ( ( 3, 2, 2, 3 ),
 ( 0.2350746268656717097, 0.2363184079601990950, 0.2375621890547264525, 0.2388059701492538378 ),
 .UNSPECIFIED. ) 
 CURVE ( )  GEOMETRIC_REPRESENTATION_ITEM ( )  RATIONAL_B_SPLINE_CURVE ( ( 0.9999999999999940048, 0.8660254037844447028, 1.000000000000000000, 0.8660254037844387076, 1.000000000000000000, 0.8660254037844267172, 1.000000000000011990 ) ) 
 REPRESENTATION_ITEM ( '' )  );
#23984=CARTESIAN_POINT ( 'NONE',  ( -10.81189881249999729, 6.242252689847871849, -132.9062500020483810 ) ) ;
#23985=CARTESIAN_POINT ( 'NONE',  ( -4.999999999999996447, 8.660254037844387298, -162.3750000040967905 ) ) ;
#23986=VERTEX_POINT ( 'NONE', #41680 ) ;
#23987=EDGE_LOOP ( 'NONE', ( #36870, #10481, #5817, #5194 ) ) ;
#23989=CARTESIAN_POINT ( 'NONE',  ( -4.999999999999996447, 8.660254037844387298, -107.9999999999999858 ) ) ;
#23990=CARTESIAN_POINT ( 'NONE',  ( 0.000000000000000000, 0.000000000000000000, -200.0000000000000000 ) ) ;
#23991=CARTESIAN_POINT ( 'NONE',  ( -10.81189881249999907, -6.242252689847864744, -166.9687500020484094 ) ) ;
#23994=CARTESIAN_POINT ( 'NONE',  ( 5.405949406249999534, 9.363379034771803333, -13.09375000204834905 ) ) ;
#23995=CARTESIAN_POINT ( 'NONE',  ( 7.070501591499376803E-16, 11.54700538379251284, -171.1250000000000000 ) ) ;
#23996=VECTOR ( 'NONE', #4189, 1000.000000000000114 ) ;
#23997=CARTESIAN_POINT ( 'NONE',  ( 5.405949406249999534, 9.363379034771803333, -146.5937500020483810 ) ) ;
#23998=VECTOR ( 'NONE', #9656, 1000.000000000000000 ) ;
#23999=CARTESIAN_POINT ( 'NONE',  ( -2.293366432827344421E-15, -12.48450537969573659, -135.2187500020483810 ) ) ;
#24000=CARTESIAN_POINT ( 'NONE',  ( -10.81189881249999729, 1.324075727343319199E-15, -105.7812500020483810 ) ) ;
#24004=CARTESIAN_POINT ( 'NONE',  ( -10.81189881249999729, 1.324075727343319199E-15, -11.09375000204834727 ) ) ;
#24010=CARTESIAN_POINT ( 'NONE',  ( -5.405949406249996869, 9.363379034771805109, -74.34375000204838102 ) ) ;
#24011=CARTESIAN_POINT ( 'NONE',  ( -10.81189881249999729, 1.324075727343319199E-15, -62.09375000204836681 ) ) ;
#24013=CARTESIAN_POINT ( 'NONE',  ( 7.644554776091147741E-16, 12.48450537969573659, -37.15625000204836681 ) ) ;
#24015=CARTESIAN_POINT ( 'NONE',  ( -9.999999999999998224, 1.224646799147353059E-15, -139.6250000040967905 ) ) ;
#24017=CARTESIAN_POINT ( 'NONE',  ( -9.999999999999998224, 1.224646799147353059E-15, -127.2499999999999716 ) ) ;
#24018=CARTESIAN_POINT ( 'NONE',  ( 5.405949406249992428, -9.363379034771808662, -133.7812500020483810 ) ) ;
#24019=CARTESIAN_POINT ( 'NONE',  ( 5.000000000000000000, 8.660254037844385522, -94.74999999999998579 ) ) ;
#24021=CARTESIAN_POINT ( 'NONE',  ( 10.81189881249999729, 0.000000000000000000, -16.53125000204835970 ) ) ;
#24022=VERTEX_POINT ( 'NONE', #35862 ) ;
#24023=( BOUNDED_CURVE ( )  B_SPLINE_CURVE ( 2, ( #15977, #35233, #35445, #6085, #35654, #5871, #42522 ),
 .UNSPECIFIED., .F., .F. ) 
 B_SPLINE_CURVE_WITH_KNOTS ( ( 3, 2, 2, 3 ),
 ( 0.007462686567164185901, 0.008706467661691551230, 0.009950248756218915691, 0.01119402985074628015 ),
 .UNSPECIFIED. ) 
 CURVE ( )  GEOMETRIC_REPRESENTATION_ITEM ( )  RATIONAL_B_SPLINE_CURVE ( ( 0.9999999999999993339, 0.8660254037844394848, 1.000000000000000000, 0.8660254037844387076, 1.000000000000000000, 0.8660254037844373753, 1.000000000000001332 ) ) 
 REPRESENTATION_ITEM ( '' )  );
#24027=CARTESIAN_POINT ( 'NONE',  ( -9.999999999999998224, 1.224646799147353059E-15, -36.12500000409676915 ) ) ;
#24028=EDGE_CURVE ( 'NONE', #24638, #32801, #12118, .T. ) ;
#24032=CARTESIAN_POINT ( 'NONE',  ( 9.999999999999479527, 5.773502691896553074, -76.87499999999997158 ) ) ;
#24033=CARTESIAN_POINT ( 'NONE',  ( -10.81189881249999729, 6.242252689847871849, -155.4062500020483810 ) ) ;
#24034=CARTESIAN_POINT ( 'NONE',  ( 10.81189881249999551, -6.242252689847874514, -137.9687500020483810 ) ) ;
#24037=VERTEX_POINT ( 'NONE', #25729 ) ;
#24040=ORIENTED_EDGE ( 'NONE', *, *, #28585, .F. ) ;
#24041=CARTESIAN_POINT ( 'NONE',  ( 5.405949406249992428, -9.363379034771808662, -108.0937500020483810 ) ) ;
#24043=CARTESIAN_POINT ( 'NONE',  ( -2.293366432827344421E-15, -12.48450537969573659, -192.2187500020484379 ) ) ;
#24044=CARTESIAN_POINT ( 'NONE',  ( -5.405949406249996869, 9.363379034771805109, -35.34375000204836681 ) ) ;
#24046=DIRECTION ( 'NONE',  ( 1.000000000000000000, 0.000000000000000000, 0.000000000000000000 ) ) ;
#24047=CARTESIAN_POINT ( 'NONE',  ( -10.81189881249999729, 1.324075727343319199E-15, -170.0937500020484094 ) ) ;
#24048=CARTESIAN_POINT ( 'NONE',  ( 10.81189881249999729, 0.000000000000000000, -161.8437500020484094 ) ) ;
#24052=CARTESIAN_POINT ( 'NONE',  ( -5.000000000000003553, -8.660254037844383745, -155.5000000000000000 ) ) ;
#24053=CARTESIAN_POINT ( 'NONE',  ( -4.999999999999996447, 8.660254037844387298, -66.37500000409676204 ) ) ;
#24055=CARTESIAN_POINT ( 'NONE',  ( -10.81189881249999729, 1.324075727343319199E-15, -86.09375000204836681 ) ) ;
#24056=CARTESIAN_POINT ( 'NONE',  ( 10.00000000000051159, -5.773502691895965988, -72.62499999999995737 ) ) ;
#24057=CARTESIAN_POINT ( 'NONE',  ( 5.405949406249992428, -9.363379034771808662, -63.28125000204837391 ) ) ;
#24060=CARTESIAN_POINT ( 'NONE',  ( -10.81189881249999729, 1.324075727343319199E-15, -125.2812500020483668 ) ) ;
#24061=VECTOR ( 'NONE', #2368, 1000.000000000000000 ) ;
#24062=CARTESIAN_POINT ( 'NONE',  ( 10.81189881249999729, 6.242252689847867408, -152.9062500020483810 ) ) ;
#24065=CARTESIAN_POINT ( 'NONE',  ( -9.999999999999998224, 5.773502691896259087, -130.7500000040967905 ) ) ;
#24072=CARTESIAN_POINT ( 'NONE',  ( 7.644554776091147741E-16, 12.48450537969573659, -190.1562500020484094 ) ) ;
#24073=ORIENTED_EDGE ( 'NONE', *, *, #18562, .T. ) ;
#24074=CARTESIAN_POINT ( 'NONE',  ( -4.999999999999996447, 8.660254037844387298, -46.49999999999998579 ) ) ;
#24076=CARTESIAN_POINT ( 'NONE',  ( -9.999999999999998224, 5.773502691896259087, -60.25000000409677625 ) ) ;
#24077=EDGE_CURVE ( 'NONE', #28118, #258, #11011, .T. ) ;
#24078=CARTESIAN_POINT ( 'NONE',  ( -4.999999999999996447, 8.660254037844387298, -178.8750000040967905 ) ) ;
#24081=CARTESIAN_POINT ( 'NONE',  ( -5.405949406250003975, -9.363379034771801557, -60.53125000204836681 ) ) ;
#24083=VECTOR ( 'NONE', #32405, 1000.000000000000000 ) ;
#24085=CARTESIAN_POINT ( 'NONE',  ( -9.999999999999998224, 1.224646799147353059E-15, -157.6250000040967905 ) ) ;
#24086=CARTESIAN_POINT ( 'NONE',  ( 5.405949406249992428, -9.363379034771808662, -180.2812500020484094 ) ) ;
#24088=CARTESIAN_POINT ( 'NONE',  ( -9.999999999999998224, 1.224646799147353059E-15, -137.7499999999999716 ) ) ;
#24091=CARTESIAN_POINT ( 'NONE',  ( -9.999999999999998224, 1.224646799147353059E-15, -200.0000000000000000 ) ) ;
#24092=CARTESIAN_POINT ( 'NONE',  ( 10.81189881249999907, 6.242252689847868297, -83.90625000204836681 ) ) ;
#24095=EDGE_CURVE ( 'NONE', #36957, #17005, #41644, .T. ) ;
#24096=LINE ( 'NONE', #5089, #4098 ) ;
#24097=ORIENTED_EDGE ( 'NONE', *, *, #30528, .F. ) ;
#24098=( BOUNDED_CURVE ( )  B_SPLINE_CURVE ( 2, ( #26016, #35936, #29250, #29679, #7009, #6377, #3137 ),
 .UNSPECIFIED., .F., .F. ) 
 B_SPLINE_CURVE_WITH_KNOTS ( ( 3, 2, 2, 3 ),
 ( 0.8880597014925376564, 0.8893034825870650417, 0.8905472636815924270, 0.8917910447761197013 ),
 .UNSPECIFIED. ) 
 CURVE ( )  GEOMETRIC_REPRESENTATION_ITEM ( )  RATIONAL_B_SPLINE_CURVE ( ( 0.9999999999999641398, 0.8660254037844745678, 1.000000000000000000, 0.8660254037844387076, 1.000000000000000000, 0.8660254037844028474, 1.000000000000035971 ) ) 
 REPRESENTATION_ITEM ( '' )  );
#24100=CARTESIAN_POINT ( 'NONE',  ( 7.644554776091147741E-16, 12.48450537969573659, -39.96875000204835970 ) ) ;
#24101=CARTESIAN_POINT ( 'NONE',  ( 5.405949406249992428, -9.363379034771808662, -27.09375000204835970 ) ) ;
#24102=CARTESIAN_POINT ( 'NONE',  ( 5.405949406249992428, -9.363379034771808662, -16.78125000204835970 ) ) ;
#24104=CARTESIAN_POINT ( 'NONE',  ( 5.405949406249992428, -9.363379034771808662, -63.09375000204836681 ) ) ;
#24105=CARTESIAN_POINT ( 'NONE',  ( 4.999999999999992006, -8.660254037844389075, -131.2499999999999716 ) ) ;
#24108=CARTESIAN_POINT ( 'NONE',  ( -2.293366432827344421E-15, -12.48450537969573659, -184.7187500020484094 ) ) ;
#24110=CARTESIAN_POINT ( 'NONE',  ( -2.293366432827344421E-15, -12.48450537969573659, -3.218750002048363257 ) ) ;
#24111=CARTESIAN_POINT ( 'NONE',  ( 9.999999999999998224, 0.000000000000000000, -192.5000000000000000 ) ) ;
#24112=VECTOR ( 'NONE', #13310, 1000.000000000000000 ) ;
#24114=CARTESIAN_POINT ( 'NONE',  ( 10.00000000000000000, 5.773502691896255534, 0.7499999959032597197 ) ) ;
#24116=CARTESIAN_POINT ( 'NONE',  ( 5.405949406249999534, 9.363379034771803333, -112.0937500020483810 ) ) ;
#24117=CARTESIAN_POINT ( 'NONE',  ( 7.070501591499376803E-16, 11.54700538379251284, -15.12499999999997691 ) ) ;
#24118=CARTESIAN_POINT ( 'NONE',  ( -5.405949406249996869, 9.363379034771805109, -89.53125000204838102 ) ) ;
#24119=CARTESIAN_POINT ( 'NONE',  ( -5.405949406249996869, 9.363379034771805109, -102.8437500020483810 ) ) ;
#24122=CARTESIAN_POINT ( 'NONE',  ( -4.999999999999996447, 8.660254037844387298, -151.8750000040967905 ) ) ;
#24126=CARTESIAN_POINT ( 'NONE',  ( 9.999999999999998224, 0.000000000000000000, -153.8750000040967905 ) ) ;
#24128=CARTESIAN_POINT ( 'NONE',  ( -10.00000000000154188, 5.773502691895366468, -10.37499999999991296 ) ) ;
#24129=CARTESIAN_POINT ( 'NONE',  ( -9.999999999999998224, 1.224646799147353059E-15, -70.24999999999998579 ) ) ;
#24131=CARTESIAN_POINT ( 'NONE',  ( -4.999999999999996447, 8.660254037844387298, -81.37500000409677625 ) ) ;
#24132=ADVANCED_FACE ( 'NONE', ( #26567 ), #3266, .T. ) ;
#24133=CARTESIAN_POINT ( 'NONE',  ( -9.999999999999479527, -5.773502691896549521, -96.00000000409677625 ) ) ;
#24135=CARTESIAN_POINT ( 'NONE',  ( 7.644554776091147741E-16, 12.48450537969573659, -86.65625000204838102 ) ) ;
#24138=CARTESIAN_POINT ( 'NONE',  ( 9.999999999999479527, 5.773502691896553074, -113.2500000040967620 ) ) ;
#24140=EDGE_LOOP ( 'NONE', ( #22645, #13968, #40399 ) ) ;
#24141=CARTESIAN_POINT ( 'NONE',  ( 9.999999999999998224, 0.000000000000000000, -4.999999999999976907 ) ) ;
#24142=CIRCLE ( 'NONE', #10333, 9.999999999999998224 ) ;
#24145=CARTESIAN_POINT ( 'NONE',  ( 7.644554776091147741E-16, 12.48450537969573659, -12.96875000204836148 ) ) ;
#24146=CARTESIAN_POINT ( 'NONE',  ( -2.121150477449813534E-15, -11.54700538379251284, -94.25000000409677625 ) ) ;
#24148=CARTESIAN_POINT ( 'NONE',  ( -10.81189881249999729, 1.324075727343319199E-15, -131.2812500020483810 ) ) ;
#24149=( BOUNDED_CURVE ( )  B_SPLINE_CURVE ( 2, ( #10243, #39811, #36372, #23006, #29908, #23215, #29694 ),
 .UNSPECIFIED., .F., .F. ) 
 B_SPLINE_CURVE_WITH_KNOTS ( ( 3, 2, 2, 3 ),
 ( 0.7723880597014927130, 0.7736318407960200982, 0.7748756218905473725, 0.7761194029850747578 ),
 .UNSPECIFIED. ) 
 CURVE ( )  GEOMETRIC_REPRESENTATION_ITEM ( )  RATIONAL_B_SPLINE_CURVE ( ( 0.9999999999999761302, 0.8660254037844625774, 1.000000000000000000, 0.8660254037844387076, 1.000000000000000000, 0.8660254037844267172, 1.000000000000011990 ) ) 
 REPRESENTATION_ITEM ( '' )  );
#24150=CARTESIAN_POINT ( 'NONE',  ( -2.121150477449813534E-15, -11.54700538379251284, -180.8750000000000000 ) ) ;
#24151=CARTESIAN_POINT ( 'NONE',  ( -10.81189881249999729, 1.324075727343319199E-15, -110.2812500020483810 ) ) ;
#24152=EDGE_LOOP ( 'NONE', ( #15721, #14065, #18292, #1006 ) ) ;
#24153=CARTESIAN_POINT ( 'NONE',  ( -9.999999999999998224, 1.224646799147353059E-15, -154.6250000040967905 ) ) ;
#24154=ORIENTED_EDGE ( 'NONE', *, *, #34175, .F. ) ;
#24155=ORIENTED_EDGE ( 'NONE', *, *, #20273, .F. ) ;
#24156=EDGE_CURVE ( 'NONE', #32999, #8390, #16824, .T. ) ;
#24157=CARTESIAN_POINT ( 'NONE',  ( 5.405949406249999534, 9.363379034771803333, -37.28125000204837391 ) ) ;
#24159=CARTESIAN_POINT ( 'NONE',  ( -5.405949406250003975, -9.363379034771801557, -87.34375000204836681 ) ) ;
#24160=CARTESIAN_POINT ( 'NONE',  ( 9.999999999999998224, 0.000000000000000000, -200.0000000000000000 ) ) ;
#24161=FACE_OUTER_BOUND ( 'NONE', #13891, .T. ) ;
#24163=CARTESIAN_POINT ( 'NONE',  ( 5.000000000000000000, 8.660254037844385522, -58.74999999999997158 ) ) ;
#24164=CARTESIAN_POINT ( 'NONE',  ( 10.81189881249999729, 6.242252689847867408, -122.7187500020483952 ) ) ;
#24166=CARTESIAN_POINT ( 'NONE',  ( 10.81189881249999551, -6.242252689847874514, -4.656250002048354375 ) ) ;
#24167=CARTESIAN_POINT ( 'NONE',  ( 4.999999999999992006, -8.660254037844389075, -44.24999999999998579 ) ) ;
#24169=CARTESIAN_POINT ( 'NONE',  ( 9.999999999999998224, 0.000000000000000000, -176.3750000040967905 ) ) ;
#24171=CARTESIAN_POINT ( 'NONE',  ( 10.81189881249999729, 0.000000000000000000, -178.5312500020483810 ) ) ;
#24175=CARTESIAN_POINT ( 'NONE',  ( 10.81189881249999551, -6.242252689847874514, -52.46875000204836681 ) ) ;
#24176=CARTESIAN_POINT ( 'NONE',  ( 7.644554776091147741E-16, 12.48450537969573659, -42.96875000204835970 ) ) ;
#24178=CARTESIAN_POINT ( 'NONE',  ( -10.81189881249999729, 1.324075727343319199E-15, -6.781250002048377468 ) ) ;
#24180=CARTESIAN_POINT ( 'NONE',  ( 7.070501591499376803E-16, 11.54700538379251284, -145.6250000000000000 ) ) ;
#24182=CARTESIAN_POINT ( 'NONE',  ( 4.999999999999992006, -8.660254037844389075, -101.2499999999999858 ) ) ;
#24184=CARTESIAN_POINT ( 'NONE',  ( 4.999999999999992006, -8.660254037844389075, -115.1250000040967905 ) ) ;
#24185=CARTESIAN_POINT ( 'NONE',  ( -9.999999999999998224, 1.224646799147353059E-15, -169.2500000000000000 ) ) ;
#24188=CARTESIAN_POINT ( 'NONE',  ( -5.405949406250003975, -9.363379034771801557, -110.0312500020483810 ) ) ;
#24190=DIRECTION ( 'NONE',  ( -0.000000000000000000, -0.000000000000000000, 1.000000000000000000 ) ) ;
#24193=CARTESIAN_POINT ( 'NONE',  ( -10.81189881249999729, 6.242252689847871849, -164.4062500020484094 ) ) ;
#24195=VERTEX_POINT ( 'NONE', #20500 ) ;
#24196=CARTESIAN_POINT ( 'NONE',  ( 4.999999999999992006, -8.660254037844389075, -26.24999999999996803 ) ) ;
#24197=CARTESIAN_POINT ( 'NONE',  ( -5.405949406250003975, -9.363379034771801557, -39.53125000204838102 ) ) ;
#24198=CARTESIAN_POINT ( 'NONE',  ( -4.999999999999996447, 8.660254037844387298, -163.5000000000000000 ) ) ;
#24199=DIRECTION ( 'NONE',  ( -0.000000000000000000, -0.000000000000000000, 1.000000000000000000 ) ) ;
#24201=ADVANCED_FACE ( 'NONE', ( #469 ), #13584, .T. ) ;
#24202=CARTESIAN_POINT ( 'NONE',  ( -10.81189881249999729, 1.324075727343319199E-15, -135.7812500020483810 ) ) ;
#24203=CARTESIAN_POINT ( 'NONE',  ( 7.232763097364098392, 7.658562690767763748, -5.257032284683799044E-15 ) ) ;
#24204=AXIS2_PLACEMENT_3D ( 'NONE', #23227, #32731, #16294 ) ;
#24205=DIRECTION ( 'NONE',  ( -0.000000000000000000, -0.000000000000000000, 1.000000000000000000 ) ) ;
#24206=EDGE_LOOP ( 'NONE', ( #17960, #98, #20782, #11175 ) ) ;
#24207=EDGE_LOOP ( 'NONE', ( #17726, #32689, #5292, #5354 ) ) ;
#24210=CARTESIAN_POINT ( 'NONE',  ( 9.999999999999998224, 0.000000000000000000, -146.3750000040967905 ) ) ;
#24211=CARTESIAN_POINT ( 'NONE',  ( 10.81189881249999907, 6.242252689847868297, -169.2187500020483810 ) ) ;
#24212=CARTESIAN_POINT ( 'NONE',  ( -5.405949406249996869, 9.363379034771805109, -12.84375000204834905 ) ) ;
#24213=CARTESIAN_POINT ( 'NONE',  ( 0.000000000000000000, 0.000000000000000000, -200.0000000000000000 ) ) ;
#24214=CARTESIAN_POINT ( 'NONE',  ( 7.644554776091147741E-16, 12.48450537969573659, -147.9687500020484094 ) ) ;
#24215=CARTESIAN_POINT ( 'NONE',  ( 10.81189881249999729, 0.000000000000000000, -139.3437500020484094 ) ) ;
#24216=CARTESIAN_POINT ( 'NONE',  ( 5.405949406249999534, 9.363379034771803333, -104.7812500020483810 ) ) ;
#24220=CARTESIAN_POINT ( 'NONE',  ( 5.405949406249992428, -9.363379034771808662, -12.09375000204834727 ) ) ;
#24222=AXIS2_PLACEMENT_3D ( 'NONE', #25358, #1413, #8317 ) ;
#24223=CARTESIAN_POINT ( 'NONE',  ( 5.405949406249999534, 9.363379034771803333, -199.2812500020484094 ) ) ;
#24227=CARTESIAN_POINT ( 'NONE',  ( 5.405949406249999534, 9.363379034771803333, -79.09375000204838102 ) ) ;
#24228=CARTESIAN_POINT ( 'NONE',  ( 10.81189881249999907, 6.242252689847868297, -67.21875000204838102 ) ) ;
#24230=CARTESIAN_POINT ( 'NONE',  ( 7.644554776091147741E-16, 12.48450537969573659, -35.65625000204835260 ) ) ;
#24234=CARTESIAN_POINT ( 'NONE',  ( -9.999999999999998224, 1.224646799147353059E-15, -122.7500000000000000 ) ) ;
#24235=CARTESIAN_POINT ( 'NONE',  ( -5.405949406250003975, -9.363379034771801557, -134.0312500020484094 ) ) ;
#24236=DIRECTION ( 'NONE',  ( -0.000000000000000000, -0.000000000000000000, 1.000000000000000000 ) ) ;
#24238=CARTESIAN_POINT ( 'NONE',  ( 10.81189881249999729, 6.242252689847867408, -14.90625000204837036 ) ) ;
#24239=ORIENTED_EDGE ( 'NONE', *, *, #35719, .F. ) ;
#24242=CARTESIAN_POINT ( 'NONE',  ( -9.999999999998969713, -5.773502691896847949, -57.00000000409674783 ) ) ;
#24243=AXIS2_PLACEMENT_3D ( 'NONE', #37359, #7369, #34134 ) ;
#24244=CARTESIAN_POINT ( 'NONE',  ( -4.999999999999996447, 8.660254037844387298, -36.37500000409676915 ) ) ;
#24245=DIRECTION ( 'NONE',  ( -0.000000000000000000, -0.000000000000000000, 1.000000000000000000 ) ) ;
#24247=EDGE_CURVE ( 'NONE', #3072, #9067, #24274, .T. ) ;
#24249=CARTESIAN_POINT ( 'NONE',  ( -10.81189881249999729, 6.242252689847871849, -152.4062500020483810 ) ) ;
#24250=CARTESIAN_POINT ( 'NONE',  ( -10.81189881249999729, 1.324075727343319199E-15, -131.0937500020483810 ) ) ;
#24251=CARTESIAN_POINT ( 'NONE',  ( 7.070501591499376803E-16, 11.54700538379251284, -144.1250000000000000 ) ) ;
#24252=ORIENTED_EDGE ( 'NONE', *, *, #31320, .F. ) ;
#24253=CARTESIAN_POINT ( 'NONE',  ( -4.999999999999996447, 8.660254037844387298, -22.49999999999996447 ) ) ;
#24255=AXIS2_PLACEMENT_3D ( 'NONE', #7114, #30432, #6898 ) ;
#24258=CARTESIAN_POINT ( 'NONE',  ( -5.405949406250003975, -9.363379034771801557, -112.8437500020483810 ) ) ;
#24259=EDGE_LOOP ( 'NONE', ( #13290, #36606, #32310, #27691 ) ) ;
#24260=EDGE_CURVE ( 'NONE', #37116, #30868, #5766, .T. ) ;
#24261=( BOUNDED_CURVE ( )  B_SPLINE_CURVE ( 2, ( #37503, #5135, #11804, #24146, #7946, #21096, #31265 ),
 .UNSPECIFIED., .F., .F. ) 
 B_SPLINE_CURVE_WITH_KNOTS ( ( 3, 2, 2, 3 ),
 ( 0.5186567164179105571, 0.5199004975124379424, 0.5211442786069653277, 0.5223880597014926019 ),
 .UNSPECIFIED. ) 
 CURVE ( )  GEOMETRIC_REPRESENTATION_ITEM ( )  RATIONAL_B_SPLINE_CURVE ( ( 0.9999999999999880096, 0.8660254037844506980, 1.000000000000000000, 0.8660254037844387076, 1.000000000000000000, 0.8660254037844267172, 1.000000000000011990 ) ) 
 REPRESENTATION_ITEM ( '' )  );
#24262=CARTESIAN_POINT ( 'NONE',  ( -2.121150477449813534E-15, -11.54700538379251284, -41.75000000409674783 ) ) ;
#24263=CARTESIAN_POINT ( 'NONE',  ( -2.293366432827344421E-15, -12.48450537969573659, -186.2187500020484094 ) ) ;
#24264=AXIS2_PLACEMENT_3D ( 'NONE', #28603, #8531, #31633 ) ;
#24265=CARTESIAN_POINT ( 'NONE',  ( -10.81189881249999729, 6.242252689847871849, -41.21875000204834549 ) ) ;
#24267=CARTESIAN_POINT ( 'NONE',  ( 9.999999999999998224, 0.000000000000000000, -195.8750000040967905 ) ) ;
#24268=CARTESIAN_POINT ( 'NONE',  ( -10.81189881249999729, 1.324075727343319199E-15, -171.5937500020484094 ) ) ;
#24269=CARTESIAN_POINT ( 'NONE',  ( 10.81189881249999551, -6.242252689847874514, -161.9687500020484094 ) ) ;
#24270=CARTESIAN_POINT ( 'NONE',  ( 10.00000000000051159, -5.773502691895965988, -122.5000000040967763 ) ) ;
#24273=CARTESIAN_POINT ( 'NONE',  ( 9.999999999999998224, 0.000000000000000000, -87.49999999999998579 ) ) ;
#24274=( BOUNDED_CURVE ( )  B_SPLINE_CURVE ( 2, ( #33687, #4113, #41783, #5549, #28652, #12009, #18701 ),
 .UNSPECIFIED., .F., .F. ) 
 B_SPLINE_CURVE_WITH_KNOTS ( ( 3, 2, 2, 3 ),
 ( 0.9291044776119405935, 0.9303482587064679787, 0.9315920398009952530, 0.9328358208955226383 ),
 .UNSPECIFIED. ) 
 CURVE ( )  GEOMETRIC_REPRESENTATION_ITEM ( )  RATIONAL_B_SPLINE_CURVE ( ( 0.9999999999999641398, 0.8660254037844745678, 1.000000000000000000, 0.8660254037844387076, 1.000000000000000000, 0.8660254037844148378, 1.000000000000023981 ) ) 
 REPRESENTATION_ITEM ( '' )  );
#24277=CARTESIAN_POINT ( 'NONE',  ( 5.405949406249992428, -9.363379034771808662, -88.59375000204838102 ) ) ;
#24278=CARTESIAN_POINT ( 'NONE',  ( -5.000000000000003553, -8.660254037844383745, -82.37500000409676204 ) ) ;
#24279=CARTESIAN_POINT ( 'NONE',  ( -5.405949406250003975, -9.363379034771801557, -57.53125000204836681 ) ) ;
#24280=CYLINDRICAL_SURFACE ( 'NONE', #33003, 9.999999999999998224 ) ;
#24282=CARTESIAN_POINT ( 'NONE',  ( 5.405949406249999534, 9.363379034771803333, -110.7812500020483810 ) ) ;
#24283=CARTESIAN_POINT ( 'NONE',  ( -10.81189881249999729, 6.242252689847871849, -153.9062500020483810 ) ) ;
#24286=CARTESIAN_POINT ( 'NONE',  ( 5.000000000000000000, 8.660254037844385522, -132.6250000040967620 ) ) ;
#24288=VECTOR ( 'NONE', #7389, 1000.000000000000000 ) ;
#24290=( BOUNDED_CURVE ( )  B_SPLINE_CURVE ( 2, ( #33739, #17091, #23806, #20550, #7613, #20338, #3525 ),
 .UNSPECIFIED., .F., .F. ) 
 B_SPLINE_CURVE_WITH_KNOTS ( ( 3, 2, 2, 3 ),
 ( 0.07089552238805976736, 0.07213930348258713876, 0.07338308457711449628, 0.07462686567164185381 ),
 .UNSPECIFIED. ) 
 CURVE ( )  GEOMETRIC_REPRESENTATION_ITEM ( )  RATIONAL_B_SPLINE_CURVE ( ( 0.9999999999999925615, 0.8660254037844461461, 1.000000000000000000, 0.8660254037844387076, 1.000000000000000000, 0.8660254037844312691, 1.000000000000007550 ) ) 
 REPRESENTATION_ITEM ( '' )  );
#24293=CARTESIAN_POINT ( 'NONE',  ( -5.405949406249996869, 9.363379034771805109, -188.5312500020484094 ) ) ;
#24294=ORIENTED_EDGE ( 'NONE', *, *, #40189, .F. ) ;
#24295=CARTESIAN_POINT ( 'NONE',  ( -10.00000000000000000, -5.773502691896251982, -50.62499999999997868 ) ) ;
#24297=CARTESIAN_POINT ( 'NONE',  ( -5.000000000000003553, -8.660254037844383745, -58.37500000409676204 ) ) ;
#24298=LINE ( 'NONE', #5072, #42365 ) ;
#24301=CARTESIAN_POINT ( 'NONE',  ( 10.81189881249999729, 0.000000000000000000, -48.03125000204838813 ) ) ;
#24304=CARTESIAN_POINT ( 'NONE',  ( -9.999999999999227285, -5.773502691896698735, -135.0000000040967620 ) ) ;
#24305=CARTESIAN_POINT ( 'NONE',  ( 10.81189881249999729, 0.000000000000000000, -180.0312500020483810 ) ) ;
#24313=CARTESIAN_POINT ( 'NONE',  ( 10.81189881249999551, -6.242252689847874514, -82.65625000204836681 ) ) ;
#24314=ORIENTED_EDGE ( 'NONE', *, *, #1014, .F. ) ;
#24317=VERTEX_POINT ( 'NONE', #18490 ) ;
#24318=CARTESIAN_POINT ( 'NONE',  ( -10.81189881249999729, 1.324075727343319199E-15, -39.59375000204837391 ) ) ;
#24319=CARTESIAN_POINT ( 'NONE',  ( 7.644554776091147741E-16, 12.48450537969573659, -27.96875000204838457 ) ) ;
#24320=CARTESIAN_POINT ( 'NONE',  ( -2.293366432827344421E-15, -12.48450537969573659, -12.40625000204835970 ) ) ;
#24321=CARTESIAN_POINT ( 'NONE',  ( 5.405949406249992428, -9.363379034771808662, -61.59375000204836681 ) ) ;
#24325=CARTESIAN_POINT ( 'NONE',  ( -5.405949406249996869, 9.363379034771805109, -186.8437500020483810 ) ) ;
#24333=DIRECTION ( 'NONE',  ( -0.000000000000000000, -0.000000000000000000, 1.000000000000000000 ) ) ;
#24334=CARTESIAN_POINT ( 'NONE',  ( -5.405949406250003975, -9.363379034771801557, -112.8437500020483810 ) ) ;
#24336=CARTESIAN_POINT ( 'NONE',  ( 7.644554776091147741E-16, 12.48450537969573659, -83.65625000204838102 ) ) ;
#24337=CARTESIAN_POINT ( 'NONE',  ( 10.81189881249999551, -6.242252689847874514, -97.46875000204838102 ) ) ;
#24340=CARTESIAN_POINT ( 'NONE',  ( 10.00000000000000000, 5.773502691896255534, -150.7500000040967905 ) ) ;
#24344=CYLINDRICAL_SURFACE ( 'NONE', #4770, 9.999999999999998224 ) ;
#24345=CARTESIAN_POINT ( 'NONE',  ( 0.000000000000000000, 0.000000000000000000, -200.0000000000000000 ) ) ;
#24348=CARTESIAN_POINT ( 'NONE',  ( 7.070501591499377789E-16, 11.54700538379251284, -70.62499999999998579 ) ) ;
#24350=CARTESIAN_POINT ( 'NONE',  ( 5.000000000000000000, 8.660254037844385522, -83.12500000409676204 ) ) ;
#24351=FACE_OUTER_BOUND ( 'NONE', #21951, .T. ) ;
#24353=CARTESIAN_POINT ( 'NONE',  ( 10.81189881249999551, -6.242252689847874514, -75.15625000204838102 ) ) ;
#24358=CARTESIAN_POINT ( 'NONE',  ( 10.81189881249999551, -6.242252689847874514, -198.1562500020484379 ) ) ;
#24360=CARTESIAN_POINT ( 'NONE',  ( -10.81189881249999729, -6.242252689847864744, -15.46875000204835793 ) ) ;
#24361=CARTESIAN_POINT ( 'NONE',  ( 9.999999999999998224, 0.000000000000000000, -117.8750000040967905 ) ) ;
#24362=( BOUNDED_CURVE ( )  B_SPLINE_CURVE ( 2, ( #12196, #24975, #34892, #41336, #41762, #5958, #5316 ),
 .UNSPECIFIED., .F., .F. ) 
 B_SPLINE_CURVE_WITH_KNOTS ( ( 3, 2, 2, 3 ),
 ( 0.4813432835820896649, 0.4825870646766170502, 0.4838308457711443800, 0.4850746268656717652 ),
 .UNSPECIFIED. ) 
 CURVE ( )  GEOMETRIC_REPRESENTATION_ITEM ( )  RATIONAL_B_SPLINE_CURVE ( ( 0.9999999999999880096, 0.8660254037844506980, 1.000000000000000000, 0.8660254037844387076, 1.000000000000000000, 0.8660254037844267172, 1.000000000000011990 ) ) 
 REPRESENTATION_ITEM ( '' )  );
#24364=CARTESIAN_POINT ( 'NONE',  ( 5.405949406249999534, 9.363379034771803333, -127.2812500020483810 ) ) ;
#24365=CARTESIAN_POINT ( 'NONE',  ( -9.999999999999998224, 5.773502691896259087, -179.8750000000000000 ) ) ;
#24366=DIRECTION ( 'NONE',  ( 1.000000000000000000, 0.000000000000000000, 0.000000000000000000 ) ) ;
#24367=CARTESIAN_POINT ( 'NONE',  ( -5.405949406250003975, -9.363379034771801557, -110.0312500020483810 ) ) ;
#24370=ORIENTED_EDGE ( 'NONE', *, *, #19569, .F. ) ;
#24371=ORIENTED_EDGE ( 'NONE', *, *, #480, .T. ) ;
#24372=CARTESIAN_POINT ( 'NONE',  ( -5.405949406249996869, 9.363379034771805109, -38.53125000204838102 ) ) ;
#24374=CARTESIAN_POINT ( 'NONE',  ( -10.81189881249999907, -6.242252689847864744, -85.96875000204836681 ) ) ;
#24375=CARTESIAN_POINT ( 'NONE',  ( 9.999999999999994671, -5.773502691896262640, -167.1250000000000000 ) ) ;
#24376=EDGE_CURVE ( 'NONE', #20021, #34021, #2112, .T. ) ;
#24379=ADVANCED_FACE ( 'NONE', ( #17674 ), #38555, .T. ) ;
#24382=LINE ( 'NONE', #1064, #5943 ) ;
#24383=CARTESIAN_POINT ( 'NONE',  ( 10.81189881249999729, 0.000000000000000000, -125.8437500020483952 ) ) ;
#24386=CARTESIAN_POINT ( 'NONE',  ( -10.81189881249999729, 6.242252689847871849, -3.906250002048350822 ) ) ;
#24389=CARTESIAN_POINT ( 'NONE',  ( 7.070501591499377789E-16, 11.54700538379251284, -176.0000000040968189 ) ) ;
#24391=CARTESIAN_POINT ( 'NONE',  ( 7.644554776091147741E-16, 12.48450537969573659, -175.1562500020484094 ) ) ;
#24395=CARTESIAN_POINT ( 'NONE',  ( 10.81189881249999729, 0.000000000000000000, -49.34375000204838102 ) ) ;
#24397=CARTESIAN_POINT ( 'NONE',  ( 10.81189881249999907, 6.242252689847868297, -13.40625000204836326 ) ) ;
#24399=CARTESIAN_POINT ( 'NONE',  ( -2.121150477449813534E-15, -11.54700538379251284, -158.7500000040968189 ) ) ;
#24401=CARTESIAN_POINT ( 'NONE',  ( 10.00000000000000000, 5.773502691896255534, -100.8750000000000000 ) ) ;
#24403=CARTESIAN_POINT ( 'NONE',  ( -9.999999999999998224, 1.224646799147353059E-15, -108.1250000040967763 ) ) ;
#24404=CARTESIAN_POINT ( 'NONE',  ( -9.999999999998456346, -5.773502691897145489, -49.50000000409673362 ) ) ;
#24407=CARTESIAN_POINT ( 'NONE',  ( 10.81189881249999729, 0.000000000000000000, -99.03125000204839523 ) ) ;
#24408=ORIENTED_EDGE ( 'NONE', *, *, #14304, .F. ) ;
#24411=CARTESIAN_POINT ( 'NONE',  ( 9.999999999999998224, 0.000000000000000000, -141.8750000040967905 ) ) ;
#24412=CARTESIAN_POINT ( 'NONE',  ( 10.81189881249999907, 6.242252689847868297, -161.9062500020484094 ) ) ;
#24414=ORIENTED_EDGE ( 'NONE', *, *, #37545, .T. ) ;
#24415=EDGE_CURVE ( 'NONE', #13534, #20251, #30662, .T. ) ;
#24416=CARTESIAN_POINT ( 'NONE',  ( -2.121150477449813534E-15, -11.54700538379251284, -27.87499999999999289 ) ) ;
#24417=CARTESIAN_POINT ( 'NONE',  ( -10.81189881249999729, 1.324075727343319199E-15, -33.78125000204837391 ) ) ;
#24418=CARTESIAN_POINT ( 'NONE',  ( -2.121150477449813534E-15, -11.54700538379251284, -158.3750000000000000 ) ) ;
#24422=CARTESIAN_POINT ( 'NONE',  ( 10.81189881249999907, 6.242252689847868297, -130.4062500020483810 ) ) ;
#24423=DIRECTION ( 'NONE',  ( 1.000000000000000000, 0.000000000000000000, 0.000000000000000000 ) ) ;
#24424=CARTESIAN_POINT ( 'NONE',  ( 10.00000000000000000, 5.773502691896255534, -167.2500000040967905 ) ) ;
#24425=ORIENTED_EDGE ( 'NONE', *, *, #10185, .T. ) ;
#24427=ORIENTED_EDGE ( 'NONE', *, *, #486, .T. ) ;
#24428=CARTESIAN_POINT ( 'NONE',  ( 4.999999999999992006, -8.660254037844389075, -120.7500000000000000 ) ) ;
#24429=CARTESIAN_POINT ( 'NONE',  ( 4.999999999999992006, -8.660254037844389075, -146.6250000040967905 ) ) ;
#24430=CARTESIAN_POINT ( 'NONE',  ( -10.81189881249999729, 6.242252689847871849, -165.7187500020483810 ) ) ;
#24432=CARTESIAN_POINT ( 'NONE',  ( -5.405949406250003975, -9.363379034771801557, -18.34375000204835260 ) ) ;
#24433=CARTESIAN_POINT ( 'NONE',  ( 0.000000000000000000, 0.000000000000000000, -200.0000000000000000 ) ) ;
#24434=CARTESIAN_POINT ( 'NONE',  ( 10.81189881249999729, 6.242252689847867408, -145.2187500020484094 ) ) ;
#24435=CARTESIAN_POINT ( 'NONE',  ( -10.81189881249999907, -6.242252689847864744, -138.4687500020484094 ) ) ;
#24436=CARTESIAN_POINT ( 'NONE',  ( 5.405949406249992428, -9.363379034771808662, -109.7812500020483810 ) ) ;
#24440=CARTESIAN_POINT ( 'NONE',  ( -10.81189881249999907, -6.242252689847864744, -1.968750002048357262 ) ) ;
#24444=EDGE_CURVE ( 'NONE', #31913, #29936, #1305, .T. ) ;
#24445=CARTESIAN_POINT ( 'NONE',  ( 5.405949406249992428, -9.363379034771808662, -73.59375000204838102 ) ) ;
#24446=CARTESIAN_POINT ( 'NONE',  ( 10.81189881249999551, -6.242252689847874514, -65.96875000204836681 ) ) ;
#24448=CARTESIAN_POINT ( 'NONE',  ( -10.81189881249999907, -6.242252689847864744, -36.65625000204835970 ) ) ;
#24451=CARTESIAN_POINT ( 'NONE',  ( 4.999999999999992006, -8.660254037844389075, -117.7500000000000000 ) ) ;
#24452=CARTESIAN_POINT ( 'NONE',  ( 10.81189881249999551, -6.242252689847874514, -133.6562500020483810 ) ) ;
#24455=CARTESIAN_POINT ( 'NONE',  ( -5.405949406250003975, -9.363379034771801557, -18.53125000204835970 ) ) ;
#24456=VERTEX_POINT ( 'NONE', #28223 ) ;
#24460=CARTESIAN_POINT ( 'NONE',  ( -2.121150477449813534E-15, -11.54700538379251284, -37.25000000409676204 ) ) ;
#24464=CARTESIAN_POINT ( 'NONE',  ( 10.81189881249999907, 6.242252689847868297, -152.9062500020483810 ) ) ;
#24465=CARTESIAN_POINT ( 'NONE',  ( -10.81189881249999907, -6.242252689847864744, -127.9687500020483810 ) ) ;
#24466=CARTESIAN_POINT ( 'NONE',  ( 9.999999999999998224, 0.000000000000000000, -144.5000000000000000 ) ) ;
#24468=CYLINDRICAL_SURFACE ( 'NONE', #13445, 9.999999999999998224 ) ;
#24472=VERTEX_POINT ( 'NONE', #33903 ) ;
#24473=CARTESIAN_POINT ( 'NONE',  ( -5.405949406249996869, 9.363379034771805109, -189.8437500020483810 ) ) ;
#24474=CARTESIAN_POINT ( 'NONE',  ( 10.81189881249999551, -6.242252689847874514, -37.46875000204836681 ) ) ;
#24475=CARTESIAN_POINT ( 'NONE',  ( -3.753323245683507281, -9.574262767213205905, 1.142019215729699996E-14 ) ) ;
#24477=CARTESIAN_POINT ( 'NONE',  ( 10.81189881249999729, 6.242252689847867408, -170.7187500020483810 ) ) ;
#24478=CARTESIAN_POINT ( 'NONE',  ( 5.405949406249999534, 9.363379034771803333, -164.5937500020484094 ) ) ;
#24479=CARTESIAN_POINT ( 'NONE',  ( -9.999999999999998224, 1.224646799147353059E-15, -200.0000000000000000 ) ) ;
#24483=CARTESIAN_POINT ( 'NONE',  ( 0.000000000000000000, 0.000000000000000000, -200.0000000000000000 ) ) ;
#24486=CARTESIAN_POINT ( 'NONE',  ( 10.81189881249999729, 0.000000000000000000, -91.34375000204838102 ) ) ;
#24487=CARTESIAN_POINT ( 'NONE',  ( -5.405949406249996869, 9.363379034771805109, -55.03125000204836681 ) ) ;
#24490=CARTESIAN_POINT ( 'NONE',  ( -5.405949406250003975, -9.363379034771801557, -114.5312500020483952 ) ) ;
#24491=CARTESIAN_POINT ( 'NONE',  ( -5.405949406249996869, 9.363379034771805109, -157.0312500020484094 ) ) ;
#24494=CARTESIAN_POINT ( 'NONE',  ( -5.000000000000003553, -8.660254037844383745, -130.3750000040967905 ) ) ;
#24496=ORIENTED_EDGE ( 'NONE', *, *, #38294, .T. ) ;
#24500=CARTESIAN_POINT ( 'NONE',  ( -5.405949406249996869, 9.363379034771805109, -182.5312500020484094 ) ) ;
#24501=VERTEX_POINT ( 'NONE', #10996 ) ;
#24502=CARTESIAN_POINT ( 'NONE',  ( -2.121150477449813534E-15, -11.54700538379251284, -51.87499999999997158 ) ) ;
#24504=CARTESIAN_POINT ( 'NONE',  ( 5.000000000000000000, 8.660254037844385522, -54.62500000409675494 ) ) ;
#24505=CARTESIAN_POINT ( 'NONE',  ( -9.999999999999998224, 1.224646799147353059E-15, -19.24999999999996092 ) ) ;
#24507=CARTESIAN_POINT ( 'NONE',  ( 7.644554776091147741E-16, 12.48450537969573659, -50.65625000204838102 ) ) ;
#24508=ADVANCED_FACE ( 'NONE', ( #21731 ), #8581, .T. ) ;
#24511=CARTESIAN_POINT ( 'NONE',  ( 7.070501591499376803E-16, 11.54700538379251284, -88.62500000000000000 ) ) ;
#24512=CARTESIAN_POINT ( 'NONE',  ( 5.405949406249992428, -9.363379034771808662, -177.2812500020484094 ) ) ;
#24513=CARTESIAN_POINT ( 'NONE',  ( -9.999999999999479527, -5.773502691896549521, -73.50000000409674783 ) ) ;
#24514=CARTESIAN_POINT ( 'NONE',  ( 4.999999999999992006, -8.660254037844389075, -81.74999999999998579 ) ) ;
#24516=LINE ( 'NONE', #26887, #7696 ) ;
#24517=CARTESIAN_POINT ( 'NONE',  ( 10.00000000000102318, -5.773502691895667560, -60.62499999999995026 ) ) ;
#24518=AXIS2_PLACEMENT_3D ( 'NONE', #14437, #24190, #23973 ) ;
#24519=( BOUNDED_CURVE ( )  B_SPLINE_CURVE ( 2, ( #42220, #25840, #17369, #16732, #23879, #33803, #10056 ),
 .UNSPECIFIED., .F., .F. ) 
 B_SPLINE_CURVE_WITH_KNOTS ( ( 3, 2, 2, 3 ),
 ( 0.1455223880597014963, 0.1467661691542288538, 0.1480099502487562391, 0.1492537313432835966 ),
 .UNSPECIFIED. ) 
 CURVE ( )  GEOMETRIC_REPRESENTATION_ITEM ( )  RATIONAL_B_SPLINE_CURVE ( ( 1.000000000000000000, 0.8660254037844387076, 1.000000000000000000, 0.8660254037844387076, 1.000000000000000000, 0.8660254037844357100, 1.000000000000003109 ) ) 
 REPRESENTATION_ITEM ( '' )  );
#24520=DIRECTION ( 'NONE',  ( -0.000000000000000000, -0.000000000000000000, 1.000000000000000000 ) ) ;
#24521=CARTESIAN_POINT ( 'NONE',  ( -10.81189881249999729, 6.242252689847871849, -89.40625000204838102 ) ) ;
#24522=ORIENTED_EDGE ( 'NONE', *, *, #39892, .F. ) ;
#24526=ORIENTED_EDGE ( 'NONE', *, *, #19360, .T. ) ;
#24527=CARTESIAN_POINT ( 'NONE',  ( -10.81189881249999729, 6.242252689847871849, -38.21875000204837391 ) ) ;
#24528=CARTESIAN_POINT ( 'NONE',  ( -10.81189881249999907, -6.242252689847864744, -24.46875000204836681 ) ) ;
#24529=CARTESIAN_POINT ( 'NONE',  ( -2.293366432827344421E-15, -12.48450537969573659, -16.90625000204838102 ) ) ;
#24530=CARTESIAN_POINT ( 'NONE',  ( -5.405949406249996869, 9.363379034771805109, -65.34375000204836681 ) ) ;
#24532=CYLINDRICAL_SURFACE ( 'NONE', #36677, 9.999999999999998224 ) ;
#24533=EDGE_CURVE ( 'NONE', #5420, #7881, #28444, .T. ) ;
#24535=CARTESIAN_POINT ( 'NONE',  ( 7.644554776091147741E-16, 12.48450537969573659, -186.9687500020483810 ) ) ;
#24537=CARTESIAN_POINT ( 'NONE',  ( -9.999999999999998224, 1.224646799147353059E-15, -183.1250000040967905 ) ) ;
#24540=LINE ( 'NONE', #17820, #3967 ) ;
#24541=CARTESIAN_POINT ( 'NONE',  ( 7.644554776091147741E-16, 12.48450537969573659, -116.4687500020483952 ) ) ;
#24542=DIRECTION ( 'NONE',  ( -0.000000000000000000, -0.000000000000000000, 1.000000000000000000 ) ) ;
#24543=CARTESIAN_POINT ( 'NONE',  ( -5.405949406249996869, 9.363379034771805109, -82.03125000204839523 ) ) ;
#24544=CARTESIAN_POINT ( 'NONE',  ( -5.405949406249996869, 9.363379034771805109, -98.34375000204838102 ) ) ;
#24548=CARTESIAN_POINT ( 'NONE',  ( 10.00000000000000000, 5.773502691896255534, -155.2500000040967905 ) ) ;
#24553=CARTESIAN_POINT ( 'NONE',  ( 9.999999999999998224, 0.000000000000000000, -200.0000000000000000 ) ) ;
#24554=CARTESIAN_POINT ( 'NONE',  ( -9.999999999999998224, 1.224646799147353059E-15, -200.0000000000000000 ) ) ;
#24556=CARTESIAN_POINT ( 'NONE',  ( 7.070501591499376803E-16, 11.54700538379251284, -42.50000000409675494 ) ) ;
#24557=CARTESIAN_POINT ( 'NONE',  ( 5.000000000000000000, 8.660254037844385522, -76.74999999999998579 ) ) ;
#24559=CARTESIAN_POINT ( 'NONE',  ( 7.070501591499377789E-16, 11.54700538379251284, -81.50000000409677625 ) ) ;
#24560=VECTOR ( 'NONE', #21114, 1000.000000000000000 ) ;
#24561=LINE ( 'NONE', #37710, #14787 ) ;
#24563=CARTESIAN_POINT ( 'NONE',  ( 10.81189881249999729, 6.242252689847867408, -79.40625000204836681 ) ) ;
#24565=CARTESIAN_POINT ( 'NONE',  ( 8.660254037844444142, 15.00000000000011191, 49.99999999999998579 ) ) ;
#24568=CARTESIAN_POINT ( 'NONE',  ( 5.405949406249992428, -9.363379034771808662, -198.2812500020484094 ) ) ;
#24571=CARTESIAN_POINT ( 'NONE',  ( -10.81189881249999729, 6.242252689847871849, -17.21875000204836681 ) ) ;
#24575=CARTESIAN_POINT ( 'NONE',  ( 10.81189881249999729, 0.000000000000000000, -127.5312500020483952 ) ) ;
#24576=CARTESIAN_POINT ( 'NONE',  ( -2.121150477449813534E-15, -11.54700538379251284, -185.3750000000000284 ) ) ;
#24578=CARTESIAN_POINT ( 'NONE',  ( 10.81189881249999907, 6.242252689847868297, -106.4062500020483952 ) ) ;
#24579=ORIENTED_EDGE ( 'NONE', *, *, #11173, .T. ) ;
#24581=ORIENTED_EDGE ( 'NONE', *, *, #33696, .T. ) ;
#24583=ORIENTED_EDGE ( 'NONE', *, *, #26212, .F. ) ;
#24584=CARTESIAN_POINT ( 'NONE',  ( -5.405949406249996869, 9.363379034771805109, -37.03125000204837391 ) ) ;
#24586=CARTESIAN_POINT ( 'NONE',  ( 10.81189881249999729, 0.000000000000000000, -85.34375000204836681 ) ) ;
#24588=LINE ( 'NONE', #1059, #15577 ) ;
#24589=CARTESIAN_POINT ( 'NONE',  ( -4.999999999999996447, 8.660254037844387298, -169.8750000040967905 ) ) ;
#24591=CARTESIAN_POINT ( 'NONE',  ( -2.293366432827344421E-15, -12.48450537969573659, -127.7187500020483952 ) ) ;
#24593=CARTESIAN_POINT ( 'NONE',  ( 5.405949406249999534, 9.363379034771803333, -2.781250002048374359 ) ) ;
#24596=CARTESIAN_POINT ( 'NONE',  ( -9.999999999999998224, 5.773502691896259087, -175.7500000040967905 ) ) ;
#24597=CARTESIAN_POINT ( 'NONE',  ( 5.405949406249999534, 9.363379034771803333, -173.7812500020484094 ) ) ;
#24598=CARTESIAN_POINT ( 'NONE',  ( -9.999999999999998224, 1.224646799147353059E-15, -1.625000004096766038 ) ) ;
#24601=CARTESIAN_POINT ( 'NONE',  ( -10.81189881249999729, 1.324075727343319199E-15, -53.09375000204835970 ) ) ;
#24603=CARTESIAN_POINT ( 'NONE',  ( -10.81189881249999907, -6.242252689847864744, -11.15625000204838457 ) ) ;
#24605=CARTESIAN_POINT ( 'NONE',  ( 9.999999999999998224, 0.000000000000000000, -152.3750000040967905 ) ) ;
#24607=CARTESIAN_POINT ( 'NONE',  ( -4.999999999999996447, 8.660254037844387298, -98.99999999999998579 ) ) ;
#24609=CARTESIAN_POINT ( 'NONE',  ( -9.999999999999998224, 1.224646799147353059E-15, -105.1250000040967763 ) ) ;
#24610=( BOUNDED_CURVE ( )  B_SPLINE_CURVE ( 2, ( #38419, #38206, #8223, #25063, #34985, #28511, #35193 ),
 .UNSPECIFIED., .F., .F. ) 
 B_SPLINE_CURVE_WITH_KNOTS ( ( 3, 2, 2, 3 ),
 ( 0.7649253731343285123, 0.7661691542288557866, 0.7674129353233831718, 0.7686567164179105571 ),
 .UNSPECIFIED. ) 
 CURVE ( )  GEOMETRIC_REPRESENTATION_ITEM ( )  RATIONAL_B_SPLINE_CURVE ( ( 0.9999999999999880096, 0.8660254037844506980, 1.000000000000000000, 0.8660254037844387076, 1.000000000000000000, 0.8660254037844267172, 1.000000000000011990 ) ) 
 REPRESENTATION_ITEM ( '' )  );
#24611=CARTESIAN_POINT ( 'NONE',  ( 9.999999999999998224, 0.000000000000000000, -189.8750000040967905 ) ) ;
#24614=CARTESIAN_POINT ( 'NONE',  ( -2.293366432827344421E-15, -12.48450537969573659, -96.40625000204838102 ) ) ;
#24615=ORIENTED_EDGE ( 'NONE', *, *, #11920, .F. ) ;
#24619=CARTESIAN_POINT ( 'NONE',  ( -10.81189881249999729, 1.324075727343319199E-15, -162.7812500020484094 ) ) ;
#24621=ORIENTED_EDGE ( 'NONE', *, *, #9588, .F. ) ;
#24622=CARTESIAN_POINT ( 'NONE',  ( -9.999999999999998224, 1.224646799147353059E-15, -22.24999999999996447 ) ) ;
#24623=ADVANCED_FACE ( 'NONE', ( #35961 ), #25827, .T. ) ;
#24625=CARTESIAN_POINT ( 'NONE',  ( 10.81189881249999729, 6.242252689847867408, -29.90625000204835970 ) ) ;
#24626=CARTESIAN_POINT ( 'NONE',  ( 10.00000000000000000, 5.773502691896255534, -157.8749999999999716 ) ) ;
#24627=CARTESIAN_POINT ( 'NONE',  ( -9.999999999999479527, -5.773502691896549521, -92.62499999999997158 ) ) ;
#24629=EDGE_CURVE ( 'NONE', #40862, #36973, #5979, .T. ) ;
#24630=EDGE_CURVE ( 'NONE', #24022, #5784, #8009, .T. ) ;
#24631=CARTESIAN_POINT ( 'NONE',  ( 10.00000000000154010, -5.773502691895370020, -23.12499999999993605 ) ) ;
#24632=CARTESIAN_POINT ( 'NONE',  ( -10.81189881249999729, 6.242252689847871849, -137.4062500020484094 ) ) ;
#24633=CARTESIAN_POINT ( 'NONE',  ( -3.495063195231654873, 9.449490074020786778, 7.031793886498072016E-15 ) ) ;
#24635=ORIENTED_EDGE ( 'NONE', *, *, #4580, .F. ) ;
#24636=CARTESIAN_POINT ( 'NONE',  ( 10.81189881249999551, -6.242252689847874514, -63.15625000204837391 ) ) ;
#24638=VERTEX_POINT ( 'NONE', #26040 ) ;
#24639=ORIENTED_EDGE ( 'NONE', *, *, #21511, .T. ) ;
#24640=ADVANCED_FACE ( 'NONE', ( #19542 ), #22372, .T. ) ;
#24642=CARTESIAN_POINT ( 'NONE',  ( -2.121150477449813534E-15, -11.54700538379251284, -55.25000000409677625 ) ) ;
#24643=CARTESIAN_POINT ( 'NONE',  ( 7.644554776091147741E-16, 12.48450537969573659, -159.9687500020483810 ) ) ;
#24644=EDGE_CURVE ( 'NONE', #26035, #3072, #35872, .T. ) ;
#24646=CARTESIAN_POINT ( 'NONE',  ( 5.405949406249992428, -9.363379034771808662, -18.09375000204835260 ) ) ;
#24647=EDGE_CURVE ( 'NONE', #13289, #20204, #12392, .T. ) ;
#24648=CARTESIAN_POINT ( 'NONE',  ( -5.405949406249996869, 9.363379034771805109, -149.3437500020483810 ) ) ;
#24649=CARTESIAN_POINT ( 'NONE',  ( 5.405949406249992428, -9.363379034771808662, -132.0937500020483810 ) ) ;
#24650=CARTESIAN_POINT ( 'NONE',  ( -2.293366432827344421E-15, -12.48450537969573659, -103.9062500020483810 ) ) ;
#24652=FACE_OUTER_BOUND ( 'NONE', #16252, .T. ) ;
#24654=CARTESIAN_POINT ( 'NONE',  ( -10.81189881249999729, 6.242252689847871849, -3.718750002048365477 ) ) ;
#24656=CARTESIAN_POINT ( 'NONE',  ( -10.81189881249999729, -6.242252689847864744, -192.6562500020484094 ) ) ;
#24657=( BOUNDED_CURVE ( )  B_SPLINE_CURVE ( 2, ( #35883, #29616, #19253, #36509, #9754, #19465, #25959 ),
 .UNSPECIFIED., .F., .F. ) 
 B_SPLINE_CURVE_WITH_KNOTS ( ( 3, 2, 2, 3 ),
 ( 0.6828358208955226383, 0.6840796019900500236, 0.6853233830845772978, 0.6865671641791046831 ),
 .UNSPECIFIED. ) 
 CURVE ( )  GEOMETRIC_REPRESENTATION_ITEM ( )  RATIONAL_B_SPLINE_CURVE ( ( 0.9999999999999761302, 0.8660254037844625774, 1.000000000000000000, 0.8660254037844387076, 1.000000000000000000, 0.8660254037844148378, 1.000000000000023981 ) ) 
 REPRESENTATION_ITEM ( '' )  );
#24661=CARTESIAN_POINT ( 'NONE',  ( -2.293366432827344421E-15, -12.48450537969573659, -72.21875000204835260 ) ) ;
#24662=CARTESIAN_POINT ( 'NONE',  ( -10.81189881249999907, -6.242252689847864744, -54.46875000204838102 ) ) ;
#24663=CARTESIAN_POINT ( 'NONE',  ( -9.999999999999998224, 1.224646799147353059E-15, -200.0000000000000000 ) ) ;
#24664=CARTESIAN_POINT ( 'NONE',  ( 5.405949406249999534, 9.363379034771803333, -37.28125000204837391 ) ) ;
#24666=CARTESIAN_POINT ( 'NONE',  ( -4.999999999999996447, 8.660254037844387298, -94.87500000409677625 ) ) ;
#24668=CARTESIAN_POINT ( 'NONE',  ( -10.00000000000000000, -5.773502691896251982, -119.6249999999999858 ) ) ;
#24671=CARTESIAN_POINT ( 'NONE',  ( -10.81189881249999729, 6.242252689847871849, -8.406250002048372139 ) ) ;
#24672=ORIENTED_EDGE ( 'NONE', *, *, #29446, .F. ) ;
#24677=CARTESIAN_POINT ( 'NONE',  ( 9.999999999999998224, 0.000000000000000000, -30.87500000409676559 ) ) ;
#24678=CARTESIAN_POINT ( 'NONE',  ( 10.00000000000154010, -5.773502691895370020, -14.12499999999992895 ) ) ;
#24681=CARTESIAN_POINT ( 'NONE',  ( 5.405949406249992428, -9.363379034771808662, -142.7812500020483810 ) ) ;
#24682=ADVANCED_FACE ( 'NONE', ( #10040 ), #36382, .T. ) ;
#24683=CARTESIAN_POINT ( 'NONE',  ( 5.405949406249999534, 9.363379034771803333, -124.0937500020483952 ) ) ;
#24684=CARTESIAN_POINT ( 'NONE',  ( -4.999999999999996447, 8.660254037844387298, -103.8750000040967763 ) ) ;
#24685=FACE_OUTER_BOUND ( 'NONE', #6312, .T. ) ;
#24686=ORIENTED_EDGE ( 'NONE', *, *, #17633, .F. ) ;
#24687=EDGE_LOOP ( 'NONE', ( #34395, #26370, #39939, #27912 ) ) ;
#24688=AXIS2_PLACEMENT_3D ( 'NONE', #40363, #33293, #908 ) ;
#24689=ORIENTED_EDGE ( 'NONE', *, *, #26728, .T. ) ;
#24690=VECTOR ( 'NONE', #16472, 1000.000000000000000 ) ;
#24691=ADVANCED_FACE ( 'NONE', ( #9203 ), #16079, .T. ) ;
#24692=DIRECTION ( 'NONE',  ( -0.000000000000000000, -0.000000000000000000, 1.000000000000000000 ) ) ;
#24693=CARTESIAN_POINT ( 'NONE',  ( -10.81189881249999729, 6.242252689847871849, -192.7187500020483810 ) ) ;
#24694=CARTESIAN_POINT ( 'NONE',  ( 10.81189881249999729, 0.000000000000000000, -40.34375000204837391 ) ) ;
#24695=CARTESIAN_POINT ( 'NONE',  ( 7.070501591499376803E-16, 11.54700538379251284, -110.0000000040968047 ) ) ;
#24696=CARTESIAN_POINT ( 'NONE',  ( 4.999999999999992006, -8.660254037844389075, -74.24999999999998579 ) ) ;
#24697=CARTESIAN_POINT ( 'NONE',  ( 10.81189881249999729, 6.242252689847867408, -169.2187500020483810 ) ) ;
#24698=CARTESIAN_POINT ( 'NONE',  ( 7.644554776091147741E-16, 12.48450537969573659, -152.4687500020483810 ) ) ;
#24699=CARTESIAN_POINT ( 'NONE',  ( 9.999999999999998224, 0.000000000000000000, -24.87500000409675849 ) ) ;
#24703=CARTESIAN_POINT ( 'NONE',  ( -10.00000000000102496, 5.773502691895664007, -86.87499999999997158 ) ) ;
#24704=CARTESIAN_POINT ( 'NONE',  ( 7.070501591499376803E-16, 11.54700538379251284, -70.62499999999998579 ) ) ;
#24706=CARTESIAN_POINT ( 'NONE',  ( 5.405949406249992428, -9.363379034771808662, -90.09375000204838102 ) ) ;
#24707=CARTESIAN_POINT ( 'NONE',  ( -5.000000000000003553, -8.660254037844383745, -136.0000000000000000 ) ) ;
#24708=CARTESIAN_POINT ( 'NONE',  ( -10.81189881249999907, -6.242252689847864744, -54.65625000204838102 ) ) ;
#24711=CARTESIAN_POINT ( 'NONE',  ( 7.644554776091147741E-16, 12.48450537969573659, -115.1562500020483952 ) ) ;
#24712=CARTESIAN_POINT ( 'NONE',  ( 7.644554776091147741E-16, 12.48450537969573659, -157.1562500020484094 ) ) ;
#24715=CARTESIAN_POINT ( 'NONE',  ( 4.999999999999992006, -8.660254037844389075, -127.1250000040967620 ) ) ;
#24720=CARTESIAN_POINT ( 'NONE',  ( -5.321294541346989426, 0.000000000000000000, -220.0000000000000000 ) ) ;
#24721=CARTESIAN_POINT ( 'NONE',  ( 7.644554776091147741E-16, 12.48450537969573659, -182.6562500020484094 ) ) ;
#24724=CARTESIAN_POINT ( 'NONE',  ( -9.999999999999998224, 1.224646799147353059E-15, -55.62500000409676204 ) ) ;
#24725=VECTOR ( 'NONE', #22142, 1000.000000000000000 ) ;
#24726=CARTESIAN_POINT ( 'NONE',  ( -9.999999999999998224, 1.836970198721029589E-15, 0.000000000000000000 ) ) ;
#24727=CARTESIAN_POINT ( 'NONE',  ( 0.000000000000000000, 0.000000000000000000, -200.0000000000000000 ) ) ;
#24729=CARTESIAN_POINT ( 'NONE',  ( -10.81189881249999729, 6.242252689847871849, -53.40625000204837391 ) ) ;
#24733=CARTESIAN_POINT ( 'NONE',  ( -5.405949406250003975, -9.363379034771801557, -180.5312500020483810 ) ) ;
#24734=FACE_OUTER_BOUND ( 'NONE', #13810, .T. ) ;
#24735=CARTESIAN_POINT ( 'NONE',  ( 9.999999999999998224, 0.000000000000000000, -44.37500000409677625 ) ) ;
#24736=ORIENTED_EDGE ( 'NONE', *, *, #25479, .F. ) ;
#24737=CARTESIAN_POINT ( 'NONE',  ( 9.999999999998969713, 5.773502691896851502, -84.75000000409677625 ) ) ;
#24738=CARTESIAN_POINT ( 'NONE',  ( 4.999999999999992006, -8.660254037844389075, -60.74999999999997158 ) ) ;
#24739=CARTESIAN_POINT ( 'NONE',  ( -5.000000000000003553, -8.660254037844383745, -20.49999999999996447 ) ) ;
#24740=EDGE_CURVE ( 'NONE', #14676, #18615, #33580, .T. ) ;
#24741=CARTESIAN_POINT ( 'NONE',  ( 7.644554776091147741E-16, 12.48450537969573659, -76.15625000204839523 ) ) ;
#24742=ORIENTED_EDGE ( 'NONE', *, *, #21916, .F. ) ;
#24743=CARTESIAN_POINT ( 'NONE',  ( 0.000000000000000000, 0.000000000000000000, 0.000000000000000000 ) ) ;
#24744=CARTESIAN_POINT ( 'NONE',  ( 9.999999999999479527, 5.773502691896553074, -81.37499999999997158 ) ) ;
#24746=ORIENTED_EDGE ( 'NONE', *, *, #7477, .T. ) ;
#24747=CARTESIAN_POINT ( 'NONE',  ( -5.405949406249996869, 9.363379034771805109, -41.34375000204837391 ) ) ;
#24748=CARTESIAN_POINT ( 'NONE',  ( 9.999999999999998224, 0.000000000000000000, -186.5000000000000000 ) ) ;
#24749=CARTESIAN_POINT ( 'NONE',  ( -5.405949406249996869, 9.363379034771805109, -11.53125000204835438 ) ) ;
#24750=CARTESIAN_POINT ( 'NONE',  ( 10.81189881249999551, -6.242252689847874514, -59.96875000204837391 ) ) ;
#24751=ORIENTED_EDGE ( 'NONE', *, *, #32830, .T. ) ;
#24754=CARTESIAN_POINT ( 'NONE',  ( -5.405949406250003975, -9.363379034771801557, -193.8437500020484094 ) ) ;
#24755=CARTESIAN_POINT ( 'NONE',  ( -10.81189881249999729, 6.242252689847871849, -188.2187500020483810 ) ) ;
#24757=EDGE_CURVE ( 'NONE', #1539, #35906, #36586, .T. ) ;
#24759=CARTESIAN_POINT ( 'NONE',  ( 10.00000000000031619, -5.773502691896077010, -182.5000000040967620 ) ) ;
#24761=CARTESIAN_POINT ( 'NONE',  ( 9.999999999999998224, 0.000000000000000000, -103.9999999999999858 ) ) ;
#24763=VECTOR ( 'NONE', #19963, 1000.000000000000000 ) ;
#24764=CARTESIAN_POINT ( 'NONE',  ( -5.405949406249996869, 9.363379034771805109, -110.3437500020483810 ) ) ;
#24766=CARTESIAN_POINT ( 'NONE',  ( -5.405949406249996869, 9.363379034771805109, -79.03125000204838102 ) ) ;
#24767=CARTESIAN_POINT ( 'NONE',  ( -10.81189881249999729, -6.242252689847864744, -88.96875000204838102 ) ) ;
#24770=CARTESIAN_POINT ( 'NONE',  ( 9.999999999999998224, 0.000000000000000000, -155.3750000040967905 ) ) ;
#24774=CARTESIAN_POINT ( 'NONE',  ( 9.999999999999998224, 0.000000000000000000, -12.87500000409674783 ) ) ;
#24777=CARTESIAN_POINT ( 'NONE',  ( 9.999999999999996447, -5.773502691896262640, -71.12499999999997158 ) ) ;
#24779=CARTESIAN_POINT ( 'NONE',  ( -9.999999999999998224, 1.224646799147353059E-15, -78.12500000409677625 ) ) ;
#24782=CARTESIAN_POINT ( 'NONE',  ( 10.81189881249999551, -6.242252689847874514, -78.15625000204838102 ) ) ;
#24783=( BOUNDED_CURVE ( )  B_SPLINE_CURVE ( 2, ( #97, #10208, #310, #27053, #6355, #13220, #40197 ),
 .UNSPECIFIED., .F., .F. ) 
 B_SPLINE_CURVE_WITH_KNOTS ( ( 3, 2, 2, 3 ),
 ( 0.01865671641791046345, 0.01990049751243783138, 0.02114427860696519584, 0.02238805970149256030 ),
 .UNSPECIFIED. ) 
 CURVE ( )  GEOMETRIC_REPRESENTATION_ITEM ( )  RATIONAL_B_SPLINE_CURVE ( ( 0.9999999999999981126, 0.8660254037844405950, 1.000000000000000000, 0.8660254037844387076, 1.000000000000000000, 0.8660254037844360431, 1.000000000000002665 ) ) 
 REPRESENTATION_ITEM ( '' )  );
#24785=CARTESIAN_POINT ( 'NONE',  ( 9.999999999999998224, 0.000000000000000000, -21.49999999999996447 ) ) ;
#24787=EDGE_LOOP ( 'NONE', ( #24884, #9261, #34182, #2650 ) ) ;
#24788=CARTESIAN_POINT ( 'NONE',  ( -4.999999999999996447, 8.660254037844387298, -1.499999999999973577 ) ) ;
#24790=CARTESIAN_POINT ( 'NONE',  ( 10.81189881249999551, -6.242252689847874514, -11.96875000204837214 ) ) ;
#24791=CARTESIAN_POINT ( 'NONE',  ( -5.405949406250003975, -9.363379034771801557, -139.8437500020484094 ) ) ;
#24792=CARTESIAN_POINT ( 'NONE',  ( -2.121150477449813534E-15, -11.54700538379251284, -37.25000000409676204 ) ) ;
#24793=CARTESIAN_POINT ( 'NONE',  ( 5.405949406249992428, -9.363379034771808662, -132.2812500020483810 ) ) ;
#24794=ADVANCED_FACE ( 'NONE', ( #3586 ), #1198, .T. ) ;
#24795=CARTESIAN_POINT ( 'NONE',  ( -9.999999999999998224, 5.773502691896259087, -181.3750000000000000 ) ) ;
#24796=CARTESIAN_POINT ( 'NONE',  ( 10.00000000000051159, -5.773502691895965988, -35.50000000409674072 ) ) ;
#24797=AXIS2_PLACEMENT_3D ( 'NONE', #16736, #6418, #10479 ) ;
#24798=CARTESIAN_POINT ( 'NONE',  ( -2.293366432827344421E-15, -12.48450537969573659, -109.9062500020483952 ) ) ;
#24799=ORIENTED_EDGE ( 'NONE', *, *, #12451, .T. ) ;
#24800=CARTESIAN_POINT ( 'NONE',  ( 7.070501591499376803E-16, 11.54700538379251284, -195.1250000000000284 ) ) ;
#24802=ORIENTED_EDGE ( 'NONE', *, *, #39110, .T. ) ;
#24804=CARTESIAN_POINT ( 'NONE',  ( -5.405949406250003975, -9.363379034771801557, -41.03125000204838102 ) ) ;
#24806=CARTESIAN_POINT ( 'NONE',  ( -10.81189881249999729, 1.324075727343319199E-15, -87.59375000204836681 ) ) ;
#24808=EDGE_CURVE ( 'NONE', #8991, #37209, #34491, .T. ) ;
#24809=DIRECTION ( 'NONE',  ( 1.000000000000000000, 0.000000000000000000, 0.000000000000000000 ) ) ;
#24813=CARTESIAN_POINT ( 'NONE',  ( 10.81189881249999729, 6.242252689847867408, -112.2187500020483810 ) ) ;
#24815=CARTESIAN_POINT ( 'NONE',  ( -10.81189881249999729, -6.242252689847864744, -0.6562500020483670315 ) ) ;
#24818=CARTESIAN_POINT ( 'NONE',  ( 5.000000000000000000, 8.660254037844385522, -179.1250000040968189 ) ) ;
#24819=CARTESIAN_POINT ( 'NONE',  ( -10.81189881249999729, 6.242252689847871849, -170.4062500020484094 ) ) ;
#24820=CARTESIAN_POINT ( 'NONE',  ( -10.00000000000051337, 5.773502691895962435, -103.3749999999999858 ) ) ;
#24823=CARTESIAN_POINT ( 'NONE',  ( -10.81189881249999729, 6.242252689847871849, -53.21875000204838102 ) ) ;
#24825=CARTESIAN_POINT ( 'NONE',  ( 10.81189881249999729, 0.000000000000000000, -10.53125000204835260 ) ) ;
#24827=CARTESIAN_POINT ( 'NONE',  ( 4.999999999999992006, -8.660254037844389075, -164.6250000040967905 ) ) ;
#24829=CARTESIAN_POINT ( 'NONE',  ( 10.00000000000000000, 5.773502691896255534, -99.37499999999998579 ) ) ;
#24831=CARTESIAN_POINT ( 'NONE',  ( 10.00000000000000000, 5.773502691896255534, -108.7500000040967905 ) ) ;
#24832=CARTESIAN_POINT ( 'NONE',  ( 9.999999999999998224, 0.000000000000000000, -82.99999999999997158 ) ) ;
#24835=CARTESIAN_POINT ( 'NONE',  ( 10.81189881249999729, 6.242252689847867408, -95.90625000204839523 ) ) ;
#24836=ORIENTED_EDGE ( 'NONE', *, *, #38668, .T. ) ;
#24838=CARTESIAN_POINT ( 'NONE',  ( -5.405949406250003975, -9.363379034771801557, -158.0312500020484094 ) ) ;
#24840=ORIENTED_EDGE ( 'NONE', *, *, #37524, .F. ) ;
#24841=CARTESIAN_POINT ( 'NONE',  ( -5.000000000000003553, -8.660254037844383745, -26.49999999999996803 ) ) ;
#24842=CARTESIAN_POINT ( 'NONE',  ( -2.293366432827344421E-15, -12.48450537969573659, -30.40625000204834549 ) ) ;
#24843=CARTESIAN_POINT ( 'NONE',  ( 9.999999999999998224, 0.000000000000000000, -161.0000000000000000 ) ) ;
#24844=CARTESIAN_POINT ( 'NONE',  ( -9.999999999999998224, 1.224646799147353059E-15, -92.74999999999998579 ) ) ;
#24847=CARTESIAN_POINT ( 'NONE',  ( -10.81189881249999907, -6.242252689847864744, -134.1562500020483810 ) ) ;
#24848=CARTESIAN_POINT ( 'NONE',  ( 9.599872686178903436, 4.697423173897816717, 5.369687683974984427E-15 ) ) ;
#24850=CARTESIAN_POINT ( 'NONE',  ( 5.405949406249992428, -9.363379034771808662, -58.78125000204836681 ) ) ;
#24852=ORIENTED_EDGE ( 'NONE', *, *, #42564, .T. ) ;
#24853=ORIENTED_EDGE ( 'NONE', *, *, #19452, .F. ) ;
#24854=CARTESIAN_POINT ( 'NONE',  ( 9.999999999999998224, 0.000000000000000000, -45.87500000409677625 ) ) ;
#24855=CARTESIAN_POINT ( 'NONE',  ( 10.81189881249999907, 6.242252689847868297, -161.7187500020483810 ) ) ;
#24857=CARTESIAN_POINT ( 'NONE',  ( -10.81189881249999729, 1.324075727343319199E-15, -6.593750002048370362 ) ) ;
#24858=EDGE_CURVE ( 'NONE', #32685, #7196, #13901, .T. ) ;
#24859=CARTESIAN_POINT ( 'NONE',  ( -10.81189881249999729, 1.324075727343319199E-15, -152.0937500020483810 ) ) ;
#24860=( BOUNDED_CURVE ( )  B_SPLINE_CURVE ( 2, ( #2354, #38589, #15481, #11824, #37955, #25024, #31495 ),
 .UNSPECIFIED., .F., .F. ) 
 B_SPLINE_CURVE_WITH_KNOTS ( ( 3, 2, 2, 3 ),
 ( 0.5634328358208957610, 0.5646766169154231463, 0.5659203980099504205, 0.5671641791044778058 ),
 .UNSPECIFIED. ) 
 CURVE ( )  GEOMETRIC_REPRESENTATION_ITEM ( )  RATIONAL_B_SPLINE_CURVE ( ( 0.9999999999999761302, 0.8660254037844625774, 1.000000000000000000, 0.8660254037844387076, 1.000000000000000000, 0.8660254037844148378, 1.000000000000023981 ) ) 
 REPRESENTATION_ITEM ( '' )  );
#24862=CARTESIAN_POINT ( 'NONE',  ( -2.293366432827344421E-15, -12.48450537969573659, -102.4062500020483952 ) ) ;
#24864=CARTESIAN_POINT ( 'NONE',  ( -10.00000000000102496, 5.773502691895664007, -55.37499999999994316 ) ) ;
#24866=CARTESIAN_POINT ( 'NONE',  ( -2.293366432827344421E-15, -12.48450537969573659, -3.218750002048363257 ) ) ;
#24868=CARTESIAN_POINT ( 'NONE',  ( -2.293366432827344421E-15, -12.48450537969573659, -198.4062500020484094 ) ) ;
#24869=LINE ( 'NONE', #1774, #37148 ) ;
#24872=CARTESIAN_POINT ( 'NONE',  ( 5.405949406249992428, -9.363379034771808662, -75.09375000204838102 ) ) ;
#24873=CARTESIAN_POINT ( 'NONE',  ( -5.405949406249996869, 9.363379034771805109, -59.34375000204835970 ) ) ;
#24875=CARTESIAN_POINT ( 'NONE',  ( 7.644554776091147741E-16, 12.48450537969573659, -31.15625000204835260 ) ) ;
#24879=CARTESIAN_POINT ( 'NONE',  ( 4.999999999999992006, -8.660254037844389075, -119.2500000000000000 ) ) ;
#24883=CARTESIAN_POINT ( 'NONE',  ( 5.405949406249992428, -9.363379034771808662, -7.781250002048350822 ) ) ;
#24884=ORIENTED_EDGE ( 'NONE', *, *, #1916, .T. ) ;
#24889=AXIS2_PLACEMENT_3D ( 'NONE', #29079, #32533, #42006 ) ;
#24890=CARTESIAN_POINT ( 'NONE',  ( 10.00000000000000000, 5.773502691896255534, -26.25000000409677270 ) ) ;
#24891=CARTESIAN_POINT ( 'NONE',  ( 4.999999999999992006, -8.660254037844389075, -14.24999999999995737 ) ) ;
#24893=CARTESIAN_POINT ( 'NONE',  ( 11.54700538379253416, -19.99999999999999289, 45.00000000000009237 ) ) ;
#24894=CARTESIAN_POINT ( 'NONE',  ( -10.81189881249999729, 6.242252689847871849, -147.9062500020483810 ) ) ;
#24895=CARTESIAN_POINT ( 'NONE',  ( 10.81189881249999907, 6.242252689847868297, -128.7187500020483810 ) ) ;
#24896=CARTESIAN_POINT ( 'NONE',  ( -9.999999999999998224, 1.224646799147353059E-15, -50.74999999999996447 ) ) ;
#24897=CARTESIAN_POINT ( 'NONE',  ( -9.999999999999998224, 1.224646799147353059E-15, -127.6250000040967620 ) ) ;
#24899=ORIENTED_EDGE ( 'NONE', *, *, #9783, .F. ) ;
#24900=ORIENTED_EDGE ( 'NONE', *, *, #6705, .T. ) ;
#24901=VECTOR ( 'NONE', #24245, 1000.000000000000000 ) ;
#24903=( BOUNDED_CURVE ( )  B_SPLINE_CURVE ( 2, ( #5989, #12436, #12230, #31691, #32115, #2751, #19140 ),
 .UNSPECIFIED., .F., .F. ) 
 B_SPLINE_CURVE_WITH_KNOTS ( ( 3, 2, 2, 3 ),
 ( 0.09328358208955218889, 0.09452736318407958804, 0.09577114427860700108, 0.09701492537313441411 ),
 .UNSPECIFIED. ) 
 CURVE ( )  GEOMETRIC_REPRESENTATION_ITEM ( )  RATIONAL_B_SPLINE_CURVE ( ( 1.000000000000005995, 0.8660254037844327124, 1.000000000000000000, 0.8660254037844387076, 1.000000000000000000, 0.8660254037844297148, 1.000000000000008882 ) ) 
 REPRESENTATION_ITEM ( '' )  );
#24904=CARTESIAN_POINT ( 'NONE',  ( 5.405949406249992428, -9.363379034771808662, -181.5937500020483810 ) ) ;
#24906=CARTESIAN_POINT ( 'NONE',  ( -10.81189881249999907, -6.242252689847864744, -28.96875000204835615 ) ) ;
#24907=CARTESIAN_POINT ( 'NONE',  ( 0.000000000000000000, 0.000000000000000000, -200.0000000000000000 ) ) ;
#24908=EDGE_CURVE ( 'NONE', #41855, #32122, #7751, .T. ) ;
#24909=CARTESIAN_POINT ( 'NONE',  ( 7.644554776091147741E-16, 12.48450537969573659, -171.9687500020483810 ) ) ;
#24910=CARTESIAN_POINT ( 'NONE',  ( 10.81189881249999551, -6.242252689847874514, -152.9687500020484094 ) ) ;
#24911=CARTESIAN_POINT ( 'NONE',  ( 9.999999999999998224, 0.000000000000000000, -75.87500000409677625 ) ) ;
#24916=CARTESIAN_POINT ( 'NONE',  ( 9.999999999999998224, 0.000000000000000000, -135.5000000000000000 ) ) ;
#24917=( BOUNDED_CURVE ( )  B_SPLINE_CURVE ( 2, ( #5181, #18335, #31524, #14439, #10785, #37552, #23975 ),
 .UNSPECIFIED., .F., .F. ) 
 B_SPLINE_CURVE_WITH_KNOTS ( ( 3, 2, 2, 3 ),
 ( 0.5373134328358210032, 0.5385572139303483885, 0.5398009950248757738, 0.5410447761194030480 ),
 .UNSPECIFIED. ) 
 CURVE ( )  GEOMETRIC_REPRESENTATION_ITEM ( )  RATIONAL_B_SPLINE_CURVE ( ( 0.9999999999999880096, 0.8660254037844506980, 1.000000000000000000, 0.8660254037844387076, 1.000000000000000000, 0.8660254037844267172, 1.000000000000011990 ) ) 
 REPRESENTATION_ITEM ( '' )  );
#24920=CARTESIAN_POINT ( 'NONE',  ( 5.405949406249999534, 9.363379034771803333, -79.09375000204838102 ) ) ;
#24921=CARTESIAN_POINT ( 'NONE',  ( 7.070501591499376803E-16, 11.54700538379251284, -180.5000000040967905 ) ) ;
#24922=CARTESIAN_POINT ( 'NONE',  ( -10.81189881249999729, 1.324075727343319199E-15, -59.28125000204836681 ) ) ;
#24925=CARTESIAN_POINT ( 'NONE',  ( -10.81189881249999729, 1.324075727343319199E-15, -116.2812500020483952 ) ) ;
#24926=CARTESIAN_POINT ( 'NONE',  ( -10.81189881249999729, -6.242252689847864744, -155.1562500020484663 ) ) ;
#24928=FACE_OUTER_BOUND ( 'NONE', #35141, .T. ) ;
#24930=CARTESIAN_POINT ( 'NONE',  ( -10.00000000000000000, -5.773502691896251982, -118.5000000040967905 ) ) ;
#24932=VERTEX_POINT ( 'NONE', #355 ) ;
#24936=CARTESIAN_POINT ( 'NONE',  ( 10.81189881249999551, -6.242252689847874514, -177.1562500020484094 ) ) ;
#24937=EDGE_LOOP ( 'NONE', ( #10029, #40232, #6589, #19617, #16355, #39623 ) ) ;
#24939=CARTESIAN_POINT ( 'NONE',  ( -9.999999999999998224, 1.224646799147353059E-15, -58.62500000409676204 ) ) ;
#24941=LINE ( 'NONE', #34224, #100 ) ;
#24943=VECTOR ( 'NONE', #10160, 1000.000000000000000 ) ;
#24946=CARTESIAN_POINT ( 'NONE',  ( -2.121150477449813534E-15, -11.54700538379251284, -148.2500000040968189 ) ) ;
#24947=CARTESIAN_POINT ( 'NONE',  ( -5.405949406250003975, -9.363379034771801557, -167.0312500020484094 ) ) ;
#24949=CARTESIAN_POINT ( 'NONE',  ( -4.999999999999996447, 8.660254037844387298, -198.0000000000000000 ) ) ;
#24950=ORIENTED_EDGE ( 'NONE', *, *, #15533, .T. ) ;
#24952=FACE_OUTER_BOUND ( 'NONE', #25489, .T. ) ;
#24953=CARTESIAN_POINT ( 'NONE',  ( 9.999999999999998224, 0.000000000000000000, -195.8750000040967905 ) ) ;
#24954=VECTOR ( 'NONE', #13392, 1000.000000000000000 ) ;
#24955=CARTESIAN_POINT ( 'NONE',  ( -10.81189881249999907, -6.242252689847864744, -74.15625000204835260 ) ) ;
#24958=CARTESIAN_POINT ( 'NONE',  ( -2.121150477449813534E-15, -11.54700538379251284, -140.3750000000000000 ) ) ;
#24959=VERTEX_POINT ( 'NONE', #10887 ) ;
#24961=VERTEX_POINT ( 'NONE', #37443 ) ;
#24962=CARTESIAN_POINT ( 'NONE',  ( -10.81189881249999729, 1.324075727343319199E-15, -36.59375000204836681 ) ) ;
#24963=CARTESIAN_POINT ( 'NONE',  ( -10.00000000000051337, 5.773502691895962435, -73.75000000409674783 ) ) ;
#24964=CARTESIAN_POINT ( 'NONE',  ( -2.293366432827344421E-15, -12.48450537969573659, -7.906250002048370362 ) ) ;
#24965=CARTESIAN_POINT ( 'NONE',  ( -10.81189881249999729, 1.324075727343319199E-15, -65.09375000204836681 ) ) ;
#24966=VERTEX_POINT ( 'NONE', #7886 ) ;
#24969=CARTESIAN_POINT ( 'NONE',  ( -5.405949406249996869, 9.363379034771805109, -197.3437500020484094 ) ) ;
#24970=CARTESIAN_POINT ( 'NONE',  ( -10.81189881249999729, 1.324075727343319199E-15, -174.5937500020484094 ) ) ;
#24975=CARTESIAN_POINT ( 'NONE',  ( -9.999999999999479527, -5.773502691896549521, -102.0000000040967620 ) ) ;
#24977=CARTESIAN_POINT ( 'NONE',  ( 10.81189881249999907, 6.242252689847868297, -103.2187500020483810 ) ) ;
#24978=DIRECTION ( 'NONE',  ( -0.000000000000000000, -0.000000000000000000, 1.000000000000000000 ) ) ;
#24979=CARTESIAN_POINT ( 'NONE',  ( 7.644554776091147741E-16, 12.48450537969573659, -82.15625000204838102 ) ) ;
#24980=CARTESIAN_POINT ( 'NONE',  ( 5.405949406249999534, 9.363379034771803333, -91.09375000204838102 ) ) ;
#24982=CARTESIAN_POINT ( 'NONE',  ( -9.999999999999998224, 5.773502691896259087, -153.2500000040967620 ) ) ;
#24988=CARTESIAN_POINT ( 'NONE',  ( 9.999999999999998224, 0.000000000000000000, -91.99999999999998579 ) ) ;
#24990=ORIENTED_EDGE ( 'NONE', *, *, #1993, .F. ) ;
#24991=CARTESIAN_POINT ( 'NONE',  ( 4.999999999999992006, -8.660254037844389075, -66.74999999999997158 ) ) ;
#24993=CARTESIAN_POINT ( 'NONE',  ( 4.999999999999992006, -8.660254037844389075, -83.62500000409677625 ) ) ;
#24998=CARTESIAN_POINT ( 'NONE',  ( 10.81189881249999729, 6.242252689847867408, -73.40625000204838102 ) ) ;
#25000=DIRECTION ( 'NONE',  ( -0.000000000000000000, -0.000000000000000000, 1.000000000000000000 ) ) ;
#25002=EDGE_LOOP ( 'NONE', ( #37614, #6828, #19556, #41103 ) ) ;
#25003=CARTESIAN_POINT ( 'NONE',  ( 7.644554776091147741E-16, 12.48450537969573659, -190.1562500020484094 ) ) ;
#25005=CARTESIAN_POINT ( 'NONE',  ( -10.81189881249999729, -6.242252689847864744, -7.968750002048352599 ) ) ;
#25006=CARTESIAN_POINT ( 'NONE',  ( 9.999999999999998224, 0.000000000000000000, -122.0000000000000000 ) ) ;
#25007=CARTESIAN_POINT ( 'NONE',  ( 10.81189881249999907, 6.242252689847868297, -146.7187500020484094 ) ) ;
#25008=CARTESIAN_POINT ( 'NONE',  ( 7.070501591499376803E-16, 11.54700538379251284, -133.6250000000000000 ) ) ;
#25010=CARTESIAN_POINT ( 'NONE',  ( 5.000000000000000000, 8.660254037844385522, -180.2500000000000284 ) ) ;
#25011=CARTESIAN_POINT ( 'NONE',  ( -4.999999999999996447, 8.660254037844387298, -106.4999999999999858 ) ) ;
#25012=CARTESIAN_POINT ( 'NONE',  ( 10.81189881249999729, 0.000000000000000000, -103.5312500020483810 ) ) ;
#25013=ORIENTED_EDGE ( 'NONE', *, *, #37146, .T. ) ;
#25014=CARTESIAN_POINT ( 'NONE',  ( 9.999999999999742428, 5.773502691896404748, -138.7500000040967905 ) ) ;
#25015=ORIENTED_EDGE ( 'NONE', *, *, #21578, .F. ) ;
#25016=ORIENTED_EDGE ( 'NONE', *, *, #12166, .T. ) ;
#25017=CARTESIAN_POINT ( 'NONE',  ( 5.405949406249992428, -9.363379034771808662, -39.28125000204838102 ) ) ;
#25019=CARTESIAN_POINT ( 'NONE',  ( 10.81189881249999907, 6.242252689847868297, -88.21875000204838102 ) ) ;
#25020=CARTESIAN_POINT ( 'NONE',  ( 9.999999999999998224, 0.000000000000000000, -156.5000000000000000 ) ) ;
#25022=CARTESIAN_POINT ( 'NONE',  ( -9.999999999999996447, 5.773502691896259975, -169.7500000040967905 ) ) ;
#25024=CARTESIAN_POINT ( 'NONE',  ( 10.00000000000102318, -5.773502691895667560, -86.12499999999992895 ) ) ;
#25025=CARTESIAN_POINT ( 'NONE',  ( 5.405949406249992428, -9.363379034771808662, -115.5937500020483810 ) ) ;
#25027=CARTESIAN_POINT ( 'NONE',  ( -10.81189881249999729, -6.242252689847864744, -2.156250002048374359 ) ) ;
#25030=CARTESIAN_POINT ( 'NONE',  ( -2.121150477449813534E-15, -11.54700538379251284, -175.2500000040968189 ) ) ;
#25031=CARTESIAN_POINT ( 'NONE',  ( 7.644554776091147741E-16, 12.48450537969573659, -172.1562500020484094 ) ) ;
#25032=( BOUNDED_CURVE ( )  B_SPLINE_CURVE ( 2, ( #15622, #19090, #34876, #25166, #32274, #35720, #5299 ),
 .UNSPECIFIED., .F., .F. ) 
 B_SPLINE_CURVE_WITH_KNOTS ( ( 3, 2, 2, 3 ),
 ( 0.8432835820895525636, 0.8445273631840799489, 0.8457711442786073341, 0.8470149253731346084 ),
 .UNSPECIFIED. ) 
 CURVE ( )  GEOMETRIC_REPRESENTATION_ITEM ( )  RATIONAL_B_SPLINE_CURVE ( ( 0.9999999999999641398, 0.8660254037844745678, 1.000000000000000000, 0.8660254037844387076, 1.000000000000000000, 0.8660254037844028474, 1.000000000000035971 ) ) 
 REPRESENTATION_ITEM ( '' )  );
#25033=CARTESIAN_POINT ( 'NONE',  ( 9.999999999999998224, 0.000000000000000000, -69.49999999999997158 ) ) ;
#25036=CARTESIAN_POINT ( 'NONE',  ( -10.81189881249999729, -6.242252689847864744, -42.46875000204835260 ) ) ;
#25038=CARTESIAN_POINT ( 'NONE',  ( -5.405949406250003975, -9.363379034771801557, -2.031250002048373915 ) ) ;
#25040=CARTESIAN_POINT ( 'NONE',  ( -2.121150477449813534E-15, -11.54700538379251284, -164.7500000040968189 ) ) ;
#25042=CARTESIAN_POINT ( 'NONE',  ( 4.999999999999992006, -8.660254037844389075, -86.24999999999998579 ) ) ;
#25044=CARTESIAN_POINT ( 'NONE',  ( 9.999999999999998224, 0.000000000000000000, -107.3750000040967763 ) ) ;
#25045=CARTESIAN_POINT ( 'NONE',  ( 11.54700538379253416, -19.99999999999999289, 0.000000000000000000 ) ) ;
#25048=CARTESIAN_POINT ( 'NONE',  ( -10.81189881249999729, -6.242252689847864744, -101.1562500020483952 ) ) ;
#25051=CARTESIAN_POINT ( 'NONE',  ( -4.999999999999996447, 8.660254037844387298, -4.499999999999976019 ) ) ;
#25052=CARTESIAN_POINT ( 'NONE',  ( -10.81189881249999907, -6.242252689847864744, -155.1562500020484094 ) ) ;
#25055=CARTESIAN_POINT ( 'NONE',  ( 9.999999999999996447, -5.773502691896262640, -26.12499999999998224 ) ) ;
#25056=CARTESIAN_POINT ( 'NONE',  ( -10.81189881249999729, -6.242252689847864744, -29.15625000204835970 ) ) ;
#25057=CARTESIAN_POINT ( 'NONE',  ( -10.00000000000000000, -5.773502691896251982, -161.6250000000000284 ) ) ;
#25061=CARTESIAN_POINT ( 'NONE',  ( -2.293366432827344421E-15, -12.48450537969573659, -127.9062500020483952 ) ) ;
#25062=CARTESIAN_POINT ( 'NONE',  ( -3.096741045364464817, 9.605691705790990298, 4.524943085473206850E-15 ) ) ;
#25063=CARTESIAN_POINT ( 'NONE',  ( -2.121150477449813534E-15, -11.54700538379251284, -44.75000000409676204 ) ) ;
#25064=ORIENTED_EDGE ( 'NONE', *, *, #37835, .F. ) ;
#25065=CARTESIAN_POINT ( 'NONE',  ( -5.405949406250003975, -9.363379034771801557, -65.03125000204838102 ) ) ;
#25067=CARTESIAN_POINT ( 'NONE',  ( 10.81189881249999729, 0.000000000000000000, -107.8437500020483810 ) ) ;
#25070=CARTESIAN_POINT ( 'NONE',  ( -9.999999999999676703, -5.773502691896437611, -184.1249999999999716 ) ) ;
#25071=CARTESIAN_POINT ( 'NONE',  ( 10.81189881249999551, -6.242252689847874514, -154.4687500020484094 ) ) ;
#25073=CARTESIAN_POINT ( 'NONE',  ( -10.81189881249999729, 1.324075727343319199E-15, -11.09375000204834727 ) ) ;
#25074=CARTESIAN_POINT ( 'NONE',  ( 10.81189881249999729, 0.000000000000000000, -140.8437500020483810 ) ) ;
#25075=CARTESIAN_POINT ( 'NONE',  ( 10.81189881249999551, -6.242252689847874514, -97.65625000204839523 ) ) ;
#25077=CARTESIAN_POINT ( 'NONE',  ( -4.999999999999996447, 8.660254037844387298, -187.5000000000000000 ) ) ;
#25079=CARTESIAN_POINT ( 'NONE',  ( -10.81189881249999907, -6.242252689847864744, -4.968750002048339276 ) ) ;
#25081=CARTESIAN_POINT ( 'NONE',  ( -10.81189881249999729, 6.242252689847871849, -191.4062500020484094 ) ) ;
#25082=CARTESIAN_POINT ( 'NONE',  ( 10.00000000000102318, -5.773502691895667560, -5.500000004096742501 ) ) ;
#25085=CARTESIAN_POINT ( 'NONE',  ( 10.81189881249999729, 6.242252689847867408, -64.21875000204838102 ) ) ;
#25086=CARTESIAN_POINT ( 'NONE',  ( 7.644554776091147741E-16, 12.48450537969573659, -59.46875000204837391 ) ) ;
#25088=CARTESIAN_POINT ( 'NONE',  ( 10.81189881249999729, 0.000000000000000000, -27.03125000204836681 ) ) ;
#25090=DIRECTION ( 'NONE',  ( 1.000000000000000000, 0.000000000000000000, 0.000000000000000000 ) ) ;
#25092=CARTESIAN_POINT ( 'NONE',  ( 9.999999999999998224, 0.000000000000000000, -119.0000000000000000 ) ) ;
#25096=CARTESIAN_POINT ( 'NONE',  ( 10.81189881249999729, 0.000000000000000000, -13.53125000204835615 ) ) ;
#25097=ORIENTED_EDGE ( 'NONE', *, *, #30417, .T. ) ;
#25102=CARTESIAN_POINT ( 'NONE',  ( 7.070501591499377789E-16, 11.54700538379251284, -26.00000000409676915 ) ) ;
#25105=CARTESIAN_POINT ( 'NONE',  ( -2.121150477449813534E-15, -11.54700538379251284, -105.8749999999999858 ) ) ;
#25106=CARTESIAN_POINT ( 'NONE',  ( 10.81189881249999729, 0.000000000000000000, -148.5312500020483810 ) ) ;
#25107=CARTESIAN_POINT ( 'NONE',  ( -10.81189881249999907, -6.242252689847864744, -124.9687500020483810 ) ) ;
#25110=CARTESIAN_POINT ( 'NONE',  ( 9.999999999999998224, 0.000000000000000000, -57.49999999999996447 ) ) ;
#25114=VERTEX_POINT ( 'NONE', #34646 ) ;
#25115=( BOUNDED_CURVE ( )  B_SPLINE_CURVE ( 2, ( #7754, #34301, #17867, #859, #14840, #4718, #18089 ),
 .UNSPECIFIED., .F., .F. ) 
 B_SPLINE_CURVE_WITH_KNOTS ( ( 3, 2, 2, 3 ),
 ( 0.6529850746268659467, 0.6542288557213932210, 0.6554726368159206062, 0.6567164179104479915 ),
 .UNSPECIFIED. ) 
 CURVE ( )  GEOMETRIC_REPRESENTATION_ITEM ( )  RATIONAL_B_SPLINE_CURVE ( ( 0.9999999999999761302, 0.8660254037844625774, 1.000000000000000000, 0.8660254037844387076, 1.000000000000000000, 0.8660254037844148378, 1.000000000000023981 ) ) 
 REPRESENTATION_ITEM ( '' )  );
#25116=DIRECTION ( 'NONE',  ( -0.000000000000000000, -0.000000000000000000, 1.000000000000000000 ) ) ;
#25117=CARTESIAN_POINT ( 'NONE',  ( -10.81189881249999729, 1.324075727343319199E-15, -179.0937500020484094 ) ) ;
#25118=CARTESIAN_POINT ( 'NONE',  ( -10.81189881249999729, 1.324075727343319199E-15, -30.59375000204836326 ) ) ;
#25119=CARTESIAN_POINT ( 'NONE',  ( 9.999999999999998224, 0.000000000000000000, -200.0000000000000000 ) ) ;
#25120=CARTESIAN_POINT ( 'NONE',  ( 10.81189881249999729, 6.242252689847867408, -160.2187500020483810 ) ) ;
#25121=CARTESIAN_POINT ( 'NONE',  ( 10.81189881249999551, -6.242252689847874514, -151.4687500020483810 ) ) ;
#25125=FACE_OUTER_BOUND ( 'NONE', #33443, .T. ) ;
#25126=CARTESIAN_POINT ( 'NONE',  ( 9.999999999999998224, 0.000000000000000000, -158.0000000000000000 ) ) ;
#25128=CARTESIAN_POINT ( 'NONE',  ( -10.81189881249999729, 6.242252689847871849, -80.21875000204838102 ) ) ;
#25129=CARTESIAN_POINT ( 'NONE',  ( -9.999999999999998224, 1.224646799147353059E-15, -200.0000000000000000 ) ) ;
#25130=CARTESIAN_POINT ( 'NONE',  ( -2.293366432827344421E-15, -12.48450537969573659, -49.90625000204838102 ) ) ;
#25133=CARTESIAN_POINT ( 'NONE',  ( -2.293366432827344421E-15, -12.48450537969573659, -112.9062500020483952 ) ) ;
#25134=CARTESIAN_POINT ( 'NONE',  ( 10.81189881249999729, 0.000000000000000000, -150.0312500020483810 ) ) ;
#25135=CARTESIAN_POINT ( 'NONE',  ( 0.000000000000000000, 0.000000000000000000, -200.0000000000000000 ) ) ;
#25137=CARTESIAN_POINT ( 'NONE',  ( -10.00000000000000000, -5.773502691896251982, -123.0000000040968047 ) ) ;
#25142=DIRECTION ( 'NONE',  ( -0.000000000000000000, -0.000000000000000000, 1.000000000000000000 ) ) ;
#25143=CARTESIAN_POINT ( 'NONE',  ( -10.81189881249999729, 6.242252689847871849, -177.9062500020484094 ) ) ;
#25144=ORIENTED_EDGE ( 'NONE', *, *, #35571, .T. ) ;
#25146=CARTESIAN_POINT ( 'NONE',  ( 5.000000000000000000, 8.660254037844385522, -48.62500000409678336 ) ) ;
#25150=CARTESIAN_POINT ( 'NONE',  ( 9.999999999999998224, 0.000000000000000000, -147.8750000040967905 ) ) ;
#25151=CARTESIAN_POINT ( 'NONE',  ( 10.81189881249999729, 0.000000000000000000, -168.0312500020484094 ) ) ;
#25152=CARTESIAN_POINT ( 'NONE',  ( -4.999999999999996447, 8.660254037844387298, -1.875000004096766260 ) ) ;
#25153=CARTESIAN_POINT ( 'NONE',  ( -2.121150477449813534E-15, -11.54700538379251284, -56.37499999999997868 ) ) ;
#25154=ADVANCED_FACE ( 'NONE', ( #14543 ), #38295, .T. ) ;
#25156=CARTESIAN_POINT ( 'NONE',  ( 9.999999999999998224, 0.000000000000000000, -161.0000000000000000 ) ) ;
#25157=EDGE_CURVE ( 'NONE', #26580, #4606, #24941, .T. ) ;
#25158=ADVANCED_FACE ( 'NONE', ( #37872 ), #34861, .T. ) ;
#25159=CARTESIAN_POINT ( 'NONE',  ( -9.999999999999998224, 1.224646799147353059E-15, -176.7500000000000284 ) ) ;
#25163=CARTESIAN_POINT ( 'NONE',  ( -10.81189881249999729, 6.242252689847871849, -75.90625000204838102 ) ) ;
#25164=ORIENTED_EDGE ( 'NONE', *, *, #2444, .F. ) ;
#25166=CARTESIAN_POINT ( 'NONE',  ( 7.070501591499376803E-16, 11.54700538379251284, -30.12499999999995026 ) ) ;
#25169=ORIENTED_EDGE ( 'NONE', *, *, #12999, .F. ) ;
#25170=CARTESIAN_POINT ( 'NONE',  ( -5.405949406249996869, 9.363379034771805109, -26.34375000204835970 ) ) ;
#25172=CARTESIAN_POINT ( 'NONE',  ( 10.81189881249999907, 6.242252689847868297, -7.406250002048366810 ) ) ;
#25174=CARTESIAN_POINT ( 'NONE',  ( -5.405949406250003975, -9.363379034771801557, -54.34375000204835970 ) ) ;
#25175=ORIENTED_EDGE ( 'NONE', *, *, #13341, .T. ) ;
#25176=CARTESIAN_POINT ( 'NONE',  ( 0.000000000000000000, 0.000000000000000000, -200.0000000000000000 ) ) ;
#25178=ADVANCED_FACE ( 'NONE', ( #18649 ), #5073, .T. ) ;
#25179=CARTESIAN_POINT ( 'NONE',  ( -10.81189881249999729, 1.324075727343319199E-15, -194.0937500020484094 ) ) ;
#25180=CARTESIAN_POINT ( 'NONE',  ( -5.405949406249996869, 9.363379034771805109, -179.3437500020483810 ) ) ;
#25183=CARTESIAN_POINT ( 'NONE',  ( -9.999999999999998224, 1.224646799147353059E-15, -200.0000000000000000 ) ) ;
#25184=LINE ( 'NONE', #38325, #31589 ) ;
#25185=ADVANCED_FACE ( 'NONE', ( #41527 ), #15189, .T. ) ;
#25187=CARTESIAN_POINT ( 'NONE',  ( -5.405949406249996869, 9.363379034771805109, -102.8437500020483810 ) ) ;
#25188=CARTESIAN_POINT ( 'NONE',  ( 5.405949406249992428, -9.363379034771808662, -79.78125000204838102 ) ) ;
#25189=CARTESIAN_POINT ( 'NONE',  ( -10.81189881249999729, 1.324075727343319199E-15, -89.09375000204838102 ) ) ;
#25190=EDGE_CURVE ( 'NONE', #34698, #33370, #25412, .T. ) ;
#25192=CARTESIAN_POINT ( 'NONE',  ( 9.999999999999996447, -5.773502691896262640, -143.5000000040967905 ) ) ;
#25198=CARTESIAN_POINT ( 'NONE',  ( 9.999999999999998224, 0.000000000000000000, -37.99999999999997868 ) ) ;
#25200=VERTEX_POINT ( 'NONE', #31843 ) ;
#25201=CARTESIAN_POINT ( 'NONE',  ( 10.00000000000000000, 5.773502691896255534, -67.87500000000000000 ) ) ;
#25203=CARTESIAN_POINT ( 'NONE',  ( 4.999999999999992006, -8.660254037844389075, -70.12500000409677625 ) ) ;
#25204=EDGE_CURVE ( 'NONE', #20043, #6102, #8268, .T. ) ;
#25205=CARTESIAN_POINT ( 'NONE',  ( -5.000000000000003553, -8.660254037844383745, -142.3750000040967905 ) ) ;
#25207=CARTESIAN_POINT ( 'NONE',  ( -10.81189881249999729, 6.242252689847871849, -75.90625000204838102 ) ) ;
#25209=CYLINDRICAL_SURFACE ( 'NONE', #13479, 9.999999999999998224 ) ;
#25212=CARTESIAN_POINT ( 'NONE',  ( -10.81189881249999907, -6.242252689847864744, -194.1562500020484094 ) ) ;
#25214=CARTESIAN_POINT ( 'NONE',  ( 7.644554776091147741E-16, 12.48450537969573659, -5.468750002048341941 ) ) ;
#25215=CARTESIAN_POINT ( 'NONE',  ( -9.999999999999998224, 1.224646799147353059E-15, -186.1250000040967905 ) ) ;
#25216=CARTESIAN_POINT ( 'NONE',  ( 10.81189881249999729, 0.000000000000000000, -145.3437500020483810 ) ) ;
#25218=DIRECTION ( 'NONE',  ( -0.000000000000000000, -0.000000000000000000, 1.000000000000000000 ) ) ;
#25219=CARTESIAN_POINT ( 'NONE',  ( 4.999999999999992006, -8.660254037844389075, -176.2500000000000284 ) ) ;
#25220=CARTESIAN_POINT ( 'NONE',  ( -2.293366432827344421E-15, -12.48450537969573659, -103.9062500020483810 ) ) ;
#25221=ORIENTED_EDGE ( 'NONE', *, *, #18057, .F. ) ;
#25222=ORIENTED_EDGE ( 'NONE', *, *, #15218, .T. ) ;
#25223=ORIENTED_EDGE ( 'NONE', *, *, #18562, .F. ) ;
#25224=CARTESIAN_POINT ( 'NONE',  ( -2.293366432827344421E-15, -12.48450537969573659, -28.90625000204835615 ) ) ;
#25226=CARTESIAN_POINT ( 'NONE',  ( -10.81189881249999907, -6.242252689847864744, -75.46875000204836681 ) ) ;
#25228=CYLINDRICAL_SURFACE ( 'NONE', #29374, 9.999999999999998224 ) ;
#25231=DIRECTION ( 'NONE',  ( 1.000000000000000000, 0.000000000000000000, 0.000000000000000000 ) ) ;
#25233=CARTESIAN_POINT ( 'NONE',  ( -2.121150477449813534E-15, -11.54700538379251284, -14.75000000409676737 ) ) ;
#25235=CARTESIAN_POINT ( 'NONE',  ( -10.81189881249999729, 1.324075727343319199E-15, -119.0937500020483810 ) ) ;
#25236=VECTOR ( 'NONE', #30301, 1000.000000000000000 ) ;
#25237=( BOUNDED_CURVE ( )  B_SPLINE_CURVE ( 2, ( #41697, #35252, #5687, #28779, #15366, #5889, #19046 ),
 .UNSPECIFIED., .F., .F. ) 
 B_SPLINE_CURVE_WITH_KNOTS ( ( 3, 2, 2, 3 ),
 ( 0.4888059701492538101, 0.4900497512437811398, 0.4912935323383085806, 0.4925373134328359104 ),
 .UNSPECIFIED. ) 
 CURVE ( )  GEOMETRIC_REPRESENTATION_ITEM ( )  RATIONAL_B_SPLINE_CURVE ( ( 0.9999999999999940048, 0.8660254037844447028, 1.000000000000000000, 0.8660254037844387076, 1.000000000000000000, 0.8660254037844267172, 1.000000000000011990 ) ) 
 REPRESENTATION_ITEM ( '' )  );
#25241=CARTESIAN_POINT ( 'NONE',  ( 5.000000000000000000, 8.660254037844385522, -167.1250000040967905 ) ) ;
#25242=CARTESIAN_POINT ( 'NONE',  ( -10.81189881249999729, -6.242252689847864744, -168.6562500020484094 ) ) ;
#25246=CARTESIAN_POINT ( 'NONE',  ( 10.81189881249999729, 0.000000000000000000, -41.84375000204837391 ) ) ;
#25248=CARTESIAN_POINT ( 'NONE',  ( 5.405949406249999534, 9.363379034771803333, -1.281250002048373027 ) ) ;
#25250=CARTESIAN_POINT ( 'NONE',  ( -2.121150477449813534E-15, -11.54700538379251284, -152.7500000040967620 ) ) ;
#25252=CARTESIAN_POINT ( 'NONE',  ( 5.000000000000000000, 8.660254037844385522, -88.74999999999998579 ) ) ;
#25254=CARTESIAN_POINT ( 'NONE',  ( -10.00000000000000000, -5.773502691896251982, -105.0000000040967763 ) ) ;
#25257=CARTESIAN_POINT ( 'NONE',  ( 10.81189881249999729, 6.242252689847867408, -100.4062500020483952 ) ) ;
#25258=ORIENTED_EDGE ( 'NONE', *, *, #26241, .F. ) ;
#25260=CARTESIAN_POINT ( 'NONE',  ( 9.999999999998456346, 5.773502691897149042, -29.25000000409671941 ) ) ;
#25261=CARTESIAN_POINT ( 'NONE',  ( 10.81189881249999907, 6.242252689847868297, -160.4062500020484094 ) ) ;
#25263=ORIENTED_EDGE ( 'NONE', *, *, #37286, .F. ) ;
#25264=CARTESIAN_POINT ( 'NONE',  ( -2.121150477449813534E-15, -11.54700538379251284, -20.37499999999996803 ) ) ;
#25265=CARTESIAN_POINT ( 'NONE',  ( -5.405949406249996869, 9.363379034771805109, -28.03125000204837036 ) ) ;
#25266=CARTESIAN_POINT ( 'NONE',  ( -5.000000000000003553, -8.660254037844383745, -154.0000000000000000 ) ) ;
#25269=CARTESIAN_POINT ( 'NONE',  ( 4.999999999999992006, -8.660254037844389075, -195.7500000000000000 ) ) ;
#25270=CARTESIAN_POINT ( 'NONE',  ( 10.81189881249999551, -6.242252689847874514, -127.6562500020483952 ) ) ;
#25271=EDGE_LOOP ( 'NONE', ( #26836, #39595, #33953, #23398 ) ) ;
#25272=FACE_OUTER_BOUND ( 'NONE', #22292, .T. ) ;
#25274=VERTEX_POINT ( 'NONE', #28170 ) ;
#25275=CARTESIAN_POINT ( 'NONE',  ( -10.81189881249999729, 1.324075727343319199E-15, -56.28125000204836681 ) ) ;
#25277=EDGE_CURVE ( 'NONE', #15872, #26632, #40249, .T. ) ;
#25278=CARTESIAN_POINT ( 'NONE',  ( 5.405949406249992428, -9.363379034771808662, -112.5937500020483810 ) ) ;
#25280=ORIENTED_EDGE ( 'NONE', *, *, #38356, .F. ) ;
#25283=CARTESIAN_POINT ( 'NONE',  ( -10.81189881249999729, 6.242252689847871849, -158.2187500020483810 ) ) ;
#25285=CARTESIAN_POINT ( 'NONE',  ( 7.644554776091147741E-16, 12.48450537969573659, -6.968750002048349046 ) ) ;
#25286=CARTESIAN_POINT ( 'NONE',  ( -5.405949406250003975, -9.363379034771801557, -136.8437500020484094 ) ) ;
#25288=CARTESIAN_POINT ( 'NONE',  ( -9.999999999999998224, 1.224646799147353059E-15, -187.2500000000000000 ) ) ;
#25290=CARTESIAN_POINT ( 'NONE',  ( 10.81189881249999907, 6.242252689847868297, 0.2812499979516534521 ) ) ;
#25292=ADVANCED_FACE ( 'NONE', ( #28812 ), #9364, .T. ) ;
#25293=CARTESIAN_POINT ( 'NONE',  ( -10.81189881249999729, 1.324075727343319199E-15, -195.7812500020484094 ) ) ;
#25294=CARTESIAN_POINT ( 'NONE',  ( -2.121150477449813534E-15, -11.54700538379251284, -5.750000004096771811 ) ) ;
#25297=CARTESIAN_POINT ( 'NONE',  ( -10.81189881249999729, -6.242252689847864744, -67.96875000204838102 ) ) ;
#25298=CARTESIAN_POINT ( 'NONE',  ( 5.405949406249992428, -9.363379034771808662, -60.09375000204835970 ) ) ;
#25300=CARTESIAN_POINT ( 'NONE',  ( 10.81189881249999551, -6.242252689847874514, -25.65625000204839168 ) ) ;
#25302=CARTESIAN_POINT ( 'NONE',  ( 7.070501591499376803E-16, 11.54700538379251284, -32.00000000409674783 ) ) ;
#25304=CARTESIAN_POINT ( 'NONE',  ( -10.00000000000000000, -5.773502691896251982, -115.1249999999999858 ) ) ;
#25305=CARTESIAN_POINT ( 'NONE',  ( -5.000000000000003553, -8.660254037844383745, -170.5000000000000000 ) ) ;
#25308=CARTESIAN_POINT ( 'NONE',  ( 10.81189881249999729, 6.242252689847867408, -13.40625000204836326 ) ) ;
#25310=CARTESIAN_POINT ( 'NONE',  ( -4.999999999999996447, 8.660254037844387298, -121.5000000000000000 ) ) ;
#25314=CARTESIAN_POINT ( 'NONE',  ( -5.000000000000003553, -8.660254037844383745, -38.49999999999997868 ) ) ;
#25315=CARTESIAN_POINT ( 'NONE',  ( -9.999999999999998224, 1.224646799147353059E-15, -22.62500000409675849 ) ) ;
#25316=CYLINDRICAL_SURFACE ( 'NONE', #803, 9.999999999999998224 ) ;
#25318=CARTESIAN_POINT ( 'NONE',  ( -9.999999999999998224, 1.224646799147353059E-15, -78.12500000409677625 ) ) ;
#25319=CARTESIAN_POINT ( 'NONE',  ( 7.644554776091147741E-16, 12.48450537969573659, -148.1562500020484094 ) ) ;
#25320=CARTESIAN_POINT ( 'NONE',  ( 10.81189881249999729, 0.000000000000000000, -151.5312500020484094 ) ) ;
#25321=CARTESIAN_POINT ( 'NONE',  ( -10.00000000000154188, 5.773502691895366468, -50.87499999999994316 ) ) ;
#25323=ORIENTED_EDGE ( 'NONE', *, *, #30717, .T. ) ;
#25325=ORIENTED_EDGE ( 'NONE', *, *, #2221, .F. ) ;
#25327=ORIENTED_EDGE ( 'NONE', *, *, #25918, .F. ) ;
#25329=CARTESIAN_POINT ( 'NONE',  ( 5.405949406249992428, -9.363379034771808662, -180.0937500020484094 ) ) ;
#25330=CARTESIAN_POINT ( 'NONE',  ( -10.81189881249999729, 1.324075727343319199E-15, -27.59375000204836326 ) ) ;
#25331=CYLINDRICAL_SURFACE ( 'NONE', #6079, 9.999999999999998224 ) ;
#25332=CARTESIAN_POINT ( 'NONE',  ( 5.405949406249999534, 9.363379034771803333, -164.5937500020484094 ) ) ;
#25333=CARTESIAN_POINT ( 'NONE',  ( -2.293366432827344421E-15, -12.48450537969573659, -153.2187500020483810 ) ) ;
#25340=CARTESIAN_POINT ( 'NONE',  ( 10.81189881249999907, 6.242252689847868297, -77.71875000204838102 ) ) ;
#25341=CARTESIAN_POINT ( 'NONE',  ( -10.00000000000031797, 5.773502691896072569, -184.7500000040968189 ) ) ;
#25342=CARTESIAN_POINT ( 'NONE',  ( -10.81189881249999907, -6.242252689847864744, -53.15625000204837391 ) ) ;
#25344=EDGE_CURVE ( 'NONE', #12182, #17690, #38932, .T. ) ;
#25346=CARTESIAN_POINT ( 'NONE',  ( -5.000000000000003553, -8.660254037844383745, -137.5000000000000000 ) ) ;
#25347=CARTESIAN_POINT ( 'NONE',  ( 10.81189881249999551, -6.242252689847874514, -150.1562500020484094 ) ) ;
#25350=CARTESIAN_POINT ( 'NONE',  ( -2.121150477449813534E-15, -11.54700538379251284, -121.2500000040967905 ) ) ;
#25355=CARTESIAN_POINT ( 'NONE',  ( 7.070501591499376803E-16, 11.54700538379251284, -52.62499999999997868 ) ) ;
#25356=CARTESIAN_POINT ( 'NONE',  ( -2.293366432827344421E-15, -12.48450537969573659, -174.4062500020483810 ) ) ;
#25357=CARTESIAN_POINT ( 'NONE',  ( -9.999999999999998224, 5.773502691896259087, -46.75000000409677625 ) ) ;
#25358=CARTESIAN_POINT ( 'NONE',  ( 0.000000000000000000, 0.000000000000000000, -200.0000000000000000 ) ) ;
#25360=CARTESIAN_POINT ( 'NONE',  ( 9.999999999999998224, 0.000000000000000000, -43.99999999999998579 ) ) ;
#25361=CARTESIAN_POINT ( 'NONE',  ( -10.81189881249999729, 1.324075727343319199E-15, -168.7812500020484094 ) ) ;
#25364=DIRECTION ( 'NONE',  ( -0.000000000000000000, -0.000000000000000000, 1.000000000000000000 ) ) ;
#25366=DIRECTION ( 'NONE',  ( 1.000000000000000000, 0.000000000000000000, 0.000000000000000000 ) ) ;
#25368=CARTESIAN_POINT ( 'NONE',  ( -9.999999999999998224, 1.224646799147353059E-15, -12.12500000409674783 ) ) ;
#25369=CARTESIAN_POINT ( 'NONE',  ( 9.999999999999998224, 0.000000000000000000, -27.49999999999996803 ) ) ;
#25370=CARTESIAN_POINT ( 'NONE',  ( 10.81189881249999729, 0.000000000000000000, -81.03125000204839523 ) ) ;
#25371=VERTEX_POINT ( 'NONE', #19493 ) ;
#25372=CARTESIAN_POINT ( 'NONE',  ( 9.999999999999998224, 0.000000000000000000, -140.0000000000000000 ) ) ;
#25375=CARTESIAN_POINT ( 'NONE',  ( -10.81189881249999729, 1.324075727343319199E-15, -30.59375000204836326 ) ) ;
#25376=CARTESIAN_POINT ( 'NONE',  ( -9.999999999999998224, 1.224646799147353059E-15, -76.62500000409677625 ) ) ;
#25377=CARTESIAN_POINT ( 'NONE',  ( 7.644554776091147741E-16, 12.48450537969573659, -2.656250002048344161 ) ) ;
#25378=CARTESIAN_POINT ( 'NONE',  ( 10.81189881249999551, -6.242252689847874514, -56.96875000204838102 ) ) ;
#25379=VERTEX_POINT ( 'NONE', #42155 ) ;
#25382=CARTESIAN_POINT ( 'NONE',  ( -5.405949406249996869, 9.363379034771805109, -189.8437500020483810 ) ) ;
#25383=CARTESIAN_POINT ( 'NONE',  ( 10.81189881249999907, 6.242252689847868297, -175.2187500020484094 ) ) ;
#25386=CARTESIAN_POINT ( 'NONE',  ( 10.00000000000154010, -5.773502691895370020, -24.62499999999995026 ) ) ;
#25388=CARTESIAN_POINT ( 'NONE',  ( 7.644554776091147741E-16, 12.48450537969573659, -104.4687500020483668 ) ) ;
#25389=CARTESIAN_POINT ( 'NONE',  ( 4.999999999999992006, -8.660254037844389075, -47.62500000409677625 ) ) ;
#25390=AXIS2_PLACEMENT_3D ( 'NONE', #17818, #15638, #22353 ) ;
#25391=CARTESIAN_POINT ( 'NONE',  ( 7.644554776091147741E-16, 12.48450537969573659, -74.65625000204838102 ) ) ;
#25392=ADVANCED_FACE ( 'NONE', ( #29649 ), #22964, .T. ) ;
#25393=CARTESIAN_POINT ( 'NONE',  ( 10.81189881249999729, 6.242252689847867408, -91.21875000204838102 ) ) ;
#25396=CARTESIAN_POINT ( 'NONE',  ( 9.999999999999996447, -5.773502691896262640, -149.5000000040968189 ) ) ;
#25398=ORIENTED_EDGE ( 'NONE', *, *, #30362, .T. ) ;
#25401=DIRECTION ( 'NONE',  ( -0.000000000000000000, -0.000000000000000000, 1.000000000000000000 ) ) ;
#25402=CARTESIAN_POINT ( 'NONE',  ( 9.999999999999998224, 0.000000000000000000, -200.0000000000000000 ) ) ;
#25405=CARTESIAN_POINT ( 'NONE',  ( 9.999999999999996447, -5.773502691896262640, -62.12499999999997868 ) ) ;
#25407=CARTESIAN_POINT ( 'NONE',  ( -5.000000000000003553, -8.660254037844383745, -73.37500000409677625 ) ) ;
#25411=CARTESIAN_POINT ( 'NONE',  ( -10.81189881249999729, -6.242252689847864744, -69.65625000204839523 ) ) ;
#25412=( BOUNDED_CURVE ( )  B_SPLINE_CURVE ( 2, ( #4640, #4856, #11524, #17787, #31410, #28386, #30984 ),
 .UNSPECIFIED., .F., .F. ) 
 B_SPLINE_CURVE_WITH_KNOTS ( ( 3, 2, 2, 3 ),
 ( 0.1343283582089551953, 0.1355721393034825528, 0.1368159203980099381, 0.1380597014925373234 ),
 .UNSPECIFIED. ) 
 CURVE ( )  GEOMETRIC_REPRESENTATION_ITEM ( )  RATIONAL_B_SPLINE_CURVE ( ( 1.000000000000003109, 0.8660254037844358210, 1.000000000000000000, 0.8660254037844387076, 1.000000000000000000, 0.8660254037844387076, 1.000000000000000000 ) ) 
 REPRESENTATION_ITEM ( '' )  );
#25414=CARTESIAN_POINT ( 'NONE',  ( -5.000000000000003553, -8.660254037844383745, -77.87500000409677625 ) ) ;
#25416=CARTESIAN_POINT ( 'NONE',  ( 0.000000000000000000, 0.000000000000000000, -200.0000000000000000 ) ) ;
#25417=CARTESIAN_POINT ( 'NONE',  ( -10.81189881249999907, -6.242252689847864744, -189.6562500020484094 ) ) ;
#25419=CARTESIAN_POINT ( 'NONE',  ( 7.644554776091147741E-16, 12.48450537969573659, -3.968750002048366810 ) ) ;
#25420=DIRECTION ( 'NONE',  ( 1.000000000000000000, 0.000000000000000000, 0.000000000000000000 ) ) ;
#25421=EDGE_CURVE ( 'NONE', #26946, #29087, #29017, .T. ) ;
#25422=CARTESIAN_POINT ( 'NONE',  ( -5.000000000000003553, -8.660254037844383745, -50.49999999999998579 ) ) ;
#25423=CARTESIAN_POINT ( 'NONE',  ( -9.999999999999998224, 1.224646799147353059E-15, -159.1250000040967905 ) ) ;
#25424=( BOUNDED_CURVE ( )  B_SPLINE_CURVE ( 2, ( #38510, #1852, #5504, #2284, #18653, #32263, #38730 ),
 .UNSPECIFIED., .F., .F. ) 
 B_SPLINE_CURVE_WITH_KNOTS ( ( 3, 2, 2, 3 ),
 ( 0.9552238805970153512, 0.9564676616915426255, 0.9577114427860698997, 0.9589552238805971740 ),
 .UNSPECIFIED. ) 
 CURVE ( )  GEOMETRIC_REPRESENTATION_ITEM ( )  RATIONAL_B_SPLINE_CURVE ( ( 0.9999999999999521494, 0.8660254037844865582, 1.000000000000000000, 0.8660254037844387076, 1.000000000000000000, 0.8660254037844267172, 1.000000000000011990 ) ) 
 REPRESENTATION_ITEM ( '' )  );
#25425=CARTESIAN_POINT ( 'NONE',  ( -5.000000000000003553, -8.660254037844383745, -173.5000000000000284 ) ) ;
#25426=CARTESIAN_POINT ( 'NONE',  ( -4.999999999999996447, 8.660254037844387298, -166.5000000000000000 ) ) ;
#25427=CARTESIAN_POINT ( 'NONE',  ( 5.405949406249992428, -9.363379034771808662, -105.2812500020483810 ) ) ;
#25428=ORIENTED_EDGE ( 'NONE', *, *, #14835, .F. ) ;
#25429=CYLINDRICAL_SURFACE ( 'NONE', #21411, 9.999999999999998224 ) ;
#25430=EDGE_CURVE ( 'NONE', #38098, #42101, #23763, .T. ) ;
#25432=ORIENTED_EDGE ( 'NONE', *, *, #6580, .F. ) ;
#25433=EDGE_LOOP ( 'NONE', ( #13896, #28615, #5782, #26420 ) ) ;
#25434=CARTESIAN_POINT ( 'NONE',  ( 10.81189881249999551, -6.242252689847874514, -28.65625000204838813 ) ) ;
#25436=CARTESIAN_POINT ( 'NONE',  ( 5.405949406249999534, 9.363379034771803333, -82.09375000204836681 ) ) ;
#25438=CARTESIAN_POINT ( 'NONE',  ( 10.81189881249999907, 6.242252689847868297, -197.7187500020484094 ) ) ;
#25439=CARTESIAN_POINT ( 'NONE',  ( -5.000000000000003553, -8.660254037844383745, -130.3750000040967905 ) ) ;
#25442=CARTESIAN_POINT ( 'NONE',  ( 5.000000000000000000, 8.660254037844385522, -9.625000004096746054 ) ) ;
#25444=CARTESIAN_POINT ( 'NONE',  ( 7.644554776091147741E-16, 12.48450537969573659, -128.4687500020483810 ) ) ;
#25445=ADVANCED_FACE ( 'NONE', ( #12796 ), #5719, .T. ) ;
#25446=CARTESIAN_POINT ( 'NONE',  ( -2.293366432827344421E-15, -12.48450537969573659, -115.7187500020483668 ) ) ;
#25449=CARTESIAN_POINT ( 'NONE',  ( -4.999999999999996447, 8.660254037844387298, -172.8750000040968189 ) ) ;
#25450=CARTESIAN_POINT ( 'NONE',  ( -10.81189881249999729, -6.242252689847864744, -171.6562500020484094 ) ) ;
#25451=EDGE_CURVE ( 'NONE', #37898, #19247, #26786, .T. ) ;
#25452=CARTESIAN_POINT ( 'NONE',  ( 9.999999999999994671, -5.773502691896262640, -133.0000000040967905 ) ) ;
#25455=CARTESIAN_POINT ( 'NONE',  ( 10.81189881249999551, -6.242252689847874514, -44.96875000204836681 ) ) ;
#25458=CARTESIAN_POINT ( 'NONE',  ( 10.81189881249999729, 0.000000000000000000, -0.03125000204837191653 ) ) ;
#25462=CARTESIAN_POINT ( 'NONE',  ( -2.121150477449813534E-15, -11.54700538379251284, -89.37499999999997158 ) ) ;
#25464=CARTESIAN_POINT ( 'NONE',  ( -5.000000000000003553, -8.660254037844383745, -98.87500000409677625 ) ) ;
#25465=AXIS2_PLACEMENT_3D ( 'NONE', #2507, #15213, #35095 ) ;
#25466=CYLINDRICAL_SURFACE ( 'NONE', #30004, 9.999999999999998224 ) ;
#25468=CARTESIAN_POINT ( 'NONE',  ( 10.81189881249999729, 0.000000000000000000, -91.53125000204838102 ) ) ;
#25471=CARTESIAN_POINT ( 'NONE',  ( 9.999999999999998224, 0.000000000000000000, -200.0000000000000000 ) ) ;
#25472=CARTESIAN_POINT ( 'NONE',  ( 5.405949406249999534, 9.363379034771803333, -158.7812500020484094 ) ) ;
#25474=ORIENTED_EDGE ( 'NONE', *, *, #26996, .F. ) ;
#25475=CARTESIAN_POINT ( 'NONE',  ( 5.000000000000000000, 8.660254037844385522, -13.74999999999995737 ) ) ;
#25476=CARTESIAN_POINT ( 'NONE',  ( 10.81189881249999551, -6.242252689847874514, -24.15625000204838102 ) ) ;
#25477=CARTESIAN_POINT ( 'NONE',  ( 9.999999999999998224, 0.000000000000000000, -150.5000000000000000 ) ) ;
#25479=EDGE_CURVE ( 'NONE', #5730, #28672, #35364, .T. ) ;
#25480=CARTESIAN_POINT ( 'NONE',  ( 7.070501591499377789E-16, 11.54700538379251284, -199.6250000000000000 ) ) ;
#25481=CARTESIAN_POINT ( 'NONE',  ( -10.81189881249999729, 6.242252689847871849, -128.4062500020484094 ) ) ;
#25483=CARTESIAN_POINT ( 'NONE',  ( 9.999999999999998224, 0.000000000000000000, -117.8750000040967905 ) ) ;
#25484=VERTEX_POINT ( 'NONE', #17093 ) ;
#25485=CARTESIAN_POINT ( 'NONE',  ( 10.81189881249999551, -6.242252689847874514, -54.15625000204837391 ) ) ;
#25487=CARTESIAN_POINT ( 'NONE',  ( -5.405949406249996869, 9.363379034771805109, -101.3437500020483810 ) ) ;
#25489=EDGE_LOOP ( 'NONE', ( #16784, #33648, #19932, #20237 ) ) ;
#25491=CARTESIAN_POINT ( 'NONE',  ( -9.999999999999998224, 1.224646799147353059E-15, -200.0000000000000000 ) ) ;
#25493=CARTESIAN_POINT ( 'NONE',  ( 7.644554776091147741E-16, 12.48450537969573659, -156.9687500020484094 ) ) ;
#25495=CARTESIAN_POINT ( 'NONE',  ( 7.644554776091147741E-16, 12.48450537969573659, -3.968750002048366810 ) ) ;
#25496=FACE_OUTER_BOUND ( 'NONE', #29378, .T. ) ;
#25497=CARTESIAN_POINT ( 'NONE',  ( -10.81189881249999729, -6.242252689847864744, -141.4687500020483810 ) ) ;
#25501=CARTESIAN_POINT ( 'NONE',  ( -2.121150477449813534E-15, -11.54700538379251284, -196.2500000040967905 ) ) ;
#25503=CARTESIAN_POINT ( 'NONE',  ( 10.81189881249999729, 0.000000000000000000, -195.0312500020484094 ) ) ;
#25504=VECTOR ( 'NONE', #36528, 1000.000000000000000 ) ;
#25505=CYLINDRICAL_SURFACE ( 'NONE', #28212, 9.999999999999998224 ) ;
#25508=CARTESIAN_POINT ( 'NONE',  ( 7.644554776091147741E-16, 12.48450537969573659, -71.46875000204836681 ) ) ;
#25509=CARTESIAN_POINT ( 'NONE',  ( -10.81189881249999729, 6.242252689847871849, -56.21875000204837391 ) ) ;
#25511=CARTESIAN_POINT ( 'NONE',  ( 10.81189881249999729, 0.000000000000000000, -28.53125000204837036 ) ) ;
#25515=CARTESIAN_POINT ( 'NONE',  ( 4.999999999999992006, -8.660254037844389075, -113.2499999999999858 ) ) ;
#25519=CARTESIAN_POINT ( 'NONE',  ( 10.81189881249999729, 6.242252689847867408, -10.40625000204838102 ) ) ;
#25520=EDGE_LOOP ( 'NONE', ( #2530, #34722, #12288, #32692 ) ) ;
#25523=CARTESIAN_POINT ( 'NONE',  ( -5.000000000000003553, -8.660254037844383745, -38.87500000409676915 ) ) ;
#25525=CARTESIAN_POINT ( 'NONE',  ( 9.999999999999996447, -5.773502691896262640, -41.12499999999997158 ) ) ;
#25527=CARTESIAN_POINT ( 'NONE',  ( -2.121150477449813534E-15, -11.54700538379251284, -22.25000000409676915 ) ) ;
#25528=CARTESIAN_POINT ( 'NONE',  ( 5.405949406249992428, -9.363379034771808662, -51.28125000204835970 ) ) ;
#25529=CARTESIAN_POINT ( 'NONE',  ( -9.999999999999998224, 1.224646799147353059E-15, -22.62500000409675849 ) ) ;
#25531=CARTESIAN_POINT ( 'NONE',  ( -9.999999999999479527, -5.773502691896549521, -106.1249999999999716 ) ) ;
#25532=CARTESIAN_POINT ( 'NONE',  ( 7.644554776091147741E-16, 12.48450537969573659, -146.6562500020484379 ) ) ;
#25533=CARTESIAN_POINT ( 'NONE',  ( 7.644554776091147741E-16, 12.48450537969573659, -148.1562500020484094 ) ) ;
#25534=CYLINDRICAL_SURFACE ( 'NONE', #8271, 9.999999999999998224 ) ;
#25536=ORIENTED_EDGE ( 'NONE', *, *, #35256, .T. ) ;
#25538=VERTEX_POINT ( 'NONE', #23808 ) ;
#25539=VERTEX_POINT ( 'NONE', #33741 ) ;
#25541=CARTESIAN_POINT ( 'NONE',  ( -10.81189881249999729, 1.324075727343319199E-15, -185.0937500020483810 ) ) ;
#25542=CARTESIAN_POINT ( 'NONE',  ( -2.293366432827344421E-15, -12.48450537969573659, -34.71875000204835260 ) ) ;
#25544=CARTESIAN_POINT ( 'NONE',  ( 5.405949406249992428, -9.363379034771808662, -165.0937500020484094 ) ) ;
#25545=CARTESIAN_POINT ( 'NONE',  ( 7.644554776091147741E-16, 12.48450537969573659, -155.4687500020484094 ) ) ;
#25546=DIRECTION ( 'NONE',  ( -0.000000000000000000, -0.000000000000000000, 1.000000000000000000 ) ) ;
#25549=CARTESIAN_POINT ( 'NONE',  ( -5.405949406250003975, -9.363379034771801557, -19.84375000204835615 ) ) ;
#25551=CARTESIAN_POINT ( 'NONE',  ( -10.00000000000154188, 5.773502691895366468, -10.75000000409672118 ) ) ;
#25553=VECTOR ( 'NONE', #33174, 1000.000000000000000 ) ;
#25554=CARTESIAN_POINT ( 'NONE',  ( 10.81189881249999551, -6.242252689847874514, -83.96875000204838102 ) ) ;
#25555=CARTESIAN_POINT ( 'NONE',  ( 9.999999999999998224, 0.000000000000000000, -200.0000000000000000 ) ) ;
#25556=CARTESIAN_POINT ( 'NONE',  ( -5.405949406249996869, 9.363379034771805109, -53.53125000204836681 ) ) ;
#25559=AXIS2_PLACEMENT_3D ( 'NONE', #2282, #2064, #38089 ) ;
#25560=CARTESIAN_POINT ( 'NONE',  ( -5.000000000000003553, -8.660254037844383745, -136.0000000000000000 ) ) ;
#25561=CARTESIAN_POINT ( 'NONE',  ( 5.405949406249992428, -9.363379034771808662, -144.2812500020483810 ) ) ;
#25562=CARTESIAN_POINT ( 'NONE',  ( 9.999999999999998224, 0.000000000000000000, -15.87500000409675138 ) ) ;
#25564=CARTESIAN_POINT ( 'NONE',  ( -4.999999999999996447, 8.660254037844387298, -124.8750000040967763 ) ) ;
#25569=CARTESIAN_POINT ( 'NONE',  ( 4.999999999999992006, -8.660254037844389075, -22.12500000409675494 ) ) ;
#25570=CARTESIAN_POINT ( 'NONE',  ( 10.81189881249999551, -6.242252689847874514, -169.6562500020484094 ) ) ;
#25571=CARTESIAN_POINT ( 'NONE',  ( 9.999999999999998224, 0.000000000000000000, -51.87500000409675494 ) ) ;
#25574=CARTESIAN_POINT ( 'NONE',  ( 5.405949406249992428, -9.363379034771808662, -172.7812500020484094 ) ) ;
#25575=CARTESIAN_POINT ( 'NONE',  ( -9.999999999999998224, 1.224646799147353059E-15, -82.24999999999998579 ) ) ;
#25576=DIRECTION ( 'NONE',  ( -0.000000000000000000, -0.000000000000000000, 1.000000000000000000 ) ) ;
#25578=ORIENTED_EDGE ( 'NONE', *, *, #39156, .F. ) ;
#25580=DIRECTION ( 'NONE',  ( 1.000000000000000000, 0.000000000000000000, 0.000000000000000000 ) ) ;
#25582=CARTESIAN_POINT ( 'NONE',  ( -10.81189881249999729, 1.324075727343319199E-15, -74.28125000204838102 ) ) ;
#25585=ORIENTED_EDGE ( 'NONE', *, *, #23826, .F. ) ;
#25586=ORIENTED_EDGE ( 'NONE', *, *, #22769, .F. ) ;
#25587=CARTESIAN_POINT ( 'NONE',  ( 10.81189881249999729, 0.000000000000000000, -29.84375000204836326 ) ) ;
#25588=CARTESIAN_POINT ( 'NONE',  ( -10.81189881249999729, 6.242252689847871849, -8.406250002048372139 ) ) ;
#25589=CARTESIAN_POINT ( 'NONE',  ( 7.644554776091147741E-16, 12.48450537969573659, -56.46875000204837391 ) ) ;
#25590=ORIENTED_EDGE ( 'NONE', *, *, #3279, .F. ) ;
#25591=CARTESIAN_POINT ( 'NONE',  ( -9.999999999999998224, 1.224646799147353059E-15, -179.7500000000000284 ) ) ;
#25593=CARTESIAN_POINT ( 'NONE',  ( 5.405949406249992428, -9.363379034771808662, -186.0937500020483810 ) ) ;
#25594=CARTESIAN_POINT ( 'NONE',  ( -10.81189881249999907, -6.242252689847864744, -175.9687500020483526 ) ) ;
#25597=CARTESIAN_POINT ( 'NONE',  ( 9.999999999999479527, 5.773502691896553074, -41.25000000409674783 ) ) ;
#25598=CARTESIAN_POINT ( 'NONE',  ( 10.00000000000015632, -5.773502691896169381, -191.5000000040968757 ) ) ;
#25600=CARTESIAN_POINT ( 'NONE',  ( 5.405949406249999534, 9.363379034771803333, -106.0937500020483810 ) ) ;
#25602=CARTESIAN_POINT ( 'NONE',  ( 5.405949406249999534, 9.363379034771803333, -73.28125000204838102 ) ) ;
#25603=CARTESIAN_POINT ( 'NONE',  ( 5.405949406249992428, -9.363379034771808662, -88.59375000204838102 ) ) ;
#25605=CARTESIAN_POINT ( 'NONE',  ( -5.000000000000003553, -8.660254037844383745, -145.3750000040967905 ) ) ;
#25607=ORIENTED_EDGE ( 'NONE', *, *, #32743, .F. ) ;
#25611=CARTESIAN_POINT ( 'NONE',  ( 10.81189881249999907, 6.242252689847868297, -194.9062500020484379 ) ) ;
#25614=VERTEX_POINT ( 'NONE', #17519 ) ;
#25615=CARTESIAN_POINT ( 'NONE',  ( 4.999999999999992006, -8.660254037844389075, -65.24999999999997158 ) ) ;
#25617=CARTESIAN_POINT ( 'NONE',  ( 9.999999999999998224, 0.000000000000000000, -77.37500000409677625 ) ) ;
#25618=CARTESIAN_POINT ( 'NONE',  ( 9.999999999999998224, 0.000000000000000000, -66.49999999999997158 ) ) ;
#25619=( BOUNDED_CURVE ( )  B_SPLINE_CURVE ( 2, ( #19035, #25531, #5881, #25105, #34816, #38680, #32009 ),
 .UNSPECIFIED., .F., .F. ) 
 B_SPLINE_CURVE_WITH_KNOTS ( ( 3, 2, 2, 3 ),
 ( 0.4664179104477613191, 0.4676616915422886489, 0.4689054726368160342, 0.4701492537313434195 ),
 .UNSPECIFIED. ) 
 CURVE ( )  GEOMETRIC_REPRESENTATION_ITEM ( )  RATIONAL_B_SPLINE_CURVE ( ( 0.9999999999999880096, 0.8660254037844506980, 1.000000000000000000, 0.8660254037844387076, 1.000000000000000000, 0.8660254037844267172, 1.000000000000011990 ) ) 
 REPRESENTATION_ITEM ( '' )  );
#25620=DIRECTION ( 'NONE',  ( 0.000000000000000000, 0.08715574274765837404, -0.9961946980917455452 ) ) ;
#25622=CARTESIAN_POINT ( 'NONE',  ( -5.405949406249996869, 9.363379034771805109, -64.03125000204836681 ) ) ;
#25624=CARTESIAN_POINT ( 'NONE',  ( 10.00000000000051159, -5.773502691895965988, -77.50000000409677625 ) ) ;
#25626=CARTESIAN_POINT ( 'NONE',  ( 9.999999999999998224, 0.000000000000000000, -33.87500000409676915 ) ) ;
#25627=CARTESIAN_POINT ( 'NONE',  ( 5.405949406249999534, 9.363379034771803333, -191.7812500020484094 ) ) ;
#25629=CARTESIAN_POINT ( 'NONE',  ( -5.405949406250003975, -9.363379034771801557, -4.843750002048369474 ) ) ;
#25630=CARTESIAN_POINT ( 'NONE',  ( 7.070501591499376803E-16, 11.54700538379251284, -140.0000000040967905 ) ) ;
#25632=CARTESIAN_POINT ( 'NONE',  ( -9.999999999999998224, 1.224646799147353059E-15, -125.7499999999999716 ) ) ;
#25633=CARTESIAN_POINT ( 'NONE',  ( -9.999999999999998224, 1.224646799147353059E-15, -172.2500000000000000 ) ) ;
#25634=CARTESIAN_POINT ( 'NONE',  ( 10.81189881249999907, 6.242252689847868297, -98.90625000204839523 ) ) ;
#25635=VERTEX_POINT ( 'NONE', #10621 ) ;
#25636=CARTESIAN_POINT ( 'NONE',  ( 9.999999999999998224, 0.000000000000000000, -37.99999999999997868 ) ) ;
#25637=EDGE_CURVE ( 'NONE', #19402, #24501, #7405, .T. ) ;
#25639=ADVANCED_FACE ( 'NONE', ( #14270 ), #9988, .T. ) ;
#25642=CARTESIAN_POINT ( 'NONE',  ( -10.81189881249999729, 6.242252689847871849, -26.40625000204837747 ) ) ;
#25643=CARTESIAN_POINT ( 'NONE',  ( 10.81189881249999907, 6.242252689847868297, -80.71875000204838102 ) ) ;
#25644=CARTESIAN_POINT ( 'NONE',  ( -4.999999999999996447, 8.660254037844387298, -126.0000000000000000 ) ) ;
#25646=CARTESIAN_POINT ( 'NONE',  ( -2.121150477449813534E-15, -11.54700538379251284, -130.2500000040967905 ) ) ;
#25647=CARTESIAN_POINT ( 'NONE',  ( -9.999999999999998224, 1.224646799147353059E-15, -200.0000000000000000 ) ) ;
#25649=CARTESIAN_POINT ( 'NONE',  ( -10.00000000000000000, -5.773502691896251982, -7.500000004096747830 ) ) ;
#25651=CARTESIAN_POINT ( 'NONE',  ( -9.999999999999479527, -5.773502691896549521, -77.62499999999995737 ) ) ;
#25652=CARTESIAN_POINT ( 'NONE',  ( 7.644554776091147741E-16, 12.48450537969573659, -131.4687500020483810 ) ) ;
#25653=CARTESIAN_POINT ( 'NONE',  ( -5.405949406250003975, -9.363379034771801557, -114.3437500020483810 ) ) ;
#25656=CARTESIAN_POINT ( 'NONE',  ( -9.999999999999998224, 5.773502691896259087, -166.7500000040967905 ) ) ;
#25657=( BOUNDED_CURVE ( )  B_SPLINE_CURVE ( 2, ( #3140, #35939, #18681, #12828, #12199, #22356, #2517 ),
 .UNSPECIFIED., .F., .F. ) 
 B_SPLINE_CURVE_WITH_KNOTS ( ( 3, 2, 2, 3 ),
 ( 0.5708955223880599616, 0.5721393034825872359, 0.5733830845771146212, 0.5746268656716420065 ),
 .UNSPECIFIED. ) 
 CURVE ( )  GEOMETRIC_REPRESENTATION_ITEM ( )  RATIONAL_B_SPLINE_CURVE ( ( 0.9999999999999761302, 0.8660254037844625774, 1.000000000000000000, 0.8660254037844387076, 1.000000000000000000, 0.8660254037844148378, 1.000000000000023981 ) ) 
 REPRESENTATION_ITEM ( '' )  );
#25658=CARTESIAN_POINT ( 'NONE',  ( -10.00000000000051337, 5.773502691895962435, -81.25000000409677625 ) ) ;
#25661=CARTESIAN_POINT ( 'NONE',  ( -2.293366432827344421E-15, -12.48450537969573659, -45.21875000204837391 ) ) ;
#25663=CARTESIAN_POINT ( 'NONE',  ( -10.81189881249999729, 1.324075727343319199E-15, -0.7812500020483725827 ) ) ;
#25665=CARTESIAN_POINT ( 'NONE',  ( 10.00000000000102318, -5.773502691895667560, -59.50000000409674072 ) ) ;
#25667=CARTESIAN_POINT ( 'NONE',  ( 9.999999999999998224, 0.000000000000000000, -91.99999999999998579 ) ) ;
#25669=CARTESIAN_POINT ( 'NONE',  ( -4.999999999999996447, 8.660254037844387298, -94.87500000409677625 ) ) ;
#25672=CARTESIAN_POINT ( 'NONE',  ( 10.81189881249999729, 0.000000000000000000, -90.03125000204838102 ) ) ;
#25673=EDGE_LOOP ( 'NONE', ( #29904, #27160, #16987, #29661 ) ) ;
#25675=( BOUNDED_CURVE ( )  B_SPLINE_CURVE ( 2, ( #23164, #16446, #7184, #3953, #936, #19912, #10832 ),
 .UNSPECIFIED., .F., .F. ) 
 B_SPLINE_CURVE_WITH_KNOTS ( ( 3, 2, 2, 3 ),
 ( 0.7985074626865673597, 0.7997512437810947450, 0.8009950248756220192, 0.8022388059701494045 ),
 .UNSPECIFIED. ) 
 CURVE ( )  GEOMETRIC_REPRESENTATION_ITEM ( )  RATIONAL_B_SPLINE_CURVE ( ( 0.9999999999999761302, 0.8660254037844625774, 1.000000000000000000, 0.8660254037844387076, 1.000000000000000000, 0.8660254037844267172, 1.000000000000011990 ) ) 
 REPRESENTATION_ITEM ( '' )  );
#25677=DIRECTION ( 'NONE',  ( 1.000000000000000000, 0.000000000000000000, 0.000000000000000000 ) ) ;
#25679=ORIENTED_EDGE ( 'NONE', *, *, #34402, .F. ) ;
#25680=CARTESIAN_POINT ( 'NONE',  ( 7.070501591499377789E-16, 11.54700538379251284, -16.62499999999996447 ) ) ;
#25681=CARTESIAN_POINT ( 'NONE',  ( 5.405949406249999534, 9.363379034771803333, -22.28125000204836326 ) ) ;
#25682=CARTESIAN_POINT ( 'NONE',  ( -9.999999999999998224, 1.224646799147353059E-15, -149.7500000000000000 ) ) ;
#25685=CARTESIAN_POINT ( 'NONE',  ( 9.999999999999998224, 0.000000000000000000, -195.5000000000000000 ) ) ;
#25686=CARTESIAN_POINT ( 'NONE',  ( 7.644554776091147741E-16, 12.48450537969573659, -127.1562500020483952 ) ) ;
#25687=VERTEX_POINT ( 'NONE', #6761 ) ;
#25689=EDGE_CURVE ( 'NONE', #6874, #25274, #34235, .T. ) ;
#25690=EDGE_CURVE ( 'NONE', #37716, #12293, #10412, .T. ) ;
#25691=VERTEX_POINT ( 'NONE', #40191 ) ;
#25692=ADVANCED_FACE ( 'NONE', ( #40390 ), #3529, .T. ) ;
#25693=CARTESIAN_POINT ( 'NONE',  ( -10.81189881249999907, -6.242252689847864744, -53.15625000204837391 ) ) ;
#25695=CARTESIAN_POINT ( 'NONE',  ( -10.81189881249999729, 1.324075727343319199E-15, -101.0937500020483810 ) ) ;
#25696=VERTEX_POINT ( 'NONE', #7616 ) ;
#25697=ORIENTED_EDGE ( 'NONE', *, *, #37512, .F. ) ;
#25700=CARTESIAN_POINT ( 'NONE',  ( 9.999999999999998224, 0.000000000000000000, -119.0000000000000000 ) ) ;
#25701=CARTESIAN_POINT ( 'NONE',  ( 10.81189881249999729, 0.000000000000000000, -151.3437500020483810 ) ) ;
#25703=CARTESIAN_POINT ( 'NONE',  ( -10.81189881249999729, 1.324075727343319199E-15, -9.593750002048345493 ) ) ;
#25704=DIRECTION ( 'NONE',  ( 1.000000000000000000, 0.000000000000000000, 0.000000000000000000 ) ) ;
#25705=CARTESIAN_POINT ( 'NONE',  ( 10.81189881249999729, 6.242252689847867408, -143.7187500020484094 ) ) ;
#25707=CARTESIAN_POINT ( 'NONE',  ( -5.000000000000003553, -8.660254037844383745, -148.0000000000000000 ) ) ;
#25709=CARTESIAN_POINT ( 'NONE',  ( -2.121150477449813534E-15, -11.54700538379251284, -194.7500000040967905 ) ) ;
#25711=CARTESIAN_POINT ( 'NONE',  ( 5.405949406249992428, -9.363379034771808662, -186.2812500020484094 ) ) ;
#25712=CARTESIAN_POINT ( 'NONE',  ( 4.999999999999992006, -8.660254037844389075, -47.24999999999998579 ) ) ;
#25716=CARTESIAN_POINT ( 'NONE',  ( -5.405949406249996869, 9.363379034771805109, -66.84375000204836681 ) ) ;
#25717=CARTESIAN_POINT ( 'NONE',  ( -5.405949406250003975, -9.363379034771801557, -45.34375000204838102 ) ) ;
#25719=CARTESIAN_POINT ( 'NONE',  ( -5.405949406249996869, 9.363379034771805109, -23.53125000204836681 ) ) ;
#25723=CARTESIAN_POINT ( 'NONE',  ( 7.070501591499377789E-16, 11.54700538379251284, -111.1249999999999716 ) ) ;
#25724=LINE ( 'NONE', #12111, #3818 ) ;
#25727=CARTESIAN_POINT ( 'NONE',  ( -10.81189881249999729, 6.242252689847871849, -119.4062500020483952 ) ) ;
#25728=ORIENTED_EDGE ( 'NONE', *, *, #30976, .F. ) ;
#25729=CARTESIAN_POINT ( 'NONE',  ( -9.999999999999998224, 1.224646799147353059E-15, -104.7499999999999858 ) ) ;
#25733=CARTESIAN_POINT ( 'NONE',  ( 9.999999999999996447, -5.773502691896262640, -38.12499999999995737 ) ) ;
#25734=CARTESIAN_POINT ( 'NONE',  ( -2.121150477449813534E-15, -11.54700538379251284, -29.75000000409675849 ) ) ;
#25735=CARTESIAN_POINT ( 'NONE',  ( -10.81189881249999729, -6.242252689847864744, -44.15625000204838102 ) ) ;
#25736=EDGE_CURVE ( 'NONE', #2293, #17414, #28181, .T. ) ;
#25737=CARTESIAN_POINT ( 'NONE',  ( 10.00000000000051159, -5.773502691895965988, -141.6250000000000000 ) ) ;
#25739=CARTESIAN_POINT ( 'NONE',  ( 9.999999999999998224, 0.000000000000000000, -185.0000000000000000 ) ) ;
#25740=CARTESIAN_POINT ( 'NONE',  ( 5.405949406249992428, -9.363379034771808662, -133.7812500020483810 ) ) ;
#25741=CARTESIAN_POINT ( 'NONE',  ( -10.81189881249999907, -6.242252689847864744, -153.6562500020484094 ) ) ;
#25743=( BOUNDED_CURVE ( )  B_SPLINE_CURVE ( 2, ( #25126, #35266, #5261, #32239, #32031, #18413, #15590 ),
 .UNSPECIFIED., .F., .F. ) 
 B_SPLINE_CURVE_WITH_KNOTS ( ( 3, 2, 2, 3 ),
 ( 0.2089552238805970630, 0.2101990049751244205, 0.2114427860696518058, 0.2126865671641791633 ),
 .UNSPECIFIED. ) 
 CURVE ( )  GEOMETRIC_REPRESENTATION_ITEM ( )  RATIONAL_B_SPLINE_CURVE ( ( 0.9999999999999940048, 0.8660254037844447028, 1.000000000000000000, 0.8660254037844387076, 1.000000000000000000, 0.8660254037844327124, 1.000000000000005995 ) ) 
 REPRESENTATION_ITEM ( '' )  );
#25745=ORIENTED_EDGE ( 'NONE', *, *, #4288, .T. ) ;
#25747=ORIENTED_EDGE ( 'NONE', *, *, #18589, .T. ) ;
#25749=CARTESIAN_POINT ( 'NONE',  ( 7.644554776091147741E-16, 12.48450537969573659, -180.9687500020484094 ) ) ;
#25750=CARTESIAN_POINT ( 'NONE',  ( 5.405949406249992428, -9.363379034771808662, -34.59375000204836681 ) ) ;
#25751=ADVANCED_FACE ( 'NONE', ( #16878 ), #36538, .T. ) ;
#25752=LINE ( 'NONE', #38905, #4675 ) ;
#25753=CARTESIAN_POINT ( 'NONE',  ( -5.405949406250003975, -9.363379034771801557, -163.8437500020484094 ) ) ;
#25754=CARTESIAN_POINT ( 'NONE',  ( -5.405949406250003975, -9.363379034771801557, -144.3437500020483810 ) ) ;
#25755=CARTESIAN_POINT ( 'NONE',  ( 9.999999999999998224, 0.000000000000000000, -131.0000000000000000 ) ) ;
#25758=CARTESIAN_POINT ( 'NONE',  ( -5.405949406250003975, -9.363379034771801557, -18.34375000204835260 ) ) ;
#25760=DIRECTION ( 'NONE',  ( 1.000000000000000000, 0.000000000000000000, 0.000000000000000000 ) ) ;
#25763=CARTESIAN_POINT ( 'NONE',  ( 5.405949406249999534, 9.363379034771803333, -80.59375000204838102 ) ) ;
#25764=CARTESIAN_POINT ( 'NONE',  ( -2.293366432827344421E-15, -12.48450537969573659, -51.40625000204838102 ) ) ;
#25768=CARTESIAN_POINT ( 'NONE',  ( 9.999999999999998224, 0.000000000000000000, -137.0000000000000000 ) ) ;
#25769=CARTESIAN_POINT ( 'NONE',  ( 10.81189881249999729, 0.000000000000000000, -144.0312500020483810 ) ) ;
#25771=CARTESIAN_POINT ( 'NONE',  ( 10.00000000000000000, 5.773502691896255534, -122.2500000040968047 ) ) ;
#25773=ORIENTED_EDGE ( 'NONE', *, *, #2979, .T. ) ;
#25777=CARTESIAN_POINT ( 'NONE',  ( 7.644554776091147741E-16, 12.48450537969573659, -169.1562500020484094 ) ) ;
#25778=CARTESIAN_POINT ( 'NONE',  ( -2.121150477449813534E-15, -11.54700538379251284, -53.75000000409677625 ) ) ;
#25781=( BOUNDED_CURVE ( )  B_SPLINE_CURVE ( 2, ( #20897, #30045, #11602, #8180, #1925, #34299, #17646 ),
 .UNSPECIFIED., .F., .F. ) 
 B_SPLINE_CURVE_WITH_KNOTS ( ( 3, 2, 2, 3 ),
 ( 0.8246268656716420065, 0.8258706467661693917, 0.8271144278606967770, 0.8283582089552240513 ),
 .UNSPECIFIED. ) 
 CURVE ( )  GEOMETRIC_REPRESENTATION_ITEM ( )  RATIONAL_B_SPLINE_CURVE ( ( 0.9999999999999761302, 0.8660254037844625774, 1.000000000000000000, 0.8660254037844387076, 1.000000000000000000, 0.8660254037844148378, 1.000000000000023981 ) ) 
 REPRESENTATION_ITEM ( '' )  );
#25782=FACE_OUTER_BOUND ( 'NONE', #14215, .T. ) ;
#25783=CARTESIAN_POINT ( 'NONE',  ( 5.405949406249999534, 9.363379034771803333, -169.2812500020484094 ) ) ;
#25784=ORIENTED_EDGE ( 'NONE', *, *, #31748, .T. ) ;
#25785=FACE_OUTER_BOUND ( 'NONE', #2075, .T. ) ;
#25787=CARTESIAN_POINT ( 'NONE',  ( 10.81189881249999551, -6.242252689847874514, -69.15625000204839523 ) ) ;
#25790=CARTESIAN_POINT ( 'NONE',  ( -5.000000000000003553, -8.660254037844383745, -143.5000000000000000 ) ) ;
#25793=CARTESIAN_POINT ( 'NONE',  ( 10.81189881249999551, -6.242252689847874514, -31.46875000204835260 ) ) ;
#25795=CARTESIAN_POINT ( 'NONE',  ( -5.405949406250003975, -9.363379034771801557, -5.031250002048376579 ) ) ;
#25796=CARTESIAN_POINT ( 'NONE',  ( -10.81189881249999729, 6.242252689847871849, -51.71875000204836681 ) ) ;
#25798=CYLINDRICAL_SURFACE ( 'NONE', #3386, 9.999999999999998224 ) ;
#25800=CARTESIAN_POINT ( 'NONE',  ( 10.81189881249999729, 0.000000000000000000, -188.8437500020483810 ) ) ;
#25801=CARTESIAN_POINT ( 'NONE',  ( 10.81189881249999729, 0.000000000000000000, -167.8437500020484094 ) ) ;
#25804=CARTESIAN_POINT ( 'NONE',  ( -9.999999999999998224, 1.224646799147353059E-15, -124.2500000000000000 ) ) ;
#25805=CARTESIAN_POINT ( 'NONE',  ( 4.999999999999992006, -8.660254037844389075, -24.74999999999996803 ) ) ;
#25807=CARTESIAN_POINT ( 'NONE',  ( -10.81189881249999729, 6.242252689847871849, -108.7187500020483810 ) ) ;
#25808=CARTESIAN_POINT ( 'NONE',  ( -4.999999999999996447, 8.660254037844387298, -196.5000000000000000 ) ) ;
#25809=CARTESIAN_POINT ( 'NONE',  ( 10.81189881249999729, 0.000000000000000000, -76.53125000204838102 ) ) ;
#25810=CARTESIAN_POINT ( 'NONE',  ( 9.999999999999998224, 0.000000000000000000, -131.3750000040967905 ) ) ;
#25811=CARTESIAN_POINT ( 'NONE',  ( 7.644554776091147741E-16, 12.48450537969573659, -87.96875000204838102 ) ) ;
#25813=CARTESIAN_POINT ( 'NONE',  ( -9.999999999999998224, 1.224646799147353059E-15, -145.6250000040967905 ) ) ;
#25815=EDGE_CURVE ( 'NONE', #39684, #26894, #38632, .T. ) ;
#25816=ORIENTED_EDGE ( 'NONE', *, *, #30940, .F. ) ;
#25819=CARTESIAN_POINT ( 'NONE',  ( 10.81189881249999551, -6.242252689847874514, -193.6562500020484379 ) ) ;
#25822=ORIENTED_EDGE ( 'NONE', *, *, #40984, .T. ) ;
#25823=CARTESIAN_POINT ( 'NONE',  ( 4.999999999999992006, -8.660254037844389075, -68.24999999999997158 ) ) ;
#25825=CARTESIAN_POINT ( 'NONE',  ( 10.00000000000000000, 5.773502691896255534, -71.25000000409676204 ) ) ;
#25826=DIRECTION ( 'NONE',  ( -0.000000000000000000, -0.000000000000000000, 1.000000000000000000 ) ) ;
#25827=CYLINDRICAL_SURFACE ( 'NONE', #35551, 9.999999999999998224 ) ;
#25829=CARTESIAN_POINT ( 'NONE',  ( -2.293366432827344421E-15, -12.48450537969573659, -67.90625000204840944 ) ) ;
#25832=VERTEX_POINT ( 'NONE', #11908 ) ;
#25833=CARTESIAN_POINT ( 'NONE',  ( -10.81189881249999907, -6.242252689847864744, -197.1562500020484379 ) ) ;
#25835=CARTESIAN_POINT ( 'NONE',  ( 5.405949406249992428, -9.363379034771808662, -6.093750002048370362 ) ) ;
#25836=CARTESIAN_POINT ( 'NONE',  ( 4.999999999999992006, -8.660254037844389075, -110.6250000040967763 ) ) ;
#25838=CARTESIAN_POINT ( 'NONE',  ( -5.000000000000003553, -8.660254037844383745, -112.3750000040967763 ) ) ;
#25839=CARTESIAN_POINT ( 'NONE',  ( -9.999999999999998224, 1.224646799147353059E-15, -176.7500000000000284 ) ) ;
#25840=CARTESIAN_POINT ( 'NONE',  ( -10.00000000000000000, -5.773502691896252870, -169.5000000040967905 ) ) ;
#25841=CARTESIAN_POINT ( 'NONE',  ( -10.81189881249999729, 6.242252689847871849, -99.90625000204838102 ) ) ;
#25844=LINE ( 'NONE', #12863, #35895 ) ;
#25845=ORIENTED_EDGE ( 'NONE', *, *, #30964, .F. ) ;
#25848=CARTESIAN_POINT ( 'NONE',  ( -5.405949406249996869, 9.363379034771805109, -35.34375000204836681 ) ) ;
#25850=CARTESIAN_POINT ( 'NONE',  ( -10.81189881249999729, 6.242252689847871849, -27.90625000204838102 ) ) ;
#25852=CARTESIAN_POINT ( 'NONE',  ( -10.81189881249999729, 1.324075727343319199E-15, -77.09375000204838102 ) ) ;
#25855=CARTESIAN_POINT ( 'NONE',  ( -10.00000000000051337, 5.773502691895962435, -69.25000000409677625 ) ) ;
#25858=CARTESIAN_POINT ( 'NONE',  ( -10.00000000000000000, -5.773502691896251982, -15.00000000409676737 ) ) ;
#25859=CARTESIAN_POINT ( 'NONE',  ( -9.999999999999998224, 1.224646799147353059E-15, -80.74999999999998579 ) ) ;
#25860=CARTESIAN_POINT ( 'NONE',  ( -5.405949406250003975, -9.363379034771801557, -126.3437500020483952 ) ) ;
#25861=CARTESIAN_POINT ( 'NONE',  ( -10.81189881249999729, 1.324075727343319199E-15, -98.28125000204839523 ) ) ;
#25862=CARTESIAN_POINT ( 'NONE',  ( 5.405949406249999534, 9.363379034771803333, -112.0937500020483810 ) ) ;
#25866=CARTESIAN_POINT ( 'NONE',  ( -10.00000000000000000, -5.773502691896251982, -166.5000000040967905 ) ) ;
#25867=CARTESIAN_POINT ( 'NONE',  ( -4.999999999999996447, 8.660254037844387298, -81.37500000409677625 ) ) ;
#25871=LINE ( 'NONE', #9462, #852 ) ;
#25875=ADVANCED_FACE ( 'NONE', ( #41476 ), #1798, .T. ) ;
#25876=CARTESIAN_POINT ( 'NONE',  ( -9.999999999999998224, 5.773502691896259087, -88.37499999999998579 ) ) ;
#25878=CARTESIAN_POINT ( 'NONE',  ( -4.999999999999996447, 8.660254037844387298, -97.87500000409677625 ) ) ;
#25881=CARTESIAN_POINT ( 'NONE',  ( 5.405949406249999534, 9.363379034771803333, -92.78125000204838102 ) ) ;
#25882=ORIENTED_EDGE ( 'NONE', *, *, #15907, .T. ) ;
#25883=CIRCLE ( 'NONE', #23810, 9.999999999999998224 ) ;
#25886=ORIENTED_EDGE ( 'NONE', *, *, #15852, .F. ) ;
#25887=CARTESIAN_POINT ( 'NONE',  ( 9.999999999999996447, -5.773502691896262640, -17.12499999999997158 ) ) ;
#25888=CARTESIAN_POINT ( 'NONE',  ( 5.000000000000000000, 8.660254037844385522, -156.2500000000000000 ) ) ;
#25890=CARTESIAN_POINT ( 'NONE',  ( 9.999999999999998224, 0.000000000000000000, -84.49999999999997158 ) ) ;
#25891=CARTESIAN_POINT ( 'NONE',  ( -10.81189881249999907, -6.242252689847864744, -128.1562500020483810 ) ) ;
#25892=ORIENTED_EDGE ( 'NONE', *, *, #18751, .F. ) ;
#25893=CARTESIAN_POINT ( 'NONE',  ( -2.121150477449813534E-15, -11.54700538379251284, -21.87499999999997513 ) ) ;
#25896=CARTESIAN_POINT ( 'NONE',  ( -10.81189881249999729, 1.324075727343319199E-15, -54.78125000204836681 ) ) ;
#25898=CARTESIAN_POINT ( 'NONE',  ( 10.81189881249999907, 6.242252689847868297, -101.7187500020483810 ) ) ;
#25901=AXIS2_PLACEMENT_3D ( 'NONE', #9996, #10420, #33329 ) ;
#25902=FACE_OUTER_BOUND ( 'NONE', #1259, .T. ) ;
#25903=CARTESIAN_POINT ( 'NONE',  ( -4.999999999999996447, 8.660254037844387298, -77.99999999999998579 ) ) ;
#25906=CARTESIAN_POINT ( 'NONE',  ( -4.999999999999996447, 8.660254037844387298, -175.5000000000000284 ) ) ;
#25907=CARTESIAN_POINT ( 'NONE',  ( 0.000000000000000000, 0.000000000000000000, -200.0000000000000000 ) ) ;
#25908=CARTESIAN_POINT ( 'NONE',  ( 10.81189881249999729, 6.242252689847867408, -137.7187500020483810 ) ) ;
#25910=CYLINDRICAL_SURFACE ( 'NONE', #6351, 9.999999999999998224 ) ;
#25912=CARTESIAN_POINT ( 'NONE',  ( -2.121150477449813534E-15, -11.54700538379251284, -190.2500000040967905 ) ) ;
#25914=CARTESIAN_POINT ( 'NONE',  ( 10.81189881249999729, 6.242252689847867408, -184.4062500020484094 ) ) ;
#25915=CARTESIAN_POINT ( 'NONE',  ( 10.00000000000051159, -5.773502691895965988, -95.12499999999997158 ) ) ;
#25918=EDGE_CURVE ( 'NONE', #42281, #15678, #2011, .T. ) ;
#25919=CARTESIAN_POINT ( 'NONE',  ( 10.81189881249999729, 6.242252689847867408, -67.21875000204838102 ) ) ;
#25920=CARTESIAN_POINT ( 'NONE',  ( 10.81189881249999907, 6.242252689847868297, -49.21875000204835260 ) ) ;
#25922=CARTESIAN_POINT ( 'NONE',  ( 5.405949406249999534, 9.363379034771803333, -29.78125000204837036 ) ) ;
#25924=CARTESIAN_POINT ( 'NONE',  ( 7.070501591499376803E-16, 11.54700538379251284, -27.50000000409677980 ) ) ;
#25926=EDGE_CURVE ( 'NONE', #39297, #33849, #27914, .T. ) ;
#25927=CARTESIAN_POINT ( 'NONE',  ( 4.999999999999992006, -8.660254037844389075, -116.2499999999999858 ) ) ;
#25928=CARTESIAN_POINT ( 'NONE',  ( 4.999999999999992006, -8.660254037844389075, -114.7499999999999858 ) ) ;
#25929=EDGE_CURVE ( 'NONE', #6727, #38512, #4217, .T. ) ;
#25930=AXIS2_PLACEMENT_3D ( 'NONE', #18995, #31760, #28937 ) ;
#25933=CARTESIAN_POINT ( 'NONE',  ( -5.405949406250003975, -9.363379034771801557, -117.5312500020483952 ) ) ;
#25934=EDGE_LOOP ( 'NONE', ( #5274, #36397, #3474, #39991 ) ) ;
#25939=ORIENTED_EDGE ( 'NONE', *, *, #36120, .T. ) ;
#25940=CARTESIAN_POINT ( 'NONE',  ( -10.00000000000000000, -5.773502691896251982, -43.12499999999997868 ) ) ;
#25941=CARTESIAN_POINT ( 'NONE',  ( 4.999999999999992006, -8.660254037844389075, -16.12500000409675138 ) ) ;
#25942=CARTESIAN_POINT ( 'NONE',  ( 10.81189881249999729, 6.242252689847867408, -43.40625000204837391 ) ) ;
#25943=DIRECTION ( 'NONE',  ( -0.000000000000000000, -0.000000000000000000, 1.000000000000000000 ) ) ;
#25946=CARTESIAN_POINT ( 'NONE',  ( -4.999999999999996447, 8.660254037844387298, -156.3750000040967905 ) ) ;
#25947=CARTESIAN_POINT ( 'NONE',  ( 10.81189881249999551, -6.242252689847874514, -141.1562500020484094 ) ) ;
#25948=CARTESIAN_POINT ( 'NONE',  ( -10.81189881249999907, -6.242252689847864744, -146.1562500020484094 ) ) ;
#25949=EDGE_CURVE ( 'NONE', #23986, #35200, #13270, .T. ) ;
#25950=CARTESIAN_POINT ( 'NONE',  ( 4.999999999999992006, -8.660254037844389075, -110.2499999999999858 ) ) ;
#25951=ORIENTED_EDGE ( 'NONE', *, *, #14883, .T. ) ;
#25952=EDGE_LOOP ( 'NONE', ( #4081, #7575, #37234, #16468 ) ) ;
#25953=ORIENTED_EDGE ( 'NONE', *, *, #1153, .F. ) ;
#25954=EDGE_CURVE ( 'NONE', #3545, #1841, #11694, .T. ) ;
#25955=AXIS2_PLACEMENT_3D ( 'NONE', #18472, #28205, #17822 ) ;
#25957=CARTESIAN_POINT ( 'NONE',  ( 10.81189881249999907, 6.242252689847868297, -173.7187500020484094 ) ) ;
#25958=CARTESIAN_POINT ( 'NONE',  ( -10.81189881249999907, -6.242252689847864744, -19.96875000204838102 ) ) ;
#25959=CARTESIAN_POINT ( 'NONE',  ( 9.999999999999998224, 0.000000000000000000, -60.87500000409676204 ) ) ;
#25960=CARTESIAN_POINT ( 'NONE',  ( -10.81189881249999729, 1.324075727343319199E-15, -162.5937500020484094 ) ) ;
#25961=CARTESIAN_POINT ( 'NONE',  ( -2.293366432827344421E-15, -12.48450537969573659, -144.2187500020483810 ) ) ;
#25962=CARTESIAN_POINT ( 'NONE',  ( 8.614196012143711556, -6.533971456633876684, 2.775557561562891351E-14 ) ) ;
#25965=CARTESIAN_POINT ( 'NONE',  ( -5.405949406250003975, -9.363379034771801557, -15.34375000204835082 ) ) ;
#25968=CARTESIAN_POINT ( 'NONE',  ( -9.999999999999998224, 1.224646799147353059E-15, -25.24999999999996803 ) ) ;
#25971=CARTESIAN_POINT ( 'NONE',  ( 10.81189881249999907, 6.242252689847868297, -76.21875000204836681 ) ) ;
#25972=CARTESIAN_POINT ( 'NONE',  ( 7.644554776091147741E-16, 12.48450537969573659, -47.65625000204836681 ) ) ;
#25976=CARTESIAN_POINT ( 'NONE',  ( 10.00000000000000000, 5.773502691896255534, -141.3750000000000000 ) ) ;
#25977=CARTESIAN_POINT ( 'NONE',  ( -5.405949406250003975, -9.363379034771801557, -141.5312500020483810 ) ) ;
#25979=CARTESIAN_POINT ( 'NONE',  ( 9.999999999999996447, -5.773502691896262640, -110.5000000040967763 ) ) ;
#25981=EDGE_CURVE ( 'NONE', #41327, #36343, #10504, .T. ) ;
#25985=CARTESIAN_POINT ( 'NONE',  ( 0.000000000000000000, 0.000000000000000000, -200.0000000000000000 ) ) ;
#25986=EDGE_CURVE ( 'NONE', #31643, #6545, #1581, .T. ) ;
#25987=CARTESIAN_POINT ( 'NONE',  ( -5.405949406250003975, -9.363379034771801557, -173.0312500020484094 ) ) ;
#25988=CARTESIAN_POINT ( 'NONE',  ( 10.00000000000000000, 5.773502691896255534, -50.25000000409675494 ) ) ;
#25989=( BOUNDED_CURVE ( )  B_SPLINE_CURVE ( 2, ( #34035, #27983, #4245, #31232, #27124, #1230, #14577 ),
 .UNSPECIFIED., .F., .F. ) 
 B_SPLINE_CURVE_WITH_KNOTS ( ( 3, 2, 2, 3 ),
 ( 0.2910447761194031036, 0.2922885572139304333, 0.2935323383084578186, 0.2947761194029852039 ),
 .UNSPECIFIED. ) 
 CURVE ( )  GEOMETRIC_REPRESENTATION_ITEM ( )  RATIONAL_B_SPLINE_CURVE ( ( 0.9999999999999880096, 0.8660254037844506980, 1.000000000000000000, 0.8660254037844387076, 1.000000000000000000, 0.8660254037844267172, 1.000000000000011990 ) ) 
 REPRESENTATION_ITEM ( '' )  );
#25990=CARTESIAN_POINT ( 'NONE',  ( -9.999999999999479527, -5.773502691896549521, -91.50000000409676204 ) ) ;
#25993=LINE ( 'NONE', #39143, #12435 ) ;
#25994=CARTESIAN_POINT ( 'NONE',  ( -10.81189881249999907, -6.242252689847864744, -158.1562500020484094 ) ) ;
#25995=CARTESIAN_POINT ( 'NONE',  ( -10.81189881249999729, 6.242252689847871849, -141.7187500020483810 ) ) ;
#25996=CARTESIAN_POINT ( 'NONE',  ( 9.999999999999998224, 0.000000000000000000, -50.37500000409675494 ) ) ;
#25997=FACE_OUTER_BOUND ( 'NONE', #8546, .T. ) ;
#26000=CARTESIAN_POINT ( 'NONE',  ( 5.405949406249999534, 9.363379034771803333, -71.78125000204838102 ) ) ;
#26003=CARTESIAN_POINT ( 'NONE',  ( -2.293366432827344421E-15, -12.48450537969573659, -123.2187500020483952 ) ) ;
#26004=ORIENTED_EDGE ( 'NONE', *, *, #3396, .T. ) ;
#26005=ORIENTED_EDGE ( 'NONE', *, *, #4875, .T. ) ;
#26006=CARTESIAN_POINT ( 'NONE',  ( -5.405949406250003975, -9.363379034771801557, -27.34375000204835970 ) ) ;
#26007=CARTESIAN_POINT ( 'NONE',  ( 9.999999999999742428, 5.773502691896404748, -159.3749999999999716 ) ) ;
#26008=CARTESIAN_POINT ( 'NONE',  ( 10.81189881249999551, -6.242252689847874514, -194.9687500020484094 ) ) ;
#26009=CARTESIAN_POINT ( 'NONE',  ( 10.81189881249999729, 0.000000000000000000, -53.84375000204835970 ) ) ;
#26011=CARTESIAN_POINT ( 'NONE',  ( 10.81189881249999729, 6.242252689847867408, -191.7187500020484094 ) ) ;
#26012=CARTESIAN_POINT ( 'NONE',  ( 10.81189881249999907, 6.242252689847868297, -172.2187500020483810 ) ) ;
#26015=DIRECTION ( 'NONE',  ( -0.000000000000000000, -0.000000000000000000, 1.000000000000000000 ) ) ;
#26016=CARTESIAN_POINT ( 'NONE',  ( 9.999999999999998224, 0.000000000000000000, -20.37500000409675494 ) ) ;
#26018=CARTESIAN_POINT ( 'NONE',  ( 10.81189881249999551, -6.242252689847874514, -95.96875000204838102 ) ) ;
#26019=CARTESIAN_POINT ( 'NONE',  ( -10.00000000000154188, 5.773502691895366468, -17.87499999999993250 ) ) ;
#26020=CARTESIAN_POINT ( 'NONE',  ( 10.81189881249999907, 6.242252689847868297, -73.40625000204836681 ) ) ;
#26023=CARTESIAN_POINT ( 'NONE',  ( 5.405949406249992428, -9.363379034771808662, -82.59375000204836681 ) ) ;
#26025=CARTESIAN_POINT ( 'NONE',  ( 9.999999999999998224, 0.000000000000000000, -146.3750000040967905 ) ) ;
#26028=ORIENTED_EDGE ( 'NONE', *, *, #31921, .T. ) ;
#26031=CARTESIAN_POINT ( 'NONE',  ( 0.000000000000000000, 0.000000000000000000, -200.0000000000000000 ) ) ;
#26032=CARTESIAN_POINT ( 'NONE',  ( 4.999999999999992006, -8.660254037844389075, -38.24999999999997868 ) ) ;
#26035=VERTEX_POINT ( 'NONE', #12330 ) ;
#26036=CARTESIAN_POINT ( 'NONE',  ( 5.000000000000000000, 8.660254037844385522, -60.24999999999997158 ) ) ;
#26038=CARTESIAN_POINT ( 'NONE',  ( 7.070501591499377789E-16, 11.54700538379251284, -77.00000000409677625 ) ) ;
#26040=CARTESIAN_POINT ( 'NONE',  ( 7.071067811865472841, 7.071067811865472841, -200.0000000000000000 ) ) ;
#26042=CARTESIAN_POINT ( 'NONE',  ( -10.81189881249999729, -6.242252689847864744, -66.65625000204839523 ) ) ;
#26045=CARTESIAN_POINT ( 'NONE',  ( -9.999999999999742428, -5.773502691896402084, -151.5000000040967620 ) ) ;
#26046=CARTESIAN_POINT ( 'NONE',  ( 10.81189881249999729, 0.000000000000000000, -181.5312500020483810 ) ) ;
#26047=ADVANCED_FACE ( 'NONE', ( #5672 ), #6092, .F. ) ;
#26049=CARTESIAN_POINT ( 'NONE',  ( 9.999999999998969713, 5.773502691896851502, -79.87499999999997158 ) ) ;
#26050=CARTESIAN_POINT ( 'NONE',  ( -9.999999999999998224, 1.224646799147353059E-15, -200.0000000000000000 ) ) ;
#26051=CARTESIAN_POINT ( 'NONE',  ( -9.999999999999998224, 1.836970198721029589E-15, 0.000000000000000000 ) ) ;
#26052=CARTESIAN_POINT ( 'NONE',  ( 9.999999999999998224, 0.000000000000000000, -200.0000000000000000 ) ) ;
#26053=CARTESIAN_POINT ( 'NONE',  ( 7.070501591499377789E-16, 11.54700538379251284, -177.1250000000000000 ) ) ;
#26055=CARTESIAN_POINT ( 'NONE',  ( -5.405949406249996869, 9.363379034771805109, -94.03125000204838102 ) ) ;
#26056=VERTEX_POINT ( 'NONE', #2852 ) ;
#26057=CARTESIAN_POINT ( 'NONE',  ( -10.00000000000076916, 5.773502691895813221, -106.7500000040967620 ) ) ;
#26058=EDGE_LOOP ( 'NONE', ( #12179, #23758, #11471, #15206 ) ) ;
#26059=VERTEX_POINT ( 'NONE', #22701 ) ;
#26061=CARTESIAN_POINT ( 'NONE',  ( 5.405949406249999534, 9.363379034771803333, -35.59375000204836681 ) ) ;
#26062=CARTESIAN_POINT ( 'NONE',  ( -2.293366432827344421E-15, -12.48450537969573659, -18.40625000204837036 ) ) ;
#26064=CARTESIAN_POINT ( 'NONE',  ( -10.81189881249999907, -6.242252689847864744, -76.96875000204836681 ) ) ;
#26065=CARTESIAN_POINT ( 'NONE',  ( 9.999999999999998224, 0.000000000000000000, -105.4999999999999858 ) ) ;
#26066=AXIS2_PLACEMENT_3D ( 'NONE', #23407, #7002, #32697 ) ;
#26067=CARTESIAN_POINT ( 'NONE',  ( -10.81189881249999729, 6.242252689847871849, -191.2187500020484663 ) ) ;
#26068=CARTESIAN_POINT ( 'NONE',  ( 7.070501591499376803E-16, 11.54700538379251284, -69.50000000409679046 ) ) ;
#26069=CARTESIAN_POINT ( 'NONE',  ( 10.00000000000051159, -5.773502691895965988, -143.5000000040967905 ) ) ;
#26071=CARTESIAN_POINT ( 'NONE',  ( 5.000000000000000000, 8.660254037844385522, -0.6250000040967651493 ) ) ;
#26072=CARTESIAN_POINT ( 'NONE',  ( -9.999999999999998224, 1.224646799147353059E-15, -103.6250000040967763 ) ) ;
#26073=CARTESIAN_POINT ( 'NONE',  ( 10.81189881249999907, 6.242252689847868297, -125.7187500020483810 ) ) ;
#26074=CARTESIAN_POINT ( 'NONE',  ( -2.293366432827344421E-15, -12.48450537969573659, -100.9062500020483952 ) ) ;
#26075=CARTESIAN_POINT ( 'NONE',  ( 5.405949406249999534, 9.363379034771803333, -107.5937500020483810 ) ) ;
#26078=CARTESIAN_POINT ( 'NONE',  ( 9.999999999999996447, -5.773502691896262640, -172.0000000040967905 ) ) ;
#26079=CARTESIAN_POINT ( 'NONE',  ( -9.183694056713487929E-15, -20.00000000000000355, 12.49999999999999112 ) ) ;
#26085=DIRECTION ( 'NONE',  ( 1.000000000000000000, 0.000000000000000000, 0.000000000000000000 ) ) ;
#26087=CARTESIAN_POINT ( 'NONE',  ( -9.999999999999998224, 5.773502691896259087, -85.37499999999997158 ) ) ;
#26089=CARTESIAN_POINT ( 'NONE',  ( -5.000000000000003553, -8.660254037844383745, -95.87500000409677625 ) ) ;
#26092=CARTESIAN_POINT ( 'NONE',  ( -10.81189881249999729, 6.242252689847871849, -92.40625000204838102 ) ) ;
#26093=VERTEX_POINT ( 'NONE', #22281 ) ;
#26098=ORIENTED_EDGE ( 'NONE', *, *, #38885, .F. ) ;
#26099=CARTESIAN_POINT ( 'NONE',  ( -10.00000000000000000, -5.773502691896251982, -14.62499999999997335 ) ) ;
#26100=CARTESIAN_POINT ( 'NONE',  ( -9.999999999999998224, 5.773502691896259087, -143.8750000000000000 ) ) ;
#26102=CARTESIAN_POINT ( 'NONE',  ( -9.999999999999998224, 5.773502691896259087, -197.8750000000000000 ) ) ;
#26103=CARTESIAN_POINT ( 'NONE',  ( -5.405949406249996869, 9.363379034771805109, -119.5312500020483952 ) ) ;
#26104=VERTEX_POINT ( 'NONE', #25529 ) ;
#26105=CARTESIAN_POINT ( 'NONE',  ( 10.70731569305672615, 1.500182182589836044, 0.000000000000000000 ) ) ;
#26107=EDGE_LOOP ( 'NONE', ( #377, #1645, #5837, #14705 ) ) ;
#26108=CARTESIAN_POINT ( 'NONE',  ( 5.405949406249999534, 9.363379034771803333, -52.28125000204835970 ) ) ;
#26110=CARTESIAN_POINT ( 'NONE',  ( -10.81189881249999729, 1.324075727343319199E-15, -99.59375000204838102 ) ) ;
#26111=ORIENTED_EDGE ( 'NONE', *, *, #15084, .T. ) ;
#26112=CARTESIAN_POINT ( 'NONE',  ( -10.00000000000051337, 5.773502691895962435, -77.87499999999997158 ) ) ;
#26114=CARTESIAN_POINT ( 'NONE',  ( 7.644554776091147741E-16, 12.48450537969573659, -0.9687500020483524876 ) ) ;
#26115=CARTESIAN_POINT ( 'NONE',  ( -4.999999999999996447, 8.660254037844387298, -0.3750000040967649273 ) ) ;
#26116=CARTESIAN_POINT ( 'NONE',  ( 5.405949406249992428, -9.363379034771808662, -132.0937500020483810 ) ) ;
#26119=DIRECTION ( 'NONE',  ( 0.000000000000000000, -0.000000000000000000, 1.000000000000000000 ) ) ;
#26121=CARTESIAN_POINT ( 'NONE',  ( 10.00000000000000000, 5.773502691896255534, -194.2500000040968189 ) ) ;
#26123=CARTESIAN_POINT ( 'NONE',  ( 10.81189881249999729, 0.000000000000000000, -187.5312500020484094 ) ) ;
#26127=CARTESIAN_POINT ( 'NONE',  ( 10.81189881249999551, -6.242252689847874514, -62.96875000204839523 ) ) ;
#26129=CARTESIAN_POINT ( 'NONE',  ( 10.81189881249999907, 6.242252689847868297, -47.71875000204835970 ) ) ;
#26132=CARTESIAN_POINT ( 'NONE',  ( 7.644554776091147741E-16, 12.48450537969573659, -19.15625000204837391 ) ) ;
#26136=CARTESIAN_POINT ( 'NONE',  ( -9.999999999999998224, 1.224646799147353059E-15, -116.7499999999999858 ) ) ;
#26137=CARTESIAN_POINT ( 'NONE',  ( -9.999999999999998224, 1.224646799147353059E-15, -28.24999999999996803 ) ) ;
#26140=CARTESIAN_POINT ( 'NONE',  ( -10.81189881249999729, 6.242252689847871849, -114.9062500020483952 ) ) ;
#26141=VERTEX_POINT ( 'NONE', #19447 ) ;
#26142=CARTESIAN_POINT ( 'NONE',  ( -9.999999999999998224, 1.224646799147353059E-15, -176.7500000000000284 ) ) ;
#26144=CARTESIAN_POINT ( 'NONE',  ( 9.999999999999998224, 0.000000000000000000, -123.8750000040967905 ) ) ;
#26147=CARTESIAN_POINT ( 'NONE',  ( -9.999999999999998224, 5.773502691896259087, -40.37499999999997158 ) ) ;
#26148=CARTESIAN_POINT ( 'NONE',  ( 7.070501591499377789E-16, 11.54700538379251284, -17.00000000409675849 ) ) ;
#26149=CARTESIAN_POINT ( 'NONE',  ( -5.405949406250003975, -9.363379034771801557, -42.53125000204838102 ) ) ;
#26150=CARTESIAN_POINT ( 'NONE',  ( 9.999999999999998224, 0.000000000000000000, -200.0000000000000000 ) ) ;
#26153=( BOUNDED_CURVE ( )  B_SPLINE_CURVE ( 2, ( #6143, #38301, #31634, #21899, #9161, #22330, #35506 ),
 .UNSPECIFIED., .F., .F. ) 
 B_SPLINE_CURVE_WITH_KNOTS ( ( 3, 2, 2, 3 ),
 ( 0.6716417910447763928, 0.6728855721393036671, 0.6741293532338310523, 0.6753731343283584376 ),
 .UNSPECIFIED. ) 
 CURVE ( )  GEOMETRIC_REPRESENTATION_ITEM ( )  RATIONAL_B_SPLINE_CURVE ( ( 0.9999999999999761302, 0.8660254037844625774, 1.000000000000000000, 0.8660254037844387076, 1.000000000000000000, 0.8660254037844148378, 1.000000000000023981 ) ) 
 REPRESENTATION_ITEM ( '' )  );
#26154=DIRECTION ( 'NONE',  ( -0.3779644730092265315, 0.6546536707079755324, 0.6546536707079790851 ) ) ;
#26155=CARTESIAN_POINT ( 'NONE',  ( 5.405949406249999534, 9.363379034771803333, -136.2812500020483810 ) ) ;
#26156=CARTESIAN_POINT ( 'NONE',  ( -5.405949406249996869, 9.363379034771805109, -151.0312500020483810 ) ) ;
#26157=CARTESIAN_POINT ( 'NONE',  ( -9.999999999999998224, 1.224646799147353059E-15, -168.1250000040967905 ) ) ;
#26159=VECTOR ( 'NONE', #4872, 1000.000000000000000 ) ;
#26163=EDGE_CURVE ( 'NONE', #17527, #7578, #20464, .T. ) ;
#26164=CARTESIAN_POINT ( 'NONE',  ( -5.000000000000003553, -8.660254037844383745, -121.3750000040967905 ) ) ;
#26165=CARTESIAN_POINT ( 'NONE',  ( 10.81189881249999551, -6.242252689847874514, -175.4687500020484094 ) ) ;
#26166=AXIS2_PLACEMENT_3D ( 'NONE', #25135, #8512, #18860 ) ;
#26167=CARTESIAN_POINT ( 'NONE',  ( -2.293366432827344421E-15, -12.48450537969573659, -27.21875000204838102 ) ) ;
#26169=CARTESIAN_POINT ( 'NONE',  ( -5.405949406250003975, -9.363379034771801557, -156.3437500020483810 ) ) ;
#26170=CARTESIAN_POINT ( 'NONE',  ( -2.293366432827344421E-15, -12.48450537969573659, -147.2187500020484094 ) ) ;
#26171=CARTESIAN_POINT ( 'NONE',  ( 4.999999999999992006, -8.660254037844389075, -8.625000004096744277 ) ) ;
#26174=CARTESIAN_POINT ( 'NONE',  ( -10.81189881249999907, -6.242252689847864744, -19.96875000204838102 ) ) ;
#26176=DIRECTION ( 'NONE',  ( 1.000000000000000000, 0.000000000000000000, 0.000000000000000000 ) ) ;
#26177=LINE ( 'NONE', #3507, #29594 ) ;
#26180=CARTESIAN_POINT ( 'NONE',  ( 10.81189881249999551, -6.242252689847874514, -74.96875000204838102 ) ) ;
#26181=CARTESIAN_POINT ( 'NONE',  ( 5.405949406249999534, 9.363379034771803333, -38.78125000204838102 ) ) ;
#26185=CARTESIAN_POINT ( 'NONE',  ( 9.999999999999998224, 0.000000000000000000, -135.5000000000000000 ) ) ;
#26186=CARTESIAN_POINT ( 'NONE',  ( -5.405949406249996869, 9.363379034771805109, -136.0312500020484094 ) ) ;
#26188=CARTESIAN_POINT ( 'NONE',  ( 5.000000000000000000, 8.660254037844385522, -110.1250000040967763 ) ) ;
#26190=EDGE_LOOP ( 'NONE', ( #23332, #25016, #29504, #8602 ) ) ;
#26193=VECTOR ( 'NONE', #13493, 1000.000000000000000 ) ;
#26194=CARTESIAN_POINT ( 'NONE',  ( 10.81189881249999551, -6.242252689847874514, -175.6562500020484094 ) ) ;
#26195=CARTESIAN_POINT ( 'NONE',  ( 5.000000000000000000, 8.660254037844385522, -44.12500000409677625 ) ) ;
#26196=CARTESIAN_POINT ( 'NONE',  ( -4.999999999999996447, 8.660254037844387298, -48.37500000409677625 ) ) ;
#26198=CARTESIAN_POINT ( 'NONE',  ( 4.999999999999992006, -8.660254037844389075, -63.74999999999997158 ) ) ;
#26199=CARTESIAN_POINT ( 'NONE',  ( -2.293366432827344421E-15, -12.48450537969573659, -162.4062500020483810 ) ) ;
#26200=CARTESIAN_POINT ( 'NONE',  ( 10.81189881249999729, 0.000000000000000000, -140.8437500020483810 ) ) ;
#26201=FACE_OUTER_BOUND ( 'NONE', #14120, .T. ) ;
#26202=CARTESIAN_POINT ( 'NONE',  ( -9.999999999999998224, 1.224646799147353059E-15, -115.6250000040967905 ) ) ;
#26203=ORIENTED_EDGE ( 'NONE', *, *, #15983, .F. ) ;
#26204=CARTESIAN_POINT ( 'NONE',  ( 9.999999999999998224, 0.000000000000000000, -42.49999999999998579 ) ) ;
#26205=CARTESIAN_POINT ( 'NONE',  ( -2.293366432827344421E-15, -12.48450537969573659, -69.40625000204838102 ) ) ;
#26206=ORIENTED_EDGE ( 'NONE', *, *, #23342, .F. ) ;
#26208=ADVANCED_FACE ( 'NONE', ( #22067 ), #25316, .T. ) ;
#26209=CARTESIAN_POINT ( 'NONE',  ( 7.644554776091147741E-16, 12.48450537969573659, -119.4687500020483952 ) ) ;
#26211=ORIENTED_EDGE ( 'NONE', *, *, #31977, .F. ) ;
#26212=EDGE_CURVE ( 'NONE', #10842, #318, #11902, .T. ) ;
#26213=CARTESIAN_POINT ( 'NONE',  ( 10.81189881249999551, -6.242252689847874514, -22.46875000204837391 ) ) ;
#26214=CARTESIAN_POINT ( 'NONE',  ( -10.81189881249999729, 6.242252689847871849, -198.7187500020484379 ) ) ;
#26216=CARTESIAN_POINT ( 'NONE',  ( -5.405949406250003975, -9.363379034771801557, -46.84375000204838102 ) ) ;
#26217=EDGE_CURVE ( 'NONE', #414, #39570, #16291, .T. ) ;
#26218=DIRECTION ( 'NONE',  ( -0.000000000000000000, -0.000000000000000000, 1.000000000000000000 ) ) ;
#26220=CARTESIAN_POINT ( 'NONE',  ( 10.81189881249999729, 0.000000000000000000, -185.8437500020483810 ) ) ;
#26221=CARTESIAN_POINT ( 'NONE',  ( -5.405949406250003975, -9.363379034771801557, -165.3437500020484094 ) ) ;
#26225=CARTESIAN_POINT ( 'NONE',  ( -2.121150477449813534E-15, -11.54700538379251284, -118.2500000040968189 ) ) ;
#26226=CARTESIAN_POINT ( 'NONE',  ( 9.999999999999742428, 5.773502691896404748, -188.2500000040968189 ) ) ;
#26228=CARTESIAN_POINT ( 'NONE',  ( -5.405949406249996869, 9.363379034771805109, -95.34375000204838102 ) ) ;
#26230=CARTESIAN_POINT ( 'NONE',  ( -2.293366432827344421E-15, -12.48450537969573659, -73.90625000204836681 ) ) ;
#26231=CARTESIAN_POINT ( 'NONE',  ( 4.999999999999992006, -8.660254037844389075, -131.6250000040967620 ) ) ;
#26233=CARTESIAN_POINT ( 'NONE',  ( 5.405949406249999534, 9.363379034771803333, -164.7812500020484094 ) ) ;
#26236=CARTESIAN_POINT ( 'NONE',  ( -10.00000000000000000, -5.773502691896251982, -136.5000000040967905 ) ) ;
#26241=EDGE_CURVE ( 'NONE', #28547, #21458, #14009, .T. ) ;
#26242=CARTESIAN_POINT ( 'NONE',  ( -10.81189881249999729, 6.242252689847871849, -198.9062500020484094 ) ) ;
#26243=LINE ( 'NONE', #39392, #36472 ) ;
#26245=ORIENTED_EDGE ( 'NONE', *, *, #39381, .T. ) ;
#26246=CARTESIAN_POINT ( 'NONE',  ( 5.000000000000000000, 8.660254037844385522, -58.74999999999997158 ) ) ;
#26248=CARTESIAN_POINT ( 'NONE',  ( -2.121150477449813534E-15, -11.54700538379251284, -64.25000000409677625 ) ) ;
#26251=CARTESIAN_POINT ( 'NONE',  ( -5.405949406249996869, 9.363379034771805109, -71.53125000204838102 ) ) ;
#26255=CARTESIAN_POINT ( 'NONE',  ( 7.070501591499376803E-16, 11.54700538379251284, -38.00000000409676204 ) ) ;
#26256=CARTESIAN_POINT ( 'NONE',  ( 5.405949406249992428, -9.363379034771808662, -186.2812500020484094 ) ) ;
#26259=CARTESIAN_POINT ( 'NONE',  ( 9.999999999999998224, 0.000000000000000000, -171.8750000040968189 ) ) ;
#26260=CARTESIAN_POINT ( 'NONE',  ( 7.070501591499376803E-16, 11.54700538379251284, -165.1250000000000000 ) ) ;
#26262=CARTESIAN_POINT ( 'NONE',  ( -7.071067811865472841, -7.071067811865472841, -200.0000000000000000 ) ) ;
#26263=CARTESIAN_POINT ( 'NONE',  ( 9.999999999999998224, 0.000000000000000000, -167.0000000000000000 ) ) ;
#26264=CYLINDRICAL_SURFACE ( 'NONE', #35837, 9.999999999999998224 ) ;
#26265=CARTESIAN_POINT ( 'NONE',  ( 5.405949406249992428, -9.363379034771808662, -91.78125000204838102 ) ) ;
#26266=EDGE_LOOP ( 'NONE', ( #41209, #23351, #24154, #21584 ) ) ;
#26267=FACE_OUTER_BOUND ( 'NONE', #20261, .T. ) ;
#26269=ORIENTED_EDGE ( 'NONE', *, *, #35621, .F. ) ;
#26271=CARTESIAN_POINT ( 'NONE',  ( 10.81189881249999729, 0.000000000000000000, -34.34375000204836681 ) ) ;
#26272=CARTESIAN_POINT ( 'NONE',  ( 5.405949406249992428, -9.363379034771808662, -21.28125000204836326 ) ) ;
#26274=CARTESIAN_POINT ( 'NONE',  ( -10.81189881249999729, 6.242252689847871849, -74.21875000204836681 ) ) ;
#26275=DIRECTION ( 'NONE',  ( -1.000000000000000000, 0.000000000000000000, -0.000000000000000000 ) ) ;
#26276=CARTESIAN_POINT ( 'NONE',  ( 10.81189881249999551, -6.242252689847874514, -190.4687500020484094 ) ) ;
#26277=VECTOR ( 'NONE', #34121, 1000.000000000000000 ) ;
#26278=( BOUNDED_CURVE ( )  B_SPLINE_CURVE ( 2, ( #9960, #19887, #60, #16000, #9334, #42335, #22935 ),
 .UNSPECIFIED., .F., .F. ) 
 B_SPLINE_CURVE_WITH_KNOTS ( ( 3, 2, 2, 3 ),
 ( 0.3470149253731344974, 0.3482587064676618271, 0.3495024875621891569, 0.3507462686567164867 ),
 .UNSPECIFIED. ) 
 CURVE ( )  GEOMETRIC_REPRESENTATION_ITEM ( )  RATIONAL_B_SPLINE_CURVE ( ( 0.9999999999999820144, 0.8660254037844566932, 1.000000000000000000, 0.8660254037844387076, 1.000000000000000000, 0.8660254037844327124, 1.000000000000005995 ) ) 
 REPRESENTATION_ITEM ( '' )  );
#26279=CARTESIAN_POINT ( 'NONE',  ( 10.00000000000102318, -5.773502691895667560, -79.00000000409673362 ) ) ;
#26282=CARTESIAN_POINT ( 'NONE',  ( 4.999999999999992006, -8.660254037844389075, -4.125000004096768258 ) ) ;
#26283=CARTESIAN_POINT ( 'NONE',  ( 9.999999999998969713, 5.773502691896851502, -50.25000000409674072 ) ) ;
#26285=EDGE_CURVE ( 'NONE', #23818, #11901, #26992, .T. ) ;
#26286=CARTESIAN_POINT ( 'NONE',  ( 5.405949406249999534, 9.363379034771803333, -121.0937500020483952 ) ) ;
#26287=CARTESIAN_POINT ( 'NONE',  ( -2.293366432827344421E-15, -12.48450537969573659, -96.40625000204839523 ) ) ;
#26288=CARTESIAN_POINT ( 'NONE',  ( -2.293366432827344421E-15, -12.48450537969573659, -111.2187500020483668 ) ) ;
#26291=CARTESIAN_POINT ( 'NONE',  ( 7.070501591499377789E-16, 11.54700538379251284, -164.0000000040967905 ) ) ;
#26292=( BOUNDED_CURVE ( )  B_SPLINE_CURVE ( 2, ( #63, #16208, #26590, #30050, #16851, #39741, #10385 ),
 .UNSPECIFIED., .F., .F. ) 
 B_SPLINE_CURVE_WITH_KNOTS ( ( 3, 2, 2, 3 ),
 ( 0.1268656716417910224, 0.1281094527363183799, 0.1293532338308457652, 0.1305970149253731227 ),
 .UNSPECIFIED. ) 
 CURVE ( )  GEOMETRIC_REPRESENTATION_ITEM ( )  RATIONAL_B_SPLINE_CURVE ( ( 1.000000000000003109, 0.8660254037844358210, 1.000000000000000000, 0.8660254037844387076, 1.000000000000000000, 0.8660254037844387076, 1.000000000000000000 ) ) 
 REPRESENTATION_ITEM ( '' )  );
#26293=FACE_OUTER_BOUND ( 'NONE', #6993, .T. ) ;
#26297=CARTESIAN_POINT ( 'NONE',  ( -2.121150477449813534E-15, -11.54700538379251284, -156.8750000000000000 ) ) ;
#26299=CARTESIAN_POINT ( 'NONE',  ( 9.999999999998969713, 5.773502691896851502, -6.374999999999940492 ) ) ;
#26301=CARTESIAN_POINT ( 'NONE',  ( 9.999999999999998224, 0.000000000000000000, -79.99999999999998579 ) ) ;
#26303=CARTESIAN_POINT ( 'NONE',  ( -4.999999999999996447, 8.660254037844387298, -99.37500000409679046 ) ) ;
#26306=CARTESIAN_POINT ( 'NONE',  ( -5.405949406250003975, -9.363379034771801557, -89.03125000204838102 ) ) ;
#26307=ORIENTED_EDGE ( 'NONE', *, *, #8561, .T. ) ;
#26309=CARTESIAN_POINT ( 'NONE',  ( 5.000000000000000000, 8.660254037844385522, -48.24999999999998579 ) ) ;
#26311=VERTEX_POINT ( 'NONE', #36704 ) ;
#26312=CARTESIAN_POINT ( 'NONE',  ( 9.999999999999998224, 0.000000000000000000, -7.999999999999952038 ) ) ;
#26313=CARTESIAN_POINT ( 'NONE',  ( -9.999999999999998224, 1.224646799147353059E-15, -146.7500000000000000 ) ) ;
#26316=CARTESIAN_POINT ( 'NONE',  ( 9.999999999999998224, 0.000000000000000000, -191.0000000000000000 ) ) ;
#26317=CARTESIAN_POINT ( 'NONE',  ( 10.81189881249999551, -6.242252689847874514, -118.6562500020483952 ) ) ;
#26318=ORIENTED_EDGE ( 'NONE', *, *, #12588, .F. ) ;
#26319=DIRECTION ( 'NONE',  ( 1.000000000000000000, 0.000000000000000000, 0.000000000000000000 ) ) ;
#26321=CARTESIAN_POINT ( 'NONE',  ( -5.405949406249996869, 9.363379034771805109, -44.53125000204838102 ) ) ;
#26323=CARTESIAN_POINT ( 'NONE',  ( -10.81189881249999907, -6.242252689847864744, -106.9687500020483668 ) ) ;
#26324=CARTESIAN_POINT ( 'NONE',  ( -10.81189881249999729, 1.324075727343319199E-15, -125.2812500020483668 ) ) ;
#26326=CARTESIAN_POINT ( 'NONE',  ( -2.121150477449813534E-15, -11.54700538379251284, -85.25000000409676204 ) ) ;
#26327=CARTESIAN_POINT ( 'NONE',  ( 9.999999999999998224, 0.000000000000000000, -125.3750000040967905 ) ) ;
#26329=CARTESIAN_POINT ( 'NONE',  ( -2.121150477449813534E-15, -11.54700538379251284, -26.37499999999998224 ) ) ;
#26330=CARTESIAN_POINT ( 'NONE',  ( 9.999999999999998224, 0.000000000000000000, -0.8750000040967653714 ) ) ;
#26331=CARTESIAN_POINT ( 'NONE',  ( 10.81189881249999551, -6.242252689847874514, -130.4687500020483810 ) ) ;
#26334=CARTESIAN_POINT ( 'NONE',  ( 7.070501591499377789E-16, 11.54700538379251284, -197.0000000040968189 ) ) ;
#26336=CARTESIAN_POINT ( 'NONE',  ( 7.644554776091147741E-16, 12.48450537969573659, -187.1562500020484094 ) ) ;
#26338=FACE_OUTER_BOUND ( 'NONE', #32895, .T. ) ;
#26341=CARTESIAN_POINT ( 'NONE',  ( 5.405949406249999534, 9.363379034771803333, -61.09375000204836681 ) ) ;
#26342=CARTESIAN_POINT ( 'NONE',  ( -10.81189881249999729, 1.324075727343319199E-15, -48.59375000204838102 ) ) ;
#26344=CARTESIAN_POINT ( 'NONE',  ( -10.81189881249999907, -6.242252689847864744, -21.65625000204837036 ) ) ;
#26347=CARTESIAN_POINT ( 'NONE',  ( 9.999999999999996447, -5.773502691896262640, -102.6249999999999858 ) ) ;
#26349=CARTESIAN_POINT ( 'NONE',  ( 10.00000000000102318, -5.773502691895667560, -27.62499999999995737 ) ) ;
#26352=CARTESIAN_POINT ( 'NONE',  ( 5.405949406249999534, 9.363379034771803333, -113.7812500020483952 ) ) ;
#26353=EDGE_CURVE ( 'NONE', #38098, #27593, #16403, .T. ) ;
#26354=ORIENTED_EDGE ( 'NONE', *, *, #40947, .T. ) ;
#26359=VERTEX_POINT ( 'NONE', #30248 ) ;
#26360=CARTESIAN_POINT ( 'NONE',  ( -9.999999999999998224, 1.224646799147353059E-15, -29.74999999999997158 ) ) ;
#26362=CARTESIAN_POINT ( 'NONE',  ( 9.999999999999998224, 0.000000000000000000, -21.87500000409675494 ) ) ;
#26363=CARTESIAN_POINT ( 'NONE',  ( 5.405949406249999534, 9.363379034771803333, -43.28125000204838102 ) ) ;
#26364=CARTESIAN_POINT ( 'NONE',  ( 4.999999999999992006, -8.660254037844389075, -90.74999999999998579 ) ) ;
#26367=CARTESIAN_POINT ( 'NONE',  ( 5.405949406249999534, 9.363379034771803333, -140.7812500020483810 ) ) ;
#26368=CARTESIAN_POINT ( 'NONE',  ( 7.644554776091147741E-16, 12.48450537969573659, -140.6562500020484094 ) ) ;
#26369=DIRECTION ( 'NONE',  ( -0.000000000000000000, -0.000000000000000000, 1.000000000000000000 ) ) ;
#26370=ORIENTED_EDGE ( 'NONE', *, *, #30711, .T. ) ;
#26372=EDGE_CURVE ( 'NONE', #39976, #28849, #29822, .T. ) ;
#26373=ORIENTED_EDGE ( 'NONE', *, *, #25637, .F. ) ;
#26374=CARTESIAN_POINT ( 'NONE',  ( 10.00000000000025402, -5.773502691896113426, -121.0000000040967763 ) ) ;
#26375=CARTESIAN_POINT ( 'NONE',  ( -5.405949406249996869, 9.363379034771805109, -171.8437500020484094 ) ) ;
#26377=CARTESIAN_POINT ( 'NONE',  ( 10.81189881249999551, -6.242252689847874514, -22.46875000204837391 ) ) ;
#26378=DIRECTION ( 'NONE',  ( -0.000000000000000000, -0.000000000000000000, 1.000000000000000000 ) ) ;
#26379=CARTESIAN_POINT ( 'NONE',  ( 10.81189881249999551, -6.242252689847874514, -158.9687500020484094 ) ) ;
#26380=CARTESIAN_POINT ( 'NONE',  ( -10.81189881249999907, -6.242252689847864744, -144.4687500020484094 ) ) ;
#26384=CARTESIAN_POINT ( 'NONE',  ( 10.81189881249999551, -6.242252689847874514, -16.46875000204836326 ) ) ;
#26387=CYLINDRICAL_SURFACE ( 'NONE', #31667, 9.999999999999998224 ) ;
#26389=CARTESIAN_POINT ( 'NONE',  ( -2.121150477449813534E-15, -11.54700538379251284, -167.7500000040968189 ) ) ;
#26390=CARTESIAN_POINT ( 'NONE',  ( 5.405949406249999534, 9.363379034771803333, -70.09375000204836681 ) ) ;
#26391=CARTESIAN_POINT ( 'NONE',  ( 5.405949406249999534, 9.363379034771803333, -43.28125000204838102 ) ) ;
#26395=CARTESIAN_POINT ( 'NONE',  ( 10.00000000000000000, 5.773502691896255534, -130.8750000000000000 ) ) ;
#26396=CARTESIAN_POINT ( 'NONE',  ( 10.81189881249999729, 6.242252689847867408, -142.4062500020484094 ) ) ;
#26397=LINE ( 'NONE', #23378, #25504 ) ;
#26398=CARTESIAN_POINT ( 'NONE',  ( 10.00000000000000000, 5.773502691896255534, -111.7500000040967763 ) ) ;
#26400=( BOUNDED_CURVE ( )  B_SPLINE_CURVE ( 2, ( #8334, #24744, #30573, #40253, #1004, #34020, #17583 ),
 .UNSPECIFIED., .F., .F. ) 
 B_SPLINE_CURVE_WITH_KNOTS ( ( 3, 2, 2, 3 ),
 ( 0.5895522388059702967, 0.5907960199004975710, 0.5920398009950249563, 0.5932835820895523415 ),
 .UNSPECIFIED. ) 
 CURVE ( )  GEOMETRIC_REPRESENTATION_ITEM ( )  RATIONAL_B_SPLINE_CURVE ( ( 0.9999999999999880096, 0.8660254037844506980, 1.000000000000000000, 0.8660254037844387076, 1.000000000000000000, 0.8660254037844267172, 1.000000000000011990 ) ) 
 REPRESENTATION_ITEM ( '' )  );
#26401=ORIENTED_EDGE ( 'NONE', *, *, #27778, .F. ) ;
#26405=CARTESIAN_POINT ( 'NONE',  ( -10.81189881249999729, 1.324075727343319199E-15, -165.7812500020484094 ) ) ;
#26406=CARTESIAN_POINT ( 'NONE',  ( 7.070501591499377789E-16, 11.54700538379251284, -39.50000000409675494 ) ) ;
#26407=EDGE_CURVE ( 'NONE', #2222, #17679, #35617, .T. ) ;
#26408=CARTESIAN_POINT ( 'NONE',  ( 7.070501591499376803E-16, 11.54700538379251284, -48.50000000409676915 ) ) ;
#26410=CARTESIAN_POINT ( 'NONE',  ( -9.999999999999998224, 1.224646799147353059E-15, -175.2500000000000284 ) ) ;
#26411=CARTESIAN_POINT ( 'NONE',  ( -10.81189881249999907, -6.242252689847864744, -162.6562500020483810 ) ) ;
#26412=CARTESIAN_POINT ( 'NONE',  ( -5.405949406249996869, 9.363379034771805109, -138.8437500020484094 ) ) ;
#26413=CARTESIAN_POINT ( 'NONE',  ( 9.999999999999998224, 0.000000000000000000, -93.87500000409677625 ) ) ;
#26414=ORIENTED_EDGE ( 'NONE', *, *, #25918, .T. ) ;
#26415=CARTESIAN_POINT ( 'NONE',  ( 10.81189881249999907, 6.242252689847868297, -68.90625000204839523 ) ) ;
#26416=ORIENTED_EDGE ( 'NONE', *, *, #10897, .F. ) ;
#26418=CARTESIAN_POINT ( 'NONE',  ( -10.81189881249999729, 6.242252689847871849, -120.7187500020483952 ) ) ;
#26420=ORIENTED_EDGE ( 'NONE', *, *, #7371, .F. ) ;
#26421=CARTESIAN_POINT ( 'NONE',  ( 7.644554776091147741E-16, 12.48450537969573659, -20.46875000204836326 ) ) ;
#26422=CARTESIAN_POINT ( 'NONE',  ( 5.405949406249999534, 9.363379034771803333, -197.5937500020484094 ) ) ;
#26423=CARTESIAN_POINT ( 'NONE',  ( 7.644554776091147741E-16, 12.48450537969573659, -44.46875000204836681 ) ) ;
#26424=LINE ( 'NONE', #20153, #8910 ) ;
#26426=CARTESIAN_POINT ( 'NONE',  ( -10.81189881249999729, 1.324075727343319199E-15, -180.5937500020484094 ) ) ;
#26427=CARTESIAN_POINT ( 'NONE',  ( 7.644554776091147741E-16, 12.48450537969573659, -168.9687500020483810 ) ) ;
#26433=CARTESIAN_POINT ( 'NONE',  ( 5.405949406249992428, -9.363379034771808662, -100.5937500020483810 ) ) ;
#26434=CARTESIAN_POINT ( 'NONE',  ( 4.999999999999992006, -8.660254037844389075, -101.2499999999999858 ) ) ;
#26435=CARTESIAN_POINT ( 'NONE',  ( -10.81189881249999729, 1.324075727343319199E-15, -68.28125000204838102 ) ) ;
#26438=CARTESIAN_POINT ( 'NONE',  ( -5.405949406250003975, -9.363379034771801557, -123.5312500020483952 ) ) ;
#26439=CARTESIAN_POINT ( 'NONE',  ( 10.81189881249999729, 6.242252689847867408, -161.9062500020483810 ) ) ;
#26441=CARTESIAN_POINT ( 'NONE',  ( 7.070501591499377789E-16, 11.54700538379251284, -137.0000000040967905 ) ) ;
#26446=CARTESIAN_POINT ( 'NONE',  ( 10.81189881249999907, 6.242252689847868297, -196.4062500020484379 ) ) ;
#26447=CARTESIAN_POINT ( 'NONE',  ( 7.070501591499376803E-16, 11.54700538379251284, -131.0000000040967905 ) ) ;
#26450=CARTESIAN_POINT ( 'NONE',  ( -9.999999999999998224, 1.224646799147353059E-15, -55.24999999999996447 ) ) ;
#26452=CARTESIAN_POINT ( 'NONE',  ( 9.999999999999998224, 0.000000000000000000, -63.87500000409676915 ) ) ;
#26453=EDGE_CURVE ( 'NONE', #31054, #22217, #23125, .T. ) ;
#26458=CARTESIAN_POINT ( 'NONE',  ( -5.405949406250003975, -9.363379034771801557, -57.53125000204836681 ) ) ;
#26459=EDGE_CURVE ( 'NONE', #10615, #30730, #32343, .T. ) ;
#26462=CARTESIAN_POINT ( 'NONE',  ( 9.999999999999998224, 0.000000000000000000, -150.8750000040967905 ) ) ;
#26463=CARTESIAN_POINT ( 'NONE',  ( 5.405949406249992428, -9.363379034771808662, -183.2812500020484094 ) ) ;
#26465=CARTESIAN_POINT ( 'NONE',  ( -9.999999999999998224, 1.224646799147353059E-15, -116.7499999999999858 ) ) ;
#26466=LINE ( 'NONE', #23447, #6205 ) ;
#26468=DIRECTION ( 'NONE',  ( -0.000000000000000000, -0.000000000000000000, 1.000000000000000000 ) ) ;
#26469=CARTESIAN_POINT ( 'NONE',  ( -2.121150477449813534E-15, -11.54700538379251284, -170.3750000000000284 ) ) ;
#26470=CARTESIAN_POINT ( 'NONE',  ( 9.999999999999998224, 0.000000000000000000, -137.3750000040967905 ) ) ;
#26471=CARTESIAN_POINT ( 'NONE',  ( 10.81189881249999729, 0.000000000000000000, -91.53125000204838102 ) ) ;
#26472=ORIENTED_EDGE ( 'NONE', *, *, #29207, .F. ) ;
#26473=CARTESIAN_POINT ( 'NONE',  ( -9.999999999999998224, 1.224646799147353059E-15, -200.0000000000000000 ) ) ;
#26475=CARTESIAN_POINT ( 'NONE',  ( 5.000000000000000000, 8.660254037844385522, -162.2500000000000000 ) ) ;
#26476=ORIENTED_EDGE ( 'NONE', *, *, #10106, .T. ) ;
#26478=CARTESIAN_POINT ( 'NONE',  ( -2.293366432827344421E-15, -12.48450537969573659, -36.21875000204835970 ) ) ;
#26479=CARTESIAN_POINT ( 'NONE',  ( -2.293366432827344421E-15, -12.48450537969573659, -19.90625000204837747 ) ) ;
#26482=CARTESIAN_POINT ( 'NONE',  ( -10.81189881249999907, -6.242252689847864744, -72.46875000204835260 ) ) ;
#26483=EDGE_CURVE ( 'NONE', #35357, #30453, #23510, .T. ) ;
#26484=CARTESIAN_POINT ( 'NONE',  ( -2.293366432827344421E-15, -12.48450537969573659, -196.7187500020484094 ) ) ;
#26485=CARTESIAN_POINT ( 'NONE',  ( -10.81189881249999729, 6.242252689847871849, -153.7187500020483526 ) ) ;
#26486=( BOUNDED_CURVE ( )  B_SPLINE_CURVE ( 2, ( #17437, #10967, #24163, #37309, #1280, #14408, #27602 ),
 .UNSPECIFIED., .F., .F. ) 
 B_SPLINE_CURVE_WITH_KNOTS ( ( 3, 2, 2, 3 ),
 ( 0.7014925373134330844, 0.7027363184079604697, 0.7039800995024877439, 0.7052238805970151292 ),
 .UNSPECIFIED. ) 
 CURVE ( )  GEOMETRIC_REPRESENTATION_ITEM ( )  RATIONAL_B_SPLINE_CURVE ( ( 0.9999999999999761302, 0.8660254037844625774, 1.000000000000000000, 0.8660254037844387076, 1.000000000000000000, 0.8660254037844148378, 1.000000000000023981 ) ) 
 REPRESENTATION_ITEM ( '' )  );
#26487=CARTESIAN_POINT ( 'NONE',  ( 5.000000000000000000, 8.660254037844385522, -72.62500000409677625 ) ) ;
#26488=DIRECTION ( 'NONE',  ( -0.000000000000000000, -0.000000000000000000, 1.000000000000000000 ) ) ;
#26490=CARTESIAN_POINT ( 'NONE',  ( 9.999999999999996447, -5.773502691896262640, 0.4999999959032586094 ) ) ;
#26491=CARTESIAN_POINT ( 'NONE',  ( 0.000000000000000000, 0.000000000000000000, -200.0000000000000000 ) ) ;
#26492=CARTESIAN_POINT ( 'NONE',  ( 10.81189881249999907, 6.242252689847868297, -121.2187500020483952 ) ) ;
#26493=CARTESIAN_POINT ( 'NONE',  ( 9.999999999999998224, 0.000000000000000000, -66.49999999999997158 ) ) ;
#26494=CARTESIAN_POINT ( 'NONE',  ( -10.81189881249999729, 6.242252689847871849, -87.90625000204838102 ) ) ;
#26495=CARTESIAN_POINT ( 'NONE',  ( -10.81189881249999729, -6.242252689847864744, -109.9687500020483810 ) ) ;
#26499=CARTESIAN_POINT ( 'NONE',  ( 9.999999999999998224, 0.000000000000000000, -164.3750000040967905 ) ) ;
#26503=CARTESIAN_POINT ( 'NONE',  ( 9.999999999999998224, 0.000000000000000000, -156.5000000000000000 ) ) ;
#26505=CYLINDRICAL_SURFACE ( 'NONE', #40577, 9.999999999999998224 ) ;
#26507=CARTESIAN_POINT ( 'NONE',  ( -5.000000000000003553, -8.660254037844383745, -80.49999999999998579 ) ) ;
#26509=CARTESIAN_POINT ( 'NONE',  ( 9.999999999999996447, -5.773502691896262640, -88.00000000409677625 ) ) ;
#26512=CARTESIAN_POINT ( 'NONE',  ( -10.81189881249999729, -6.242252689847864744, -80.15625000204836681 ) ) ;
#26513=VERTEX_POINT ( 'NONE', #34767 ) ;
#26514=EDGE_CURVE ( 'NONE', #37214, #35978, #13013, .T. ) ;
#26519=CARTESIAN_POINT ( 'NONE',  ( 10.00000000000000000, 5.773502691896255534, -6.374999999999966249 ) ) ;
#26520=CARTESIAN_POINT ( 'NONE',  ( 4.999999999999992006, -8.660254037844389075, -141.7500000000000000 ) ) ;
#26521=CARTESIAN_POINT ( 'NONE',  ( 5.000000000000000000, 8.660254037844385522, -45.62500000409677625 ) ) ;
#26523=CARTESIAN_POINT ( 'NONE',  ( 4.999999999999992006, -8.660254037844389075, -189.7500000000000000 ) ) ;
#26524=CARTESIAN_POINT ( 'NONE',  ( -2.121150477449813534E-15, -11.54700538379251284, -184.2500000040967905 ) ) ;
#26525=CARTESIAN_POINT ( 'NONE',  ( 10.81189881249999551, -6.242252689847874514, -115.6562500020483810 ) ) ;
#26526=ORIENTED_EDGE ( 'NONE', *, *, #32055, .F. ) ;
#26529=EDGE_CURVE ( 'NONE', #22060, #25538, #7492, .T. ) ;
#26530=( BOUNDED_CURVE ( )  B_SPLINE_CURVE ( 2, ( #9023, #2560, #2766, #5360, #35150, #18517, #15270 ),
 .UNSPECIFIED., .F., .F. ) 
 B_SPLINE_CURVE_WITH_KNOTS ( ( 3, 2, 2, 3 ),
 ( 0.9664179104477613746, 0.9676616915422887599, 0.9689054726368161452, 0.9701492537313435305 ),
 .UNSPECIFIED. ) 
 CURVE ( )  GEOMETRIC_REPRESENTATION_ITEM ( )  RATIONAL_B_SPLINE_CURVE ( ( 0.9999999999999761302, 0.8660254037844625774, 1.000000000000000000, 0.8660254037844387076, 1.000000000000000000, 0.8660254037844148378, 1.000000000000023981 ) ) 
 REPRESENTATION_ITEM ( '' )  );
#26531=CARTESIAN_POINT ( 'NONE',  ( -10.81189881249999729, 1.324075727343319199E-15, -45.78125000204838813 ) ) ;
#26533=CARTESIAN_POINT ( 'NONE',  ( 10.81189881249999729, 0.000000000000000000, -91.34375000204838102 ) ) ;
#26534=CARTESIAN_POINT ( 'NONE',  ( -2.293366432827344421E-15, -12.48450537969573659, -126.4062500020483810 ) ) ;
#26535=ORIENTED_EDGE ( 'NONE', *, *, #31434, .F. ) ;
#26536=CARTESIAN_POINT ( 'NONE',  ( 9.999999999999998224, 0.000000000000000000, -82.99999999999997158 ) ) ;
#26537=CARTESIAN_POINT ( 'NONE',  ( 9.999999999999998224, 0.000000000000000000, -115.9999999999999858 ) ) ;
#26538=( BOUNDED_CURVE ( )  B_SPLINE_CURVE ( 2, ( #5947, #26007, #3921, #39733, #36504, #10583, #19095 ),
 .UNSPECIFIED., .F., .F. ) 
 B_SPLINE_CURVE_WITH_KNOTS ( ( 3, 2, 2, 3 ),
 ( 0.2014925373134328901, 0.2027363184079602476, 0.2039800995024875774, 0.2052238805970149627 ),
 .UNSPECIFIED. ) 
 CURVE ( )  GEOMETRIC_REPRESENTATION_ITEM ( )  RATIONAL_B_SPLINE_CURVE ( ( 0.9999999999999940048, 0.8660254037844447028, 1.000000000000000000, 0.8660254037844387076, 1.000000000000000000, 0.8660254037844357100, 1.000000000000002887 ) ) 
 REPRESENTATION_ITEM ( '' )  );
#26541=CARTESIAN_POINT ( 'NONE',  ( -5.405949406249996869, 9.363379034771805109, -128.3437500020484094 ) ) ;
#26543=DIRECTION ( 'NONE',  ( -0.000000000000000000, -0.000000000000000000, 1.000000000000000000 ) ) ;
#26545=CARTESIAN_POINT ( 'NONE',  ( -9.999999999999998224, 5.773502691896259087, -189.2500000040967905 ) ) ;
#26547=CARTESIAN_POINT ( 'NONE',  ( 10.81189881249999729, 0.000000000000000000, -184.5312500020484094 ) ) ;
#26549=CARTESIAN_POINT ( 'NONE',  ( -9.999999999999479527, -5.773502691896549521, -95.62499999999995737 ) ) ;
#26553=CARTESIAN_POINT ( 'NONE',  ( -10.81189881249999729, 1.324075727343319199E-15, -63.59375000204836681 ) ) ;
#26554=CARTESIAN_POINT ( 'NONE',  ( -10.81189881249999729, 6.242252689847871849, -48.71875000204835970 ) ) ;
#26556=CARTESIAN_POINT ( 'NONE',  ( -5.405949406250003975, -9.363379034771801557, -18.53125000204835970 ) ) ;
#26560=CARTESIAN_POINT ( 'NONE',  ( -9.999999999999998224, 5.773502691896259087, -104.8749999999999858 ) ) ;
#26562=CARTESIAN_POINT ( 'NONE',  ( 4.999999999999992006, -8.660254037844389075, -27.74999999999996803 ) ) ;
#26565=CARTESIAN_POINT ( 'NONE',  ( -5.405949406249996869, 9.363379034771805109, -112.0312500020483810 ) ) ;
#26567=FACE_OUTER_BOUND ( 'NONE', #40649, .T. ) ;
#26572=CARTESIAN_POINT ( 'NONE',  ( -2.121150477449813534E-15, -11.54700538379251284, -35.37499999999996447 ) ) ;
#26573=CARTESIAN_POINT ( 'NONE',  ( 10.00000000000000000, 5.773502691896255534, -20.25000000409677625 ) ) ;
#26574=CARTESIAN_POINT ( 'NONE',  ( -5.405949406250003975, -9.363379034771801557, -41.03125000204838102 ) ) ;
#26575=CARTESIAN_POINT ( 'NONE',  ( 7.070501591499376803E-16, 11.54700538379251284, -35.00000000409674783 ) ) ;
#26577=ADVANCED_FACE ( 'NONE', ( #40988 ), #8435, .T. ) ;
#26578=CARTESIAN_POINT ( 'NONE',  ( 5.405949406249999534, 9.363379034771803333, -143.7812500020483810 ) ) ;
#26580=VERTEX_POINT ( 'NONE', #34550 ) ;
#26583=EDGE_CURVE ( 'NONE', #4760, #6102, #4541, .T. ) ;
#26585=CARTESIAN_POINT ( 'NONE',  ( -5.405949406249996869, 9.363379034771805109, -170.3437500020484094 ) ) ;
#26586=CARTESIAN_POINT ( 'NONE',  ( -5.405949406249996869, 9.363379034771805109, -21.84375000204835615 ) ) ;
#26587=LINE ( 'NONE', #32860, #22610 ) ;
#26588=CARTESIAN_POINT ( 'NONE',  ( 10.81189881249999729, 6.242252689847867408, -157.2187500020483810 ) ) ;
#26589=CARTESIAN_POINT ( 'NONE',  ( 5.405949406249992428, -9.363379034771808662, -145.5937500020483810 ) ) ;
#26590=CARTESIAN_POINT ( 'NONE',  ( 5.000000000000000000, 8.660254037844385522, -173.1250000040968189 ) ) ;
#26594=CARTESIAN_POINT ( 'NONE',  ( -2.293366432827344421E-15, -12.48450537969573659, -7.718750002048352599 ) ) ;
#26597=VECTOR ( 'NONE', #11324, 1000.000000000000000 ) ;
#26598=DIRECTION ( 'NONE',  ( -0.000000000000000000, -0.000000000000000000, 1.000000000000000000 ) ) ;
#26600=CARTESIAN_POINT ( 'NONE',  ( 5.000000000000000000, 8.660254037844385522, -56.12500000409676204 ) ) ;
#26601=CARTESIAN_POINT ( 'NONE',  ( 7.644554776091147741E-16, 12.48450537969573659, -74.46875000204838102 ) ) ;
#26602=CARTESIAN_POINT ( 'NONE',  ( -2.293366432827344421E-15, -12.48450537969573659, -43.90625000204838102 ) ) ;
#26604=DIRECTION ( 'NONE',  ( -0.000000000000000000, 1.000000000000000000, -0.000000000000000000 ) ) ;
#26606=CARTESIAN_POINT ( 'NONE',  ( 5.000000000000000000, 8.660254037844385522, -126.2499999999999716 ) ) ;
#26607=AXIS2_PLACEMENT_3D ( 'NONE', #21217, #27704, #28735 ) ;
#26608=CARTESIAN_POINT ( 'NONE',  ( -10.81189881249999729, 6.242252689847871849, -135.9062500020484094 ) ) ;
#26609=( BOUNDED_CURVE ( )  B_SPLINE_CURVE ( 2, ( #10671, #6814, #14324, #36381, #39818, #33155, #4212 ),
 .UNSPECIFIED., .F., .F. ) 
 B_SPLINE_CURVE_WITH_KNOTS ( ( 3, 2, 2, 3 ),
 ( 0.8805970149253734558, 0.8818407960199008411, 0.8830845771144281153, 0.8843283582089555006 ),
 .UNSPECIFIED. ) 
 CURVE ( )  GEOMETRIC_REPRESENTATION_ITEM ( )  RATIONAL_B_SPLINE_CURVE ( ( 0.9999999999999641398, 0.8660254037844745678, 1.000000000000000000, 0.8660254037844387076, 1.000000000000000000, 0.8660254037844148378, 1.000000000000023981 ) ) 
 REPRESENTATION_ITEM ( '' )  );
#26611=CARTESIAN_POINT ( 'NONE',  ( 10.00000000000000000, 5.773502691896255534, -114.7500000040967763 ) ) ;
#26613=ORIENTED_EDGE ( 'NONE', *, *, #17490, .T. ) ;
#26616=CARTESIAN_POINT ( 'NONE',  ( 9.999999999999998224, 0.000000000000000000, -134.0000000000000000 ) ) ;
#26617=CARTESIAN_POINT ( 'NONE',  ( -5.405949406250003975, -9.363379034771801557, -165.5312500020484094 ) ) ;
#26618=CARTESIAN_POINT ( 'NONE',  ( 4.999999999999992006, -8.660254037844389075, -43.12500000409677625 ) ) ;
#26619=CARTESIAN_POINT ( 'NONE',  ( 7.070501591499376803E-16, 11.54700538379251284, -155.0000000040968189 ) ) ;
#26621=EDGE_CURVE ( 'NONE', #39524, #20204, #34337, .T. ) ;
#26622=CARTESIAN_POINT ( 'NONE',  ( 7.070501591499376803E-16, 11.54700538379251284, -45.12499999999997158 ) ) ;
#26623=CARTESIAN_POINT ( 'NONE',  ( 7.644554776091147741E-16, 12.48450537969573659, -164.6562500020484094 ) ) ;
#26624=CARTESIAN_POINT ( 'NONE',  ( -10.81189881249999907, -6.242252689847864744, -135.4687500020483810 ) ) ;
#26625=FACE_OUTER_BOUND ( 'NONE', #1215, .T. ) ;
#26626=CARTESIAN_POINT ( 'NONE',  ( 9.999999999999998224, 0.000000000000000000, -179.0000000000000000 ) ) ;
#26628=CARTESIAN_POINT ( 'NONE',  ( -10.81189881249999729, 6.242252689847871849, -69.90625000204839523 ) ) ;
#26629=VERTEX_POINT ( 'NONE', #7998 ) ;
#26631=CARTESIAN_POINT ( 'NONE',  ( 10.81189881249999551, -6.242252689847874514, -121.4687500020484094 ) ) ;
#26632=VERTEX_POINT ( 'NONE', #1314 ) ;
#26633=ORIENTED_EDGE ( 'NONE', *, *, #31857, .T. ) ;
#26634=CARTESIAN_POINT ( 'NONE',  ( 10.81189881249999729, 6.242252689847867408, -17.71875000204836681 ) ) ;
#26635=CARTESIAN_POINT ( 'NONE',  ( -10.81189881249999729, 6.242252689847871849, -195.7187500020484379 ) ) ;
#26636=CARTESIAN_POINT ( 'NONE',  ( 5.405949406249992428, -9.363379034771808662, -43.59375000204837391 ) ) ;
#26637=DIRECTION ( 'NONE',  ( 1.000000000000000000, 0.000000000000000000, 0.000000000000000000 ) ) ;
#26639=CARTESIAN_POINT ( 'NONE',  ( -4.999999999999996447, 8.660254037844387298, -151.8750000040967905 ) ) ;
#26640=CARTESIAN_POINT ( 'NONE',  ( 5.405949406249999534, 9.363379034771803333, -178.0937500020484094 ) ) ;
#26641=CARTESIAN_POINT ( 'NONE',  ( -5.405949406250003975, -9.363379034771801557, -166.8437500020484094 ) ) ;
#26645=CARTESIAN_POINT ( 'NONE',  ( -9.999999999999998224, 1.224646799147353059E-15, -118.6250000040967905 ) ) ;
#26647=CARTESIAN_POINT ( 'NONE',  ( 5.405949406249992428, -9.363379034771808662, -96.09375000204838102 ) ) ;
#26648=CARTESIAN_POINT ( 'NONE',  ( -9.999999999999998224, 1.224646799147353059E-15, -34.24999999999997158 ) ) ;
#26649=CARTESIAN_POINT ( 'NONE',  ( 10.81189881249999907, 6.242252689847868297, -70.40625000204839523 ) ) ;
#26652=CARTESIAN_POINT ( 'NONE',  ( 10.81189881249999551, -6.242252689847874514, -126.1562500020483810 ) ) ;
#26653=CARTESIAN_POINT ( 'NONE',  ( 10.81189881249999551, -6.242252689847874514, -160.6562500020484094 ) ) ;
#26655=CARTESIAN_POINT ( 'NONE',  ( 7.070501591499377789E-16, 11.54700538379251284, -135.5000000040967905 ) ) ;
#26657=VERTEX_POINT ( 'NONE', #7795 ) ;
#26660=CARTESIAN_POINT ( 'NONE',  ( 7.644554776091147741E-16, 12.48450537969573659, -188.6562500020484379 ) ) ;
#26663=ORIENTED_EDGE ( 'NONE', *, *, #31803, .F. ) ;
#26664=CARTESIAN_POINT ( 'NONE',  ( 7.070501591499377789E-16, 11.54700538379251284, -57.12499999999997868 ) ) ;
#26666=CARTESIAN_POINT ( 'NONE',  ( 9.999999999999996447, -5.773502691896262640, -64.00000000409679046 ) ) ;
#26667=CARTESIAN_POINT ( 'NONE',  ( -2.121150477449813534E-15, -11.54700538379251284, -179.3750000000000000 ) ) ;
#26670=CARTESIAN_POINT ( 'NONE',  ( -5.405949406250003975, -9.363379034771801557, -56.03125000204836681 ) ) ;
#26674=CARTESIAN_POINT ( 'NONE',  ( -5.405949406250003975, -9.363379034771801557, -188.0312500020484094 ) ) ;
#26676=CARTESIAN_POINT ( 'NONE',  ( 4.999999999999992006, -8.660254037844389075, -172.1250000040968189 ) ) ;
#26677=CARTESIAN_POINT ( 'NONE',  ( -2.121150477449813534E-15, -11.54700538379251284, -117.8749999999999858 ) ) ;
#26678=LINE ( 'NONE', #10262, #41449 ) ;
#26679=LINE ( 'NONE', #26262, #36918 ) ;
#26680=CARTESIAN_POINT ( 'NONE',  ( -9.999999999999998224, 5.773502691896259087, -167.8749999999999716 ) ) ;
#26681=DIRECTION ( 'NONE',  ( -0.000000000000000000, -0.000000000000000000, 1.000000000000000000 ) ) ;
#26682=CARTESIAN_POINT ( 'NONE',  ( -10.81189881249999729, 1.324075727343319199E-15, -93.78125000204838102 ) ) ;
#26683=ORIENTED_EDGE ( 'NONE', *, *, #11564, .T. ) ;
#26684=CARTESIAN_POINT ( 'NONE',  ( -4.999999999999996447, 8.660254037844387298, -106.8750000040967763 ) ) ;
#26686=ORIENTED_EDGE ( 'NONE', *, *, #4445, .T. ) ;
#26687=ORIENTED_EDGE ( 'NONE', *, *, #2237, .T. ) ;
#26688=CARTESIAN_POINT ( 'NONE',  ( 7.644554776091147741E-16, 12.48450537969573659, -33.96875000204834549 ) ) ;
#26689=CARTESIAN_POINT ( 'NONE',  ( -2.293366432827344421E-15, -12.48450537969573659, -22.90625000204837747 ) ) ;
#26690=CARTESIAN_POINT ( 'NONE',  ( 10.81189881249999907, 6.242252689847868297, -68.71875000204838102 ) ) ;
#26692=EDGE_CURVE ( 'NONE', #37209, #3867, #28073, .T. ) ;
#26693=CARTESIAN_POINT ( 'NONE',  ( -10.81189881249999729, 6.242252689847871849, -195.7187500020484379 ) ) ;
#26694=CARTESIAN_POINT ( 'NONE',  ( -5.405949406249996869, 9.363379034771805109, -150.8437500020483810 ) ) ;
#26695=ADVANCED_FACE ( 'NONE', ( #8218 ), #1749, .T. ) ;
#26696=CARTESIAN_POINT ( 'NONE',  ( 9.999999999999479527, 5.773502691896553074, -99.37499999999995737 ) ) ;
#26697=CARTESIAN_POINT ( 'NONE',  ( -10.00000000000076916, 5.773502691895813221, -112.3749999999999858 ) ) ;
#26699=CARTESIAN_POINT ( 'NONE',  ( -2.121150477449813534E-15, -11.54700538379251284, 0.2499999959032573882 ) ) ;
#26700=CARTESIAN_POINT ( 'NONE',  ( 7.644554776091147741E-16, 12.48450537969573659, -123.9687500020483952 ) ) ;
#26702=CARTESIAN_POINT ( 'NONE',  ( -5.405949406249996869, 9.363379034771805109, -94.03125000204838102 ) ) ;
#26703=CARTESIAN_POINT ( 'NONE',  ( -2.293366432827344421E-15, -12.48450537969573659, -106.7187500020483668 ) ) ;
#26706=CARTESIAN_POINT ( 'NONE',  ( -4.999999999999996447, 8.660254037844387298, -159.3750000040967905 ) ) ;
#26710=CARTESIAN_POINT ( 'NONE',  ( 4.999999999999992006, -8.660254037844389075, -189.7500000000000000 ) ) ;
#26712=DIRECTION ( 'NONE',  ( -0.000000000000000000, -0.000000000000000000, 1.000000000000000000 ) ) ;
#26714=CARTESIAN_POINT ( 'NONE',  ( -9.999999999999998224, 1.224646799147353059E-15, -82.24999999999998579 ) ) ;
#26716=CARTESIAN_POINT ( 'NONE',  ( 9.999999999999996447, -5.773502691896262640, -89.50000000409676204 ) ) ;
#26717=CARTESIAN_POINT ( 'NONE',  ( -9.999999999999996447, 5.773502691896259975, -168.2500000040968189 ) ) ;
#26719=CARTESIAN_POINT ( 'NONE',  ( 5.405949406249992428, -9.363379034771808662, -87.28125000204838102 ) ) ;
#26720=VERTEX_POINT ( 'NONE', #14876 ) ;
#26722=CYLINDRICAL_SURFACE ( 'NONE', #11216, 9.999999999999998224 ) ;
#26724=VERTEX_POINT ( 'NONE', #14899 ) ;
#26725=CARTESIAN_POINT ( 'NONE',  ( -9.999999999999998224, 5.773502691896259087, -5.874999999999963585 ) ) ;
#26726=CARTESIAN_POINT ( 'NONE',  ( 9.999999999999996447, -5.773502691896262640, -141.6250000000000000 ) ) ;
#26727=LINE ( 'NONE', #211, #1390 ) ;
#26728=EDGE_CURVE ( 'NONE', #11948, #14436, #28098, .T. ) ;
#26730=CARTESIAN_POINT ( 'NONE',  ( -9.999999999999998224, 1.224646799147353059E-15, -193.2500000000000000 ) ) ;
#26731=CARTESIAN_POINT ( 'NONE',  ( 9.999999999999479527, 5.773502691896553074, -96.37499999999997158 ) ) ;
#26732=CARTESIAN_POINT ( 'NONE',  ( 5.405949406249992428, -9.363379034771808662, -118.7812500020483952 ) ) ;
#26733=ORIENTED_EDGE ( 'NONE', *, *, #538, .F. ) ;
#26735=CARTESIAN_POINT ( 'NONE',  ( -10.00000000000102496, 5.773502691895664007, -22.75000000409674072 ) ) ;
#26736=AXIS2_PLACEMENT_3D ( 'NONE', #33187, #10074, #10280 ) ;
#26738=ORIENTED_EDGE ( 'NONE', *, *, #40405, .F. ) ;
#26739=CARTESIAN_POINT ( 'NONE',  ( 5.405949406249992428, -9.363379034771808662, -45.28125000204838102 ) ) ;
#26741=CARTESIAN_POINT ( 'NONE',  ( 10.81189881249999907, 6.242252689847868297, -95.71875000204838102 ) ) ;
#26742=CARTESIAN_POINT ( 'NONE',  ( 7.644554776091147741E-16, 12.48450537969573659, -127.1562500020483810 ) ) ;
#26743=ADVANCED_FACE ( 'NONE', ( #24652 ), #41864, .T. ) ;
#26745=CARTESIAN_POINT ( 'NONE',  ( 9.999999999999998224, 0.000000000000000000, -132.5000000000000000 ) ) ;
#26746=CARTESIAN_POINT ( 'NONE',  ( 5.000000000000000000, 8.660254037844385522, -78.24999999999998579 ) ) ;
#26747=EDGE_CURVE ( 'NONE', #17891, #18350, #3087, .T. ) ;
#26749=CARTESIAN_POINT ( 'NONE',  ( 7.070501591499376803E-16, 11.54700538379251284, -14.00000000409676382 ) ) ;
#26751=CARTESIAN_POINT ( 'NONE',  ( 7.644554776091147741E-16, 12.48450537969573659, -134.4687500020483810 ) ) ;
#26753=CARTESIAN_POINT ( 'NONE',  ( -2.121150477449813534E-15, -11.54700538379251284, -44.37499999999997158 ) ) ;
#26755=CARTESIAN_POINT ( 'NONE',  ( -9.999999999999998224, 5.773502691896259087, -183.2500000040968189 ) ) ;
#26757=CARTESIAN_POINT ( 'NONE',  ( 10.81189881249999729, 0.000000000000000000, -181.5312500020483810 ) ) ;
#26758=CARTESIAN_POINT ( 'NONE',  ( -9.999999999999998224, 1.224646799147353059E-15, -2.749999999999974687 ) ) ;
#26759=LINE ( 'NONE', #37100, #3837 ) ;
#26761=CARTESIAN_POINT ( 'NONE',  ( 10.81189881249999551, -6.242252689847874514, -58.46875000204836681 ) ) ;
#26762=CARTESIAN_POINT ( 'NONE',  ( 10.81189881249999907, 6.242252689847868297, -43.21875000204835970 ) ) ;
#26764=CARTESIAN_POINT ( 'NONE',  ( -10.81189881249999907, -6.242252689847864744, -17.15625000204838102 ) ) ;
#26768=CARTESIAN_POINT ( 'NONE',  ( -9.999999999999998224, 1.224646799147353059E-15, -107.7499999999999858 ) ) ;
#26771=CARTESIAN_POINT ( 'NONE',  ( 9.999999999999998224, 0.000000000000000000, -48.87500000409678336 ) ) ;
#26774=CARTESIAN_POINT ( 'NONE',  ( 10.81189881249999551, -6.242252689847874514, -108.1562500020483810 ) ) ;
#26776=EDGE_LOOP ( 'NONE', ( #35328, #15735, #27961, #36324 ) ) ;
#26777=CARTESIAN_POINT ( 'NONE',  ( 0.000000000000000000, 0.000000000000000000, -200.0000000000000000 ) ) ;
#26782=CARTESIAN_POINT ( 'NONE',  ( 4.999999999999992006, -8.660254037844389075, -30.74999999999997158 ) ) ;
#26783=CARTESIAN_POINT ( 'NONE',  ( -2.293366432827344421E-15, -12.48450537969573659, -31.90625000204835970 ) ) ;
#26786=( BOUNDED_CURVE ( )  B_SPLINE_CURVE ( 2, ( #5926, #32052, #2481, #32258, #12586, #15609, #32474 ),
 .UNSPECIFIED., .F., .F. ) 
 B_SPLINE_CURVE_WITH_KNOTS ( ( 3, 2, 2, 3 ),
 ( 0.5037313432835821558, 0.5049751243781095411, 0.5062189054726369264, 0.5074626865671643117 ),
 .UNSPECIFIED. ) 
 CURVE ( )  GEOMETRIC_REPRESENTATION_ITEM ( )  RATIONAL_B_SPLINE_CURVE ( ( 0.9999999999999880096, 0.8660254037844506980, 1.000000000000000000, 0.8660254037844387076, 1.000000000000000000, 0.8660254037844267172, 1.000000000000011990 ) ) 
 REPRESENTATION_ITEM ( '' )  );
#26787=LINE ( 'NONE', #21534, #10715 ) ;
#26788=CARTESIAN_POINT ( 'NONE',  ( -5.405949406250003975, -9.363379034771801557, -144.5312500020483810 ) ) ;
#26789=CARTESIAN_POINT ( 'NONE',  ( -9.999999999999479527, -5.773502691896549521, -124.1249999999999858 ) ) ;
#26790=ORIENTED_EDGE ( 'NONE', *, *, #20159, .T. ) ;
#26791=( BOUNDED_CURVE ( )  B_SPLINE_CURVE ( 2, ( #4545, #31749, #23610, #31102, #1534, #27857, #1752 ),
 .UNSPECIFIED., .F., .F. ) 
 B_SPLINE_CURVE_WITH_KNOTS ( ( 3, 2, 2, 3 ),
 ( 0.8246268656716420065, 0.8258706467661693917, 0.8271144278606967770, 0.8283582089552240513 ),
 .UNSPECIFIED. ) 
 CURVE ( )  GEOMETRIC_REPRESENTATION_ITEM ( )  RATIONAL_B_SPLINE_CURVE ( ( 0.9999999999999761302, 0.8660254037844625774, 1.000000000000000000, 0.8660254037844387076, 1.000000000000000000, 0.8660254037844148378, 1.000000000000023981 ) ) 
 REPRESENTATION_ITEM ( '' )  );
#26792=VERTEX_POINT ( 'NONE', #15536 ) ;
#26793=VECTOR ( 'NONE', #3306, 1000.000000000000000 ) ;
#26796=CARTESIAN_POINT ( 'NONE',  ( -10.81189881249999729, 1.324075727343319199E-15, -164.0937500020484094 ) ) ;
#26798=CARTESIAN_POINT ( 'NONE',  ( 7.644554776091147741E-16, 12.48450537969573659, -20.46875000204836326 ) ) ;
#26799=CARTESIAN_POINT ( 'NONE',  ( -9.999999999999998224, 1.224646799147353059E-15, -122.7500000000000000 ) ) ;
#26800=CARTESIAN_POINT ( 'NONE',  ( 10.00000000000000000, 5.773502691896255534, -171.3750000000000000 ) ) ;
#26801=CARTESIAN_POINT ( 'NONE',  ( 10.81189881249999551, -6.242252689847874514, -157.4687500020484379 ) ) ;
#26802=CARTESIAN_POINT ( 'NONE',  ( 5.405949406249992428, -9.363379034771808662, -135.0937500020483810 ) ) ;
#26807=CARTESIAN_POINT ( 'NONE',  ( -10.81189881249999729, 1.324075727343319199E-15, -9.593750002048345493 ) ) ;
#26809=CARTESIAN_POINT ( 'NONE',  ( 9.999999999999998224, 0.000000000000000000, -165.8750000040967905 ) ) ;
#26810=CARTESIAN_POINT ( 'NONE',  ( 9.999999999999998224, 0.000000000000000000, -195.8750000040967905 ) ) ;
#26812=ADVANCED_FACE ( 'NONE', ( #34787 ), #9083, .T. ) ;
#26813=CARTESIAN_POINT ( 'NONE',  ( -2.293366432827344421E-15, -12.48450537969573659, -81.21875000204838102 ) ) ;
#26814=CARTESIAN_POINT ( 'NONE',  ( -10.81189881249999907, -6.242252689847864744, -76.96875000204836681 ) ) ;
#26815=CARTESIAN_POINT ( 'NONE',  ( 10.81189881249999729, 0.000000000000000000, -43.53125000204838102 ) ) ;
#26817=CARTESIAN_POINT ( 'NONE',  ( 4.999999999999992006, -8.660254037844389075, -113.6250000040967763 ) ) ;
#26819=CARTESIAN_POINT ( 'NONE',  ( 9.999999999999996447, -5.773502691896262640, -129.6250000000000000 ) ) ;
#26820=CARTESIAN_POINT ( 'NONE',  ( 5.405949406249992428, -9.363379034771808662, -135.2812500020483810 ) ) ;
#26822=CARTESIAN_POINT ( 'NONE',  ( 10.81189881249999729, 6.242252689847867408, -16.40625000204838102 ) ) ;
#26827=CARTESIAN_POINT ( 'NONE',  ( 5.000000000000000000, 8.660254037844385522, -41.12500000409677625 ) ) ;
#26831=CARTESIAN_POINT ( 'NONE',  ( -5.405949406250003975, -9.363379034771801557, -164.0312500020484094 ) ) ;
#26833=CARTESIAN_POINT ( 'NONE',  ( -10.81189881249999907, -6.242252689847864744, -133.9687500020483810 ) ) ;
#26834=CARTESIAN_POINT ( 'NONE',  ( -2.121150477449813534E-15, -11.54700538379251284, -80.75000000409677625 ) ) ;
#26835=CARTESIAN_POINT ( 'NONE',  ( 5.000000000000000000, 8.660254037844385522, -151.7500000000000000 ) ) ;
#26836=ORIENTED_EDGE ( 'NONE', *, *, #10650, .T. ) ;
#26837=CARTESIAN_POINT ( 'NONE',  ( 5.000000000000000000, 8.660254037844385522, -114.6250000040967763 ) ) ;
#26838=VECTOR ( 'NONE', #21235, 1000.000000000000000 ) ;
#26839=CARTESIAN_POINT ( 'NONE',  ( 10.81189881249999907, 6.242252689847868297, -65.90625000204839523 ) ) ;
#26840=ORIENTED_EDGE ( 'NONE', *, *, #41781, .F. ) ;
#26842=CARTESIAN_POINT ( 'NONE',  ( 7.644554776091147741E-16, 12.48450537969573659, -120.9687500020483952 ) ) ;
#26843=ORIENTED_EDGE ( 'NONE', *, *, #25344, .T. ) ;
#26844=CARTESIAN_POINT ( 'NONE',  ( 5.405949406249999534, 9.363379034771803333, -23.59375000204835970 ) ) ;
#26845=CARTESIAN_POINT ( 'NONE',  ( 10.81189881249999907, 6.242252689847868297, -197.7187500020484094 ) ) ;
#26846=CARTESIAN_POINT ( 'NONE',  ( -10.81189881249999729, 6.242252689847871849, -48.71875000204835970 ) ) ;
#26847=DIRECTION ( 'NONE',  ( 1.000000000000000000, 0.000000000000000000, 0.000000000000000000 ) ) ;
#26848=CARTESIAN_POINT ( 'NONE',  ( -9.999999999999998224, 1.224646799147353059E-15, -31.62500000409676559 ) ) ;
#26849=CARTESIAN_POINT ( 'NONE',  ( -5.405949406249996869, 9.363379034771805109, -176.3437500020483810 ) ) ;
#26850=CARTESIAN_POINT ( 'NONE',  ( 7.644554776091147741E-16, 12.48450537969573659, -159.9687500020483810 ) ) ;
#26851=( BOUNDED_CURVE ( )  B_SPLINE_CURVE ( 2, ( #24185, #10990, #4527, #13793, #30864, #33897, #21136 ),
 .UNSPECIFIED., .F., .F. ) 
 B_SPLINE_CURVE_WITH_KNOTS ( ( 3, 2, 2, 3 ),
 ( 0.1529850746268656692, 0.1542288557213930267, 0.1554726368159203842, 0.1567164179104477695 ),
 .UNSPECIFIED. ) 
 CURVE ( )  GEOMETRIC_REPRESENTATION_ITEM ( )  RATIONAL_B_SPLINE_CURVE ( ( 1.000000000000000000, 0.8660254037844387076, 1.000000000000000000, 0.8660254037844387076, 1.000000000000000000, 0.8660254037844387076, 1.000000000000000000 ) ) 
 REPRESENTATION_ITEM ( '' )  );
#26855=DIRECTION ( 'NONE',  ( 1.000000000000000000, 0.000000000000000000, 0.000000000000000000 ) ) ;
#26858=CARTESIAN_POINT ( 'NONE',  ( 10.81189881249999551, -6.242252689847874514, -98.96875000204838102 ) ) ;
#26859=CARTESIAN_POINT ( 'NONE',  ( -8.675003188131697129, -4.974413003141672895, -0.0003472602639886801512 ) ) ;
#26860=CARTESIAN_POINT ( 'NONE',  ( -10.81189881249999729, 6.242252689847871849, -68.40625000204840944 ) ) ;
#26863=CARTESIAN_POINT ( 'NONE',  ( -2.293366432827344421E-15, -12.48450537969573659, -118.9062500020483952 ) ) ;
#26864=CARTESIAN_POINT ( 'NONE',  ( 10.81189881249999551, -6.242252689847874514, -159.1562500020484094 ) ) ;
#26866=CARTESIAN_POINT ( 'NONE',  ( 7.070501591499377789E-16, 11.54700538379251284, -138.5000000040967905 ) ) ;
#26868=ORIENTED_EDGE ( 'NONE', *, *, #14669, .F. ) ;
#26871=CARTESIAN_POINT ( 'NONE',  ( -10.81189881249999907, -6.242252689847864744, -188.1562500020484094 ) ) ;
#26873=EDGE_LOOP ( 'NONE', ( #6672, #40881, #30732, #3123 ) ) ;
#26874=CARTESIAN_POINT ( 'NONE',  ( -2.121150477449813534E-15, -11.54700538379251284, -60.87499999999998579 ) ) ;
#26876=CARTESIAN_POINT ( 'NONE',  ( 9.999999999999996447, -5.773502691896262640, -67.00000000409676204 ) ) ;
#26880=CARTESIAN_POINT ( 'NONE',  ( -10.81189881249999729, 6.242252689847871849, -57.90625000204837391 ) ) ;
#26883=FACE_OUTER_BOUND ( 'NONE', #32226, .T. ) ;
#26884=CARTESIAN_POINT ( 'NONE',  ( -10.81189881249999729, 6.242252689847871849, -186.9062500020484094 ) ) ;
#26887=CARTESIAN_POINT ( 'NONE',  ( 9.999999999999998224, 0.000000000000000000, -200.0000000000000000 ) ) ;
#26889=CARTESIAN_POINT ( 'NONE',  ( 9.999999999999998224, 0.000000000000000000, -200.0000000000000000 ) ) ;
#26891=CARTESIAN_POINT ( 'NONE',  ( 10.81189881249999551, -6.242252689847874514, -94.65625000204838102 ) ) ;
#26894=VERTEX_POINT ( 'NONE', #11452 ) ;
#26897=CARTESIAN_POINT ( 'NONE',  ( 5.405949406249992428, -9.363379034771808662, -22.59375000204835615 ) ) ;
#26898=CARTESIAN_POINT ( 'NONE',  ( -10.81189881249999729, 1.324075727343319199E-15, -20.28125000204836326 ) ) ;
#26899=CARTESIAN_POINT ( 'NONE',  ( -2.293366432827344421E-15, -12.48450537969573659, -73.71875000204835260 ) ) ;
#26902=CARTESIAN_POINT ( 'NONE',  ( -2.293366432827344421E-15, -12.48450537969573659, -192.2187500020484379 ) ) ;
#26903=CARTESIAN_POINT ( 'NONE',  ( 5.405949406249999534, 9.363379034771803333, -152.5937500020483810 ) ) ;
#26904=DIRECTION ( 'NONE',  ( -0.000000000000000000, -0.000000000000000000, -1.000000000000000000 ) ) ;
#26907=CARTESIAN_POINT ( 'NONE',  ( -2.121150477449813534E-15, -11.54700538379251284, -4.250000004096763817 ) ) ;
#26909=CARTESIAN_POINT ( 'NONE',  ( -10.81189881249999729, 6.242252689847871849, -123.7187500020483952 ) ) ;
#26910=DIRECTION ( 'NONE',  ( -0.000000000000000000, -0.000000000000000000, 1.000000000000000000 ) ) ;
#26911=CARTESIAN_POINT ( 'NONE',  ( -10.81189881249999729, 1.324075727343319199E-15, -90.78125000204838102 ) ) ;
#26912=CARTESIAN_POINT ( 'NONE',  ( 5.405949406249999534, 9.363379034771803333, -97.09375000204838102 ) ) ;
#26915=CARTESIAN_POINT ( 'NONE',  ( 4.999999999999992006, -8.660254037844389075, -163.1250000040967905 ) ) ;
#26918=CARTESIAN_POINT ( 'NONE',  ( -10.00000000000015987, 5.773502691896167605, -192.2500000040968473 ) ) ;
#26919=CARTESIAN_POINT ( 'NONE',  ( -9.999999999999998224, 1.224646799147353059E-15, -146.7500000000000000 ) ) ;
#26920=CARTESIAN_POINT ( 'NONE',  ( 9.999999999999998224, 0.000000000000000000, -108.4999999999999858 ) ) ;
#26922=CARTESIAN_POINT ( 'NONE',  ( -5.000000000000003553, -8.660254037844383745, -81.99999999999998579 ) ) ;
#26924=CARTESIAN_POINT ( 'NONE',  ( 10.00000000000000000, 5.773502691896255534, -87.75000000409677625 ) ) ;
#26925=VECTOR ( 'NONE', #4432, 1000.000000000000000 ) ;
#26926=CARTESIAN_POINT ( 'NONE',  ( 7.070501591499376803E-16, 11.54700538379251284, -168.5000000040967620 ) ) ;
#26928=CARTESIAN_POINT ( 'NONE',  ( -10.81189881249999729, 1.324075727343319199E-15, -81.78125000204839523 ) ) ;
#26932=ORIENTED_EDGE ( 'NONE', *, *, #10920, .F. ) ;
#26933=CARTESIAN_POINT ( 'NONE',  ( -5.000000000000003553, -8.660254037844383745, -12.99999999999995559 ) ) ;
#26935=EDGE_CURVE ( 'NONE', #22340, #26513, #20724, .T. ) ;
#26936=CARTESIAN_POINT ( 'NONE',  ( -10.00000000000000000, -5.773502691896251982, -148.1249999999999716 ) ) ;
#26937=DIRECTION ( 'NONE',  ( 1.000000000000000000, 0.000000000000000000, 0.000000000000000000 ) ) ;
#26939=EDGE_CURVE ( 'NONE', #20834, #28118, #39747, .T. ) ;
#26940=CARTESIAN_POINT ( 'NONE',  ( 10.00000000000000000, 5.773502691896255534, -192.3750000000000000 ) ) ;
#26942=CARTESIAN_POINT ( 'NONE',  ( 10.81189881249999907, 6.242252689847868297, -115.4062500020484094 ) ) ;
#26944=CARTESIAN_POINT ( 'NONE',  ( -10.00000000000154188, 5.773502691895366468, -13.37499999999992717 ) ) ;
#26946=VERTEX_POINT ( 'NONE', #1985 ) ;
#26947=CARTESIAN_POINT ( 'NONE',  ( -10.81189881249999729, 6.242252689847871849, -42.90625000204838102 ) ) ;
#26950=CARTESIAN_POINT ( 'NONE',  ( 10.81189881249999907, 6.242252689847868297, -92.71875000204836681 ) ) ;
#26951=CARTESIAN_POINT ( 'NONE',  ( 10.81189881249999729, 6.242252689847867408, -119.9062500020483810 ) ) ;
#26952=ORIENTED_EDGE ( 'NONE', *, *, #19280, .T. ) ;
#26953=CARTESIAN_POINT ( 'NONE',  ( 9.999999999999998224, 0.000000000000000000, -51.87500000409675494 ) ) ;
#26954=CARTESIAN_POINT ( 'NONE',  ( -2.293366432827344421E-15, -12.48450537969573659, -198.2187500020484094 ) ) ;
#26957=CARTESIAN_POINT ( 'NONE',  ( -2.293366432827344421E-15, -12.48450537969573659, -133.7187500020483810 ) ) ;
#26960=CARTESIAN_POINT ( 'NONE',  ( -9.999999999999998224, 1.224646799147353059E-15, -183.1250000040967905 ) ) ;
#26962=CARTESIAN_POINT ( 'NONE',  ( -5.405949406250003975, -9.363379034771801557, -176.0312500020483810 ) ) ;
#26966=CARTESIAN_POINT ( 'NONE',  ( 10.81189881249999551, -6.242252689847874514, -61.46875000204838813 ) ) ;
#26967=CARTESIAN_POINT ( 'NONE',  ( -10.81189881249999729, 6.242252689847871849, -41.21875000204834549 ) ) ;
#26969=CARTESIAN_POINT ( 'NONE',  ( 5.405949406249999534, 9.363379034771803333, -16.28125000204835970 ) ) ;
#26973=CARTESIAN_POINT ( 'NONE',  ( -4.999999999999996447, 8.660254037844387298, -107.9999999999999858 ) ) ;
#26975=DIRECTION ( 'NONE',  ( -0.000000000000000000, -0.000000000000000000, 1.000000000000000000 ) ) ;
#26978=CARTESIAN_POINT ( 'NONE',  ( 5.405949406249992428, -9.363379034771808662, -109.7812500020483810 ) ) ;
#26980=VECTOR ( 'NONE', #18391, 1000.000000000000000 ) ;
#26981=CARTESIAN_POINT ( 'NONE',  ( 0.000000000000000000, 0.000000000000000000, -200.0000000000000000 ) ) ;
#26986=CARTESIAN_POINT ( 'NONE',  ( 7.070501591499377789E-16, 11.54700538379251284, -36.12499999999996447 ) ) ;
#26988=EDGE_CURVE ( 'NONE', #18833, #13430, #33718, .T. ) ;
#26990=CARTESIAN_POINT ( 'NONE',  ( 10.81189881249999729, 6.242252689847867408, -35.90625000204835260 ) ) ;
#26992=LINE ( 'NONE', #33913, #13160 ) ;
#26993=( BOUNDED_CURVE ( )  B_SPLINE_CURVE ( 2, ( #15673, #15465, #25838, #28666, #2962, #18932, #21748 ),
 .UNSPECIFIED., .F., .F. ) 
 B_SPLINE_CURVE_WITH_KNOTS ( ( 3, 2, 2, 3 ),
 ( 0.4291044776119404269, 0.4303482587064677567, 0.4315920398009951975, 0.4328358208955225273 ),
 .UNSPECIFIED. ) 
 CURVE ( )  GEOMETRIC_REPRESENTATION_ITEM ( )  RATIONAL_B_SPLINE_CURVE ( ( 0.9999999999999880096, 0.8660254037844506980, 1.000000000000000000, 0.8660254037844387076, 1.000000000000000000, 0.8660254037844207220, 1.000000000000017986 ) ) 
 REPRESENTATION_ITEM ( '' )  );
#26995=EDGE_CURVE ( 'NONE', #36343, #2376, #1710, .T. ) ;
#26996=EDGE_CURVE ( 'NONE', #41377, #17005, #16369, .T. ) ;
#26998=AXIS2_PLACEMENT_3D ( 'NONE', #10169, #17059, #20095 ) ;
#26999=CARTESIAN_POINT ( 'NONE',  ( 10.81189881249999907, 6.242252689847868297, -143.9062500020484094 ) ) ;
#27003=VERTEX_POINT ( 'NONE', #22669 ) ;
#27004=EDGE_CURVE ( 'NONE', #18939, #26093, #12924, .T. ) ;
#27005=CARTESIAN_POINT ( 'NONE',  ( -10.00000000000051337, 5.773502691895962435, -113.8749999999999858 ) ) ;
#27006=AXIS2_PLACEMENT_3D ( 'NONE', #13978, #33456, #30847 ) ;
#27007=CARTESIAN_POINT ( 'NONE',  ( -9.999999999999998224, 1.224646799147353059E-15, -147.1250000040967905 ) ) ;
#27008=CARTESIAN_POINT ( 'NONE',  ( 10.81189881249999729, 0.000000000000000000, -163.3437500020484094 ) ) ;
#27011=CARTESIAN_POINT ( 'NONE',  ( 7.644554776091147741E-16, 12.48450537969573659, -18.96875000204837391 ) ) ;
#27012=CARTESIAN_POINT ( 'NONE',  ( -4.999999999999996447, 8.660254037844387298, -171.0000000000000000 ) ) ;
#27013=CARTESIAN_POINT ( 'NONE',  ( -5.405949406250003975, -9.363379034771801557, -154.8437500020483810 ) ) ;
#27014=CARTESIAN_POINT ( 'NONE',  ( -10.81189881249999729, 6.242252689847871849, -137.2187500020483810 ) ) ;
#27019=( BOUNDED_CURVE ( )  B_SPLINE_CURVE ( 2, ( #2968, #28462, #8599, #16095, #41595, #38367, #18937 ),
 .UNSPECIFIED., .F., .F. ) 
 B_SPLINE_CURVE_WITH_KNOTS ( ( 3, 2, 2, 3 ),
 ( 0.1753731343283582433, 0.1766169154228856009, 0.1778606965174129861, 0.1791044776119403437 ),
 .UNSPECIFIED. ) 
 CURVE ( )  GEOMETRIC_REPRESENTATION_ITEM ( )  RATIONAL_B_SPLINE_CURVE ( ( 0.9999999999999970024, 0.8660254037844417052, 1.000000000000000000, 0.8660254037844387076, 1.000000000000000000, 0.8660254037844327124, 1.000000000000005995 ) ) 
 REPRESENTATION_ITEM ( '' )  );
#27020=CARTESIAN_POINT ( 'NONE',  ( -5.405949406250003975, -9.363379034771801557, -7.843750002048343717 ) ) ;
#27022=CARTESIAN_POINT ( 'NONE',  ( 10.81189881249999729, 6.242252689847867408, -199.4062500020484379 ) ) ;
#27027=CARTESIAN_POINT ( 'NONE',  ( -10.81189881249999729, -6.242252689847864744, -85.96875000204836681 ) ) ;
#27028=CARTESIAN_POINT ( 'NONE',  ( 5.405949406249992428, -9.363379034771808662, -67.59375000204836681 ) ) ;
#27030=CARTESIAN_POINT ( 'NONE',  ( 10.81189881249999729, 0.000000000000000000, -42.03125000204838102 ) ) ;
#27032=CARTESIAN_POINT ( 'NONE',  ( 10.81189881249999729, 0.000000000000000000, -199.3437500020484094 ) ) ;
#27034=CARTESIAN_POINT ( 'NONE',  ( 5.000000000000000000, 8.660254037844385522, -130.7499999999999716 ) ) ;
#27035=CARTESIAN_POINT ( 'NONE',  ( -5.405949406250003975, -9.363379034771801557, -128.0312500020484094 ) ) ;
#27036=EDGE_CURVE ( 'NONE', #39976, #22389, #14919, .T. ) ;
#27037=CARTESIAN_POINT ( 'NONE',  ( 9.999999999999998224, 0.000000000000000000, -94.99999999999998579 ) ) ;
#27039=CARTESIAN_POINT ( 'NONE',  ( 10.81189881249999729, 6.242252689847867408, -19.40625000204837747 ) ) ;
#27045=CARTESIAN_POINT ( 'NONE',  ( 4.999999999999992006, -8.660254037844389075, -44.62500000409677625 ) ) ;
#27046=CARTESIAN_POINT ( 'NONE',  ( 10.00000000000102318, -5.773502691895667560, -58.00000000409673362 ) ) ;
#27049=( BOUNDED_CURVE ( )  B_SPLINE_CURVE ( 2, ( #20767, #33956, #4378, #30716, #11048, #41682, #9107 ),
 .UNSPECIFIED., .F., .F. ) 
 B_SPLINE_CURVE_WITH_KNOTS ( ( 3, 2, 2, 3 ),
 ( 0.9477611940298510396, 0.9490049751243784248, 0.9502487562189058101, 0.9514925373134331954 ),
 .UNSPECIFIED. ) 
 CURVE ( )  GEOMETRIC_REPRESENTATION_ITEM ( )  RATIONAL_B_SPLINE_CURVE ( ( 0.9999999999999641398, 0.8660254037844745678, 1.000000000000000000, 0.8660254037844387076, 1.000000000000000000, 0.8660254037844028474, 1.000000000000035971 ) ) 
 REPRESENTATION_ITEM ( '' )  );
#27050=CARTESIAN_POINT ( 'NONE',  ( 10.00000000000102318, -5.773502691895667560, -40.00000000409673362 ) ) ;
#27051=CARTESIAN_POINT ( 'NONE',  ( -5.405949406250003975, -9.363379034771801557, -153.5312500020484094 ) ) ;
#27052=CARTESIAN_POINT ( 'NONE',  ( -5.405949406250003975, -9.363379034771801557, -138.3437500020484094 ) ) ;
#27053=CARTESIAN_POINT ( 'NONE',  ( -2.121150477449813534E-15, -11.54700538379251284, -195.8750000000000284 ) ) ;
#27054=ORIENTED_EDGE ( 'NONE', *, *, #9872, .F. ) ;
#27056=EDGE_CURVE ( 'NONE', #36297, #22119, #33022, .T. ) ;
#27057=CARTESIAN_POINT ( 'NONE',  ( -5.405949406249996869, 9.363379034771805109, -61.03125000204837391 ) ) ;
#27058=ORIENTED_EDGE ( 'NONE', *, *, #9872, .T. ) ;
#27060=CARTESIAN_POINT ( 'NONE',  ( 10.81189881249999551, -6.242252689847874514, -113.9687500020483810 ) ) ;
#27061=ORIENTED_EDGE ( 'NONE', *, *, #37295, .F. ) ;
#27062=CARTESIAN_POINT ( 'NONE',  ( -10.81189881249999729, 6.242252689847871849, -18.71875000204837036 ) ) ;
#27063=CARTESIAN_POINT ( 'NONE',  ( 10.81189881249999551, -6.242252689847874514, -193.4687500020484094 ) ) ;
#27064=CARTESIAN_POINT ( 'NONE',  ( 5.405949406249999534, 9.363379034771803333, -50.59375000204835260 ) ) ;
#27065=CARTESIAN_POINT ( 'NONE',  ( -10.00000000000102496, 5.773502691895664007, -61.75000000409674783 ) ) ;
#27066=CARTESIAN_POINT ( 'NONE',  ( 10.00000000000102318, -5.773502691895667560, -31.00000000409671586 ) ) ;
#27067=CARTESIAN_POINT ( 'NONE',  ( -5.405949406249996869, 9.363379034771805109, -179.3437500020483810 ) ) ;
#27068=CARTESIAN_POINT ( 'NONE',  ( 10.81189881249999907, 6.242252689847868297, -161.7187500020483810 ) ) ;
#27071=CARTESIAN_POINT ( 'NONE',  ( -9.999999999999998224, 1.224646799147353059E-15, -86.74999999999998579 ) ) ;
#27074=CARTESIAN_POINT ( 'NONE',  ( 10.81189881249999907, 6.242252689847868297, -89.71875000204836681 ) ) ;
#27075=CARTESIAN_POINT ( 'NONE',  ( -2.121150477449813534E-15, -11.54700538379251284, -72.87499999999997158 ) ) ;
#27076=CARTESIAN_POINT ( 'NONE',  ( 10.81189881249999729, 0.000000000000000000, -66.03125000204838102 ) ) ;
#27079=CARTESIAN_POINT ( 'NONE',  ( -5.405949406249996869, 9.363379034771805109, -125.5312500020483952 ) ) ;
#27080=CARTESIAN_POINT ( 'NONE',  ( 5.405949406249992428, -9.363379034771808662, -162.2812500020484094 ) ) ;
#27082=CARTESIAN_POINT ( 'NONE',  ( -2.121150477449813534E-15, -11.54700538379251284, -136.2500000040967620 ) ) ;
#27087=CARTESIAN_POINT ( 'NONE',  ( -2.293366432827344421E-15, -12.48450537969573659, -186.4062500020484094 ) ) ;
#27089=ORIENTED_EDGE ( 'NONE', *, *, #7198, .F. ) ;
#27090=CARTESIAN_POINT ( 'NONE',  ( 10.00000000000000000, 5.773502691896255534, -51.37499999999999289 ) ) ;
#27092=CARTESIAN_POINT ( 'NONE',  ( -9.999999999999998224, 1.224646799147353059E-15, -63.12500000409676204 ) ) ;
#27094=CARTESIAN_POINT ( 'NONE',  ( 4.999999999999992006, -8.660254037844389075, -165.7500000000000000 ) ) ;
#27096=CARTESIAN_POINT ( 'NONE',  ( 10.81189881249999551, -6.242252689847874514, -63.15625000204837391 ) ) ;
#27099=CARTESIAN_POINT ( 'NONE',  ( -10.00000000000102496, 5.773502691895664007, -88.37499999999997158 ) ) ;
#27100=CARTESIAN_POINT ( 'NONE',  ( -10.81189881249999729, 6.242252689847871849, -176.4062500020484094 ) ) ;
#27102=CARTESIAN_POINT ( 'NONE',  ( 4.999999999999992006, -8.660254037844389075, -73.12500000409677625 ) ) ;
#27103=CARTESIAN_POINT ( 'NONE',  ( 9.999999999999998224, 0.000000000000000000, -48.87500000409678336 ) ) ;
#27106=CARTESIAN_POINT ( 'NONE',  ( 9.999999999999998224, 0.000000000000000000, -122.0000000000000000 ) ) ;
#27107=ADVANCED_FACE ( 'NONE', ( #32399, #42291 ), #19628, .F. ) ;
#27108=CARTESIAN_POINT ( 'NONE',  ( 7.644554776091147741E-16, 12.48450537969573659, -85.15625000204838102 ) ) ;
#27109=ORIENTED_EDGE ( 'NONE', *, *, #10646, .F. ) ;
#27113=ORIENTED_EDGE ( 'NONE', *, *, #3754, .T. ) ;
#27114=CARTESIAN_POINT ( 'NONE',  ( 7.644554776091147741E-16, 12.48450537969573659, -26.46875000204837747 ) ) ;
#27115=CARTESIAN_POINT ( 'NONE',  ( 10.81189881249999907, 6.242252689847868297, -13.40625000204836326 ) ) ;
#27117=CARTESIAN_POINT ( 'NONE',  ( 5.405949406249999534, 9.363379034771803333, -70.09375000204836681 ) ) ;
#27121=CARTESIAN_POINT ( 'NONE',  ( -5.405949406250003975, -9.363379034771801557, -181.8437500020483810 ) ) ;
#27122=ADVANCED_FACE ( 'NONE', ( #39273 ), #25910, .T. ) ;
#27123=CYLINDRICAL_SURFACE ( 'NONE', #26736, 9.999999999999998224 ) ;
#27124=CARTESIAN_POINT ( 'NONE',  ( -4.999999999999996447, 8.660254037844387298, -141.0000000000000000 ) ) ;
#27126=CARTESIAN_POINT ( 'NONE',  ( 5.405949406249992428, -9.363379034771808662, -109.5937500020483810 ) ) ;
#27127=CARTESIAN_POINT ( 'NONE',  ( 9.999999999999998224, 0.000000000000000000, -194.0000000000000000 ) ) ;
#27128=CARTESIAN_POINT ( 'NONE',  ( -5.405949406250003975, -9.363379034771801557, -90.53125000204838102 ) ) ;
#27129=CARTESIAN_POINT ( 'NONE',  ( 5.405949406249999534, 9.363379034771803333, -98.59375000204838102 ) ) ;
#27132=CARTESIAN_POINT ( 'NONE',  ( -10.00000000000000000, -5.773502691896251982, -163.5000000040967620 ) ) ;
#27136=CARTESIAN_POINT ( 'NONE',  ( -9.999999999999479527, -5.773502691896549521, -149.6249999999999716 ) ) ;
#27139=CARTESIAN_POINT ( 'NONE',  ( -9.999999999999998224, 1.224646799147353059E-15, -74.74999999999998579 ) ) ;
#27141=CARTESIAN_POINT ( 'NONE',  ( -9.999999999999998224, 5.773502691896259087, -93.25000000409677625 ) ) ;
#27142=CARTESIAN_POINT ( 'NONE',  ( -2.121150477449813534E-15, -11.54700538379251284, -95.75000000409677625 ) ) ;
#27144=CARTESIAN_POINT ( 'NONE',  ( -5.405949406249996869, 9.363379034771805109, -82.03125000204839523 ) ) ;
#27148=ORIENTED_EDGE ( 'NONE', *, *, #17095, .T. ) ;
#27149=CARTESIAN_POINT ( 'NONE',  ( 5.000000000000000000, 8.660254037844385522, -10.74999999999995381 ) ) ;
#27150=EDGE_CURVE ( 'NONE', #25371, #16036, #7241, .T. ) ;
#27152=CARTESIAN_POINT ( 'NONE',  ( -10.81189881249999729, 1.324075727343319199E-15, -9.593750002048345493 ) ) ;
#27154=CARTESIAN_POINT ( 'NONE',  ( -5.405949406250003975, -9.363379034771801557, -135.5312500020484094 ) ) ;
#27155=( BOUNDED_CURVE ( )  B_SPLINE_CURVE ( 2, ( #21080, #5116, #40703, #17613, #30808, #21723, #34906 ),
 .UNSPECIFIED., .F., .F. ) 
 B_SPLINE_CURVE_WITH_KNOTS ( ( 3, 2, 2, 3 ),
 ( 0.01119402985074628015, 0.01243781094527364461, 0.01368159203980100908, 0.01492537313432837180 ),
 .UNSPECIFIED. ) 
 CURVE ( )  GEOMETRIC_REPRESENTATION_ITEM ( )  RATIONAL_B_SPLINE_CURVE ( ( 0.9999999999999986677, 0.8660254037844400399, 1.000000000000000000, 0.8660254037844387076, 1.000000000000000000, 0.8660254037844372643, 1.000000000000001554 ) ) 
 REPRESENTATION_ITEM ( '' )  );
#27156=ADVANCED_FACE ( 'NONE', ( #29789 ), #230, .T. ) ;
#27157=CARTESIAN_POINT ( 'NONE',  ( 9.999999999999998224, 0.000000000000000000, -188.0000000000000000 ) ) ;
#27158=CARTESIAN_POINT ( 'NONE',  ( 5.000000000000000000, 8.660254037844385522, -96.24999999999998579 ) ) ;
#27159=CARTESIAN_POINT ( 'NONE',  ( -2.293366432827344421E-15, -12.48450537969573659, -106.9062500020483952 ) ) ;
#27160=ORIENTED_EDGE ( 'NONE', *, *, #20133, .T. ) ;
#27161=CARTESIAN_POINT ( 'NONE',  ( 9.999999999999998224, 0.000000000000000000, -36.87500000409676915 ) ) ;
#27163=ORIENTED_EDGE ( 'NONE', *, *, #713, .T. ) ;
#27164=CARTESIAN_POINT ( 'NONE',  ( 10.81189881249999729, 0.000000000000000000, -45.03125000204838102 ) ) ;
#27166=CARTESIAN_POINT ( 'NONE',  ( 5.405949406249992428, -9.363379034771808662, -99.09375000204838102 ) ) ;
#27167=CARTESIAN_POINT ( 'NONE',  ( -2.293366432827344421E-15, -12.48450537969573659, -124.9062500020483810 ) ) ;
#27169=CARTESIAN_POINT ( 'NONE',  ( 5.405949406249999534, 9.363379034771803333, -199.0937500020484094 ) ) ;
#27171=CARTESIAN_POINT ( 'NONE',  ( 4.999999999999992006, -8.660254037844389075, -138.7499999999999716 ) ) ;
#27173=CARTESIAN_POINT ( 'NONE',  ( 10.81189881249999729, 6.242252689847867408, -127.2187500020483810 ) ) ;
#27177=CARTESIAN_POINT ( 'NONE',  ( -4.999999999999996447, 8.660254037844387298, -189.3750000040967905 ) ) ;
#27179=CARTESIAN_POINT ( 'NONE',  ( -10.81189881249999729, -6.242252689847864744, -180.6562500020484094 ) ) ;
#27183=CARTESIAN_POINT ( 'NONE',  ( 7.644554776091147741E-16, 12.48450537969573659, -54.96875000204836681 ) ) ;
#27184=CARTESIAN_POINT ( 'NONE',  ( 10.81189881249999729, 0.000000000000000000, -38.84375000204837391 ) ) ;
#27186=CARTESIAN_POINT ( 'NONE',  ( 7.644554776091147741E-16, 12.48450537969573659, -10.15625000204837924 ) ) ;
#27190=CARTESIAN_POINT ( 'NONE',  ( 7.070501591499377789E-16, 11.54700538379251284, -97.62499999999997158 ) ) ;
#27192=DIRECTION ( 'NONE',  ( 1.000000000000000000, 0.000000000000000000, 0.000000000000000000 ) ) ;
#27195=CARTESIAN_POINT ( 'NONE',  ( -2.293366432827344421E-15, -12.48450537969573659, -105.4062500020483810 ) ) ;
#27196=ORIENTED_EDGE ( 'NONE', *, *, #39410, .T. ) ;
#27197=DIRECTION ( 'NONE',  ( -0.000000000000000000, -0.000000000000000000, 1.000000000000000000 ) ) ;
#27202=CARTESIAN_POINT ( 'NONE',  ( -10.00000000000000000, -5.773502691896251982, -37.12499999999995026 ) ) ;
#27203=CARTESIAN_POINT ( 'NONE',  ( -10.81189881249999729, 6.242252689847871849, -35.40625000204836681 ) ) ;
#27204=CARTESIAN_POINT ( 'NONE',  ( -9.999999999999998224, 1.224646799147353059E-15, -111.1250000040967763 ) ) ;
#27207=CARTESIAN_POINT ( 'NONE',  ( -10.81189881249999729, 1.324075727343319199E-15, -138.7812500020483810 ) ) ;
#27208=CARTESIAN_POINT ( 'NONE',  ( 9.999999999999998224, 0.000000000000000000, -119.3750000040967905 ) ) ;
#27209=VERTEX_POINT ( 'NONE', #20268 ) ;
#27210=ORIENTED_EDGE ( 'NONE', *, *, #1586, .F. ) ;
#27212=CARTESIAN_POINT ( 'NONE',  ( -5.405949406250003975, -9.363379034771801557, -163.8437500020484094 ) ) ;
#27213=AXIS2_PLACEMENT_3D ( 'NONE', #6654, #19804, #36431 ) ;
#27215=ADVANCED_FACE ( 'NONE', ( #40318 ), #20051, .T. ) ;
#27216=CARTESIAN_POINT ( 'NONE',  ( -2.293366432827344421E-15, -12.48450537969573659, -13.71875000204836503 ) ) ;
#27217=CARTESIAN_POINT ( 'NONE',  ( -9.999999999999998224, 1.224646799147353059E-15, -200.0000000000000000 ) ) ;
#27219=CARTESIAN_POINT ( 'NONE',  ( -2.293366432827344421E-15, -12.48450537969573659, -144.2187500020484094 ) ) ;
#27220=CARTESIAN_POINT ( 'NONE',  ( 10.81189881249999729, 0.000000000000000000, -140.8437500020483810 ) ) ;
#27221=EDGE_CURVE ( 'NONE', #38243, #6565, #39905, .T. ) ;
#27222=CARTESIAN_POINT ( 'NONE',  ( 10.81189881249999907, 6.242252689847868297, -106.4062500020483952 ) ) ;
#27226=CARTESIAN_POINT ( 'NONE',  ( -5.405949406249996869, 9.363379034771805109, -9.843750002048345493 ) ) ;
#27229=CARTESIAN_POINT ( 'NONE',  ( 9.999999999999998224, 0.000000000000000000, -11.37500000409674783 ) ) ;
#27232=CARTESIAN_POINT ( 'NONE',  ( 5.405949406249999534, 9.363379034771803333, -80.59375000204838102 ) ) ;
#27233=CARTESIAN_POINT ( 'NONE',  ( 10.81189881249999729, 0.000000000000000000, -62.84375000204836681 ) ) ;
#27235=CARTESIAN_POINT ( 'NONE',  ( 10.81189881249999729, 0.000000000000000000, -34.53125000204837391 ) ) ;
#27237=CARTESIAN_POINT ( 'NONE',  ( -10.00000000000031797, 5.773502691896072569, -185.8750000000000000 ) ) ;
#27239=CARTESIAN_POINT ( 'NONE',  ( 10.00000000000000000, 5.773502691896255534, -132.3750000000000000 ) ) ;
#27240=CARTESIAN_POINT ( 'NONE',  ( 7.644554776091147741E-16, 12.48450537969573659, -133.1562500020483810 ) ) ;
#27241=CARTESIAN_POINT ( 'NONE',  ( 0.000000000000000000, 0.000000000000000000, -220.0000000000000000 ) ) ;
#27242=VECTOR ( 'NONE', #2426, 1000.000000000000000 ) ;
#27244=CARTESIAN_POINT ( 'NONE',  ( -10.81189881249999729, -6.242252689847864744, -20.15625000204838102 ) ) ;
#27248=CARTESIAN_POINT ( 'NONE',  ( 5.000000000000000000, 8.660254037844385522, -32.12500000409676204 ) ) ;
#27252=DIRECTION ( 'NONE',  ( -0.000000000000000000, -0.000000000000000000, 1.000000000000000000 ) ) ;
#27253=CARTESIAN_POINT ( 'NONE',  ( -5.405949406249996869, 9.363379034771805109, -151.0312500020483810 ) ) ;
#27254=CARTESIAN_POINT ( 'NONE',  ( 7.644554776091147741E-16, 12.48450537969573659, -132.9687500020483810 ) ) ;
#27255=CARTESIAN_POINT ( 'NONE',  ( 9.999999999999998224, 0.000000000000000000, -3.875000004096768258 ) ) ;
#27256=EDGE_CURVE ( 'NONE', #2239, #684, #38126, .T. ) ;
#27257=ORIENTED_EDGE ( 'NONE', *, *, #36970, .T. ) ;
#27262=CARTESIAN_POINT ( 'NONE',  ( 7.644554776091147741E-16, 12.48450537969573659, -108.9687500020483952 ) ) ;
#27263=ORIENTED_EDGE ( 'NONE', *, *, #9831, .F. ) ;
#27264=AXIS2_PLACEMENT_3D ( 'NONE', #8713, #25546, #28785 ) ;
#27265=( BOUNDED_CURVE ( )  B_SPLINE_CURVE ( 2, ( #3603, #32952, #23235, #33171, #33593, #6826, #26470 ),
 .UNSPECIFIED., .F., .F. ) 
 B_SPLINE_CURVE_WITH_KNOTS ( ( 3, 2, 2, 3 ),
 ( 0.3022388059701494045, 0.3034825870646767343, 0.3047263681592040085, 0.3059701492537313383 ),
 .UNSPECIFIED. ) 
 CURVE ( )  GEOMETRIC_REPRESENTATION_ITEM ( )  RATIONAL_B_SPLINE_CURVE ( ( 0.9999999999999820144, 0.8660254037844566932, 1.000000000000000000, 0.8660254037844387076, 1.000000000000000000, 0.8660254037844387076, 1.000000000000000000 ) ) 
 REPRESENTATION_ITEM ( '' )  );
#27266=CARTESIAN_POINT ( 'NONE',  ( 7.070501591499376803E-16, 11.54700538379251284, -189.1250000000000000 ) ) ;
#27267=CARTESIAN_POINT ( 'NONE',  ( 10.81189881249999729, 0.000000000000000000, -190.3437500020484094 ) ) ;
#27268=AXIS2_PLACEMENT_3D ( 'NONE', #20197, #579, #4013 ) ;
#27269=CARTESIAN_POINT ( 'NONE',  ( -5.405949406250003975, -9.363379034771801557, -42.34375000204837391 ) ) ;
#27270=CARTESIAN_POINT ( 'NONE',  ( 2.525711100651609531, -10.23860432883650162, 1.566949817559350803E-14 ) ) ;
#27272=ADVANCED_FACE ( 'NONE', ( #13774 ), #862, .T. ) ;
#27273=CARTESIAN_POINT ( 'NONE',  ( 7.644554776091147741E-16, 12.48450537969573659, -174.9687500020484094 ) ) ;
#27275=CARTESIAN_POINT ( 'NONE',  ( 5.405949406249999534, 9.363379034771803333, -160.0937500020484094 ) ) ;
#27276=CARTESIAN_POINT ( 'NONE',  ( -9.999999999999998224, 1.224646799147353059E-15, -178.2500000000000284 ) ) ;
#27280=CARTESIAN_POINT ( 'NONE',  ( -9.999999999999998224, 1.224646799147353059E-15, -126.1250000040967620 ) ) ;
#27284=CARTESIAN_POINT ( 'NONE',  ( -10.81189881249999907, -6.242252689847864744, -87.46875000204838102 ) ) ;
#27286=CARTESIAN_POINT ( 'NONE',  ( -10.81189881249999729, 6.242252689847871849, -65.40625000204838102 ) ) ;
#27287=CARTESIAN_POINT ( 'NONE',  ( 5.000000000000000000, 8.660254037844385522, -146.1250000040967905 ) ) ;
#27289=CARTESIAN_POINT ( 'NONE',  ( -10.81189881249999729, 6.242252689847871849, -122.4062500020483952 ) ) ;
#27290=CARTESIAN_POINT ( 'NONE',  ( -10.81189881249999729, 6.242252689847871849, -155.4062500020483810 ) ) ;
#27293=CARTESIAN_POINT ( 'NONE',  ( 7.070501591499377789E-16, 11.54700538379251284, -131.0000000040967905 ) ) ;
#27295=ORIENTED_EDGE ( 'NONE', *, *, #37696, .T. ) ;
#27300=CARTESIAN_POINT ( 'NONE',  ( 5.405949406249999534, 9.363379034771803333, -191.7812500020484094 ) ) ;
#27301=ORIENTED_EDGE ( 'NONE', *, *, #35719, .T. ) ;
#27302=CARTESIAN_POINT ( 'NONE',  ( 9.999999999999998224, 0.000000000000000000, -46.99999999999998579 ) ) ;
#27304=CARTESIAN_POINT ( 'NONE',  ( -9.999999999999998224, 5.773502691896259087, -55.75000000409678336 ) ) ;
#27305=CARTESIAN_POINT ( 'NONE',  ( 4.999999999999992006, -8.660254037844389075, -179.2500000000000284 ) ) ;
#27308=AXIS2_PLACEMENT_3D ( 'NONE', #31014, #31233, #14789 ) ;
#27309=CARTESIAN_POINT ( 'NONE',  ( -10.81189881249999729, 6.242252689847871849, -62.40625000204838813 ) ) ;
#27310=EDGE_CURVE ( 'NONE', #33916, #5939, #36980, .T. ) ;
#27314=CARTESIAN_POINT ( 'NONE',  ( -5.405949406250003975, -9.363379034771801557, -176.0312500020483810 ) ) ;
#27317=CARTESIAN_POINT ( 'NONE',  ( -9.999999999999998224, 1.224646799147353059E-15, -197.7500000000000000 ) ) ;
#27319=CARTESIAN_POINT ( 'NONE',  ( -4.999999999999996447, 8.660254037844387298, -105.3750000040967763 ) ) ;
#27320=CYLINDRICAL_SURFACE ( 'NONE', #9642, 9.999999999999998224 ) ;
#27321=CARTESIAN_POINT ( 'NONE',  ( -5.405949406250003975, -9.363379034771801557, -84.53125000204838102 ) ) ;
#27322=VERTEX_POINT ( 'NONE', #2124 ) ;
#27324=ORIENTED_EDGE ( 'NONE', *, *, #23769, .T. ) ;
#27326=ORIENTED_EDGE ( 'NONE', *, *, #38108, .F. ) ;
#27327=CARTESIAN_POINT ( 'NONE',  ( 10.81189881249999729, 0.000000000000000000, -34.34375000204836681 ) ) ;
#27328=CARTESIAN_POINT ( 'NONE',  ( -5.405949406249996869, 9.363379034771805109, -27.84375000204836326 ) ) ;
#27329=CARTESIAN_POINT ( 'NONE',  ( 7.644554776091147741E-16, 12.48450537969573659, -13.15625000204836148 ) ) ;
#27330=CARTESIAN_POINT ( 'NONE',  ( -10.81189881249999907, -6.242252689847864744, -63.46875000204838102 ) ) ;
#27331=FACE_OUTER_BOUND ( 'NONE', #22787, .T. ) ;
#27333=CARTESIAN_POINT ( 'NONE',  ( -10.81189881249999907, -6.242252689847864744, -181.9687500020484094 ) ) ;
#27335=CARTESIAN_POINT ( 'NONE',  ( -5.405949406250003975, -9.363379034771801557, -1.843750002048366587 ) ) ;
#27336=CARTESIAN_POINT ( 'NONE',  ( -5.000000000000003553, -8.660254037844383745, -182.8750000040967905 ) ) ;
#27340=CARTESIAN_POINT ( 'NONE',  ( 10.81189881249999551, -6.242252689847874514, -116.9687500020483952 ) ) ;
#27341=CARTESIAN_POINT ( 'NONE',  ( 9.999999999998456346, 5.773502691897149042, -15.37499999999994138 ) ) ;
#27342=CARTESIAN_POINT ( 'NONE',  ( -10.81189881249999729, 1.324075727343319199E-15, -87.78125000204838102 ) ) ;
#27343=CARTESIAN_POINT ( 'NONE',  ( -2.293366432827344421E-15, -12.48450537969573659, -99.21875000204836681 ) ) ;
#27346=CARTESIAN_POINT ( 'NONE',  ( 10.00000000000000000, 5.773502691896255534, -156.7500000040967905 ) ) ;
#27350=EDGE_CURVE ( 'NONE', #23935, #21158, #41384, .T. ) ;
#27352=DIRECTION ( 'NONE',  ( -0.000000000000000000, -0.000000000000000000, 1.000000000000000000 ) ) ;
#27354=CARTESIAN_POINT ( 'NONE',  ( 7.070501591499376803E-16, 11.54700538379251284, -63.12499999999997158 ) ) ;
#27355=CARTESIAN_POINT ( 'NONE',  ( 7.070501591499377789E-16, 11.54700538379251284, -73.62499999999995737 ) ) ;
#27357=CARTESIAN_POINT ( 'NONE',  ( -5.000000000000003553, -8.660254037844383745, -89.87500000409677625 ) ) ;
#27358=CARTESIAN_POINT ( 'NONE',  ( -9.999999999999998224, 1.224646799147353059E-15, -172.2500000000000000 ) ) ;
#27360=CARTESIAN_POINT ( 'NONE',  ( 10.81189881249999551, -6.242252689847874514, -85.65625000204839523 ) ) ;
#27362=CARTESIAN_POINT ( 'NONE',  ( -4.999999999999996447, 8.660254037844387298, -19.49999999999996092 ) ) ;
#27364=ORIENTED_EDGE ( 'NONE', *, *, #1968, .F. ) ;
#27365=CARTESIAN_POINT ( 'NONE',  ( -10.00000000000000000, -5.773502691896251982, -2.624999999999948486 ) ) ;
#27367=CARTESIAN_POINT ( 'NONE',  ( -5.405949406250003975, -9.363379034771801557, -12.34375000204834905 ) ) ;
#27368=DIRECTION ( 'NONE',  ( -0.000000000000000000, -0.000000000000000000, 1.000000000000000000 ) ) ;
#27369=( BOUNDED_CURVE ( )  B_SPLINE_CURVE ( 2, ( #34151, #39962, #3936, #14033, #4569, #17711, #17074 ),
 .UNSPECIFIED., .F., .F. ) 
 B_SPLINE_CURVE_WITH_KNOTS ( ( 3, 2, 2, 3 ),
 ( 0.9626865671641793298, 0.9639303482587067151, 0.9651741293532341004, 0.9664179104477613746 ),
 .UNSPECIFIED. ) 
 CURVE ( )  GEOMETRIC_REPRESENTATION_ITEM ( )  RATIONAL_B_SPLINE_CURVE ( ( 0.9999999999999761302, 0.8660254037844625774, 1.000000000000000000, 0.8660254037844387076, 1.000000000000000000, 0.8660254037844148378, 1.000000000000023981 ) ) 
 REPRESENTATION_ITEM ( '' )  );
#27371=CARTESIAN_POINT ( 'NONE',  ( -5.405949406249996869, 9.363379034771805109, -127.0312500020483952 ) ) ;
#27372=EDGE_CURVE ( 'NONE', #30360, #29087, #24903, .T. ) ;
#27373=CARTESIAN_POINT ( 'NONE',  ( 7.070501591499377789E-16, 11.54700538379251284, -180.1250000000000000 ) ) ;
#27374=CARTESIAN_POINT ( 'NONE',  ( 9.999999999999998224, 0.000000000000000000, -144.8750000040967905 ) ) ;
#27375=CARTESIAN_POINT ( 'NONE',  ( -10.81189881249999729, 6.242252689847871849, -113.4062500020483810 ) ) ;
#27377=DIRECTION ( 'NONE',  ( -0.000000000000000000, -0.000000000000000000, 1.000000000000000000 ) ) ;
#27378=ORIENTED_EDGE ( 'NONE', *, *, #24260, .T. ) ;
#27379=ORIENTED_EDGE ( 'NONE', *, *, #39059, .F. ) ;
#27380=CARTESIAN_POINT ( 'NONE',  ( -2.293366432827344421E-15, -12.48450537969573659, -34.90625000204836681 ) ) ;
#27382=CARTESIAN_POINT ( 'NONE',  ( 5.405949406249992428, -9.363379034771808662, -91.59375000204838102 ) ) ;
#27383=CYLINDRICAL_SURFACE ( 'NONE', #32581, 9.999999999999998224 ) ;
#27385=CARTESIAN_POINT ( 'NONE',  ( 10.81189881249999729, 0.000000000000000000, -199.3437500020484094 ) ) ;
#27387=CARTESIAN_POINT ( 'NONE',  ( 5.000000000000000000, 8.660254037844385522, -138.2499999999999716 ) ) ;
#27388=CARTESIAN_POINT ( 'NONE',  ( 10.81189881249999729, 6.242252689847867408, -124.2187500020483952 ) ) ;
#27390=CARTESIAN_POINT ( 'NONE',  ( 7.644554776091147741E-16, 12.48450537969573659, -5.656250002048358816 ) ) ;
#27393=CARTESIAN_POINT ( 'NONE',  ( 5.000000000000000000, 8.660254037844385522, -180.6250000040967905 ) ) ;
#27395=CARTESIAN_POINT ( 'NONE',  ( -10.81189881249999729, 1.324075727343319199E-15, -177.7812500020484094 ) ) ;
#27400=CARTESIAN_POINT ( 'NONE',  ( -5.405949406249996869, 9.363379034771805109, -53.34375000204835970 ) ) ;
#27401=CARTESIAN_POINT ( 'NONE',  ( -10.81189881249999729, 6.242252689847871849, -42.71875000204835970 ) ) ;
#27403=CARTESIAN_POINT ( 'NONE',  ( 10.81189881249999907, 6.242252689847868297, -7.406250002048366810 ) ) ;
#27405=CARTESIAN_POINT ( 'NONE',  ( -9.999999999999479527, -5.773502691896549521, -124.5000000040967620 ) ) ;
#27407=CARTESIAN_POINT ( 'NONE',  ( 9.999999999999998224, 0.000000000000000000, -99.49999999999998579 ) ) ;
#27409=CARTESIAN_POINT ( 'NONE',  ( -5.000000000000003553, -8.660254037844383745, -116.8750000040967905 ) ) ;
#27410=CYLINDRICAL_SURFACE ( 'NONE', #9327, 9.999999999999998224 ) ;
#27413=CARTESIAN_POINT ( 'NONE',  ( 5.405949406249999534, 9.363379034771803333, -104.7812500020483810 ) ) ;
#27415=( BOUNDED_CURVE ( )  B_SPLINE_CURVE ( 2, ( #13876, #40630, #7642, #10861, #14518, #10647, #17975 ),
 .UNSPECIFIED., .F., .F. ) 
 B_SPLINE_CURVE_WITH_KNOTS ( ( 3, 2, 2, 3 ),
 ( 0.5261194029850747578, 0.5273631840796021431, 0.5286069651741294173, 0.5298507462686568026 ),
 .UNSPECIFIED. ) 
 CURVE ( )  GEOMETRIC_REPRESENTATION_ITEM ( )  RATIONAL_B_SPLINE_CURVE ( ( 0.9999999999999880096, 0.8660254037844506980, 1.000000000000000000, 0.8660254037844387076, 1.000000000000000000, 0.8660254037844267172, 1.000000000000011990 ) ) 
 REPRESENTATION_ITEM ( '' )  );
#27418=CARTESIAN_POINT ( 'NONE',  ( 7.070501591499376803E-16, 11.54700538379251284, -141.5000000040967905 ) ) ;
#27419=CARTESIAN_POINT ( 'NONE',  ( -5.405949406249996869, 9.363379034771805109, -166.0312500020484094 ) ) ;
#27422=CARTESIAN_POINT ( 'NONE',  ( 4.999999999999992006, -8.660254037844389075, -29.24999999999997158 ) ) ;
#27423=AXIS2_PLACEMENT_3D ( 'NONE', #24213, #13819, #4349 ) ;
#27424=CARTESIAN_POINT ( 'NONE',  ( 10.81189881249999551, -6.242252689847874514, -37.65625000204836681 ) ) ;
#27425=CARTESIAN_POINT ( 'NONE',  ( 9.999999999999996447, -5.773502691896262640, -164.1249999999999716 ) ) ;
#27426=VECTOR ( 'NONE', #28249, 1000.000000000000000 ) ;
#27427=EDGE_CURVE ( 'NONE', #36710, #12497, #29298, .T. ) ;
#27429=CARTESIAN_POINT ( 'NONE',  ( 5.405949406249999534, 9.363379034771803333, -131.7812500020483810 ) ) ;
#27430=CARTESIAN_POINT ( 'NONE',  ( -1.034724182395691638, 10.15477877528964257, -4.586030929915079049E-15 ) ) ;
#27431=CARTESIAN_POINT ( 'NONE',  ( 9.999999999999742428, 5.773502691896404748, -162.7500000040968189 ) ) ;
#27432=ORIENTED_EDGE ( 'NONE', *, *, #22293, .T. ) ;
#27433=VERTEX_POINT ( 'NONE', #41147 ) ;
#27436=CARTESIAN_POINT ( 'NONE',  ( 0.000000000000000000, 0.000000000000000000, -200.0000000000000000 ) ) ;
#27437=CARTESIAN_POINT ( 'NONE',  ( -5.405949406250003975, -9.363379034771801557, -166.8437500020484094 ) ) ;
#27439=CARTESIAN_POINT ( 'NONE',  ( -10.81189881249999729, 6.242252689847871849, -15.71875000204835793 ) ) ;
#27440=CARTESIAN_POINT ( 'NONE',  ( 9.999999999999998224, 0.000000000000000000, -75.49999999999998579 ) ) ;
#27442=CARTESIAN_POINT ( 'NONE',  ( 5.405949406249992428, -9.363379034771808662, -150.0937500020483810 ) ) ;
#27444=CARTESIAN_POINT ( 'NONE',  ( 7.644554776091147741E-16, 12.48450537969573659, -138.9687500020484094 ) ) ;
#27445=CARTESIAN_POINT ( 'NONE',  ( 10.81189881249999551, -6.242252689847874514, -108.1562500020483810 ) ) ;
#27449=CARTESIAN_POINT ( 'NONE',  ( 7.644554776091147741E-16, 12.48450537969573659, -12.96875000204836148 ) ) ;
#27451=CYLINDRICAL_SURFACE ( 'NONE', #30234, 9.999999999999998224 ) ;
#27455=CARTESIAN_POINT ( 'NONE',  ( 10.81189881249999729, 6.242252689847867408, -76.21875000204838102 ) ) ;
#27456=CARTESIAN_POINT ( 'NONE',  ( 10.81189881249999551, -6.242252689847874514, -61.46875000204838102 ) ) ;
#27458=CARTESIAN_POINT ( 'NONE',  ( -10.81189881249999729, 6.242252689847871849, -36.90625000204835970 ) ) ;
#27460=CARTESIAN_POINT ( 'NONE',  ( 9.999999999999998224, 0.000000000000000000, -200.0000000000000000 ) ) ;
#27462=CARTESIAN_POINT ( 'NONE',  ( -5.000000000000003553, -8.660254037844383745, -119.5000000000000000 ) ) ;
#27463=CARTESIAN_POINT ( 'NONE',  ( 10.81189881249999729, 0.000000000000000000, -132.0312500020484094 ) ) ;
#27464=CARTESIAN_POINT ( 'NONE',  ( -9.999999999999998224, 1.224646799147353059E-15, -187.6250000040967905 ) ) ;
#27466=CARTESIAN_POINT ( 'NONE',  ( 5.405949406249992428, -9.363379034771808662, -16.78125000204835970 ) ) ;
#27470=CARTESIAN_POINT ( 'NONE',  ( 9.999999999999998224, 0.000000000000000000, -33.87500000409676915 ) ) ;
#27474=CARTESIAN_POINT ( 'NONE',  ( -5.405949406250003975, -9.363379034771801557, -156.5312500020484094 ) ) ;
#27475=CARTESIAN_POINT ( 'NONE',  ( 10.81189881249999551, -6.242252689847874514, -128.9687500020483810 ) ) ;
#27476=CARTESIAN_POINT ( 'NONE',  ( -4.999999999999996447, 8.660254037844387298, -144.0000000000000000 ) ) ;
#27477=EDGE_CURVE ( 'NONE', #4157, #22331, #1454, .T. ) ;
#27479=ORIENTED_EDGE ( 'NONE', *, *, #41809, .F. ) ;
#27480=EDGE_CURVE ( 'NONE', #27322, #6831, #8646, .T. ) ;
#27481=CARTESIAN_POINT ( 'NONE',  ( -4.999999999999996447, 8.660254037844387298, -31.49999999999997158 ) ) ;
#27482=ORIENTED_EDGE ( 'NONE', *, *, #26747, .F. ) ;
#27483=ORIENTED_EDGE ( 'NONE', *, *, #16415, .T. ) ;
#27484=CARTESIAN_POINT ( 'NONE',  ( -10.81189881249999729, 6.242252689847871849, -113.2187500020483952 ) ) ;
#27486=CARTESIAN_POINT ( 'NONE',  ( -9.999999999998969713, -5.773502691896847949, -42.00000000409673362 ) ) ;
#27487=CARTESIAN_POINT ( 'NONE',  ( -10.81189881249999729, 1.324075727343319199E-15, -186.5937500020483810 ) ) ;
#27488=CARTESIAN_POINT ( 'NONE',  ( 5.405949406249992428, -9.363379034771808662, -42.09375000204837391 ) ) ;
#27489=CARTESIAN_POINT ( 'NONE',  ( -4.999999999999996447, 8.660254037844387298, -61.87500000409676204 ) ) ;
#27490=CARTESIAN_POINT ( 'NONE',  ( -9.999999999999998224, 1.224646799147353059E-15, -10.62500000409674605 ) ) ;
#27491=CARTESIAN_POINT ( 'NONE',  ( -10.81189881249999729, 1.324075727343319199E-15, -176.0937500020484094 ) ) ;
#27492=CARTESIAN_POINT ( 'NONE',  ( 10.81189881249999907, 6.242252689847868297, -157.2187500020483810 ) ) ;
#27493=CARTESIAN_POINT ( 'NONE',  ( 9.999999999999998224, 0.000000000000000000, -65.37500000409676204 ) ) ;
#27496=CARTESIAN_POINT ( 'NONE',  ( -10.00000000000076916, 5.773502691895813221, -126.2500000040967763 ) ) ;
#27499=CARTESIAN_POINT ( 'NONE',  ( 7.644554776091147741E-16, 12.48450537969573659, -86.46875000204838102 ) ) ;
#27500=CARTESIAN_POINT ( 'NONE',  ( 10.00000000000076916, -5.773502691895816774, -113.1249999999999716 ) ) ;
#27501=CARTESIAN_POINT ( 'NONE',  ( -10.81189881249999907, -6.242252689847864744, -62.15625000204838102 ) ) ;
#27502=CARTESIAN_POINT ( 'NONE',  ( -9.999999999999998224, 1.224646799147353059E-15, -87.12500000409677625 ) ) ;
#27504=CARTESIAN_POINT ( 'NONE',  ( 10.81189881249999551, -6.242252689847874514, -112.6562500020483810 ) ) ;
#27506=CARTESIAN_POINT ( 'NONE',  ( -10.81189881249999729, 1.324075727343319199E-15, -155.2812500020484094 ) ) ;
#27509=CARTESIAN_POINT ( 'NONE',  ( 7.070501591499377789E-16, 11.54700538379251284, -129.5000000040967620 ) ) ;
#27511=ORIENTED_EDGE ( 'NONE', *, *, #18294, .T. ) ;
#27515=VECTOR ( 'NONE', #41570, 1000.000000000000000 ) ;
#27516=CARTESIAN_POINT ( 'NONE',  ( -2.293366432827344421E-15, -12.48450537969573659, -189.4062500020484094 ) ) ;
#27518=CARTESIAN_POINT ( 'NONE',  ( -2.121150477449813534E-15, -11.54700538379251284, -45.87499999999996447 ) ) ;
#27520=CARTESIAN_POINT ( 'NONE',  ( 10.00000000000000000, 5.773502691896255534, -60.75000000409676915 ) ) ;
#27523=CARTESIAN_POINT ( 'NONE',  ( 5.405949406249992428, -9.363379034771808662, -48.28125000204838813 ) ) ;
#27525=AXIS2_PLACEMENT_3D ( 'NONE', #27928, #36777, #34623 ) ;
#27527=CARTESIAN_POINT ( 'NONE',  ( -10.81189881249999729, 1.324075727343319199E-15, -173.2812500020484094 ) ) ;
#27530=CARTESIAN_POINT ( 'NONE',  ( 10.00000000000051159, -5.773502691895965988, -81.62499999999995737 ) ) ;
#27531=ADVANCED_FACE ( 'NONE', ( #6200 ), #33385, .T. ) ;
#27533=CARTESIAN_POINT ( 'NONE',  ( -5.000000000000003553, -8.660254037844383745, -60.99999999999997158 ) ) ;
#27534=( BOUNDED_CURVE ( )  B_SPLINE_CURVE ( 2, ( #33387, #19769, #3382, #23451, #10266, #29717, #36600 ),
 .UNSPECIFIED., .F., .F. ) 
 B_SPLINE_CURVE_WITH_KNOTS ( ( 3, 2, 2, 3 ),
 ( 0.6828358208955226383, 0.6840796019900500236, 0.6853233830845772978, 0.6865671641791046831 ),
 .UNSPECIFIED. ) 
 CURVE ( )  GEOMETRIC_REPRESENTATION_ITEM ( )  RATIONAL_B_SPLINE_CURVE ( ( 0.9999999999999761302, 0.8660254037844625774, 1.000000000000000000, 0.8660254037844387076, 1.000000000000000000, 0.8660254037844148378, 1.000000000000023981 ) ) 
 REPRESENTATION_ITEM ( '' )  );
#27536=CARTESIAN_POINT ( 'NONE',  ( 10.00000000000102318, -5.773502691895667560, -20.12499999999993960 ) ) ;
#27537=CARTESIAN_POINT ( 'NONE',  ( 5.405949406249999534, 9.363379034771803333, -85.28125000204838102 ) ) ;
#27538=VERTEX_POINT ( 'NONE', #42428 ) ;
#27542=ORIENTED_EDGE ( 'NONE', *, *, #15090, .T. ) ;
#27543=CARTESIAN_POINT ( 'NONE',  ( -10.81189881249999729, 6.242252689847871849, -39.71875000204835970 ) ) ;
#27544=CARTESIAN_POINT ( 'NONE',  ( -10.81189881249999729, 6.242252689847871849, -24.71875000204837036 ) ) ;
#27545=CARTESIAN_POINT ( 'NONE',  ( -5.405949406250003975, -9.363379034771801557, -14.03125000204835615 ) ) ;
#27547=CARTESIAN_POINT ( 'NONE',  ( 10.81189881249999907, 6.242252689847868297, -61.21875000204838102 ) ) ;
#27548=DIRECTION ( 'NONE',  ( 1.000000000000000000, 0.000000000000000000, 0.000000000000000000 ) ) ;
#27550=CARTESIAN_POINT ( 'NONE',  ( -10.81189881249999729, 1.324075727343319199E-15, -185.0937500020483810 ) ) ;
#27553=CYLINDRICAL_SURFACE ( 'NONE', #28133, 9.999999999999998224 ) ;
#27555=EDGE_CURVE ( 'NONE', #23028, #13495, #15953, .T. ) ;
#27557=CARTESIAN_POINT ( 'NONE',  ( -5.405949406250003975, -9.363379034771801557, -111.3437500020483810 ) ) ;
#27559=CARTESIAN_POINT ( 'NONE',  ( -10.81189881249999729, 6.242252689847871849, -78.90625000204838102 ) ) ;
#27560=CARTESIAN_POINT ( 'NONE',  ( -5.405949406250003975, -9.363379034771801557, -97.84375000204838102 ) ) ;
#27563=CARTESIAN_POINT ( 'NONE',  ( -2.121150477449813534E-15, -11.54700538379251284, -151.2500000040967620 ) ) ;
#27567=CARTESIAN_POINT ( 'NONE',  ( -9.999999999999998224, 1.224646799147353059E-15, -108.1250000040967763 ) ) ;
#27571=CARTESIAN_POINT ( 'NONE',  ( 9.999999999999996447, -5.773502691896262640, -74.12499999999997158 ) ) ;
#27573=CARTESIAN_POINT ( 'NONE',  ( -2.121150477449813534E-15, -11.54700538379251284, -80.75000000409677625 ) ) ;
#27574=CARTESIAN_POINT ( 'NONE',  ( 4.999999999999992006, -8.660254037844389075, -171.7500000000000000 ) ) ;
#27576=CARTESIAN_POINT ( 'NONE',  ( 10.81189881249999551, -6.242252689847874514, -72.15625000204836681 ) ) ;
#27578=CARTESIAN_POINT ( 'NONE',  ( 9.999999999999998224, 0.000000000000000000, -113.3750000040967763 ) ) ;
#27580=ORIENTED_EDGE ( 'NONE', *, *, #4173, .T. ) ;
#27581=CARTESIAN_POINT ( 'NONE',  ( 5.405949406249999534, 9.363379034771803333, -199.2812500020484094 ) ) ;
#27583=CARTESIAN_POINT ( 'NONE',  ( 7.644554776091147741E-16, 12.48450537969573659, -15.96875000204835615 ) ) ;
#27586=CARTESIAN_POINT ( 'NONE',  ( -2.293366432827344421E-15, -12.48450537969573659, -129.4062500020483810 ) ) ;
#27587=CARTESIAN_POINT ( 'NONE',  ( 7.070501591499377789E-16, 11.54700538379251284, -184.6250000000000000 ) ) ;
#27588=CARTESIAN_POINT ( 'NONE',  ( 5.000000000000000000, 8.660254037844385522, -106.7499999999999858 ) ) ;
#27589=CARTESIAN_POINT ( 'NONE',  ( 10.81189881249999729, 0.000000000000000000, -112.5312500020483952 ) ) ;
#27590=ORIENTED_EDGE ( 'NONE', *, *, #18991, .T. ) ;
#27592=VERTEX_POINT ( 'NONE', #12857 ) ;
#27593=VERTEX_POINT ( 'NONE', #13278 ) ;
#27594=CARTESIAN_POINT ( 'NONE',  ( -2.293366432827344421E-15, -12.48450537969573659, -39.40625000204835260 ) ) ;
#27597=CARTESIAN_POINT ( 'NONE',  ( 5.405949406249992428, -9.363379034771808662, -88.59375000204838102 ) ) ;
#27602=CARTESIAN_POINT ( 'NONE',  ( -9.999999999999998224, 1.224646799147353059E-15, -58.24999999999997158 ) ) ;
#27604=CARTESIAN_POINT ( 'NONE',  ( 5.405949406249999534, 9.363379034771803333, -125.5937500020483668 ) ) ;
#27606=DIRECTION ( 'NONE',  ( -0.000000000000000000, -0.000000000000000000, 1.000000000000000000 ) ) ;
#27609=CARTESIAN_POINT ( 'NONE',  ( -9.999999999999998224, 5.773502691896259087, -181.7500000040967905 ) ) ;
#27611=CARTESIAN_POINT ( 'NONE',  ( 10.81189881249999729, 0.000000000000000000, -175.5312500020483810 ) ) ;
#27612=CARTESIAN_POINT ( 'NONE',  ( -10.00000000000102496, 5.773502691895664007, -2.874999999999923617 ) ) ;
#27615=CARTESIAN_POINT ( 'NONE',  ( 10.81189881249999729, 0.000000000000000000, -52.34375000204835260 ) ) ;
#27617=CARTESIAN_POINT ( 'NONE',  ( -10.81189881249999907, -6.242252689847864744, -8.156250002048370362 ) ) ;
#27621=CARTESIAN_POINT ( 'NONE',  ( 7.070501591499377789E-16, 11.54700538379251284, -100.6250000000000000 ) ) ;
#27623=CARTESIAN_POINT ( 'NONE',  ( 10.00000000000000000, 5.773502691896255534, -104.2500000040967763 ) ) ;
#27624=( BOUNDED_CURVE ( )  B_SPLINE_CURVE ( 2, ( #41130, #18053, #11361, #24556, #1676, #28000, #11570 ),
 .UNSPECIFIED., .F., .F. ) 
 B_SPLINE_CURVE_WITH_KNOTS ( ( 3, 2, 2, 3 ),
 ( 0.7761194029850747578, 0.7773631840796021431, 0.7786069651741295283, 0.7798507462686569136 ),
 .UNSPECIFIED. ) 
 CURVE ( )  GEOMETRIC_REPRESENTATION_ITEM ( )  RATIONAL_B_SPLINE_CURVE ( ( 0.9999999999999880096, 0.8660254037844506980, 1.000000000000000000, 0.8660254037844387076, 1.000000000000000000, 0.8660254037844148378, 1.000000000000023981 ) ) 
 REPRESENTATION_ITEM ( '' )  );
#27625=DIRECTION ( 'NONE',  ( -0.000000000000000000, -0.000000000000000000, 1.000000000000000000 ) ) ;
#27628=CARTESIAN_POINT ( 'NONE',  ( -10.81189881249999729, -6.242252689847864744, -108.6562500020483952 ) ) ;
#27629=EDGE_LOOP ( 'NONE', ( #39470, #1836, #27726, #16837 ) ) ;
#27631=CARTESIAN_POINT ( 'NONE',  ( 9.999999999999998224, 0.000000000000000000, -88.99999999999998579 ) ) ;
#27632=CARTESIAN_POINT ( 'NONE',  ( 10.81189881249999729, 0.000000000000000000, -165.0312500020484094 ) ) ;
#27635=CARTESIAN_POINT ( 'NONE',  ( -2.121150477449813534E-15, -11.54700538379251284, -24.87499999999998934 ) ) ;
#27636=CARTESIAN_POINT ( 'NONE',  ( 7.644554776091147741E-16, 12.48450537969573659, -37.15625000204836681 ) ) ;
#27637=CARTESIAN_POINT ( 'NONE',  ( -10.00000000000000000, -5.773502691896251982, -160.1250000000000284 ) ) ;
#27638=DIRECTION ( 'NONE',  ( -0.000000000000000000, -0.000000000000000000, 1.000000000000000000 ) ) ;
#27641=CARTESIAN_POINT ( 'NONE',  ( -10.81189881249999907, -6.242252689847864744, -135.6562500020484094 ) ) ;
#27642=CARTESIAN_POINT ( 'NONE',  ( -4.999999999999996447, 8.660254037844387298, -46.49999999999998579 ) ) ;
#27643=CARTESIAN_POINT ( 'NONE',  ( 9.999999999999998224, 0.000000000000000000, -174.8750000040967905 ) ) ;
#27644=EDGE_LOOP ( 'NONE', ( #20731, #1089, #17584, #9329 ) ) ;
#27645=ORIENTED_EDGE ( 'NONE', *, *, #12168, .F. ) ;
#27646=ORIENTED_EDGE ( 'NONE', *, *, #14315, .F. ) ;
#27647=CARTESIAN_POINT ( 'NONE',  ( -5.000000000000003553, -8.660254037844383745, -46.37500000409677625 ) ) ;
#27649=CARTESIAN_POINT ( 'NONE',  ( 10.81189881249999551, -6.242252689847874514, -161.9687500020484094 ) ) ;
#27651=CARTESIAN_POINT ( 'NONE',  ( -10.81189881249999907, -6.242252689847864744, -18.46875000204837036 ) ) ;
#27652=CARTESIAN_POINT ( 'NONE',  ( -9.999999999999998224, 1.224646799147353059E-15, -58.62500000409676204 ) ) ;
#27653=CARTESIAN_POINT ( 'NONE',  ( 10.81189881249999729, 0.000000000000000000, -149.8437500020483810 ) ) ;
#27654=CARTESIAN_POINT ( 'NONE',  ( 5.405949406249999534, 9.363379034771803333, -139.0937500020483810 ) ) ;
#27655=CARTESIAN_POINT ( 'NONE',  ( 5.405949406249992428, -9.363379034771808662, -108.2812500020483810 ) ) ;
#27659=CARTESIAN_POINT ( 'NONE',  ( 10.81189881249999551, -6.242252689847874514, -5.968750002048344605 ) ) ;
#27662=AXIS2_PLACEMENT_3D ( 'NONE', #33958, #20552, #16664 ) ;
#27669=CARTESIAN_POINT ( 'NONE',  ( 10.81189881249999551, -6.242252689847874514, -77.96875000204838102 ) ) ;
#27670=CARTESIAN_POINT ( 'NONE',  ( -5.405949406250003975, -9.363379034771801557, -67.84375000204836681 ) ) ;
#27671=CARTESIAN_POINT ( 'NONE',  ( 10.00000000000102318, -5.773502691895667560, -19.00000000409674428 ) ) ;
#27672=CARTESIAN_POINT ( 'NONE',  ( -5.405949406249996869, 9.363379034771805109, -31.03125000204837036 ) ) ;
#27676=CARTESIAN_POINT ( 'NONE',  ( -10.00000000000000000, -5.773502691896251982, -118.1250000000000142 ) ) ;
#27677=CARTESIAN_POINT ( 'NONE',  ( -10.81189881249999729, 1.324075727343319199E-15, -131.2812500020483810 ) ) ;
#27680=CARTESIAN_POINT ( 'NONE',  ( -5.405949406249996869, 9.363379034771805109, -19.03125000204835970 ) ) ;
#27685=CARTESIAN_POINT ( 'NONE',  ( -4.999999999999996447, 8.660254037844387298, -33.37500000409676915 ) ) ;
#27686=CARTESIAN_POINT ( 'NONE',  ( 5.000000000000000000, 8.660254037844385522, -75.24999999999998579 ) ) ;
#27688=CARTESIAN_POINT ( 'NONE',  ( 10.81189881249999551, -6.242252689847874514, -154.6562500020484379 ) ) ;
#27690=CARTESIAN_POINT ( 'NONE',  ( -5.405949406249996869, 9.363379034771805109, -128.3437500020484094 ) ) ;
#27691=ORIENTED_EDGE ( 'NONE', *, *, #15619, .F. ) ;
#27693=ORIENTED_EDGE ( 'NONE', *, *, #1146, .T. ) ;
#27696=EDGE_LOOP ( 'NONE', ( #8845, #11866, #10957, #42016 ) ) ;
#27697=CARTESIAN_POINT ( 'NONE',  ( -2.293366432827344421E-15, -12.48450537969573659, -108.2187500020483668 ) ) ;
#27699=CARTESIAN_POINT ( 'NONE',  ( 10.00000000000051159, -5.773502691895965988, -41.50000000409674072 ) ) ;
#27700=CARTESIAN_POINT ( 'NONE',  ( -10.81189881249999729, 1.324075727343319199E-15, -191.0937500020484094 ) ) ;
#27701=VECTOR ( 'NONE', #20140, 1000.000000000000000 ) ;
#27702=CARTESIAN_POINT ( 'NONE',  ( -10.81189881249999907, -6.242252689847864744, -37.96875000204837391 ) ) ;
#27703=CARTESIAN_POINT ( 'NONE',  ( 7.446394548109336320, -7.792472342551713282, 3.494387113477268989E-15 ) ) ;
#27704=DIRECTION ( 'NONE',  ( -0.000000000000000000, -0.000000000000000000, 1.000000000000000000 ) ) ;
#27705=CARTESIAN_POINT ( 'NONE',  ( -2.293366432827344421E-15, -12.48450537969573659, -168.2187500020483810 ) ) ;
#27706=CARTESIAN_POINT ( 'NONE',  ( -2.293366432827344421E-15, -12.48450537969573659, -162.2187500020483810 ) ) ;
#27707=CARTESIAN_POINT ( 'NONE',  ( -9.999999999998456346, -5.773502691897145489, -66.00000000409674783 ) ) ;
#27711=CARTESIAN_POINT ( 'NONE',  ( -9.999999999999998224, 1.224646799147353059E-15, -155.7500000000000000 ) ) ;
#27714=CARTESIAN_POINT ( 'NONE',  ( -10.81189881249999729, 1.324075727343319199E-15, -89.09375000204838102 ) ) ;
#27715=CARTESIAN_POINT ( 'NONE',  ( -9.999999999999998224, 1.224646799147353059E-15, -180.1250000040968189 ) ) ;
#27716=CARTESIAN_POINT ( 'NONE',  ( -5.405949406249996869, 9.363379034771805109, -56.53125000204836681 ) ) ;
#27717=DIRECTION ( 'NONE',  ( -0.000000000000000000, -0.000000000000000000, 1.000000000000000000 ) ) ;
#27720=CARTESIAN_POINT ( 'NONE',  ( 7.644554776091147741E-16, 12.48450537969573659, -118.1562500020483952 ) ) ;
#27721=CARTESIAN_POINT ( 'NONE',  ( -10.81189881249999729, -6.242252689847864744, -152.1562500020484094 ) ) ;
#27722=DIRECTION ( 'NONE',  ( 1.000000000000000000, 0.000000000000000000, 0.000000000000000000 ) ) ;
#27724=CARTESIAN_POINT ( 'NONE',  ( 4.999999999999992006, -8.660254037844389075, -130.1250000040967620 ) ) ;
#27726=ORIENTED_EDGE ( 'NONE', *, *, #37811, .F. ) ;
#27729=DIRECTION ( 'NONE',  ( 1.000000000000000000, 0.000000000000000000, 0.000000000000000000 ) ) ;
#27730=CARTESIAN_POINT ( 'NONE',  ( -2.293366432827344421E-15, -12.48450537969573659, -180.4062500020484379 ) ) ;
#27731=EDGE_LOOP ( 'NONE', ( #6926, #39046, #18113, #41543 ) ) ;
#27732=CARTESIAN_POINT ( 'NONE',  ( 9.999999999999996447, -5.773502691896262640, -51.62499999999999289 ) ) ;
#27734=CARTESIAN_POINT ( 'NONE',  ( 9.999999999999996447, -5.773502691896262640, -55.00000000409678336 ) ) ;
#27736=CARTESIAN_POINT ( 'NONE',  ( 9.999999999999998224, 0.000000000000000000, -131.0000000000000000 ) ) ;
#27738=CARTESIAN_POINT ( 'NONE',  ( -5.405949406250003975, -9.363379034771801557, -54.53125000204836681 ) ) ;
#27741=CARTESIAN_POINT ( 'NONE',  ( -9.999999999999998224, 1.224646799147353059E-15, -30.12500000409676204 ) ) ;
#27742=CARTESIAN_POINT ( 'NONE',  ( -10.81189881249999729, 6.242252689847871849, -177.9062500020484094 ) ) ;
#27743=AXIS2_PLACEMENT_3D ( 'NONE', #19702, #18868, #9569 ) ;
#27744=CARTESIAN_POINT ( 'NONE',  ( -4.999999999999996447, 8.660254037844387298, -147.3750000040967905 ) ) ;
#27745=CARTESIAN_POINT ( 'NONE',  ( 9.999999999999998224, 0.000000000000000000, -45.87500000409677625 ) ) ;
#27746=CARTESIAN_POINT ( 'NONE',  ( 9.999999999999998224, 0.000000000000000000, -200.0000000000000000 ) ) ;
#27747=DIRECTION ( 'NONE',  ( -0.08682659386424779191, 0.08682659386424779191, 0.9924325091389669673 ) ) ;
#27748=CARTESIAN_POINT ( 'NONE',  ( 0.000000000000000000, 0.000000000000000000, -200.0000000000000000 ) ) ;
#27749=CARTESIAN_POINT ( 'NONE',  ( 5.405949406249999534, 9.363379034771803333, -88.28125000204838102 ) ) ;
#27751=DIRECTION ( 'NONE',  ( -0.3779644730092256433, -0.6546536707079758655, -0.6546536707079793072 ) ) ;
#27753=ORIENTED_EDGE ( 'NONE', *, *, #3590, .F. ) ;
#27754=CARTESIAN_POINT ( 'NONE',  ( 10.81189881249999551, -6.242252689847874514, -40.46875000204835260 ) ) ;
#27755=CARTESIAN_POINT ( 'NONE',  ( -5.405949406250003975, -9.363379034771801557, -25.84375000204835970 ) ) ;
#27756=CARTESIAN_POINT ( 'NONE',  ( -10.81189881249999907, -6.242252689847864744, -12.65625000204835970 ) ) ;
#27757=CARTESIAN_POINT ( 'NONE',  ( -10.81189881249999729, 1.324075727343319199E-15, -66.59375000204836681 ) ) ;
#27759=DIRECTION ( 'NONE',  ( -0.000000000000000000, -0.000000000000000000, 1.000000000000000000 ) ) ;
#27761=CARTESIAN_POINT ( 'NONE',  ( 10.81189881249999729, 0.000000000000000000, -188.8437500020483810 ) ) ;
#27764=CARTESIAN_POINT ( 'NONE',  ( -9.999999999999676703, -5.773502691896437611, -183.0000000040967905 ) ) ;
#27765=CARTESIAN_POINT ( 'NONE',  ( -9.999999999999998224, 1.224646799147353059E-15, -200.0000000000000000 ) ) ;
#27767=CARTESIAN_POINT ( 'NONE',  ( -9.999999999999998224, 1.224646799147353059E-15, -188.7500000000000000 ) ) ;
#27768=CARTESIAN_POINT ( 'NONE',  ( -10.81189881249999729, 1.324075727343319199E-15, -113.0937500020483810 ) ) ;
#27769=LINE ( 'NONE', #40692, #7347 ) ;
#27770=CARTESIAN_POINT ( 'NONE',  ( -10.81189881249999729, 1.324075727343319199E-15, -81.78125000204839523 ) ) ;
#27772=CARTESIAN_POINT ( 'NONE',  ( 5.405949406249999534, 9.363379034771803333, -100.0937500020483810 ) ) ;
#27774=EDGE_CURVE ( 'NONE', #15995, #41544, #4467, .T. ) ;
#27776=CARTESIAN_POINT ( 'NONE',  ( 4.999999999999992006, -8.660254037844389075, -152.6250000040967905 ) ) ;
#27778=EDGE_CURVE ( 'NONE', #25691, #24966, #26678, .T. ) ;
#27781=CARTESIAN_POINT ( 'NONE',  ( 5.000000000000000000, 8.660254037844385522, -98.12500000409677625 ) ) ;
#27782=CARTESIAN_POINT ( 'NONE',  ( -9.999999999999998224, 1.224646799147353059E-15, -32.74999999999997158 ) ) ;
#27785=CARTESIAN_POINT ( 'NONE',  ( -9.999999999999998224, 1.224646799147353059E-15, -76.24999999999998579 ) ) ;
#27787=CARTESIAN_POINT ( 'NONE',  ( 9.999999999999996447, -5.773502691896262640, -80.50000000409676204 ) ) ;
#27791=CARTESIAN_POINT ( 'NONE',  ( 5.405949406249992428, -9.363379034771808662, -76.78125000204838102 ) ) ;
#27792=( BOUNDED_CURVE ( )  B_SPLINE_CURVE ( 2, ( #38519, #6151, #25790, #15416, #41542, #38946, #9379 ),
 .UNSPECIFIED., .F., .F. ) 
 B_SPLINE_CURVE_WITH_KNOTS ( ( 3, 2, 2, 3 ),
 ( 0.2798507462686568026, 0.2810945273631841879, 0.2823383084577115731, 0.2835820895522389029 ),
 .UNSPECIFIED. ) 
 CURVE ( )  GEOMETRIC_REPRESENTATION_ITEM ( )  RATIONAL_B_SPLINE_CURVE ( ( 0.9999999999999880096, 0.8660254037844506980, 1.000000000000000000, 0.8660254037844387076, 1.000000000000000000, 0.8660254037844267172, 1.000000000000011990 ) ) 
 REPRESENTATION_ITEM ( '' )  );
#27794=CARTESIAN_POINT ( 'NONE',  ( -9.999999999999998224, 1.224646799147353059E-15, -133.2499999999999716 ) ) ;
#27797=CARTESIAN_POINT ( 'NONE',  ( 7.644554776091147741E-16, 12.48450537969573659, -197.6562500020484379 ) ) ;
#27799=CARTESIAN_POINT ( 'NONE',  ( -10.81189881249999729, 1.324075727343319199E-15, -11.09375000204834727 ) ) ;
#27802=CARTESIAN_POINT ( 'NONE',  ( -5.405949406250003975, -9.363379034771801557, -126.5312500020483952 ) ) ;
#27803=ADVANCED_FACE ( 'NONE', ( #35771 ), #2961, .T. ) ;
#27804=CARTESIAN_POINT ( 'NONE',  ( 7.070501591499377789E-16, 11.54700538379251284, -183.1250000000000000 ) ) ;
#27806=CARTESIAN_POINT ( 'NONE',  ( -5.405949406250003975, -9.363379034771801557, -113.0312500020483952 ) ) ;
#27808=FACE_OUTER_BOUND ( 'NONE', #22319, .T. ) ;
#27809=EDGE_CURVE ( 'NONE', #10098, #18914, #29554, .T. ) ;
#27810=VERTEX_POINT ( 'NONE', #30140 ) ;
#27811=ORIENTED_EDGE ( 'NONE', *, *, #38726, .F. ) ;
#27812=CARTESIAN_POINT ( 'NONE',  ( 5.405949406249992428, -9.363379034771808662, -34.78125000204837391 ) ) ;
#27814=CARTESIAN_POINT ( 'NONE',  ( -10.81189881249999907, -6.242252689847864744, -88.96875000204836681 ) ) ;
#27815=CARTESIAN_POINT ( 'NONE',  ( -2.121150477449813534E-15, -11.54700538379251284, -167.3750000000000000 ) ) ;
#27817=DIRECTION ( 'NONE',  ( 1.000000000000000000, 0.000000000000000000, 0.000000000000000000 ) ) ;
#27820=CARTESIAN_POINT ( 'NONE',  ( 10.81189881249999551, -6.242252689847874514, -127.4687500020483810 ) ) ;
#27822=CARTESIAN_POINT ( 'NONE',  ( -10.81189881249999729, 6.242252689847871849, -0.9062500020483681418 ) ) ;
#27825=CARTESIAN_POINT ( 'NONE',  ( -5.000000000000003553, -8.660254037844383745, -179.8750000040967905 ) ) ;
#27827=CARTESIAN_POINT ( 'NONE',  ( -2.293366432827344421E-15, -12.48450537969573659, -166.9062500020484379 ) ) ;
#27829=CARTESIAN_POINT ( 'NONE',  ( 9.999999999998969713, 5.773502691896851502, -69.37499999999997158 ) ) ;
#27832=CARTESIAN_POINT ( 'NONE',  ( 10.81189881249999729, 0.000000000000000000, -55.34375000204835970 ) ) ;
#27834=CARTESIAN_POINT ( 'NONE',  ( -10.81189881249999729, 1.324075727343319199E-15, -14.28125000204835615 ) ) ;
#27836=CARTESIAN_POINT ( 'NONE',  ( 10.00000000000012257, -5.773502691896187144, -193.0000000040968189 ) ) ;
#27838=CARTESIAN_POINT ( 'NONE',  ( 7.070501591499377789E-16, 11.54700538379251284, -96.12500000000000000 ) ) ;
#27840=CARTESIAN_POINT ( 'NONE',  ( 9.999999999999996447, -5.773502691896262640, -107.5000000040967763 ) ) ;
#27841=CARTESIAN_POINT ( 'NONE',  ( -2.121150477449813534E-15, -11.54700538379251284, -190.2500000040967905 ) ) ;
#27844=CARTESIAN_POINT ( 'NONE',  ( -2.293366432827344421E-15, -12.48450537969573659, -99.40625000204839523 ) ) ;
#27845=VERTEX_POINT ( 'NONE', #11323 ) ;
#27848=CARTESIAN_POINT ( 'NONE',  ( -2.293366432827344421E-15, -12.48450537969573659, -163.9062500020483810 ) ) ;
#27850=ORIENTED_EDGE ( 'NONE', *, *, #23823, .F. ) ;
#27851=CARTESIAN_POINT ( 'NONE',  ( -9.999999999999998224, 5.773502691896259087, -22.37499999999997868 ) ) ;
#27852=CARTESIAN_POINT ( 'NONE',  ( 10.81189881249999729, 0.000000000000000000, -31.53125000204837391 ) ) ;
#27853=CARTESIAN_POINT ( 'NONE',  ( -9.999999999999998224, 1.224646799147353059E-15, -158.7500000000000000 ) ) ;
#27856=EDGE_CURVE ( 'NONE', #41318, #41327, #24516, .T. ) ;
#27857=CARTESIAN_POINT ( 'NONE',  ( 10.00000000000102318, -5.773502691895667560, -33.62499999999993605 ) ) ;
#27858=CARTESIAN_POINT ( 'NONE',  ( -10.81189881249999729, 1.324075727343319199E-15, -134.2812500020483810 ) ) ;
#27859=CARTESIAN_POINT ( 'NONE',  ( 9.999999999999479527, 5.773502691896553074, -75.75000000409676204 ) ) ;
#27860=CARTESIAN_POINT ( 'NONE',  ( -9.999999999999868550, 5.773502691896333694, -174.2500000040967905 ) ) ;
#27861=ORIENTED_EDGE ( 'NONE', *, *, #8554, .T. ) ;
#27862=CARTESIAN_POINT ( 'NONE',  ( -5.405949406249996869, 9.363379034771805109, -65.53125000204838102 ) ) ;
#27863=ORIENTED_EDGE ( 'NONE', *, *, #36779, .F. ) ;
#27864=ORIENTED_EDGE ( 'NONE', *, *, #2377, .F. ) ;
#27865=CYLINDRICAL_SURFACE ( 'NONE', #32530, 9.999999999999998224 ) ;
#27866=CARTESIAN_POINT ( 'NONE',  ( 10.81189881249999729, 0.000000000000000000, -155.8437500020483810 ) ) ;
#27868=CARTESIAN_POINT ( 'NONE',  ( 7.644554776091147741E-16, 12.48450537969573659, -11.46875000204836859 ) ) ;
#27869=CARTESIAN_POINT ( 'NONE',  ( 0.000000000000000000, 0.000000000000000000, -200.0000000000000000 ) ) ;
#27870=CARTESIAN_POINT ( 'NONE',  ( 10.81189881249999729, 6.242252689847867408, -151.2187500020484094 ) ) ;
#27871=CARTESIAN_POINT ( 'NONE',  ( -10.81189881249999729, 1.324075727343319199E-15, -131.0937500020483810 ) ) ;
#27872=( BOUNDED_CURVE ( )  B_SPLINE_CURVE ( 2, ( #31323, #1755, #5193, #14884, #28079, #41208, #11647 ),
 .UNSPECIFIED., .F., .F. ) 
 B_SPLINE_CURVE_WITH_KNOTS ( ( 3, 2, 2, 3 ),
 ( 0.6455223880597016350, 0.6467661691542290203, 0.6480099502487564056, 0.6492537313432837909 ),
 .UNSPECIFIED. ) 
 CURVE ( )  GEOMETRIC_REPRESENTATION_ITEM ( )  RATIONAL_B_SPLINE_CURVE ( ( 0.9999999999999880096, 0.8660254037844506980, 1.000000000000000000, 0.8660254037844387076, 1.000000000000000000, 0.8660254037844148378, 1.000000000000023981 ) ) 
 REPRESENTATION_ITEM ( '' )  );
#27873=CARTESIAN_POINT ( 'NONE',  ( 10.81189881249999907, 6.242252689847868297, -109.4062500020483952 ) ) ;
#27875=CARTESIAN_POINT ( 'NONE',  ( -9.999999999999998224, 1.224646799147353059E-15, -190.6250000040967905 ) ) ;
#27877=CARTESIAN_POINT ( 'NONE',  ( 5.405949406249992428, -9.363379034771808662, -3.093750002048367698 ) ) ;
#27879=CARTESIAN_POINT ( 'NONE',  ( 9.999999999999998224, 0.000000000000000000, -54.49999999999996447 ) ) ;
#27880=CARTESIAN_POINT ( 'NONE',  ( -9.999999999999996447, 5.773502691896259975, -165.2500000040967905 ) ) ;
#27883=CARTESIAN_POINT ( 'NONE',  ( -10.81189881249999729, -6.242252689847864744, -72.46875000204836681 ) ) ;
#27884=CARTESIAN_POINT ( 'NONE',  ( 7.644554776091147741E-16, 12.48450537969573659, -57.96875000204836681 ) ) ;
#27885=CARTESIAN_POINT ( 'NONE',  ( -9.999999999999998224, 1.224646799147353059E-15, -117.1250000040967905 ) ) ;
#27886=CARTESIAN_POINT ( 'NONE',  ( -2.293366432827344421E-15, -12.48450537969573659, -37.90625000204836681 ) ) ;
#27888=FACE_OUTER_BOUND ( 'NONE', #35183, .T. ) ;
#27890=CARTESIAN_POINT ( 'NONE',  ( 5.000000000000000000, 8.660254037844385522, -121.7500000000000000 ) ) ;
#27891=CARTESIAN_POINT ( 'NONE',  ( -10.81189881249999729, -6.242252689847864744, -129.6562500020483810 ) ) ;
#27894=CARTESIAN_POINT ( 'NONE',  ( -10.81189881249999729, 1.324075727343319199E-15, -12.78125000204835615 ) ) ;
#27895=ORIENTED_EDGE ( 'NONE', *, *, #11969, .T. ) ;
#27900=EDGE_CURVE ( 'NONE', #5939, #23120, #17576, .T. ) ;
#27901=CARTESIAN_POINT ( 'NONE',  ( 5.000000000000000000, 8.660254037844385522, -35.12500000409676915 ) ) ;
#27903=CARTESIAN_POINT ( 'NONE',  ( 10.81189881249999907, 6.242252689847868297, -154.4062500020484094 ) ) ;
#27904=CARTESIAN_POINT ( 'NONE',  ( -2.293366432827344421E-15, -12.48450537969573659, -124.7187500020483668 ) ) ;
#27906=ORIENTED_EDGE ( 'NONE', *, *, #41442, .F. ) ;
#27908=CARTESIAN_POINT ( 'NONE',  ( -9.999999999999998224, 1.224646799147353059E-15, -22.24999999999996447 ) ) ;
#27909=ORIENTED_EDGE ( 'NONE', *, *, #34660, .T. ) ;
#27910=EDGE_CURVE ( 'NONE', #29986, #18454, #42521, .T. ) ;
#27911=ORIENTED_EDGE ( 'NONE', *, *, #1065, .T. ) ;
#27912=ORIENTED_EDGE ( 'NONE', *, *, #2743, .F. ) ;
#27914=( BOUNDED_CURVE ( )  B_SPLINE_CURVE ( 2, ( #5237, #21198, #11477, #38040, #24891, #24678, #15356 ),
 .UNSPECIFIED., .F., .F. ) 
 B_SPLINE_CURVE_WITH_KNOTS ( ( 3, 2, 2, 3 ),
 ( 0.9216417910447763928, 0.9228855721393036671, 0.9241293532338311634, 0.9253731343283585487 ),
 .UNSPECIFIED. ) 
 CURVE ( )  GEOMETRIC_REPRESENTATION_ITEM ( )  RATIONAL_B_SPLINE_CURVE ( ( 0.9999999999999761302, 0.8660254037844625774, 1.000000000000000000, 0.8660254037844387076, 1.000000000000000000, 0.8660254037844028474, 1.000000000000035971 ) ) 
 REPRESENTATION_ITEM ( '' )  );
#27915=CARTESIAN_POINT ( 'NONE',  ( -10.81189881249999729, 1.324075727343319199E-15, -189.5937500020483810 ) ) ;
#27916=CARTESIAN_POINT ( 'NONE',  ( -5.405949406250003975, -9.363379034771801557, -39.34375000204837391 ) ) ;
#27917=CARTESIAN_POINT ( 'NONE',  ( -7.750360283152410545, -6.449078031086257212, -1.202135122527668287E-14 ) ) ;
#27918=CYLINDRICAL_SURFACE ( 'NONE', #2498, 9.999999999999998224 ) ;
#27919=CARTESIAN_POINT ( 'NONE',  ( -2.293366432827344421E-15, -12.48450537969573659, -172.7187500020483810 ) ) ;
#27920=CARTESIAN_POINT ( 'NONE',  ( -10.81189881249999907, -6.242252689847864744, -150.4687500020484094 ) ) ;
#27921=CARTESIAN_POINT ( 'NONE',  ( 9.999999999999998224, 0.000000000000000000, -122.3750000040967905 ) ) ;
#27923=AXIS2_PLACEMENT_3D ( 'NONE', #26777, #17040, #30240 ) ;
#27928=CARTESIAN_POINT ( 'NONE',  ( 0.000000000000000000, 0.000000000000000000, -200.0000000000000000 ) ) ;
#27930=CARTESIAN_POINT ( 'NONE',  ( 7.644554776091147741E-16, 12.48450537969573659, -90.96875000204838102 ) ) ;
#27931=CARTESIAN_POINT ( 'NONE',  ( -5.000000000000003553, -8.660254037844383745, -113.4999999999999858 ) ) ;
#27932=CARTESIAN_POINT ( 'NONE',  ( 5.405949406249992428, -9.363379034771808662, -57.28125000204836681 ) ) ;
#27935=CARTESIAN_POINT ( 'NONE',  ( 5.405949406249992428, -9.363379034771808662, -111.2812500020483810 ) ) ;
#27936=CARTESIAN_POINT ( 'NONE',  ( -10.81189881249999729, 1.324075727343319199E-15, -156.7812500020484094 ) ) ;
#27939=CARTESIAN_POINT ( 'NONE',  ( -2.121150477449813534E-15, -11.54700538379251284, -131.7500000040967905 ) ) ;
#27942=ORIENTED_EDGE ( 'NONE', *, *, #18445, .T. ) ;
#27943=AXIS2_PLACEMENT_3D ( 'NONE', #9774, #6969, #6340 ) ;
#27946=CARTESIAN_POINT ( 'NONE',  ( 9.999999999999998224, 0.000000000000000000, -185.0000000000000000 ) ) ;
#27947=CARTESIAN_POINT ( 'NONE',  ( -5.405949406249996869, 9.363379034771805109, -181.0312500020483810 ) ) ;
#27948=VERTEX_POINT ( 'NONE', #20830 ) ;
#27950=CARTESIAN_POINT ( 'NONE',  ( -9.999999999999998224, 1.224646799147353059E-15, -54.12500000409675494 ) ) ;
#27952=DIRECTION ( 'NONE',  ( 1.000000000000000000, 0.000000000000000000, 0.000000000000000000 ) ) ;
#27954=CARTESIAN_POINT ( 'NONE',  ( 10.81189881249999729, 0.000000000000000000, -51.03125000204835970 ) ) ;
#27957=CARTESIAN_POINT ( 'NONE',  ( 9.999999999998969713, 5.773502691896851502, -88.87499999999998579 ) ) ;
#27958=CARTESIAN_POINT ( 'NONE',  ( -10.81189881249999729, 6.242252689847871849, -174.9062500020483810 ) ) ;
#27959=CARTESIAN_POINT ( 'NONE',  ( -2.121150477449813534E-15, -11.54700538379251284, -87.87500000000000000 ) ) ;
#27960=CARTESIAN_POINT ( 'NONE',  ( 9.999999999999998224, 0.000000000000000000, -198.5000000000000000 ) ) ;
#27961=ORIENTED_EDGE ( 'NONE', *, *, #13792, .T. ) ;
#27962=CARTESIAN_POINT ( 'NONE',  ( -9.999999999999998224, 1.224646799147353059E-15, -16.62500000409675138 ) ) ;
#27963=CARTESIAN_POINT ( 'NONE',  ( 9.999999999999998224, 0.000000000000000000, -60.49999999999997158 ) ) ;
#27964=CARTESIAN_POINT ( 'NONE',  ( 5.000000000000000000, 8.660254037844385522, -39.62500000409676915 ) ) ;
#27965=CARTESIAN_POINT ( 'NONE',  ( 5.405949406249992428, -9.363379034771808662, -82.78125000204838102 ) ) ;
#27967=CARTESIAN_POINT ( 'NONE',  ( -10.00000000000154188, 5.773502691895366468, -24.25000000409672296 ) ) ;
#27970=ORIENTED_EDGE ( 'NONE', *, *, #33871, .T. ) ;
#27971=ORIENTED_EDGE ( 'NONE', *, *, #3823, .T. ) ;
#27972=CARTESIAN_POINT ( 'NONE',  ( -10.81189881249999729, -6.242252689847864744, -39.46875000204835970 ) ) ;
#27974=CARTESIAN_POINT ( 'NONE',  ( 10.81189881249999551, -6.242252689847874514, -13.65625000204836503 ) ) ;
#27975=CARTESIAN_POINT ( 'NONE',  ( -10.81189881249999729, 1.324075727343319199E-15, -60.59375000204836681 ) ) ;
#27976=ORIENTED_EDGE ( 'NONE', *, *, #37433, .T. ) ;
#27979=CARTESIAN_POINT ( 'NONE',  ( -10.81189881249999907, -6.242252689847864744, -183.4687500020484379 ) ) ;
#27982=CARTESIAN_POINT ( 'NONE',  ( 4.999999999999992006, -8.660254037844389075, -182.6250000040967905 ) ) ;
#27983=CARTESIAN_POINT ( 'NONE',  ( 9.999999999999479527, 5.773502691896553074, -141.3750000000000000 ) ) ;
#27984=CARTESIAN_POINT ( 'NONE',  ( -9.999999999999998224, 1.224646799147353059E-15, -21.12500000409675494 ) ) ;
#27986=CARTESIAN_POINT ( 'NONE',  ( 10.81189881249999551, -6.242252689847874514, -110.9687500020483810 ) ) ;
#27988=CARTESIAN_POINT ( 'NONE',  ( 10.81189881249999551, -6.242252689847874514, -79.65625000204838102 ) ) ;
#27989=CARTESIAN_POINT ( 'NONE',  ( -10.81189881249999729, 1.324075727343319199E-15, -95.09375000204838102 ) ) ;
#27993=CARTESIAN_POINT ( 'NONE',  ( 4.999999999999992006, -8.660254037844389075, -154.1250000040967905 ) ) ;
#27997=LINE ( 'NONE', #24553, #37866 ) ;
#27998=FACE_OUTER_BOUND ( 'NONE', #39624, .T. ) ;
#28000=CARTESIAN_POINT ( 'NONE',  ( -10.00000000000102496, 5.773502691895664007, -42.25000000409672651 ) ) ;
#28001=CARTESIAN_POINT ( 'NONE',  ( -5.000000000000003553, -8.660254037844383745, -71.49999999999998579 ) ) ;
#28003=CARTESIAN_POINT ( 'NONE',  ( -4.999999999999996447, 8.660254037844387298, -78.37500000409677625 ) ) ;
#28004=( BOUNDED_CURVE ( )  B_SPLINE_CURVE ( 2, ( #22954, #19483, #36108, #32670, #3098, #6542, #9979 ),
 .UNSPECIFIED., .F., .F. ) 
 B_SPLINE_CURVE_WITH_KNOTS ( ( 3, 2, 2, 3 ),
 ( 0.4962686567164180107, 0.4975124378109453960, 0.4987562189054727257, 0.5000000000000001110 ),
 .UNSPECIFIED. ) 
 CURVE ( )  GEOMETRIC_REPRESENTATION_ITEM ( )  RATIONAL_B_SPLINE_CURVE ( ( 0.9999999999999880096, 0.8660254037844506980, 1.000000000000000000, 0.8660254037844387076, 1.000000000000000000, 0.8660254037844267172, 1.000000000000011990 ) ) 
 REPRESENTATION_ITEM ( '' )  );
#28005=CARTESIAN_POINT ( 'NONE',  ( 5.000000000000000000, 8.660254037844385522, -26.12500000409675849 ) ) ;
#28007=CARTESIAN_POINT ( 'NONE',  ( 5.405949406249992428, -9.363379034771808662, -73.78125000204838102 ) ) ;
#28008=B_SPLINE_CURVE_WITH_KNOTS ( 'NONE', 3,
 ( #9847, #16300, #3806, #6824, #16730, #7251, #16516, #23233, #32737, #19767 ),
 .UNSPECIFIED., .F., .F.,
 ( 4, 2, 2, 2, 4 ),
 ( 0.000000000000000000, 0.04166666664189333513, 0.08333333328378667026, 0.1249999999256800054, 0.1666666665675733405 ),
 .UNSPECIFIED. ) ;
#28010=CARTESIAN_POINT ( 'NONE',  ( 7.070501591499376803E-16, 11.54700538379251284, -113.0000000040967763 ) ) ;
#28013=CARTESIAN_POINT ( 'NONE',  ( -5.000000000000003553, -8.660254037844383745, -5.499999999999976907 ) ) ;
#28015=CARTESIAN_POINT ( 'NONE',  ( -10.81189881249999729, 6.242252689847871849, -15.71875000204835793 ) ) ;
#28016=CARTESIAN_POINT ( 'NONE',  ( 9.999999999999998224, 0.000000000000000000, -63.87500000409676915 ) ) ;
#28018=CARTESIAN_POINT ( 'NONE',  ( -10.00000000000025580, 5.773502691896109873, -160.7500000040967620 ) ) ;
#28019=CARTESIAN_POINT ( 'NONE',  ( -5.405949406249996869, 9.363379034771805109, -133.0312500020484094 ) ) ;
#28020=CARTESIAN_POINT ( 'NONE',  ( -5.000000000000003553, -8.660254037844383745, -184.0000000000000000 ) ) ;
#28021=CARTESIAN_POINT ( 'NONE',  ( -2.121150477449813534E-15, -11.54700538379251284, -35.75000000409675494 ) ) ;
#28022=CARTESIAN_POINT ( 'NONE',  ( 5.405949406249992428, -9.363379034771808662, -111.2812500020483810 ) ) ;
#28023=ORIENTED_EDGE ( 'NONE', *, *, #11053, .F. ) ;
#28024=CARTESIAN_POINT ( 'NONE',  ( -9.999999999999612754, -5.773502691896474914, -154.5000000040967905 ) ) ;
#28028=VECTOR ( 'NONE', #16581, 1000.000000000000000 ) ;
#28030=CARTESIAN_POINT ( 'NONE',  ( -2.293366432827344421E-15, -12.48450537969573659, -40.90625000204836681 ) ) ;
#28032=CARTESIAN_POINT ( 'NONE',  ( 5.405949406249999534, 9.363379034771803333, -85.09375000204836681 ) ) ;
#28033=DIRECTION ( 'NONE',  ( 1.000000000000000000, 0.000000000000000000, 0.000000000000000000 ) ) ;
#28035=CYLINDRICAL_SURFACE ( 'NONE', #34336, 9.999999999999998224 ) ;
#28038=CARTESIAN_POINT ( 'NONE',  ( -2.293366432827344421E-15, -12.48450537969573659, -112.7187500020483668 ) ) ;
#28041=CARTESIAN_POINT ( 'NONE',  ( 10.81189881249999729, 6.242252689847867408, -5.906250002048359704 ) ) ;
#28044=CARTESIAN_POINT ( 'NONE',  ( 10.00000000000000000, 5.773502691896255534, -180.7500000040968189 ) ) ;
#28045=CARTESIAN_POINT ( 'NONE',  ( -10.81189881249999729, 1.324075727343319199E-15, -171.7812500020484094 ) ) ;
#28046=( BOUNDED_CURVE ( )  B_SPLINE_CURVE ( 2, ( #2648, #5679, #15147, #9117, #35247, #31805, #38683 ),
 .UNSPECIFIED., .F., .F. ) 
 B_SPLINE_CURVE_WITH_KNOTS ( ( 3, 2, 2, 3 ),
 ( 0.5970149253731344974, 0.5982587064676618827, 0.5995024875621891569, 0.6007462686567165422 ),
 .UNSPECIFIED. ) 
 CURVE ( )  GEOMETRIC_REPRESENTATION_ITEM ( )  RATIONAL_B_SPLINE_CURVE ( ( 0.9999999999999761302, 0.8660254037844625774, 1.000000000000000000, 0.8660254037844387076, 1.000000000000000000, 0.8660254037844267172, 1.000000000000011990 ) ) 
 REPRESENTATION_ITEM ( '' )  );
#28047=CARTESIAN_POINT ( 'NONE',  ( 7.070501591499376803E-16, 11.54700538379251284, -103.6249999999999858 ) ) ;
#28050=CARTESIAN_POINT ( 'NONE',  ( 5.405949406249999534, 9.363379034771803333, -50.59375000204835260 ) ) ;
#28052=CARTESIAN_POINT ( 'NONE',  ( -5.405949406249996869, 9.363379034771805109, -8.531250002048352599 ) ) ;
#28056=CARTESIAN_POINT ( 'NONE',  ( -2.121150477449813534E-15, -11.54700538379251284, -95.37500000000000000 ) ) ;
#28058=CARTESIAN_POINT ( 'NONE',  ( -10.00000000000000000, -5.773502691896251982, -103.5000000040967763 ) ) ;
#28059=DIRECTION ( 'NONE',  ( -0.000000000000000000, -0.000000000000000000, 1.000000000000000000 ) ) ;
#28062=CARTESIAN_POINT ( 'NONE',  ( 5.405949406249992428, -9.363379034771808662, -102.2812500020483952 ) ) ;
#28065=LINE ( 'NONE', #31092, #12556 ) ;
#28066=CARTESIAN_POINT ( 'NONE',  ( -5.405949406249996869, 9.363379034771805109, -157.0312500020484094 ) ) ;
#28068=ORIENTED_EDGE ( 'NONE', *, *, #21446, .T. ) ;
#28069=CARTESIAN_POINT ( 'NONE',  ( 9.999999999999998224, 0.000000000000000000, -27.49999999999996803 ) ) ;
#28071=CARTESIAN_POINT ( 'NONE',  ( 5.405949406249999534, 9.363379034771803333, -23.78125000204836681 ) ) ;
#28072=CARTESIAN_POINT ( 'NONE',  ( 5.000000000000000000, 8.660254037844385522, -162.2500000000000000 ) ) ;
#28073=LINE ( 'NONE', #30880, #35288 ) ;
#28076=CARTESIAN_POINT ( 'NONE',  ( 10.81189881249999907, 6.242252689847868297, -134.9062500020483810 ) ) ;
#28077=CARTESIAN_POINT ( 'NONE',  ( 7.070501591499376803E-16, 11.54700538379251284, -111.1249999999999858 ) ) ;
#28079=CARTESIAN_POINT ( 'NONE',  ( 4.999999999999992006, -8.660254037844389075, -68.62500000409677625 ) ) ;
#28080=ORIENTED_EDGE ( 'NONE', *, *, #30729, .T. ) ;
#28081=EDGE_CURVE ( 'NONE', #25114, #15207, #6115, .T. ) ;
#28082=CARTESIAN_POINT ( 'NONE',  ( -5.405949406250003975, -9.363379034771801557, -59.03125000204836681 ) ) ;
#28084=EDGE_CURVE ( 'NONE', #37499, #7028, #4715, .T. ) ;
#28085=ORIENTED_EDGE ( 'NONE', *, *, #24858, .F. ) ;
#28087=CARTESIAN_POINT ( 'NONE',  ( -9.999999999999998224, 1.224646799147353059E-15, -161.7500000000000000 ) ) ;
#28090=CARTESIAN_POINT ( 'NONE',  ( 5.405949406249999534, 9.363379034771803333, -155.5937500020483810 ) ) ;
#28092=CARTESIAN_POINT ( 'NONE',  ( 10.81189881249999907, 6.242252689847868297, -10.21875000204836326 ) ) ;
#28093=LINE ( 'NONE', #21165, #4672 ) ;
#28095=CARTESIAN_POINT ( 'NONE',  ( -5.405949406249996869, 9.363379034771805109, -146.3437500020483810 ) ) ;
#28096=CARTESIAN_POINT ( 'NONE',  ( -10.81189881249999729, 1.324075727343319199E-15, -104.2812500020483810 ) ) ;
#28098=LINE ( 'NONE', #22251, #15959 ) ;
#28100=CARTESIAN_POINT ( 'NONE',  ( -5.405949406249996869, 9.363379034771805109, -3.843750002048368586 ) ) ;
#28102=EDGE_CURVE ( 'NONE', #17690, #18615, #14982, .T. ) ;
#28103=CARTESIAN_POINT ( 'NONE',  ( -5.405949406250003975, -9.363379034771801557, -194.0312500020484094 ) ) ;
#28106=CARTESIAN_POINT ( 'NONE',  ( 5.405949406249999534, 9.363379034771803333, -74.59375000204838102 ) ) ;
#28107=CARTESIAN_POINT ( 'NONE',  ( -10.81189881249999729, 1.324075727343319199E-15, -60.59375000204836681 ) ) ;
#28109=CARTESIAN_POINT ( 'NONE',  ( -2.293366432827344421E-15, -12.48450537969573659, -31.90625000204835970 ) ) ;
#28112=DIRECTION ( 'NONE',  ( -0.000000000000000000, -0.000000000000000000, 1.000000000000000000 ) ) ;
#28114=CARTESIAN_POINT ( 'NONE',  ( -2.121150477449813534E-15, -11.54700538379251284, -119.3749999999999858 ) ) ;
#28115=CARTESIAN_POINT ( 'NONE',  ( 7.070501591499376803E-16, 11.54700538379251284, -42.12499999999997158 ) ) ;
#28117=CARTESIAN_POINT ( 'NONE',  ( 5.405949406249992428, -9.363379034771808662, -13.78125000204835615 ) ) ;
#28118=VERTEX_POINT ( 'NONE', #25156 ) ;
#28121=LINE ( 'NONE', #1579, #38768 ) ;
#28123=CARTESIAN_POINT ( 'NONE',  ( -9.999999999999998224, 1.224646799147353059E-15, -34.62500000409676915 ) ) ;
#28124=CARTESIAN_POINT ( 'NONE',  ( -5.000000000000003553, -8.660254037844383745, -2.875000004096767370 ) ) ;
#28127=CARTESIAN_POINT ( 'NONE',  ( -5.405949406250003975, -9.363379034771801557, -146.0312500020483810 ) ) ;
#28128=CARTESIAN_POINT ( 'NONE',  ( 10.81189881249999551, -6.242252689847874514, -124.4687500020483952 ) ) ;
#28132=VERTEX_POINT ( 'NONE', #1638 ) ;
#28133=AXIS2_PLACEMENT_3D ( 'NONE', #37472, #21501, #7699 ) ;
#28134=ORIENTED_EDGE ( 'NONE', *, *, #39278, .T. ) ;
#28135=AXIS2_PLACEMENT_3D ( 'NONE', #24907, #2657, #41700 ) ;
#28136=( BOUNDED_CURVE ( )  B_SPLINE_CURVE ( 2, ( #16031, #32681, #22966, #42580, #29439, #32890, #13003 ),
 .UNSPECIFIED., .F., .F. ) 
 B_SPLINE_CURVE_WITH_KNOTS ( ( 3, 2, 2, 3 ),
 ( 0.2164179104477612636, 0.2176616915422886489, 0.2189054726368160064, 0.2201492537313433639 ),
 .UNSPECIFIED. ) 
 CURVE ( )  GEOMETRIC_REPRESENTATION_ITEM ( )  RATIONAL_B_SPLINE_CURVE ( ( 0.9999999999999910072, 0.8660254037844477004, 1.000000000000000000, 0.8660254037844387076, 1.000000000000000000, 0.8660254037844297148, 1.000000000000008882 ) ) 
 REPRESENTATION_ITEM ( '' )  );
#28137=CARTESIAN_POINT ( 'NONE',  ( -4.999999999999996447, 8.660254037844387298, -189.0000000000000000 ) ) ;
#28138=CARTESIAN_POINT ( 'NONE',  ( -10.81189881249999729, 1.324075727343319199E-15, -182.0937500020483810 ) ) ;
#28139=CARTESIAN_POINT ( 'NONE',  ( 5.405949406249999534, 9.363379034771803333, -43.09375000204837391 ) ) ;
#28141=CARTESIAN_POINT ( 'NONE',  ( -5.405949406249996869, 9.363379034771805109, -173.3437500020484094 ) ) ;
#28142=CARTESIAN_POINT ( 'NONE',  ( 7.644554776091147741E-16, 12.48450537969573659, -153.9687500020484094 ) ) ;
#28143=CARTESIAN_POINT ( 'NONE',  ( 4.999999999999992006, -8.660254037844389075, -25.12500000409675849 ) ) ;
#28149=CARTESIAN_POINT ( 'NONE',  ( -10.81189881249999907, -6.242252689847864744, -79.96875000204836681 ) ) ;
#28150=CARTESIAN_POINT ( 'NONE',  ( -9.999999999999227285, -5.773502691896698735, -136.1249999999999716 ) ) ;
#28151=CARTESIAN_POINT ( 'NONE',  ( 10.81189881249999907, 6.242252689847868297, -61.40625000204838102 ) ) ;
#28154=CARTESIAN_POINT ( 'NONE',  ( -10.81189881249999907, -6.242252689847864744, -117.6562500020483952 ) ) ;
#28155=CARTESIAN_POINT ( 'NONE',  ( 7.644554776091147741E-16, 12.48450537969573659, -154.1562500020484094 ) ) ;
#28156=CARTESIAN_POINT ( 'NONE',  ( -2.121150477449813534E-15, -11.54700538379251284, -23.75000000409677270 ) ) ;
#28158=CARTESIAN_POINT ( 'NONE',  ( -9.999999999999998224, 5.773502691896259087, -118.7500000040967905 ) ) ;
#28163=DIRECTION ( 'NONE',  ( -0.000000000000000000, 1.000000000000000000, -0.000000000000000000 ) ) ;
#28164=CARTESIAN_POINT ( 'NONE',  ( -2.293366432827344421E-15, -12.48450537969573659, -177.4062500020483810 ) ) ;
#28167=CARTESIAN_POINT ( 'NONE',  ( -5.000000000000003553, -8.660254037844383745, -59.87500000409676204 ) ) ;
#28168=VECTOR ( 'NONE', #15589, 1000.000000000000000 ) ;
#28170=CARTESIAN_POINT ( 'NONE',  ( 9.999999999999998224, 0.000000000000000000, -57.87500000409676204 ) ) ;
#28174=CARTESIAN_POINT ( 'NONE',  ( -10.00000000000154188, 5.773502691895366468, -9.250000004096717632 ) ) ;
#28175=CARTESIAN_POINT ( 'NONE',  ( 5.405949406249992428, -9.363379034771808662, -165.2812500020484094 ) ) ;
#28176=LINE ( 'NONE', #32056, #3595 ) ;
#28177=LINE ( 'NONE', #34232, #30297 ) ;
#28178=ORIENTED_EDGE ( 'NONE', *, *, #39889, .F. ) ;
#28179=DIRECTION ( 'NONE',  ( 1.000000000000000000, 0.000000000000000000, 0.000000000000000000 ) ) ;
#28180=PLANE ( 'NONE',  #14842 ) ;
#28181=( BOUNDED_CURVE ( )  B_SPLINE_CURVE ( 2, ( #304, #20340, #33533, #26619, #39768, #23388, #20134 ),
 .UNSPECIFIED., .F., .F. ) 
 B_SPLINE_CURVE_WITH_KNOTS ( ( 3, 2, 2, 3 ),
 ( 0.2164179104477612636, 0.2176616915422886489, 0.2189054726368160064, 0.2201492537313433639 ),
 .UNSPECIFIED. ) 
 CURVE ( )  GEOMETRIC_REPRESENTATION_ITEM ( )  RATIONAL_B_SPLINE_CURVE ( ( 0.9999999999999910072, 0.8660254037844477004, 1.000000000000000000, 0.8660254037844387076, 1.000000000000000000, 0.8660254037844297148, 1.000000000000008882 ) ) 
 REPRESENTATION_ITEM ( '' )  );
#28182=CYLINDRICAL_SURFACE ( 'NONE', #35167, 9.999999999999998224 ) ;
#28183=CARTESIAN_POINT ( 'NONE',  ( -2.293366432827344421E-15, -12.48450537969573659, -78.40625000204838102 ) ) ;
#28184=ORIENTED_EDGE ( 'NONE', *, *, #28081, .T. ) ;
#28186=CARTESIAN_POINT ( 'NONE',  ( -9.999999999999998224, 1.224646799147353059E-15, -140.7500000000000000 ) ) ;
#28188=ORIENTED_EDGE ( 'NONE', *, *, #9016, .T. ) ;
#28189=CARTESIAN_POINT ( 'NONE',  ( -10.81189881249999729, -6.242252689847864744, -36.46875000204835970 ) ) ;
#28190=CARTESIAN_POINT ( 'NONE',  ( 7.070501591499376803E-16, 11.54700538379251284, -74.00000000409677625 ) ) ;
#28191=CARTESIAN_POINT ( 'NONE',  ( -5.405949406249996869, 9.363379034771805109, -8.531250002048352599 ) ) ;
#28193=CARTESIAN_POINT ( 'NONE',  ( -5.405949406249996869, 9.363379034771805109, -66.84375000204836681 ) ) ;
#28197=CARTESIAN_POINT ( 'NONE',  ( 10.81189881249999551, -6.242252689847874514, -197.9687500020484094 ) ) ;
#28198=CARTESIAN_POINT ( 'NONE',  ( -2.293366432827344421E-15, -12.48450537969573659, -175.7187500020483810 ) ) ;
#28200=CARTESIAN_POINT ( 'NONE',  ( 9.999999999999998224, 0.000000000000000000, -43.99999999999998579 ) ) ;
#28201=CARTESIAN_POINT ( 'NONE',  ( -9.999999999999998224, 1.224646799147353059E-15, -112.2499999999999858 ) ) ;
#28202=CARTESIAN_POINT ( 'NONE',  ( -9.999999999999998224, 1.224646799147353059E-15, -7.625000004096743389 ) ) ;
#28204=CARTESIAN_POINT ( 'NONE',  ( 5.405949406249992428, -9.363379034771808662, -106.5937500020483810 ) ) ;
#28205=DIRECTION ( 'NONE',  ( -0.000000000000000000, -0.000000000000000000, 1.000000000000000000 ) ) ;
#28206=CARTESIAN_POINT ( 'NONE',  ( 5.405949406249992428, -9.363379034771808662, -85.78125000204838102 ) ) ;
#28207=CARTESIAN_POINT ( 'NONE',  ( 10.81189881249999729, 6.242252689847867408, -92.71875000204838102 ) ) ;
#28209=CARTESIAN_POINT ( 'NONE',  ( -9.999999999999998224, 5.773502691896259087, -151.7500000040967620 ) ) ;
#28212=AXIS2_PLACEMENT_3D ( 'NONE', #1990, #31344, #38653 ) ;
#28215=CARTESIAN_POINT ( 'NONE',  ( 9.999999999999998224, 0.000000000000000000, -200.0000000000000000 ) ) ;
#28219=CARTESIAN_POINT ( 'NONE',  ( 7.070501591499377789E-16, 11.54700538379251284, -67.62500000000001421 ) ) ;
#28221=CARTESIAN_POINT ( 'NONE',  ( -9.999999999999998224, 1.224646799147353059E-15, -84.12500000409677625 ) ) ;
#28223=CARTESIAN_POINT ( 'NONE',  ( 9.999999999999998224, 0.000000000000000000, -120.8750000040967905 ) ) ;
#28225=CARTESIAN_POINT ( 'NONE',  ( 10.81189881249999729, 6.242252689847867408, -77.90625000204836681 ) ) ;
#28227=CARTESIAN_POINT ( 'NONE',  ( 9.999999999999998224, 0.000000000000000000, -77.37500000409677625 ) ) ;
#28229=CARTESIAN_POINT ( 'NONE',  ( 4.999999999999992006, -8.660254037844389075, -0.7499999999999729106 ) ) ;
#28231=CARTESIAN_POINT ( 'NONE',  ( -2.293366432827344421E-15, -12.48450537969573659, -1.718750002048356373 ) ) ;
#28232=CARTESIAN_POINT ( 'NONE',  ( 4.999999999999992006, -8.660254037844389075, -176.6250000040968189 ) ) ;
#28233=CARTESIAN_POINT ( 'NONE',  ( -10.81189881249999729, 6.242252689847871849, -146.2187500020483810 ) ) ;
#28234=CARTESIAN_POINT ( 'NONE',  ( -9.999999999999479527, -5.773502691896549521, -108.0000000040967478 ) ) ;
#28235=CARTESIAN_POINT ( 'NONE',  ( 5.000000000000000000, 8.660254037844385522, -133.7499999999999716 ) ) ;
#28236=CARTESIAN_POINT ( 'NONE',  ( -2.121150477449813534E-15, -11.54700538379251284, -183.8750000000000284 ) ) ;
#28237=CARTESIAN_POINT ( 'NONE',  ( 0.000000000000000000, 0.000000000000000000, -200.0000000000000000 ) ) ;
#28238=CARTESIAN_POINT ( 'NONE',  ( -10.81189881249999729, 1.324075727343319199E-15, -105.7812500020483810 ) ) ;
#28240=CARTESIAN_POINT ( 'NONE',  ( 9.999999999999998224, 0.000000000000000000, -138.8750000040968189 ) ) ;
#28241=VERTEX_POINT ( 'NONE', #21689 ) ;
#28243=VECTOR ( 'NONE', #14958, 1000.000000000000114 ) ;
#28244=CARTESIAN_POINT ( 'NONE',  ( -5.405949406250003975, -9.363379034771801557, -35.03125000204837391 ) ) ;
#28246=CARTESIAN_POINT ( 'NONE',  ( 7.644554776091147741E-16, 12.48450537969573659, -83.46875000204838102 ) ) ;
#28249=DIRECTION ( 'NONE',  ( -0.000000000000000000, -0.000000000000000000, 1.000000000000000000 ) ) ;
#28251=CARTESIAN_POINT ( 'NONE',  ( -9.999999999999982236, -5.773502691896262640, -199.1250000000000284 ) ) ;
#28252=CARTESIAN_POINT ( 'NONE',  ( -5.405949406250003975, -9.363379034771801557, -117.3437500020483810 ) ) ;
#28253=( BOUNDED_CURVE ( )  B_SPLINE_CURVE ( 2, ( #33757, #17747, #37183, #7630, #34613, #33971, #7416 ),
 .UNSPECIFIED., .F., .F. ) 
 B_SPLINE_CURVE_WITH_KNOTS ( ( 3, 2, 2, 3 ),
 ( 0.3432835820895522860, 0.3445273631840797268, 0.3457711442786070566, 0.3470149253731344974 ),
 .UNSPECIFIED. ) 
 CURVE ( )  GEOMETRIC_REPRESENTATION_ITEM ( )  RATIONAL_B_SPLINE_CURVE ( ( 0.9999999999999940048, 0.8660254037844447028, 1.000000000000000000, 0.8660254037844387076, 1.000000000000000000, 0.8660254037844207220, 1.000000000000017986 ) ) 
 REPRESENTATION_ITEM ( '' )  );
#28255=CARTESIAN_POINT ( 'NONE',  ( 5.405949406249992428, -9.363379034771808662, -3.281250002048374803 ) ) ;
#28258=CARTESIAN_POINT ( 'NONE',  ( 5.000000000000000000, 8.660254037844385522, -174.6250000040968189 ) ) ;
#28259=CARTESIAN_POINT ( 'NONE',  ( 10.81189881249999729, 0.000000000000000000, -166.5312500020484094 ) ) ;
#28260=CARTESIAN_POINT ( 'NONE',  ( 4.999999999999992006, -8.660254037844389075, -1.125000004096765593 ) ) ;
#28263=CARTESIAN_POINT ( 'NONE',  ( 10.81189881249999551, -6.242252689847874514, -47.96875000204836681 ) ) ;
#28264=AXIS2_PLACEMENT_3D ( 'NONE', #31855, #38307, #25580 ) ;
#28266=CARTESIAN_POINT ( 'NONE',  ( 5.405949406249992428, -9.363379034771808662, -3.281250002048374803 ) ) ;
#28268=CARTESIAN_POINT ( 'NONE',  ( -5.000000000000003553, -8.660254037844383745, -158.8750000040967905 ) ) ;
#28270=ADVANCED_FACE ( 'NONE', ( #8958 ), #22120, .T. ) ;
#28271=CARTESIAN_POINT ( 'NONE',  ( -9.999999999999998224, 1.224646799147353059E-15, -92.74999999999998579 ) ) ;
#28273=CARTESIAN_POINT ( 'NONE',  ( -9.999999999999998224, 5.773502691896259087, -106.7500000040967620 ) ) ;
#28274=CARTESIAN_POINT ( 'NONE',  ( -9.999999999999998224, 1.224646799147353059E-15, -82.24999999999998579 ) ) ;
#28277=CARTESIAN_POINT ( 'NONE',  ( -5.405949406250003975, -9.363379034771801557, -102.5312500020483952 ) ) ;
#28280=CARTESIAN_POINT ( 'NONE',  ( 10.81189881249999551, -6.242252689847874514, -159.1562500020484094 ) ) ;
#28283=CARTESIAN_POINT ( 'NONE',  ( -9.999999999999998224, 5.773502691896259087, -23.87499999999998579 ) ) ;
#28284=CARTESIAN_POINT ( 'NONE',  ( -2.293366432827344421E-15, -12.48450537969573659, -27.40625000204838102 ) ) ;
#28285=CARTESIAN_POINT ( 'NONE',  ( 9.999999999999998224, 0.000000000000000000, -164.0000000000000000 ) ) ;
#28288=CARTESIAN_POINT ( 'NONE',  ( 5.405949406249992428, -9.363379034771808662, -135.2812500020483810 ) ) ;
#28289=CARTESIAN_POINT ( 'NONE',  ( -10.00000000000102496, 5.773502691895664007, -75.25000000409673362 ) ) ;
#28292=CARTESIAN_POINT ( 'NONE',  ( 7.644554776091147741E-16, 12.48450537969573659, -58.15625000204838102 ) ) ;
#28295=ORIENTED_EDGE ( 'NONE', *, *, #38630, .F. ) ;
#28297=DIRECTION ( 'NONE',  ( -0.000000000000000000, -0.000000000000000000, 1.000000000000000000 ) ) ;
#28298=DIRECTION ( 'NONE',  ( 1.000000000000000000, 0.000000000000000000, 0.000000000000000000 ) ) ;
#28299=( BOUNDED_CURVE ( )  B_SPLINE_CURVE ( 2, ( #14647, #11411, #14857, #25250, #1513, #38395, #24605 ),
 .UNSPECIFIED., .F., .F. ) 
 B_SPLINE_CURVE_WITH_KNOTS ( ( 3, 2, 2, 3 ),
 ( 0.2276119402985075368, 0.2288557213930349221, 0.2300995024875622796, 0.2313432835820896372 ),
 .UNSPECIFIED. ) 
 CURVE ( )  GEOMETRIC_REPRESENTATION_ITEM ( )  RATIONAL_B_SPLINE_CURVE ( ( 0.9999999999999910072, 0.8660254037844477004, 1.000000000000000000, 0.8660254037844387076, 1.000000000000000000, 0.8660254037844297148, 1.000000000000008882 ) ) 
 REPRESENTATION_ITEM ( '' )  );
#28300=CARTESIAN_POINT ( 'NONE',  ( -2.293366432827344421E-15, -12.48450537969573659, -160.7187500020483810 ) ) ;
#28302=CARTESIAN_POINT ( 'NONE',  ( -5.405949406250003975, -9.363379034771801557, -6.343750002048370362 ) ) ;
#28303=CARTESIAN_POINT ( 'NONE',  ( 10.81189881249999729, 0.000000000000000000, -143.8437500020483810 ) ) ;
#28304=CARTESIAN_POINT ( 'NONE',  ( 5.405949406249999534, 9.363379034771803333, -95.78125000204838102 ) ) ;
#28308=CARTESIAN_POINT ( 'NONE',  ( -10.81189881249999907, -6.242252689847864744, -0.4687500020483501006 ) ) ;
#28310=CARTESIAN_POINT ( 'NONE',  ( 10.81189881249999551, -6.242252689847874514, -192.1562500020484094 ) ) ;
#28314=CARTESIAN_POINT ( 'NONE',  ( -10.81189881249999729, 1.324075727343319199E-15, -80.09375000204838102 ) ) ;
#28315=CARTESIAN_POINT ( 'NONE',  ( 5.405949406249992428, -9.363379034771808662, -55.59375000204835970 ) ) ;
#28317=CARTESIAN_POINT ( 'NONE',  ( 10.81189881249999729, 0.000000000000000000, -22.53125000204836326 ) ) ;
#28321=ADVANCED_FACE ( 'NONE', ( #8747 ), #41537, .T. ) ;
#28322=CARTESIAN_POINT ( 'NONE',  ( -4.999999999999996447, 8.660254037844387298, -123.0000000000000000 ) ) ;
#28323=CARTESIAN_POINT ( 'NONE',  ( -10.00000000000102496, 5.773502691895664007, -41.87499999999994316 ) ) ;
#28324=EDGE_CURVE ( 'NONE', #40457, #3711, #22122, .T. ) ;
#28327=CARTESIAN_POINT ( 'NONE',  ( -10.81189881249999729, -6.242252689847864744, -6.656250002048365033 ) ) ;
#28328=EDGE_CURVE ( 'NONE', #17345, #35521, #5870, .T. ) ;
#28335=CARTESIAN_POINT ( 'NONE',  ( -9.999999999999998224, 5.773502691896259087, -25.75000000409677270 ) ) ;
#28336=VECTOR ( 'NONE', #42324, 1000.000000000000000 ) ;
#28337=CARTESIAN_POINT ( 'NONE',  ( -9.999999999999998224, 1.224646799147353059E-15, -74.74999999999998579 ) ) ;
#28340=LINE ( 'NONE', #41478, #28336 ) ;
#28341=CARTESIAN_POINT ( 'NONE',  ( -10.81189881249999729, 1.324075727343319199E-15, -141.7812500020483810 ) ) ;
#28342=CARTESIAN_POINT ( 'NONE',  ( 5.405949406249992428, -9.363379034771808662, -130.5937500020483810 ) ) ;
#28345=CARTESIAN_POINT ( 'NONE',  ( -9.999999999999998224, 1.224646799147353059E-15, -190.2500000000000000 ) ) ;
#28347=EDGE_CURVE ( 'NONE', #9909, #5974, #7823, .T. ) ;
#28348=ORIENTED_EDGE ( 'NONE', *, *, #15327, .T. ) ;
#28349=ORIENTED_EDGE ( 'NONE', *, *, #1167, .T. ) ;
#28351=DIRECTION ( 'NONE',  ( -0.000000000000000000, -0.000000000000000000, 1.000000000000000000 ) ) ;
#28352=CARTESIAN_POINT ( 'NONE',  ( 10.81189881249999729, 0.000000000000000000, -179.8437500020483810 ) ) ;
#28353=CARTESIAN_POINT ( 'NONE',  ( -10.81189881249999729, 6.242252689847871849, -30.71875000204834905 ) ) ;
#28355=CARTESIAN_POINT ( 'NONE',  ( 10.81189881249999551, -6.242252689847874514, -160.4687500020484094 ) ) ;
#28356=CARTESIAN_POINT ( 'NONE',  ( 10.81189881249999551, -6.242252689847874514, -155.9687500020484094 ) ) ;
#28362=CARTESIAN_POINT ( 'NONE',  ( 7.071067811865477282, -7.071067811865471064, -200.0000000000000000 ) ) ;
#28363=CARTESIAN_POINT ( 'NONE',  ( 7.070501591499376803E-16, 11.54700538379251284, -183.1250000000000000 ) ) ;
#28365=CARTESIAN_POINT ( 'NONE',  ( 10.81189881249999907, 6.242252689847868297, -79.21875000204838102 ) ) ;
#28367=CARTESIAN_POINT ( 'NONE',  ( -5.405949406249996869, 9.363379034771805109, -61.03125000204837391 ) ) ;
#28370=CARTESIAN_POINT ( 'NONE',  ( 10.81189881249999907, 6.242252689847868297, -113.9062500020483952 ) ) ;
#28371=CARTESIAN_POINT ( 'NONE',  ( -5.405949406250003975, -9.363379034771801557, -144.5312500020483810 ) ) ;
#28374=CARTESIAN_POINT ( 'NONE',  ( 7.070501591499377789E-16, 11.54700538379251284, -122.0000000040967905 ) ) ;
#28379=CARTESIAN_POINT ( 'NONE',  ( -9.999999999999998224, 1.224646799147353059E-15, -67.62500000409676204 ) ) ;
#28381=CARTESIAN_POINT ( 'NONE',  ( 10.81189881249999729, 0.000000000000000000, -178.5312500020483810 ) ) ;
#28382=ORIENTED_EDGE ( 'NONE', *, *, #9293, .T. ) ;
#28384=CARTESIAN_POINT ( 'NONE',  ( 7.070501591499377789E-16, 11.54700538379251284, -47.00000000409677625 ) ) ;
#28386=CARTESIAN_POINT ( 'NONE',  ( -9.999999999999996447, 5.773502691896259975, -171.2500000040967905 ) ) ;
#28391=CARTESIAN_POINT ( 'NONE',  ( -5.405949406249996869, 9.363379034771805109, -170.5312500020484094 ) ) ;
#28394=DIRECTION ( 'NONE',  ( 1.000000000000000000, 4.506943796211477094E-16, 0.000000000000000000 ) ) ;
#28395=CARTESIAN_POINT ( 'NONE',  ( -5.000000000000003553, -8.660254037844383745, -34.37500000409676915 ) ) ;
#28399=DIRECTION ( 'NONE',  ( 1.000000000000000000, 0.000000000000000000, 0.000000000000000000 ) ) ;
#28400=CARTESIAN_POINT ( 'NONE',  ( 9.999999999999932498, 5.773502691896291950, -195.7500000040968189 ) ) ;
#28401=AXIS2_PLACEMENT_3D ( 'NONE', #35041, #15153, #5467 ) ;
#28402=CARTESIAN_POINT ( 'NONE',  ( 5.405949406249999534, 9.363379034771803333, -77.78125000204838102 ) ) ;
#28404=CARTESIAN_POINT ( 'NONE',  ( -14.84614977916192302, -1.734723475976807094E-15, 52.14285714285716011 ) ) ;
#28406=ORIENTED_EDGE ( 'NONE', *, *, #12569, .T. ) ;
#28407=CARTESIAN_POINT ( 'NONE',  ( 10.81189881249999551, -6.242252689847874514, -25.46875000204837391 ) ) ;
#28408=CARTESIAN_POINT ( 'NONE',  ( -5.000000000000003553, -8.660254037844383745, -53.49999999999996447 ) ) ;
#28409=CARTESIAN_POINT ( 'NONE',  ( 10.81189881249999729, 0.000000000000000000, -6.031250002048377468 ) ) ;
#28410=CARTESIAN_POINT ( 'NONE',  ( 5.405949406249999534, 9.363379034771803333, -55.09375000204835970 ) ) ;
#28411=EDGE_LOOP ( 'NONE', ( #4552, #36818, #18642, #42539 ) ) ;
#28412=CARTESIAN_POINT ( 'NONE',  ( 7.070501591499376803E-16, 11.54700538379251284, -28.62499999999997513 ) ) ;
#28414=CARTESIAN_POINT ( 'NONE',  ( 10.81189881249999729, 0.000000000000000000, -194.8437500020484094 ) ) ;
#28415=CARTESIAN_POINT ( 'NONE',  ( -10.81189881249999907, -6.242252689847864744, -180.4687500020484094 ) ) ;
#28419=CARTESIAN_POINT ( 'NONE',  ( 9.999999999999998224, 0.000000000000000000, -200.0000000000000000 ) ) ;
#28422=CARTESIAN_POINT ( 'NONE',  ( -5.405949406250003975, -9.363379034771801557, -106.8437500020483810 ) ) ;
#28423=CARTESIAN_POINT ( 'NONE',  ( -9.999999999999998224, 1.224646799147353059E-15, -184.2500000000000000 ) ) ;
#28424=CARTESIAN_POINT ( 'NONE',  ( -10.81189881249999907, -6.242252689847864744, -84.65625000204836681 ) ) ;
#28425=CARTESIAN_POINT ( 'NONE',  ( 7.644554776091147741E-16, 12.48450537969573659, -92.46875000204838102 ) ) ;
#28427=CARTESIAN_POINT ( 'NONE',  ( -2.121150477449813534E-15, -11.54700538379251284, -149.7500000040968189 ) ) ;
#28429=ORIENTED_EDGE ( 'NONE', *, *, #23193, .T. ) ;
#28432=AXIS2_PLACEMENT_3D ( 'NONE', #36631, #7077, #39026 ) ;
#28434=CARTESIAN_POINT ( 'NONE',  ( -9.999999999999479527, -5.773502691896549521, -38.62499999999993605 ) ) ;
#28437=CARTESIAN_POINT ( 'NONE',  ( -2.121150477449813534E-15, -11.54700538379251284, -66.87500000000000000 ) ) ;
#28439=CARTESIAN_POINT ( 'NONE',  ( -10.00000000000000000, -5.773502691896251982, -84.00000000409677625 ) ) ;
#28443=CARTESIAN_POINT ( 'NONE',  ( -10.81189881249999729, -6.242252689847864744, -78.65625000204836681 ) ) ;
#28444=( BOUNDED_CURVE ( )  B_SPLINE_CURVE ( 2, ( #4325, #17463, #14216, #34913, #7784, #34110, #41356 ),
 .UNSPECIFIED., .F., .F. ) 
 B_SPLINE_CURVE_WITH_KNOTS ( ( 3, 2, 2, 3 ),
 ( 0.9477611940298510396, 0.9490049751243784248, 0.9502487562189058101, 0.9514925373134331954 ),
 .UNSPECIFIED. ) 
 CURVE ( )  GEOMETRIC_REPRESENTATION_ITEM ( )  RATIONAL_B_SPLINE_CURVE ( ( 0.9999999999999641398, 0.8660254037844745678, 1.000000000000000000, 0.8660254037844387076, 1.000000000000000000, 0.8660254037844028474, 1.000000000000035971 ) ) 
 REPRESENTATION_ITEM ( '' )  );
#28446=DIRECTION ( 'NONE',  ( -0.000000000000000000, -0.000000000000000000, 1.000000000000000000 ) ) ;
#28448=ORIENTED_EDGE ( 'NONE', *, *, #11167, .F. ) ;
#28449=CARTESIAN_POINT ( 'NONE',  ( -10.81189881249999729, 1.324075727343319199E-15, -189.7812500020484094 ) ) ;
#28450=EDGE_CURVE ( 'NONE', #21857, #22494, #9136, .T. ) ;
#28452=CARTESIAN_POINT ( 'NONE',  ( 5.405949406249992428, -9.363379034771808662, -7.593750002048343717 ) ) ;
#28453=FACE_OUTER_BOUND ( 'NONE', #28708, .T. ) ;
#28454=CARTESIAN_POINT ( 'NONE',  ( -5.405949406249996869, 9.363379034771805109, -143.3437500020483810 ) ) ;
#28455=CARTESIAN_POINT ( 'NONE',  ( 4.999999999999992006, -8.660254037844389075, -37.12500000409676915 ) ) ;
#28456=LINE ( 'NONE', #7046, #32130 ) ;
#28457=( BOUNDED_CURVE ( )  B_SPLINE_CURVE ( 2, ( #9277, #35203, #35625, #31545, #6052, #19202, #14891 ),
 .UNSPECIFIED., .F., .F. ) 
 B_SPLINE_CURVE_WITH_KNOTS ( ( 3, 2, 2, 3 ),
 ( 0.2686567164179105571, 0.2699004975124379424, 0.2711442786069652722, 0.2723880597014926574 ),
 .UNSPECIFIED. ) 
 CURVE ( )  GEOMETRIC_REPRESENTATION_ITEM ( )  RATIONAL_B_SPLINE_CURVE ( ( 0.9999999999999880096, 0.8660254037844506980, 1.000000000000000000, 0.8660254037844387076, 1.000000000000000000, 0.8660254037844267172, 1.000000000000011990 ) ) 
 REPRESENTATION_ITEM ( '' )  );
#28458=CARTESIAN_POINT ( 'NONE',  ( -9.999999999999998224, 1.224646799147353059E-15, -173.7500000000000284 ) ) ;
#28459=CARTESIAN_POINT ( 'NONE',  ( -9.999999999999998224, 1.224646799147353059E-15, -175.6250000040968189 ) ) ;
#28460=CARTESIAN_POINT ( 'NONE',  ( 5.405949406249999534, 9.363379034771803333, -103.2812500020483952 ) ) ;
#28461=EDGE_LOOP ( 'NONE', ( #12188, #7150, #7525, #41212 ) ) ;
#28462=CARTESIAN_POINT ( 'NONE',  ( -9.999999999999872102, -5.773502691896326589, -164.6249999999999716 ) ) ;
#28465=EDGE_CURVE ( 'NONE', #38628, #18833, #17934, .T. ) ;
#28466=CARTESIAN_POINT ( 'NONE',  ( -2.293366432827344421E-15, -12.48450537969573659, -31.90625000204835970 ) ) ;
#28468=VECTOR ( 'NONE', #1622, 1000.000000000000000 ) ;
#28469=CARTESIAN_POINT ( 'NONE',  ( -10.81189881249999729, 6.242252689847871849, -87.71875000204838102 ) ) ;
#28472=FACE_OUTER_BOUND ( 'NONE', #15575, .T. ) ;
#28474=CARTESIAN_POINT ( 'NONE',  ( 9.999999999999996447, -5.773502691896262640, -11.50000000409676559 ) ) ;
#28475=CARTESIAN_POINT ( 'NONE',  ( 4.999999999999992006, -8.660254037844389075, -198.7500000000000000 ) ) ;
#28476=CARTESIAN_POINT ( 'NONE',  ( -5.405949406249996869, 9.363379034771805109, -113.3437500020483810 ) ) ;
#28480=CARTESIAN_POINT ( 'NONE',  ( -9.999999999999998224, 5.773502691896259087, -169.7500000040967905 ) ) ;
#28481=CARTESIAN_POINT ( 'NONE',  ( 10.81189881249999551, -6.242252689847874514, -169.6562500020484094 ) ) ;
#28484=CARTESIAN_POINT ( 'NONE',  ( -5.405949406250003975, -9.363379034771801557, -46.84375000204838102 ) ) ;
#28486=CARTESIAN_POINT ( 'NONE',  ( -2.293366432827344421E-15, -12.48450537969573659, -1.906250002048373027 ) ) ;
#28488=CARTESIAN_POINT ( 'NONE',  ( 9.999999999999998224, 0.000000000000000000, -54.49999999999996447 ) ) ;
#28490=CARTESIAN_POINT ( 'NONE',  ( 9.999999999999996447, -5.773502691896262640, -87.62499999999998579 ) ) ;
#28492=CARTESIAN_POINT ( 'NONE',  ( -9.999999999999998224, 1.224646799147353059E-15, -106.6250000040967763 ) ) ;
#28496=CARTESIAN_POINT ( 'NONE',  ( -2.293366432827344421E-15, -12.48450537969573659, -97.90625000204839523 ) ) ;
#28501=CARTESIAN_POINT ( 'NONE',  ( 10.81189881249999729, 0.000000000000000000, -154.5312500020484094 ) ) ;
#28503=VERTEX_POINT ( 'NONE', #8036 ) ;
#28504=CARTESIAN_POINT ( 'NONE',  ( -5.000000000000003553, -8.660254037844383745, -20.49999999999996447 ) ) ;
#28505=CARTESIAN_POINT ( 'NONE',  ( 10.81189881249999729, 6.242252689847867408, -25.40625000204838813 ) ) ;
#28506=CARTESIAN_POINT ( 'NONE',  ( -5.000000000000003553, -8.660254037844383745, -152.5000000000000000 ) ) ;
#28508=CARTESIAN_POINT ( 'NONE',  ( -9.999999999999998224, 5.773502691896259087, -196.3750000000000568 ) ) ;
#28509=CARTESIAN_POINT ( 'NONE',  ( -10.81189881249999729, 1.324075727343319199E-15, -128.2812500020483810 ) ) ;
#28510=CARTESIAN_POINT ( 'NONE',  ( 9.999999999999998224, 0.000000000000000000, -65.37500000409676204 ) ) ;
#28511=CARTESIAN_POINT ( 'NONE',  ( 10.00000000000051159, -5.773502691895965988, -44.50000000409674783 ) ) ;
#28513=CARTESIAN_POINT ( 'NONE',  ( 5.405949406249999534, 9.363379034771803333, -55.28125000204836681 ) ) ;
#28515=CARTESIAN_POINT ( 'NONE',  ( 5.405949406249999534, 9.363379034771803333, -115.0937500020483810 ) ) ;
#28519=( BOUNDED_CURVE ( )  B_SPLINE_CURVE ( 2, ( #4950, #31292, #14850, #28047, #41173, #24820, #8410 ),
 .UNSPECIFIED., .F., .F. ) 
 B_SPLINE_CURVE_WITH_KNOTS ( ( 3, 2, 2, 3 ),
 ( 0.4776119402985076756, 0.4788557213930350054, 0.4800995024875623352, 0.4813432835820896649 ),
 .UNSPECIFIED. ) 
 CURVE ( )  GEOMETRIC_REPRESENTATION_ITEM ( )  RATIONAL_B_SPLINE_CURVE ( ( 0.9999999999999761302, 0.8660254037844625774, 1.000000000000000000, 0.8660254037844387076, 1.000000000000000000, 0.8660254037844267172, 1.000000000000011990 ) ) 
 REPRESENTATION_ITEM ( '' )  );
#28521=CARTESIAN_POINT ( 'NONE',  ( 9.999999999999998224, 0.000000000000000000, -183.5000000000000000 ) ) ;
#28522=CARTESIAN_POINT ( 'NONE',  ( 10.81189881249999551, -6.242252689847874514, -155.9687500020484094 ) ) ;
#28524=CARTESIAN_POINT ( 'NONE',  ( -2.293366432827344421E-15, -12.48450537969573659, -7.718750002048352599 ) ) ;
#28525=CARTESIAN_POINT ( 'NONE',  ( -2.293366432827344421E-15, -12.48450537969573659, -141.2187500020483810 ) ) ;
#28527=CARTESIAN_POINT ( 'NONE',  ( -5.000000000000003553, -8.660254037844383745, -161.5000000000000000 ) ) ;
#28529=CARTESIAN_POINT ( 'NONE',  ( 10.81189881249999551, -6.242252689847874514, -4.468750002048369474 ) ) ;
#28531=CARTESIAN_POINT ( 'NONE',  ( -10.81189881249999729, -6.242252689847864744, -197.1562500020484379 ) ) ;
#28535=CARTESIAN_POINT ( 'NONE',  ( 7.644554776091147741E-16, 12.48450537969573659, -69.96875000204838102 ) ) ;
#28536=CARTESIAN_POINT ( 'NONE',  ( 10.81189881249999551, -6.242252689847874514, -56.96875000204838102 ) ) ;
#28538=CARTESIAN_POINT ( 'NONE',  ( 10.81189881249999907, 6.242252689847868297, -29.90625000204836326 ) ) ;
#28540=CARTESIAN_POINT ( 'NONE',  ( 9.999999999999998224, 0.000000000000000000, -95.37500000409677625 ) ) ;
#28542=CARTESIAN_POINT ( 'NONE',  ( 9.999999999999998224, 0.000000000000000000, -109.9999999999999858 ) ) ;
#28546=CARTESIAN_POINT ( 'NONE',  ( 5.405949406249999534, 9.363379034771803333, -11.78125000204835438 ) ) ;
#28547=VERTEX_POINT ( 'NONE', #10605 ) ;
#28550=CARTESIAN_POINT ( 'NONE',  ( 9.999999999999998224, 0.000000000000000000, -57.49999999999996447 ) ) ;
#28552=CARTESIAN_POINT ( 'NONE',  ( 5.000000000000000000, 8.660254037844385522, -39.24999999999997868 ) ) ;
#28553=CARTESIAN_POINT ( 'NONE',  ( 9.999999999999996447, -5.773502691896262640, -26.50000000409677270 ) ) ;
#28557=CARTESIAN_POINT ( 'NONE',  ( -10.81189881249999729, 6.242252689847871849, -141.9062500020484094 ) ) ;
#28558=CARTESIAN_POINT ( 'NONE',  ( 10.81189881249999907, 6.242252689847868297, -151.4062500020484094 ) ) ;
#28559=CARTESIAN_POINT ( 'NONE',  ( 5.000000000000000000, 8.660254037844385522, -60.24999999999997158 ) ) ;
#28563=VERTEX_POINT ( 'NONE', #14696 ) ;
#28564=EDGE_CURVE ( 'NONE', #13865, #39976, #13520, .T. ) ;
#28565=VERTEX_POINT ( 'NONE', #716 ) ;
#28566=EDGE_CURVE ( 'NONE', #31053, #31108, #17945, .T. ) ;
#28568=CARTESIAN_POINT ( 'NONE',  ( 10.81189881249999729, 0.000000000000000000, -178.3437500020483810 ) ) ;
#28569=CARTESIAN_POINT ( 'NONE',  ( 5.405949406249999534, 9.363379034771803333, -31.09375000204836326 ) ) ;
#28571=CARTESIAN_POINT ( 'NONE',  ( 5.405949406249999534, 9.363379034771803333, -166.0937500020484094 ) ) ;
#28572=CARTESIAN_POINT ( 'NONE',  ( -10.81189881249999729, 1.324075727343319199E-15, -153.5937500020483810 ) ) ;
#28573=DIRECTION ( 'NONE',  ( -0.000000000000000000, -0.000000000000000000, 1.000000000000000000 ) ) ;
#28577=CARTESIAN_POINT ( 'NONE',  ( 9.999999999999998224, 0.000000000000000000, -152.0000000000000000 ) ) ;
#28578=CARTESIAN_POINT ( 'NONE',  ( -9.999999999999998224, 1.224646799147353059E-15, -177.1250000040968189 ) ) ;
#28580=CARTESIAN_POINT ( 'NONE',  ( -10.81189881249999729, 1.324075727343319199E-15, -84.59375000204836681 ) ) ;
#28582=CARTESIAN_POINT ( 'NONE',  ( 10.81189881249999729, 0.000000000000000000, -54.03125000204836681 ) ) ;
#28583=CARTESIAN_POINT ( 'NONE',  ( 9.999999999999998224, 0.000000000000000000, -78.87500000409677625 ) ) ;
#28585=EDGE_CURVE ( 'NONE', #36032, #34991, #8178, .T. ) ;
#28586=CARTESIAN_POINT ( 'NONE',  ( -4.999999999999996447, 8.660254037844387298, -135.0000000000000000 ) ) ;
#28587=CARTESIAN_POINT ( 'NONE',  ( 7.644554776091147741E-16, 12.48450537969573659, -148.1562500020484094 ) ) ;
#28589=CARTESIAN_POINT ( 'NONE',  ( -2.121150477449813534E-15, -11.54700538379251284, -122.7500000040967905 ) ) ;
#28594=FACE_OUTER_BOUND ( 'NONE', #23133, .T. ) ;
#28595=CARTESIAN_POINT ( 'NONE',  ( 5.405949406249992428, -9.363379034771808662, -180.2812500020484094 ) ) ;
#28596=EDGE_LOOP ( 'NONE', ( #3220, #27301, #5492, #4386 ) ) ;
#28597=CARTESIAN_POINT ( 'NONE',  ( 10.00000000000000000, 5.773502691896255534, -53.25000000409676915 ) ) ;
#28599=CARTESIAN_POINT ( 'NONE',  ( 7.070501591499376803E-16, 11.54700538379251284, -130.6250000000000000 ) ) ;
#28601=CYLINDRICAL_SURFACE ( 'NONE', #31797, 9.999999999999998224 ) ;
#28602=CARTESIAN_POINT ( 'NONE',  ( -5.405949406249996869, 9.363379034771805109, -166.0312500020484094 ) ) ;
#28603=CARTESIAN_POINT ( 'NONE',  ( 12.99038105676667954, -7.500000000000051514, 49.99999999999998579 ) ) ;
#28604=DIRECTION ( 'NONE',  ( 1.000000000000000000, 0.000000000000000000, 0.000000000000000000 ) ) ;
#28606=CARTESIAN_POINT ( 'NONE',  ( 5.000000000000000000, 8.660254037844385522, -17.12500000409675138 ) ) ;
#28608=CARTESIAN_POINT ( 'NONE',  ( 5.000000000000000000, 8.660254037844385522, -27.24999999999996803 ) ) ;
#28609=CARTESIAN_POINT ( 'NONE',  ( 10.81189881249999907, 6.242252689847868297, -74.90625000204839523 ) ) ;
#28610=ORIENTED_EDGE ( 'NONE', *, *, #5677, .F. ) ;
#28612=ADVANCED_FACE ( 'NONE', ( #4293 ), #27383, .T. ) ;
#28615=ORIENTED_EDGE ( 'NONE', *, *, #6781, .T. ) ;
#28616=ADVANCED_FACE ( 'NONE', ( #30629 ), #31279, .T. ) ;
#28617=CARTESIAN_POINT ( 'NONE',  ( 10.81189881249999551, -6.242252689847874514, -29.96875000204834549 ) ) ;
#28619=CARTESIAN_POINT ( 'NONE',  ( -10.81189881249999907, -6.242252689847864744, -6.656250002048364145 ) ) ;
#28620=CARTESIAN_POINT ( 'NONE',  ( 10.81189881249999907, 6.242252689847868297, -56.71875000204838813 ) ) ;
#28625=CARTESIAN_POINT ( 'NONE',  ( -10.81189881249999729, 1.324075727343319199E-15, -191.0937500020484094 ) ) ;
#28626=CARTESIAN_POINT ( 'NONE',  ( -10.81189881249999729, 1.324075727343319199E-15, -180.5937500020484094 ) ) ;
#28629=CARTESIAN_POINT ( 'NONE',  ( 9.999999999999998224, 0.000000000000000000, -200.0000000000000000 ) ) ;
#28630=VECTOR ( 'NONE', #6242, 1000.000000000000000 ) ;
#28633=CARTESIAN_POINT ( 'NONE',  ( -10.81189881249999729, 6.242252689847871849, -101.2187500020483810 ) ) ;
#28634=CARTESIAN_POINT ( 'NONE',  ( -9.999999999999479527, -5.773502691896549521, -73.12499999999995737 ) ) ;
#28635=CARTESIAN_POINT ( 'NONE',  ( 10.81189881249999729, 0.000000000000000000, -70.53125000204838102 ) ) ;
#28636=CARTESIAN_POINT ( 'NONE',  ( -5.405949406249996869, 9.363379034771805109, -93.84375000204838102 ) ) ;
#28638=CARTESIAN_POINT ( 'NONE',  ( 5.000000000000000000, 8.660254037844385522, -144.6250000040967905 ) ) ;
#28644=FACE_OUTER_BOUND ( 'NONE', #15264, .T. ) ;
#28645=CARTESIAN_POINT ( 'NONE',  ( -9.999999999999998224, 1.224646799147353059E-15, -119.7500000000000000 ) ) ;
#28648=CARTESIAN_POINT ( 'NONE',  ( -5.000000000000003553, -8.660254037844383745, -62.49999999999997158 ) ) ;
#28650=CARTESIAN_POINT ( 'NONE',  ( 10.00000000000000000, 5.773502691896255534, -74.25000000409677625 ) ) ;
#28652=CARTESIAN_POINT ( 'NONE',  ( 4.999999999999992006, -8.660254037844389075, -11.62500000409674783 ) ) ;
#28655=CARTESIAN_POINT ( 'NONE',  ( 10.81189881249999729, 0.000000000000000000, -66.03125000204838102 ) ) ;
#28657=LINE ( 'NONE', #41581, #29835 ) ;
#28659=CARTESIAN_POINT ( 'NONE',  ( 9.999999999999998224, 0.000000000000000000, -47.37500000409677625 ) ) ;
#28660=CARTESIAN_POINT ( 'NONE',  ( -10.81189881249999729, 6.242252689847871849, -195.9062500020484094 ) ) ;
#28662=CARTESIAN_POINT ( 'NONE',  ( -10.81189881249999729, 6.242252689847871849, -6.718750002048347270 ) ) ;
#28663=CARTESIAN_POINT ( 'NONE',  ( 9.999999999999998224, 0.000000000000000000, -140.3750000040967905 ) ) ;
#28666=CARTESIAN_POINT ( 'NONE',  ( -2.121150477449813534E-15, -11.54700538379251284, -112.2500000040967763 ) ) ;
#28667=CARTESIAN_POINT ( 'NONE',  ( 5.000000000000000000, 8.660254037844385522, -174.2500000000000284 ) ) ;
#28668=CARTESIAN_POINT ( 'NONE',  ( 9.999999999999998224, 0.000000000000000000, -167.0000000000000000 ) ) ;
#28669=CARTESIAN_POINT ( 'NONE',  ( -10.81189881249999729, 6.242252689847871849, -101.4062500020483952 ) ) ;
#28670=ORIENTED_EDGE ( 'NONE', *, *, #6276, .T. ) ;
#28671=CARTESIAN_POINT ( 'NONE',  ( -2.121150477449813534E-15, -11.54700538379251284, -161.7500000040968189 ) ) ;
#28672=VERTEX_POINT ( 'NONE', #14832 ) ;
#28673=VERTEX_POINT ( 'NONE', #18300 ) ;
#28674=CARTESIAN_POINT ( 'NONE',  ( -5.405949406249996869, 9.363379034771805109, -32.53125000204837391 ) ) ;
#28676=CARTESIAN_POINT ( 'NONE',  ( -10.81189881249999729, 1.324075727343319199E-15, -81.59375000204838102 ) ) ;
#28679=( BOUNDED_CURVE ( )  B_SPLINE_CURVE ( 2, ( #25483, #19194, #9269, #12910, #31751, #22234, #42483 ),
 .UNSPECIFIED., .F., .F. ) 
 B_SPLINE_CURVE_WITH_KNOTS ( ( 3, 2, 2, 3 ),
 ( 0.4029850746268657802, 0.4042288557213931655, 0.4054726368159204397, 0.4067164179104478250 ),
 .UNSPECIFIED. ) 
 CURVE ( )  GEOMETRIC_REPRESENTATION_ITEM ( )  RATIONAL_B_SPLINE_CURVE ( ( 0.9999999999999880096, 0.8660254037844506980, 1.000000000000000000, 0.8660254037844387076, 1.000000000000000000, 0.8660254037844327124, 1.000000000000005995 ) ) 
 REPRESENTATION_ITEM ( '' )  );
#28680=VECTOR ( 'NONE', #38151, 1000.000000000000000 ) ;
#28683=CARTESIAN_POINT ( 'NONE',  ( 4.999999999999992006, -8.660254037844389075, -10.12500000409674605 ) ) ;
#28685=ADVANCED_FACE ( 'NONE', ( #21326 ), #1492, .T. ) ;
#28686=CARTESIAN_POINT ( 'NONE',  ( 5.405949406249992428, -9.363379034771808662, -129.0937500020483810 ) ) ;
#28687=CARTESIAN_POINT ( 'NONE',  ( -5.405949406250003975, -9.363379034771801557, -112.8437500020483810 ) ) ;
#28691=CARTESIAN_POINT ( 'NONE',  ( -10.00000000000000000, -5.773502691896251982, -169.5000000040967620 ) ) ;
#28692=CARTESIAN_POINT ( 'NONE',  ( 7.644554776091147741E-16, 12.48450537969573659, -173.6562500020483810 ) ) ;
#28693=( BOUNDED_CURVE ( )  B_SPLINE_CURVE ( 2, ( #15436, #28634, #6169, #27075, #23635, #24056, #10230 ),
 .UNSPECIFIED., .F., .F. ) 
 B_SPLINE_CURVE_WITH_KNOTS ( ( 3, 2, 2, 3 ),
 ( 0.6305970149253732338, 0.6318407960199006190, 0.6330845771144280043, 0.6343283582089553896 ),
 .UNSPECIFIED. ) 
 CURVE ( )  GEOMETRIC_REPRESENTATION_ITEM ( )  RATIONAL_B_SPLINE_CURVE ( ( 0.9999999999999880096, 0.8660254037844506980, 1.000000000000000000, 0.8660254037844387076, 1.000000000000000000, 0.8660254037844267172, 1.000000000000011990 ) ) 
 REPRESENTATION_ITEM ( '' )  );
#28696=CARTESIAN_POINT ( 'NONE',  ( 7.644554776091147741E-16, 12.48450537969573659, -42.96875000204835970 ) ) ;
#28698=CARTESIAN_POINT ( 'NONE',  ( 7.070501591499376803E-16, 11.54700538379251284, -86.00000000409677625 ) ) ;
#28702=CARTESIAN_POINT ( 'NONE',  ( 5.000000000000000000, 8.660254037844385522, -85.74999999999998579 ) ) ;
#28704=CARTESIAN_POINT ( 'NONE',  ( -10.00000000000000000, -5.773502691896251982, -99.00000000409679046 ) ) ;
#28707=CARTESIAN_POINT ( 'NONE',  ( -10.81189881249999729, 1.324075727343319199E-15, -101.2812500020483952 ) ) ;
#28708=EDGE_LOOP ( 'NONE', ( #32382, #4421, #9937, #42520 ) ) ;
#28712=CARTESIAN_POINT ( 'NONE',  ( 10.81189881249999907, 6.242252689847868297, -158.9062500020483810 ) ) ;
#28714=VERTEX_POINT ( 'NONE', #7747 ) ;
#28715=CARTESIAN_POINT ( 'NONE',  ( -9.999999999999998224, 1.224646799147353059E-15, -14.74999999999995737 ) ) ;
#28716=CARTESIAN_POINT ( 'NONE',  ( -10.81189881249999729, 1.324075727343319199E-15, -24.78125000204836681 ) ) ;
#28717=CARTESIAN_POINT ( 'NONE',  ( -5.000000000000003553, -8.660254037844383745, -151.0000000000000000 ) ) ;
#28719=VECTOR ( 'NONE', #184, 1000.000000000000000 ) ;
#28720=CARTESIAN_POINT ( 'NONE',  ( 7.070501591499377789E-16, 11.54700538379251284, -198.1250000000000000 ) ) ;
#28721=CARTESIAN_POINT ( 'NONE',  ( 5.405949406249992428, -9.363379034771808662, -129.2812500020483810 ) ) ;
#28722=EDGE_LOOP ( 'NONE', ( #26245, #29871, #6622, #30418 ) ) ;
#28723=CARTESIAN_POINT ( 'NONE',  ( 9.999999999999998224, 0.000000000000000000, -170.0000000000000000 ) ) ;
#28725=CARTESIAN_POINT ( 'NONE',  ( 5.405949406249992428, -9.363379034771808662, -57.28125000204836681 ) ) ;
#28727=CARTESIAN_POINT ( 'NONE',  ( -10.81189881249999729, 6.242252689847871849, -105.7187500020483668 ) ) ;
#28728=EDGE_LOOP ( 'NONE', ( #34808, #14279, #3230, #26663 ) ) ;
#28729=ORIENTED_EDGE ( 'NONE', *, *, #5611, .F. ) ;
#28730=CARTESIAN_POINT ( 'NONE',  ( -5.000000000000003553, -8.660254037844383745, -175.3750000040967905 ) ) ;
#28731=CARTESIAN_POINT ( 'NONE',  ( 4.999999999999992006, -8.660254037844389075, -197.6250000040967905 ) ) ;
#28732=CARTESIAN_POINT ( 'NONE',  ( -5.405949406249996869, 9.363379034771805109, -161.3437500020484094 ) ) ;
#28734=CARTESIAN_POINT ( 'NONE',  ( -2.293366432827344421E-15, -12.48450537969573659, -10.71875000204836681 ) ) ;
#28735=DIRECTION ( 'NONE',  ( 1.000000000000000000, 0.000000000000000000, 0.000000000000000000 ) ) ;
#28736=CARTESIAN_POINT ( 'NONE',  ( -5.405949406249996869, 9.363379034771805109, -143.3437500020483810 ) ) ;
#28740=CARTESIAN_POINT ( 'NONE',  ( 5.000000000000000000, 8.660254037844385522, -195.6250000040967905 ) ) ;
#28742=CARTESIAN_POINT ( 'NONE',  ( -5.405949406250003975, -9.363379034771801557, -192.5312500020484094 ) ) ;
#28743=CARTESIAN_POINT ( 'NONE',  ( 7.070501591499376803E-16, 11.54700538379251284, -12.12499999999996270 ) ) ;
#28747=CARTESIAN_POINT ( 'NONE',  ( -5.405949406249996869, 9.363379034771805109, -71.34375000204836681 ) ) ;
#28748=CARTESIAN_POINT ( 'NONE',  ( -2.293366432827344421E-15, -12.48450537969573659, -54.21875000204838102 ) ) ;
#28750=CARTESIAN_POINT ( 'NONE',  ( 10.81189881249999907, 6.242252689847868297, -26.90625000204838102 ) ) ;
#28752=CARTESIAN_POINT ( 'NONE',  ( -9.999999999999998224, 1.224646799147353059E-15, -8.749999999999952038 ) ) ;
#28754=CARTESIAN_POINT ( 'NONE',  ( -5.000000000000003553, -8.660254037844383745, -111.9999999999999858 ) ) ;
#28759=CARTESIAN_POINT ( 'NONE',  ( -10.81189881249999729, 6.242252689847871849, -12.90625000204835970 ) ) ;
#28761=DIRECTION ( 'NONE',  ( -0.000000000000000000, -0.000000000000000000, 1.000000000000000000 ) ) ;
#28765=CARTESIAN_POINT ( 'NONE',  ( -10.00000000000000000, -5.773502691896251982, -40.12499999999996447 ) ) ;
#28766=CARTESIAN_POINT ( 'NONE',  ( 4.999999999999992006, -8.660254037844389075, -25.12500000409675849 ) ) ;
#28767=CARTESIAN_POINT ( 'NONE',  ( 5.405949406249999534, 9.363379034771803333, -52.28125000204835970 ) ) ;
#28771=CARTESIAN_POINT ( 'NONE',  ( -5.405949406250003975, -9.363379034771801557, -147.5312500020483810 ) ) ;
#28772=CARTESIAN_POINT ( 'NONE',  ( 7.644554776091147741E-16, 12.48450537969573659, -146.6562500020484379 ) ) ;
#28775=CARTESIAN_POINT ( 'NONE',  ( -9.999999999998969713, -5.773502691896847949, -58.12499999999997158 ) ) ;
#28776=ORIENTED_EDGE ( 'NONE', *, *, #38356, .T. ) ;
#28778=ORIENTED_EDGE ( 'NONE', *, *, #36000, .F. ) ;
#28779=CARTESIAN_POINT ( 'NONE',  ( -2.121150477449813534E-15, -11.54700538379251284, -100.2500000040967905 ) ) ;
#28780=CARTESIAN_POINT ( 'NONE',  ( -10.81189881249999907, -6.242252689847864744, -184.9687500020484094 ) ) ;
#28781=CARTESIAN_POINT ( 'NONE',  ( 10.81189881249999907, 6.242252689847868297, -29.71875000204834194 ) ) ;
#28782=CARTESIAN_POINT ( 'NONE',  ( 5.000000000000000000, 8.660254037844385522, -118.7500000000000000 ) ) ;
#28783=CARTESIAN_POINT ( 'NONE',  ( -10.81189881249999729, -6.242252689847864744, -163.9687500020483526 ) ) ;
#28784=CARTESIAN_POINT ( 'NONE',  ( 10.81189881249999729, 0.000000000000000000, -152.8437500020483810 ) ) ;
#28785=DIRECTION ( 'NONE',  ( 1.000000000000000000, 0.000000000000000000, 0.000000000000000000 ) ) ;
#28788=CARTESIAN_POINT ( 'NONE',  ( 10.81189881249999729, 0.000000000000000000, -16.34375000204835260 ) ) ;
#28791=CARTESIAN_POINT ( 'NONE',  ( 5.000000000000000000, 8.660254037844385522, -177.6250000040968189 ) ) ;
#28793=CARTESIAN_POINT ( 'NONE',  ( -10.81189881249999907, -6.242252689847864744, -84.46875000204836681 ) ) ;
#28794=CARTESIAN_POINT ( 'NONE',  ( -4.999999999999996447, 8.660254037844387298, -184.8750000040967905 ) ) ;
#28795=CARTESIAN_POINT ( 'NONE',  ( 5.405949406249992428, -9.363379034771808662, -51.28125000204835970 ) ) ;
#28799=CARTESIAN_POINT ( 'NONE',  ( 4.999999999999992006, -8.660254037844389075, -137.2499999999999716 ) ) ;
#28800=CARTESIAN_POINT ( 'NONE',  ( 7.644554776091147741E-16, 12.48450537969573659, -143.6562500020484094 ) ) ;
#28801=CARTESIAN_POINT ( 'NONE',  ( 0.000000000000000000, 0.000000000000000000, -200.0000000000000000 ) ) ;
#28803=CARTESIAN_POINT ( 'NONE',  ( -10.00000000000000000, -5.773502691896251982, -126.0000000040967905 ) ) ;
#28808=CARTESIAN_POINT ( 'NONE',  ( -4.999999999999996447, 8.660254037844387298, -52.49999999999996447 ) ) ;
#28809=CARTESIAN_POINT ( 'NONE',  ( -5.405949406250003975, -9.363379034771801557, -171.5312500020484094 ) ) ;
#28810=CARTESIAN_POINT ( 'NONE',  ( 9.999999999999996447, -5.773502691896262640, -50.50000000409675494 ) ) ;
#28811=EDGE_CURVE ( 'NONE', #35065, #16036, #37303, .T. ) ;
#28812=FACE_OUTER_BOUND ( 'NONE', #19042, .T. ) ;
#28813=ADVANCED_FACE ( 'NONE', ( #11180 ), #37087, .T. ) ;
#28815=( BOUNDED_CURVE ( )  B_SPLINE_CURVE ( 2, ( #1016, #1876, #4666, #40902, #1656, #33821, #17597 ),
 .UNSPECIFIED., .F., .F. ) 
 B_SPLINE_CURVE_WITH_KNOTS ( ( 3, 2, 2, 3 ),
 ( 0.000000000000000000, 0.001243781094527364461, 0.002487562189054728923, 0.003731343283582092950 ),
 .UNSPECIFIED. ) 
 CURVE ( )  GEOMETRIC_REPRESENTATION_ITEM ( )  RATIONAL_B_SPLINE_CURVE ( ( 1.000000000000000000, 0.8660254037844387076, 1.000000000000000000, 0.8660254037844387076, 1.000000000000000000, 0.8660254037844383745, 1.000000000000000444 ) ) 
 REPRESENTATION_ITEM ( '' )  );
#28816=CARTESIAN_POINT ( 'NONE',  ( -9.999999999999998224, 1.224646799147353059E-15, -83.74999999999997158 ) ) ;
#28817=CARTESIAN_POINT ( 'NONE',  ( 7.644554776091147741E-16, 12.48450537969573659, -172.1562500020484094 ) ) ;
#28821=CARTESIAN_POINT ( 'NONE',  ( -4.999999999999996447, 8.660254037844387298, -177.0000000000000000 ) ) ;
#28822=CARTESIAN_POINT ( 'NONE',  ( 5.000000000000000000, 8.660254037844385522, -137.1250000040967620 ) ) ;
#28823=CARTESIAN_POINT ( 'NONE',  ( -2.293366432827344421E-15, -12.48450537969573659, -75.40625000204838102 ) ) ;
#28824=VERTEX_POINT ( 'NONE', #34297 ) ;
#28826=ORIENTED_EDGE ( 'NONE', *, *, #19513, .T. ) ;
#28827=EDGE_LOOP ( 'NONE', ( #21193, #2947, #31852, #16459 ) ) ;
#28828=CARTESIAN_POINT ( 'NONE',  ( 5.405949406249999534, 9.363379034771803333, -26.59375000204835970 ) ) ;
#28829=CARTESIAN_POINT ( 'NONE',  ( -5.000000000000003553, -8.660254037844383745, -170.8750000040968189 ) ) ;
#28830=CARTESIAN_POINT ( 'NONE',  ( 10.81189881249999551, -6.242252689847874514, -6.156250002048360592 ) ) ;
#28831=CARTESIAN_POINT ( 'NONE',  ( -10.81189881249999907, -6.242252689847864744, -52.96875000204838102 ) ) ;
#28833=CYLINDRICAL_SURFACE ( 'NONE', #25465, 9.999999999999998224 ) ;
#28835=CARTESIAN_POINT ( 'NONE',  ( 10.81189881249999729, 0.000000000000000000, -187.3437500020483810 ) ) ;
#28836=CARTESIAN_POINT ( 'NONE',  ( -5.405949406250003975, -9.363379034771801557, -174.3437500020484094 ) ) ;
#28839=CARTESIAN_POINT ( 'NONE',  ( -9.999999999999998224, 1.224646799147353059E-15, -192.1250000040967905 ) ) ;
#28841=CARTESIAN_POINT ( 'NONE',  ( 10.81189881249999551, -6.242252689847874514, -101.9687500020483810 ) ) ;
#28842=CARTESIAN_POINT ( 'NONE',  ( 5.000000000000000000, 8.660254037844385522, -18.24999999999996092 ) ) ;
#28843=CARTESIAN_POINT ( 'NONE',  ( 10.81189881249999551, -6.242252689847874514, -75.15625000204838102 ) ) ;
#28844=CARTESIAN_POINT ( 'NONE',  ( -10.81189881249999729, 1.324075727343319199E-15, -93.59375000204838102 ) ) ;
#28847=CARTESIAN_POINT ( 'NONE',  ( 7.070501591499377789E-16, 11.54700538379251284, -144.5000000040967905 ) ) ;
#28849=VERTEX_POINT ( 'NONE', #20681 ) ;
#28852=CARTESIAN_POINT ( 'NONE',  ( 10.81189881249999729, 0.000000000000000000, -199.5312500020484094 ) ) ;
#28853=LINE ( 'NONE', #8989, #19920 ) ;
#28855=ORIENTED_EDGE ( 'NONE', *, *, #26353, .F. ) ;
#28856=CARTESIAN_POINT ( 'NONE',  ( -9.999999999999998224, 1.224646799147353059E-15, -67.24999999999997158 ) ) ;
#28858=CARTESIAN_POINT ( 'NONE',  ( 5.000000000000000000, 8.660254037844385522, -77.12500000409677625 ) ) ;
#28860=DIRECTION ( 'NONE',  ( -0.000000000000000000, -0.000000000000000000, 1.000000000000000000 ) ) ;
#28861=DIRECTION ( 'NONE',  ( -0.000000000000000000, -0.000000000000000000, 1.000000000000000000 ) ) ;
#28863=CARTESIAN_POINT ( 'NONE',  ( 10.81189881249999729, 6.242252689847867408, -64.40625000204838102 ) ) ;
#28864=EDGE_CURVE ( 'NONE', #37716, #31913, #17685, .T. ) ;
#28866=CARTESIAN_POINT ( 'NONE',  ( 7.070501591499376803E-16, 11.54700538379251284, -93.50000000409676204 ) ) ;
#28868=CARTESIAN_POINT ( 'NONE',  ( 7.070501591499376803E-16, 11.54700538379251284, -47.00000000409676915 ) ) ;
#28869=CARTESIAN_POINT ( 'NONE',  ( -2.293366432827344421E-15, -12.48450537969573659, -189.4062500020484094 ) ) ;
#28871=CARTESIAN_POINT ( 'NONE',  ( -10.81189881249999729, -6.242252689847864744, -4.968750002048339276 ) ) ;
#28872=CARTESIAN_POINT ( 'NONE',  ( 9.999999999999998224, 0.000000000000000000, -6.875000004096742501 ) ) ;
#28873=CARTESIAN_POINT ( 'NONE',  ( -5.000000000000003553, -8.660254037844383745, -37.37500000409676915 ) ) ;
#28875=CARTESIAN_POINT ( 'NONE',  ( 0.000000000000000000, 0.000000000000000000, -200.0000000000000000 ) ) ;
#28876=CARTESIAN_POINT ( 'NONE',  ( 7.070501591499377789E-16, 11.54700538379251284, -175.6250000000000000 ) ) ;
#28877=CARTESIAN_POINT ( 'NONE',  ( 9.999999999999479527, 5.773502691896553074, -97.87499999999997158 ) ) ;
#28878=CARTESIAN_POINT ( 'NONE',  ( 5.405949406249992428, -9.363379034771808662, -102.2812500020483952 ) ) ;
#28879=ORIENTED_EDGE ( 'NONE', *, *, #7820, .F. ) ;
#28881=VECTOR ( 'NONE', #7603, 1000.000000000000000 ) ;
#28882=ORIENTED_EDGE ( 'NONE', *, *, #13919, .T. ) ;
#28884=CARTESIAN_POINT ( 'NONE',  ( 7.644554776091147741E-16, 12.48450537969573659, -26.65625000204837747 ) ) ;
#28887=CARTESIAN_POINT ( 'NONE',  ( -5.405949406249996869, 9.363379034771805109, -78.84375000204838102 ) ) ;
#28889=CARTESIAN_POINT ( 'NONE',  ( 9.999999999999998224, 0.000000000000000000, -126.5000000000000000 ) ) ;
#28890=CARTESIAN_POINT ( 'NONE',  ( 9.999999999998969713, 5.773502691896851502, -69.75000000409677625 ) ) ;
#28893=CARTESIAN_POINT ( 'NONE',  ( -9.999999999999998224, 5.773502691896259087, -9.250000004096756712 ) ) ;
#28894=CARTESIAN_POINT ( 'NONE',  ( -9.999999999999998224, 1.224646799147353059E-15, -77.74999999999998579 ) ) ;
#28895=CARTESIAN_POINT ( 'NONE',  ( -10.81189881249999729, 6.242252689847871849, -131.2187500020483810 ) ) ;
#28896=CARTESIAN_POINT ( 'NONE',  ( -10.81189881249999729, 1.324075727343319199E-15, -114.5937500020483810 ) ) ;
#28899=CARTESIAN_POINT ( 'NONE',  ( 9.999999999999998224, 0.000000000000000000, -167.3750000040967905 ) ) ;
#28900=FACE_OUTER_BOUND ( 'NONE', #35670, .T. ) ;
#28903=CARTESIAN_POINT ( 'NONE',  ( -10.81189881249999729, 1.324075727343319199E-15, -45.59375000204838102 ) ) ;
#28905=CARTESIAN_POINT ( 'NONE',  ( 7.644554776091147741E-16, 12.48450537969573659, -2.656250002048344161 ) ) ;
#28909=CARTESIAN_POINT ( 'NONE',  ( 10.00000000000000000, 5.773502691896255534, -91.87499999999998579 ) ) ;
#28911=CARTESIAN_POINT ( 'NONE',  ( 9.999999999999998224, 0.000000000000000000, -95.37500000409677625 ) ) ;
#28912=CYLINDRICAL_SURFACE ( 'NONE', #2440, 9.999999999999998224 ) ;
#28914=CARTESIAN_POINT ( 'NONE',  ( 7.644554776091147741E-16, 12.48450537969573659, -92.65625000204838102 ) ) ;
#28915=ORIENTED_EDGE ( 'NONE', *, *, #14492, .F. ) ;
#28920=CARTESIAN_POINT ( 'NONE',  ( 4.999999999999992006, -8.660254037844389075, -17.24999999999996092 ) ) ;
#28922=CARTESIAN_POINT ( 'NONE',  ( -2.293366432827344421E-15, -12.48450537969573659, -22.90625000204837391 ) ) ;
#28923=CARTESIAN_POINT ( 'NONE',  ( 7.070501591499377789E-16, 11.54700538379251284, -150.1250000000000000 ) ) ;
#28925=AXIS2_PLACEMENT_3D ( 'NONE', #39323, #22514, #16857 ) ;
#28927=CARTESIAN_POINT ( 'NONE',  ( 7.644554776091147741E-16, 12.48450537969573659, -124.1562500020483952 ) ) ;
#28928=EDGE_LOOP ( 'NONE', ( #12134, #39782, #16521, #30756 ) ) ;
#28929=CARTESIAN_POINT ( 'NONE',  ( 7.070501591499376803E-16, 11.54700538379251284, -90.12500000000000000 ) ) ;
#28930=EDGE_LOOP ( 'NONE', ( #26307, #10453, #7022, #34934 ) ) ;
#28931=( BOUNDED_CURVE ( )  B_SPLINE_CURVE ( 2, ( #23026, #28877, #13068, #22597, #16092, #32329, #39205 ),
 .UNSPECIFIED., .F., .F. ) 
 B_SPLINE_CURVE_WITH_KNOTS ( ( 3, 2, 2, 3 ),
 ( 0.5074626865671643117, 0.5087064676616916969, 0.5099502487562189712, 0.5111940298507463565 ),
 .UNSPECIFIED. ) 
 CURVE ( )  GEOMETRIC_REPRESENTATION_ITEM ( )  RATIONAL_B_SPLINE_CURVE ( ( 0.9999999999999880096, 0.8660254037844506980, 1.000000000000000000, 0.8660254037844387076, 1.000000000000000000, 0.8660254037844267172, 1.000000000000011990 ) ) 
 REPRESENTATION_ITEM ( '' )  );
#28932=CARTESIAN_POINT ( 'NONE',  ( -5.405949406249996869, 9.363379034771805109, -53.53125000204836681 ) ) ;
#28934=CARTESIAN_POINT ( 'NONE',  ( 7.644554776091147741E-16, 12.48450537969573659, -105.9687500020483668 ) ) ;
#28935=ORIENTED_EDGE ( 'NONE', *, *, #19755, .F. ) ;
#28936=ORIENTED_EDGE ( 'NONE', *, *, #19100, .F. ) ;
#28937=DIRECTION ( 'NONE',  ( 1.000000000000000000, 0.000000000000000000, 0.000000000000000000 ) ) ;
#28938=CARTESIAN_POINT ( 'NONE',  ( -5.000000000000003553, -8.660254037844383745, -184.0000000000000000 ) ) ;
#28939=CARTESIAN_POINT ( 'NONE',  ( 5.405949406249999534, 9.363379034771803333, -151.0937500020483810 ) ) ;
#28941=CARTESIAN_POINT ( 'NONE',  ( -10.81189881249999729, 1.324075727343319199E-15, -3.593750002048368142 ) ) ;
#28943=CARTESIAN_POINT ( 'NONE',  ( 5.405949406249992428, -9.363379034771808662, -139.5937500020483810 ) ) ;
#28945=CARTESIAN_POINT ( 'NONE',  ( 10.00000000000025402, -5.773502691896113426, -158.1250000000000284 ) ) ;
#28947=CARTESIAN_POINT ( 'NONE',  ( 5.000000000000000000, 8.660254037844385522, -191.1250000040967905 ) ) ;
#28949=CARTESIAN_POINT ( 'NONE',  ( -10.81189881249999729, 6.242252689847871849, -195.9062500020484094 ) ) ;
#28950=FACE_OUTER_BOUND ( 'NONE', #22443, .T. ) ;
#28953=CARTESIAN_POINT ( 'NONE',  ( -5.405949406250003975, -9.363379034771801557, -64.84375000204836681 ) ) ;
#28954=CARTESIAN_POINT ( 'NONE',  ( -10.81189881249999729, 1.324075727343319199E-15, -53.09375000204835970 ) ) ;
#28956=CARTESIAN_POINT ( 'NONE',  ( -2.293366432827344421E-15, -12.48450537969573659, -24.40625000204838457 ) ) ;
#28958=CARTESIAN_POINT ( 'NONE',  ( -5.000000000000003553, -8.660254037844383745, -8.499999999999952038 ) ) ;
#28960=CARTESIAN_POINT ( 'NONE',  ( 7.070501591499377789E-16, 11.54700538379251284, -115.6249999999999858 ) ) ;
#28963=CARTESIAN_POINT ( 'NONE',  ( 5.405949406249999534, 9.363379034771803333, -115.2812500020483952 ) ) ;
#28964=ORIENTED_EDGE ( 'NONE', *, *, #42062, .T. ) ;
#28965=DIRECTION ( 'NONE',  ( -0.000000000000000000, -0.000000000000000000, 1.000000000000000000 ) ) ;
#28969=CARTESIAN_POINT ( 'NONE',  ( 5.000000000000000000, 8.660254037844385522, -37.74999999999997868 ) ) ;
#28970=CARTESIAN_POINT ( 'NONE',  ( 9.999999999999996447, -5.773502691896262640, -28.00000000409678336 ) ) ;
#28971=CARTESIAN_POINT ( 'NONE',  ( -5.405949406250003975, -9.363379034771801557, -50.03125000204838813 ) ) ;
#28975=CARTESIAN_POINT ( 'NONE',  ( -10.81189881249999907, -6.242252689847864744, -143.1562500020484094 ) ) ;
#28976=AXIS2_PLACEMENT_3D ( 'NONE', #29499, #42010, #32739 ) ;
#28977=CARTESIAN_POINT ( 'NONE',  ( 10.81189881249999729, 0.000000000000000000, -148.5312500020483810 ) ) ;
#28978=CARTESIAN_POINT ( 'NONE',  ( -10.00000000000019185, 5.773502691896147176, -190.3750000000000284 ) ) ;
#28980=EDGE_LOOP ( 'NONE', ( #27909, #19287, #166, #20775 ) ) ;
#28981=ORIENTED_EDGE ( 'NONE', *, *, #25637, .T. ) ;
#28982=VERTEX_POINT ( 'NONE', #25020 ) ;
#28983=ADVANCED_FACE ( 'NONE', ( #6003 ), #31705, .T. ) ;
#28984=CYLINDRICAL_SURFACE ( 'NONE', #13174, 9.999999999999998224 ) ;
#28985=CARTESIAN_POINT ( 'NONE',  ( 5.405949406249999534, 9.363379034771803333, -182.5937500020483810 ) ) ;
#28986=CARTESIAN_POINT ( 'NONE',  ( -10.81189881249999729, 6.242252689847871849, -27.71875000204838102 ) ) ;
#28987=DIRECTION ( 'NONE',  ( 1.000000000000000000, 0.000000000000000000, 0.000000000000000000 ) ) ;
#28988=CARTESIAN_POINT ( 'NONE',  ( -10.81189881249999729, 1.324075727343319199E-15, -165.5937500020484094 ) ) ;
#28989=CARTESIAN_POINT ( 'NONE',  ( 10.81189881249999551, -6.242252689847874514, -143.9687500020483810 ) ) ;
#28990=CARTESIAN_POINT ( 'NONE',  ( 9.999999999999998224, 0.000000000000000000, -125.3750000040967905 ) ) ;
#28993=CARTESIAN_POINT ( 'NONE',  ( 5.405949406249992428, -9.363379034771808662, -19.59375000204835615 ) ) ;
#28995=CARTESIAN_POINT ( 'NONE',  ( -4.999999999999996447, 8.660254037844387298, -135.0000000000000000 ) ) ;
#28998=CARTESIAN_POINT ( 'NONE',  ( 10.81189881249999551, -6.242252689847874514, -80.96875000204838102 ) ) ;
#28999=CARTESIAN_POINT ( 'NONE',  ( -5.405949406250003975, -9.363379034771801557, -50.03125000204838813 ) ) ;
#29001=CARTESIAN_POINT ( 'NONE',  ( -9.999999999999998224, 1.224646799147353059E-15, -90.12500000409677625 ) ) ;
#29003=VECTOR ( 'NONE', #12332, 1000.000000000000114 ) ;
#29004=CARTESIAN_POINT ( 'NONE',  ( -2.121150477449813534E-15, -11.54700538379251284, -134.3750000000000000 ) ) ;
#29005=CARTESIAN_POINT ( 'NONE',  ( 10.81189881249999729, 0.000000000000000000, -145.5312500020483810 ) ) ;
#29006=LINE ( 'NONE', #5709, #28243 ) ;
#29007=CARTESIAN_POINT ( 'NONE',  ( 7.070501591499377789E-16, 11.54700538379251284, -119.0000000040967763 ) ) ;
#29009=ORIENTED_EDGE ( 'NONE', *, *, #38610, .T. ) ;
#29013=ADVANCED_FACE ( 'NONE', ( #32340 ), #41807, .T. ) ;
#29014=CARTESIAN_POINT ( 'NONE',  ( 5.405949406249992428, -9.363379034771808662, -171.2812500020484094 ) ) ;
#29015=CARTESIAN_POINT ( 'NONE',  ( -9.999999999999998224, 5.773502691896259087, -49.75000000409675494 ) ) ;
#29016=( BOUNDED_CURVE ( )  B_SPLINE_CURVE ( 2, ( #29418, #3729, #26600, #13196, #16859, #6745, #42346 ),
 .UNSPECIFIED., .F., .F. ) 
 B_SPLINE_CURVE_WITH_KNOTS ( ( 3, 2, 2, 3 ),
 ( 0.7089552238805972850, 0.7101990049751245593, 0.7114427860696519446, 0.7126865671641793298 ),
 .UNSPECIFIED. ) 
 CURVE ( )  GEOMETRIC_REPRESENTATION_ITEM ( )  RATIONAL_B_SPLINE_CURVE ( ( 0.9999999999999761302, 0.8660254037844625774, 1.000000000000000000, 0.8660254037844387076, 1.000000000000000000, 0.8660254037844148378, 1.000000000000023981 ) ) 
 REPRESENTATION_ITEM ( '' )  );
#29017=LINE ( 'NONE', #19279, #21465 ) ;
#29019=ADVANCED_FACE ( 'NONE', ( #8812 ), #19151, .T. ) ;
#29020=CARTESIAN_POINT ( 'NONE',  ( 10.81189881249999551, -6.242252689847874514, -166.6562500020484094 ) ) ;
#29021=CARTESIAN_POINT ( 'NONE',  ( -9.999999999999998224, 1.224646799147353059E-15, -183.1250000040967905 ) ) ;
#29022=CARTESIAN_POINT ( 'NONE',  ( 9.999999999999998224, 0.000000000000000000, -188.3750000040967905 ) ) ;
#29023=ORIENTED_EDGE ( 'NONE', *, *, #9068, .T. ) ;
#29027=CARTESIAN_POINT ( 'NONE',  ( 5.405949406249992428, -9.363379034771808662, -78.28125000204838102 ) ) ;
#29028=ORIENTED_EDGE ( 'NONE', *, *, #40673, .T. ) ;
#29030=CARTESIAN_POINT ( 'NONE',  ( -9.999999999999479527, -5.773502691896549521, -119.6249999999999858 ) ) ;
#29033=CARTESIAN_POINT ( 'NONE',  ( -10.81189881249999729, -6.242252689847864744, -30.46875000204834549 ) ) ;
#29035=CARTESIAN_POINT ( 'NONE',  ( -10.81189881249999729, 1.324075727343319199E-15, -5.281250002048376579 ) ) ;
#29036=CARTESIAN_POINT ( 'NONE',  ( 10.81189881249999729, 0.000000000000000000, -52.34375000204835260 ) ) ;
#29037=ORIENTED_EDGE ( 'NONE', *, *, #5674, .T. ) ;
#29038=DIRECTION ( 'NONE',  ( 1.000000000000000000, 0.000000000000000000, 0.000000000000000000 ) ) ;
#29039=EDGE_CURVE ( 'NONE', #14564, #10480, #26530, .T. ) ;
#29041=CARTESIAN_POINT ( 'NONE',  ( 10.81189881249999551, -6.242252689847874514, -191.9687500020484379 ) ) ;
#29042=CARTESIAN_POINT ( 'NONE',  ( 5.405949406249992428, -9.363379034771808662, -175.5937500020484094 ) ) ;
#29048=CARTESIAN_POINT ( 'NONE',  ( 5.405949406249999534, 9.363379034771803333, -107.5937500020483810 ) ) ;
#29049=DIRECTION ( 'NONE',  ( -0.000000000000000000, -0.000000000000000000, 1.000000000000000000 ) ) ;
#29050=CARTESIAN_POINT ( 'NONE',  ( 10.81189881249999551, -6.242252689847874514, -73.65625000204836681 ) ) ;
#29052=CARTESIAN_POINT ( 'NONE',  ( 5.405949406249992428, -9.363379034771808662, -84.09375000204836681 ) ) ;
#29054=CARTESIAN_POINT ( 'NONE',  ( -4.999999999999996447, 8.660254037844387298, -148.8750000040967905 ) ) ;
#29057=VERTEX_POINT ( 'NONE', #9444 ) ;
#29061=CARTESIAN_POINT ( 'NONE',  ( 5.405949406249992428, -9.363379034771808662, -195.2812500020484094 ) ) ;
#29065=CARTESIAN_POINT ( 'NONE',  ( -10.00000000000000000, -5.773502691896251982, -68.62499999999998579 ) ) ;
#29067=CARTESIAN_POINT ( 'NONE',  ( 7.070501591499377789E-16, 11.54700538379251284, -71.00000000409676204 ) ) ;
#29068=CARTESIAN_POINT ( 'NONE',  ( 8.660254037844463681, -15.00000000000009948, 49.99999999999998579 ) ) ;
#29069=DIRECTION ( 'NONE',  ( 1.000000000000000000, 0.000000000000000000, 0.000000000000000000 ) ) ;
#29071=CARTESIAN_POINT ( 'NONE',  ( 5.405949406249992428, -9.363379034771808662, -67.78125000204838102 ) ) ;
#29075=CARTESIAN_POINT ( 'NONE',  ( 5.405949406249999534, 9.363379034771803333, -196.2812500020484094 ) ) ;
#29078=CARTESIAN_POINT ( 'NONE',  ( 10.81189881249999729, 0.000000000000000000, -7.343750002048343717 ) ) ;
#29079=CARTESIAN_POINT ( 'NONE',  ( 0.000000000000000000, 0.000000000000000000, -200.0000000000000000 ) ) ;
#29080=DIRECTION ( 'NONE',  ( -0.000000000000000000, -0.000000000000000000, 1.000000000000000000 ) ) ;
#29081=CARTESIAN_POINT ( 'NONE',  ( -9.999999999999227285, -5.773502691896698735, -137.6249999999999716 ) ) ;
#29082=CARTESIAN_POINT ( 'NONE',  ( -2.121150477449813534E-15, -11.54700538379251284, -174.8750000000000000 ) ) ;
#29083=LINE ( 'NONE', #9641, #17911 ) ;
#29084=CARTESIAN_POINT ( 'NONE',  ( 10.81189881249999907, 6.242252689847868297, -100.4062500020483952 ) ) ;
#29087=VERTEX_POINT ( 'NONE', #15891 ) ;
#29088=ORIENTED_EDGE ( 'NONE', *, *, #7502, .T. ) ;
#29090=CARTESIAN_POINT ( 'NONE',  ( 10.81189881249999729, 0.000000000000000000, -30.03125000204837036 ) ) ;
#29093=CARTESIAN_POINT ( 'NONE',  ( 5.405949406249992428, -9.363379034771808662, -79.59375000204838102 ) ) ;
#29096=CARTESIAN_POINT ( 'NONE',  ( 5.405949406249999534, 9.363379034771803333, -199.0937500020484094 ) ) ;
#29098=CARTESIAN_POINT ( 'NONE',  ( -4.999999999999996447, 8.660254037844387298, -69.37500000409677625 ) ) ;
#29099=DIRECTION ( 'NONE',  ( 1.000000000000000000, 0.000000000000000000, 0.000000000000000000 ) ) ;
#29101=CARTESIAN_POINT ( 'NONE',  ( -5.000000000000003553, -8.660254037844383745, -14.87500000409674961 ) ) ;
#29102=VECTOR ( 'NONE', #33111, 1000.000000000000000 ) ;
#29103=CARTESIAN_POINT ( 'NONE',  ( 9.999999999999998224, 0.000000000000000000, -126.5000000000000000 ) ) ;
#29104=CARTESIAN_POINT ( 'NONE',  ( -10.81189881249999907, -6.242252689847864744, -126.4687500020483810 ) ) ;
#29105=CARTESIAN_POINT ( 'NONE',  ( 10.81189881249999729, 0.000000000000000000, -96.03125000204838102 ) ) ;
#29106=CARTESIAN_POINT ( 'NONE',  ( 5.405949406249992428, -9.363379034771808662, -109.5937500020483810 ) ) ;
#29109=CARTESIAN_POINT ( 'NONE',  ( 4.999999999999992006, -8.660254037844389075, -166.1250000040967905 ) ) ;
#29110=CARTESIAN_POINT ( 'NONE',  ( 9.999999999998969713, 5.773502691896851502, -81.75000000409673362 ) ) ;
#29114=CARTESIAN_POINT ( 'NONE',  ( 9.999999999998969713, 5.773502691896851502, -86.25000000409676204 ) ) ;
#29118=CARTESIAN_POINT ( 'NONE',  ( -10.00000000000000000, -5.773502691896251982, -89.62499999999997158 ) ) ;
#29120=CARTESIAN_POINT ( 'NONE',  ( -5.000000000000003553, -8.660254037844383745, -101.8750000040967905 ) ) ;
#29124=CARTESIAN_POINT ( 'NONE',  ( -2.293366432827344421E-15, -12.48450537969573659, -91.90625000204838102 ) ) ;
#29125=ORIENTED_EDGE ( 'NONE', *, *, #2743, .T. ) ;
#29130=CARTESIAN_POINT ( 'NONE',  ( -9.999999999999998224, 5.773502691896259087, -19.37499999999998224 ) ) ;
#29131=CARTESIAN_POINT ( 'NONE',  ( -2.121150477449813534E-15, -11.54700538379251284, -155.3750000000000000 ) ) ;
#29135=CARTESIAN_POINT ( 'NONE',  ( 10.81189881249999551, -6.242252689847874514, -126.1562500020483810 ) ) ;
#29136=ORIENTED_EDGE ( 'NONE', *, *, #33578, .T. ) ;
#29137=ORIENTED_EDGE ( 'NONE', *, *, #42633, .T. ) ;
#29138=CARTESIAN_POINT ( 'NONE',  ( -5.405949406250003975, -9.363379034771801557, -50.03125000204838813 ) ) ;
#29140=CARTESIAN_POINT ( 'NONE',  ( 10.81189881249999551, -6.242252689847874514, -100.4687500020483952 ) ) ;
#29141=ORIENTED_EDGE ( 'NONE', *, *, #9126, .F. ) ;
#29142=ORIENTED_EDGE ( 'NONE', *, *, #889, .T. ) ;
#29143=LINE ( 'NONE', #25491, #23176 ) ;
#29144=CARTESIAN_POINT ( 'NONE',  ( -9.999999999999998224, 1.224646799147353059E-15, -32.74999999999997158 ) ) ;
#29147=CARTESIAN_POINT ( 'NONE',  ( 9.999999999999998224, 0.000000000000000000, -200.0000000000000000 ) ) ;
#29148=FACE_OUTER_BOUND ( 'NONE', #13742, .T. ) ;
#29150=CARTESIAN_POINT ( 'NONE',  ( 10.81189881249999551, -6.242252689847874514, -142.4687500020483810 ) ) ;
#29154=CARTESIAN_POINT ( 'NONE',  ( 9.999999999999996447, -5.773502691896262640, -193.0000000040968473 ) ) ;
#29156=CARTESIAN_POINT ( 'NONE',  ( 10.81189881249999729, 6.242252689847867408, -187.4062500020484094 ) ) ;
#29157=CARTESIAN_POINT ( 'NONE',  ( -9.999999999999479527, -5.773502691896549521, -47.62499999999995737 ) ) ;
#29160=CARTESIAN_POINT ( 'NONE',  ( 10.81189881249999551, -6.242252689847874514, -65.96875000204836681 ) ) ;
#29161=CARTESIAN_POINT ( 'NONE',  ( -5.405949406250003975, -9.363379034771801557, -48.34375000204838102 ) ) ;
#29163=CARTESIAN_POINT ( 'NONE',  ( -10.81189881249999907, -6.242252689847864744, -29.15625000204835970 ) ) ;
#29167=CARTESIAN_POINT ( 'NONE',  ( 9.999999999999998224, 0.000000000000000000, -112.9999999999999858 ) ) ;
#29171=CARTESIAN_POINT ( 'NONE',  ( -10.81189881249999729, 1.324075727343319199E-15, -117.7812500020483952 ) ) ;
#29172=EDGE_CURVE ( 'NONE', #5198, #37673, #10254, .T. ) ;
#29173=EDGE_LOOP ( 'NONE', ( #12132, #36868, #5942, #39775 ) ) ;
#29176=CYLINDRICAL_SURFACE ( 'NONE', #36026, 9.999999999999998224 ) ;
#29178=CARTESIAN_POINT ( 'NONE',  ( 9.999999999999996447, -5.773502691896262640, -44.12499999999997158 ) ) ;
#29179=CARTESIAN_POINT ( 'NONE',  ( 9.999999999999996447, -5.773502691896262640, -25.00000000409676915 ) ) ;
#29180=CARTESIAN_POINT ( 'NONE',  ( 10.81189881249999729, 6.242252689847867408, -44.90625000204836681 ) ) ;
#29186=CARTESIAN_POINT ( 'NONE',  ( 10.81189881249999907, 6.242252689847868297, -139.4062500020484094 ) ) ;
#29187=CARTESIAN_POINT ( 'NONE',  ( -5.405949406250003975, -9.363379034771801557, -147.5312500020483810 ) ) ;
#29193=CARTESIAN_POINT ( 'NONE',  ( 10.81189881249999729, 0.000000000000000000, -170.8437500020484094 ) ) ;
#29194=CARTESIAN_POINT ( 'NONE',  ( -5.405949406249996869, 9.363379034771805109, -29.34375000204836326 ) ) ;
#29196=CARTESIAN_POINT ( 'NONE',  ( 10.81189881249999729, 0.000000000000000000, -167.8437500020484094 ) ) ;
#29197=CARTESIAN_POINT ( 'NONE',  ( -5.405949406250003975, -9.363379034771801557, -147.3437500020483810 ) ) ;
#29201=CARTESIAN_POINT ( 'NONE',  ( -10.81189881249999907, -6.242252689847864744, -15.46875000204835793 ) ) ;
#29204=CARTESIAN_POINT ( 'NONE',  ( -10.00000000000102496, 5.773502691895664007, -43.75000000409673362 ) ) ;
#29206=CARTESIAN_POINT ( 'NONE',  ( 9.999999999999998224, 0.000000000000000000, -16.99999999999996092 ) ) ;
#29207=EDGE_CURVE ( 'NONE', #3061, #24037, #30943, .T. ) ;
#29208=CARTESIAN_POINT ( 'NONE',  ( 10.81189881249999729, 0.000000000000000000, -70.34375000204836681 ) ) ;
#29209=CARTESIAN_POINT ( 'NONE',  ( 10.81189881249999907, 6.242252689847868297, -53.90625000204838102 ) ) ;
#29211=CARTESIAN_POINT ( 'NONE',  ( -9.999999999999998224, 1.224646799147353059E-15, -56.74999999999996447 ) ) ;
#29213=CARTESIAN_POINT ( 'NONE',  ( 5.000000000000000000, 8.660254037844385522, -138.2499999999999716 ) ) ;
#29214=CARTESIAN_POINT ( 'NONE',  ( -2.293366432827344421E-15, -12.48450537969573659, -147.4062500020483810 ) ) ;
#29215=CARTESIAN_POINT ( 'NONE',  ( 9.999999999999998224, 0.000000000000000000, -16.99999999999996092 ) ) ;
#29216=CARTESIAN_POINT ( 'NONE',  ( -5.000000000000003553, -8.660254037844383745, -113.8750000040967763 ) ) ;
#29221=CYLINDRICAL_SURFACE ( 'NONE', #9124, 9.999999999999998224 ) ;
#29222=CARTESIAN_POINT ( 'NONE',  ( 5.405949406249992428, -9.363379034771808662, -175.7812500020484094 ) ) ;
#29223=CARTESIAN_POINT ( 'NONE',  ( -5.000000000000003553, -8.660254037844383745, -47.87500000409677625 ) ) ;
#29224=DIRECTION ( 'NONE',  ( 1.000000000000000000, 0.000000000000000000, 0.000000000000000000 ) ) ;
#29226=ADVANCED_FACE ( 'NONE', ( #23036 ), #29296, .T. ) ;
#29228=CARTESIAN_POINT ( 'NONE',  ( -10.81189881249999729, 1.324075727343319199E-15, -158.2812500020484094 ) ) ;
#29229=CARTESIAN_POINT ( 'NONE',  ( -2.293366432827344421E-15, -12.48450537969573659, -144.2187500020483810 ) ) ;
#29230=DIRECTION ( 'NONE',  ( -0.000000000000000000, -0.000000000000000000, 1.000000000000000000 ) ) ;
#29231=ORIENTED_EDGE ( 'NONE', *, *, #16931, .F. ) ;
#29232=CYLINDRICAL_SURFACE ( 'NONE', #34172, 9.999999999999998224 ) ;
#29233=CARTESIAN_POINT ( 'NONE',  ( 7.644554776091147741E-16, 12.48450537969573659, -68.65625000204840944 ) ) ;
#29236=CARTESIAN_POINT ( 'NONE',  ( -5.405949406249996869, 9.363379034771805109, -116.3437500020483810 ) ) ;
#29237=VERTEX_POINT ( 'NONE', #23463 ) ;
#29238=ORIENTED_EDGE ( 'NONE', *, *, #27350, .T. ) ;
#29239=CARTESIAN_POINT ( 'NONE',  ( 10.81189881249999729, 6.242252689847867408, -32.71875000204834549 ) ) ;
#29240=CARTESIAN_POINT ( 'NONE',  ( -5.405949406249996869, 9.363379034771805109, -194.3437500020484094 ) ) ;
#29241=CARTESIAN_POINT ( 'NONE',  ( -10.81189881249999907, -6.242252689847864744, -51.46875000204837391 ) ) ;
#29244=CARTESIAN_POINT ( 'NONE',  ( 10.81189881249999729, 0.000000000000000000, -190.3437500020484094 ) ) ;
#29245=CARTESIAN_POINT ( 'NONE',  ( 5.405949406249992428, -9.363379034771808662, -171.0937500020484094 ) ) ;
#29249=CARTESIAN_POINT ( 'NONE',  ( 5.000000000000000000, 8.660254037844385522, -124.7500000000000000 ) ) ;
#29250=CARTESIAN_POINT ( 'NONE',  ( 5.000000000000000000, 8.660254037844385522, -20.12500000409675494 ) ) ;
#29252=CARTESIAN_POINT ( 'NONE',  ( -2.293366432827344421E-15, -12.48450537969573659, -94.71875000204838102 ) ) ;
#29254=CARTESIAN_POINT ( 'NONE',  ( -10.81189881249999729, 6.242252689847871849, -72.90625000204838102 ) ) ;
#29255=CARTESIAN_POINT ( 'NONE',  ( -9.999999999999998224, 1.224646799147353059E-15, -88.62500000409677625 ) ) ;
#29257=CARTESIAN_POINT ( 'NONE',  ( 5.405949406249999534, 9.363379034771803333, -88.09375000204836681 ) ) ;
#29258=( BOUNDED_CURVE ( )  B_SPLINE_CURVE ( 2, ( #26072, #16749, #42661, #39851, #29951, #33405, #9660 ),
 .UNSPECIFIED., .F., .F. ) 
 B_SPLINE_CURVE_WITH_KNOTS ( ( 3, 2, 2, 3 ),
 ( 0.4738805970149255198, 0.4751243781094529051, 0.4763681592039803459, 0.4776119402985076756 ),
 .UNSPECIFIED. ) 
 CURVE ( )  GEOMETRIC_REPRESENTATION_ITEM ( )  RATIONAL_B_SPLINE_CURVE ( ( 0.9999999999999820144, 0.8660254037844566932, 1.000000000000000000, 0.8660254037844387076, 1.000000000000000000, 0.8660254037844148378, 1.000000000000023981 ) ) 
 REPRESENTATION_ITEM ( '' )  );
#29260=CARTESIAN_POINT ( 'NONE',  ( 7.070501591499377789E-16, 11.54700538379251284, -147.5000000040968189 ) ) ;
#29262=ORIENTED_EDGE ( 'NONE', *, *, #27056, .F. ) ;
#29265=FACE_OUTER_BOUND ( 'NONE', #41904, .T. ) ;
#29268=ORIENTED_EDGE ( 'NONE', *, *, #17169, .T. ) ;
#29269=CARTESIAN_POINT ( 'NONE',  ( 4.999999999999992006, -8.660254037844389075, -59.24999999999997158 ) ) ;
#29271=CARTESIAN_POINT ( 'NONE',  ( -10.00000000000000000, -5.773502691896251982, -73.50000000409674783 ) ) ;
#29272=EDGE_CURVE ( 'NONE', #40567, #14344, #39216, .T. ) ;
#29274=DIRECTION ( 'NONE',  ( -0.000000000000000000, -0.000000000000000000, 1.000000000000000000 ) ) ;
#29276=CARTESIAN_POINT ( 'NONE',  ( 10.81189881249999729, 6.242252689847867408, -70.40625000204839523 ) ) ;
#29279=CARTESIAN_POINT ( 'NONE',  ( -9.999999999999998224, 1.224646799147353059E-15, -16.24999999999995737 ) ) ;
#29280=CARTESIAN_POINT ( 'NONE',  ( 7.644554776091147741E-16, 12.48450537969573659, -184.1562500020484094 ) ) ;
#29282=CARTESIAN_POINT ( 'NONE',  ( -4.999999999999996447, 8.660254037844387298, -79.49999999999998579 ) ) ;
#29283=CARTESIAN_POINT ( 'NONE',  ( 5.000000000000000000, 8.660254037844385522, -186.6250000040967905 ) ) ;
#29284=CARTESIAN_POINT ( 'NONE',  ( -4.999999999999996447, 8.660254037844387298, -159.3750000040967905 ) ) ;
#29285=CARTESIAN_POINT ( 'NONE',  ( 4.999999999999992006, -8.660254037844389075, -177.7500000000000284 ) ) ;
#29286=CARTESIAN_POINT ( 'NONE',  ( 9.999999999999998224, 0.000000000000000000, -36.49999999999997868 ) ) ;
#29287=CARTESIAN_POINT ( 'NONE',  ( -5.405949406249996869, 9.363379034771805109, -95.53125000204838102 ) ) ;
#29288=VERTEX_POINT ( 'NONE', #36610 ) ;
#29289=ORIENTED_EDGE ( 'NONE', *, *, #22023, .F. ) ;
#29291=CARTESIAN_POINT ( 'NONE',  ( 10.81189881249999551, -6.242252689847874514, -37.46875000204836681 ) ) ;
#29292=CIRCLE ( 'NONE', #32748, 10.00000000000000178 ) ;
#29293=CARTESIAN_POINT ( 'NONE',  ( -5.405949406249996869, 9.363379034771805109, -29.53125000204837036 ) ) ;
#29295=CARTESIAN_POINT ( 'NONE',  ( -10.81189881249999729, 1.324075727343319199E-15, -80.09375000204838102 ) ) ;
#29296=PLANE ( 'NONE',  #8449 ) ;
#29297=CARTESIAN_POINT ( 'NONE',  ( -5.405949406249996869, 9.363379034771805109, -189.8437500020483810 ) ) ;
#29298=( BOUNDED_CURVE ( )  B_SPLINE_CURVE ( 2, ( #9214, #28234, #22384, #5777, #8799, #1906, #15036 ),
 .UNSPECIFIED., .F., .F. ) 
 B_SPLINE_CURVE_WITH_KNOTS ( ( 3, 2, 2, 3 ),
 ( 0.4514925373134329734, 0.4527363184079603031, 0.4539800995024877439, 0.4552238805970150737 ),
 .UNSPECIFIED. ) 
 CURVE ( )  GEOMETRIC_REPRESENTATION_ITEM ( )  RATIONAL_B_SPLINE_CURVE ( ( 0.9999999999999880096, 0.8660254037844506980, 1.000000000000000000, 0.8660254037844387076, 1.000000000000000000, 0.8660254037844207220, 1.000000000000017986 ) ) 
 REPRESENTATION_ITEM ( '' )  );
#29299=CARTESIAN_POINT ( 'NONE',  ( 9.999999999999998224, 0.000000000000000000, -167.0000000000000000 ) ) ;
#29303=CARTESIAN_POINT ( 'NONE',  ( 7.070501591499377789E-16, 11.54700538379251284, -8.000000004096747830 ) ) ;
#29304=FACE_OUTER_BOUND ( 'NONE', #21674, .T. ) ;
#29305=CARTESIAN_POINT ( 'NONE',  ( 10.81189881249999907, 6.242252689847868297, -131.7187500020483810 ) ) ;
#29306=CARTESIAN_POINT ( 'NONE',  ( 5.405949406249992428, -9.363379034771808662, -102.2812500020483952 ) ) ;
#29307=CARTESIAN_POINT ( 'NONE',  ( -10.81189881249999729, 6.242252689847871849, -105.7187500020483668 ) ) ;
#29311=CARTESIAN_POINT ( 'NONE',  ( 10.00000000000000000, 5.773502691896255534, -173.2500000040967905 ) ) ;
#29312=( BOUNDED_CURVE ( )  B_SPLINE_CURVE ( 2, ( #15665, #18923, #32107, #28866, #38781, #9207, #35554 ),
 .UNSPECIFIED., .F., .F. ) 
 B_SPLINE_CURVE_WITH_KNOTS ( ( 3, 2, 2, 3 ),
 ( 0.5223880597014926019, 0.5236318407960199872, 0.5248756218905473725, 0.5261194029850747578 ),
 .UNSPECIFIED. ) 
 CURVE ( )  GEOMETRIC_REPRESENTATION_ITEM ( )  RATIONAL_B_SPLINE_CURVE ( ( 0.9999999999999880096, 0.8660254037844506980, 1.000000000000000000, 0.8660254037844387076, 1.000000000000000000, 0.8660254037844267172, 1.000000000000011990 ) ) 
 REPRESENTATION_ITEM ( '' )  );
#29313=DIRECTION ( 'NONE',  ( -0.000000000000000000, -0.000000000000000000, 1.000000000000000000 ) ) ;
#29319=CARTESIAN_POINT ( 'NONE',  ( -10.00000000000076916, 5.773502691895813221, -127.3749999999999858 ) ) ;
#29321=CARTESIAN_POINT ( 'NONE',  ( 10.00000000000000000, 5.773502691896255534, -82.87499999999997158 ) ) ;
#29323=CARTESIAN_POINT ( 'NONE',  ( 9.999999999999998224, 0.000000000000000000, -98.37500000409677625 ) ) ;
#29324=CARTESIAN_POINT ( 'NONE',  ( 0.000000000000000000, 0.000000000000000000, -200.0000000000000000 ) ) ;
#29326=CARTESIAN_POINT ( 'NONE',  ( 10.81189881249999551, -6.242252689847874514, -94.65625000204838102 ) ) ;
#29328=VECTOR ( 'NONE', #35176, 1000.000000000000000 ) ;
#29332=ORIENTED_EDGE ( 'NONE', *, *, #37811, .T. ) ;
#29333=CARTESIAN_POINT ( 'NONE',  ( 5.000000000000000000, 8.660254037844385522, -15.24999999999995737 ) ) ;
#29334=ADVANCED_FACE ( 'NONE', ( #42443 ), #19566, .T. ) ;
#29335=CARTESIAN_POINT ( 'NONE',  ( 9.999999999999996447, -5.773502691896262640, -152.1250000000000284 ) ) ;
#29337=EDGE_CURVE ( 'NONE', #35521, #21267, #19084, .T. ) ;
#29338=CARTESIAN_POINT ( 'NONE',  ( -5.000000000000003553, -8.660254037844383745, -199.0000000000000000 ) ) ;
#29339=CARTESIAN_POINT ( 'NONE',  ( 10.81189881249999729, 0.000000000000000000, -124.5312500020483952 ) ) ;
#29341=VECTOR ( 'NONE', #35260, 1000.000000000000000 ) ;
#29342=VERTEX_POINT ( 'NONE', #39629 ) ;
#29344=CARTESIAN_POINT ( 'NONE',  ( 5.405949406249999534, 9.363379034771803333, -56.78125000204836681 ) ) ;
#29346=CARTESIAN_POINT ( 'NONE',  ( 7.644554776091147741E-16, 12.48450537969573659, -99.96875000204839523 ) ) ;
#29347=ORIENTED_EDGE ( 'NONE', *, *, #252, .F. ) ;
#29348=VERTEX_POINT ( 'NONE', #20417 ) ;
#29350=DIRECTION ( 'NONE',  ( 1.000000000000000000, 0.000000000000000000, 0.000000000000000000 ) ) ;
#29351=CARTESIAN_POINT ( 'NONE',  ( -10.00000000000051337, 5.773502691895962435, -32.87499999999995026 ) ) ;
#29353=CARTESIAN_POINT ( 'NONE',  ( -10.81189881249999729, 6.242252689847871849, -0.7187500020483512664 ) ) ;
#29355=CARTESIAN_POINT ( 'NONE',  ( -10.81189881249999729, -6.242252689847864744, -135.4687500020483810 ) ) ;
#29357=CARTESIAN_POINT ( 'NONE',  ( 0.000000000000000000, 0.000000000000000000, 0.000000000000000000 ) ) ;
#29359=CARTESIAN_POINT ( 'NONE',  ( 4.999999999999992006, -8.660254037844389075, -197.6250000040967905 ) ) ;
#29361=CARTESIAN_POINT ( 'NONE',  ( -10.81189881249999729, -6.242252689847864744, -186.6562500020484094 ) ) ;
#29362=CARTESIAN_POINT ( 'NONE',  ( 9.999999999999998224, 0.000000000000000000, -200.0000000000000000 ) ) ;
#29365=CARTESIAN_POINT ( 'NONE',  ( -2.293366432827344421E-15, -12.48450537969573659, -57.21875000204835970 ) ) ;
#29366=CARTESIAN_POINT ( 'NONE',  ( 10.81189881249999729, 0.000000000000000000, -49.34375000204838102 ) ) ;
#29368=CARTESIAN_POINT ( 'NONE',  ( -5.405949406250003975, -9.363379034771801557, -17.03125000204835970 ) ) ;
#29370=CARTESIAN_POINT ( 'NONE',  ( -2.121150477449813534E-15, -11.54700538379251284, -8.374999999999976907 ) ) ;
#29372=CARTESIAN_POINT ( 'NONE',  ( -10.00000000000000000, -5.773502691896251982, -112.1249999999999858 ) ) ;
#29373=DIRECTION ( 'NONE',  ( 1.000000000000000000, 0.000000000000000000, 0.000000000000000000 ) ) ;
#29374=AXIS2_PLACEMENT_3D ( 'NONE', #6004, #11820, #1923 ) ;
#29377=CARTESIAN_POINT ( 'NONE',  ( 10.81189881249999551, -6.242252689847874514, -112.6562500020483952 ) ) ;
#29378=EDGE_LOOP ( 'NONE', ( #23498, #39000, #32332, #640 ) ) ;
#29379=DIRECTION ( 'NONE',  ( 1.000000000000000000, 0.000000000000000000, 0.000000000000000000 ) ) ;
#29381=CARTESIAN_POINT ( 'NONE',  ( 9.999999999999998224, 0.000000000000000000, -128.0000000000000000 ) ) ;
#29384=CARTESIAN_POINT ( 'NONE',  ( 9.999999999999998224, 0.000000000000000000, -45.49999999999998579 ) ) ;
#29385=CARTESIAN_POINT ( 'NONE',  ( 9.999999999999998224, 0.000000000000000000, -18.87500000409675494 ) ) ;
#29387=CARTESIAN_POINT ( 'NONE',  ( -10.81189881249999729, 6.242252689847871849, -44.40625000204835970 ) ) ;
#29388=( BOUNDED_CURVE ( )  B_SPLINE_CURVE ( 2, ( #27358, #10303, #14159, #10939, #27574, #40285, #4267 ),
 .UNSPECIFIED., .F., .F. ) 
 B_SPLINE_CURVE_WITH_KNOTS ( ( 3, 2, 2, 3 ),
 ( 0.1380597014925373234, 0.1393034825870646809, 0.1405472636815920384, 0.1417910447761193959 ),
 .UNSPECIFIED. ) 
 CURVE ( )  GEOMETRIC_REPRESENTATION_ITEM ( )  RATIONAL_B_SPLINE_CURVE ( ( 1.000000000000000000, 0.8660254037844387076, 1.000000000000000000, 0.8660254037844387076, 1.000000000000000000, 0.8660254037844387076, 1.000000000000000000 ) ) 
 REPRESENTATION_ITEM ( '' )  );
#29392=EDGE_CURVE ( 'NONE', #31963, #38940, #384, .T. ) ;
#29393=CARTESIAN_POINT ( 'NONE',  ( 0.000000000000000000, 0.000000000000000000, -200.0000000000000000 ) ) ;
#29394=CARTESIAN_POINT ( 'NONE',  ( -5.405949406250003975, -9.363379034771801557, -137.0312500020484094 ) ) ;
#29396=CARTESIAN_POINT ( 'NONE',  ( 10.81189881249999907, 6.242252689847868297, -146.9062500020484094 ) ) ;
#29398=CARTESIAN_POINT ( 'NONE',  ( 4.999999999999992006, -8.660254037844389075, -123.7500000000000000 ) ) ;
#29399=ORIENTED_EDGE ( 'NONE', *, *, #29039, .F. ) ;
#29400=ORIENTED_EDGE ( 'NONE', *, *, #37817, .T. ) ;
#29401=ORIENTED_EDGE ( 'NONE', *, *, #26995, .T. ) ;
#29403=CARTESIAN_POINT ( 'NONE',  ( -10.81189881249999729, 1.324075727343319199E-15, -176.0937500020484094 ) ) ;
#29405=EDGE_CURVE ( 'NONE', #4750, #37499, #32089, .T. ) ;
#29406=CARTESIAN_POINT ( 'NONE',  ( 7.644554776091147741E-16, 12.48450537969573659, -24.96875000204837036 ) ) ;
#29407=CYLINDRICAL_SURFACE ( 'NONE', #33650, 9.999999999999998224 ) ;
#29408=CARTESIAN_POINT ( 'NONE',  ( 7.644554776091147741E-16, 12.48450537969573659, -153.9687500020484094 ) ) ;
#29409=CARTESIAN_POINT ( 'NONE',  ( -5.405949406250003975, -9.363379034771801557, -142.8437500020483810 ) ) ;
#29413=CARTESIAN_POINT ( 'NONE',  ( 10.81189881249999729, 0.000000000000000000, -22.34375000204835615 ) ) ;
#29416=CARTESIAN_POINT ( 'NONE',  ( -10.00000000000051337, 5.773502691895962435, -119.8749999999999858 ) ) ;
#29418=CARTESIAN_POINT ( 'NONE',  ( 9.999999999999998224, 0.000000000000000000, -56.37500000409676204 ) ) ;
#29419=CARTESIAN_POINT ( 'NONE',  ( -5.405949406249996869, 9.363379034771805109, -69.84375000204836681 ) ) ;
#29420=CARTESIAN_POINT ( 'NONE',  ( -2.293366432827344421E-15, -12.48450537969573659, -54.40625000204838102 ) ) ;
#29422=CARTESIAN_POINT ( 'NONE',  ( 9.999999999999998224, 0.000000000000000000, -200.0000000000000000 ) ) ;
#29424=CARTESIAN_POINT ( 'NONE',  ( -4.999999999999996447, 8.660254037844387298, -139.5000000000000000 ) ) ;
#29425=CARTESIAN_POINT ( 'NONE',  ( -5.405949406249996869, 9.363379034771805109, -137.5312500020484094 ) ) ;
#29427=CARTESIAN_POINT ( 'NONE',  ( 9.999999999999998224, 0.000000000000000000, -116.3750000040967905 ) ) ;
#29429=( BOUNDED_CURVE ( )  B_SPLINE_CURVE ( 2, ( #12130, #32435, #11700, #41481, #38045, #25321, #24896 ),
 .UNSPECIFIED., .F., .F. ) 
 B_SPLINE_CURVE_WITH_KNOTS ( ( 3, 2, 2, 3 ),
 ( 0.7388059701492539766, 0.7400497512437813619, 0.7412935323383087471, 0.7425373134328361324 ),
 .UNSPECIFIED. ) 
 CURVE ( )  GEOMETRIC_REPRESENTATION_ITEM ( )  RATIONAL_B_SPLINE_CURVE ( ( 0.9999999999999761302, 0.8660254037844625774, 1.000000000000000000, 0.8660254037844387076, 1.000000000000000000, 0.8660254037844028474, 1.000000000000035971 ) ) 
 REPRESENTATION_ITEM ( '' )  );
#29430=ORIENTED_EDGE ( 'NONE', *, *, #1153, .T. ) ;
#29434=CARTESIAN_POINT ( 'NONE',  ( 7.644554776091147741E-16, 12.48450537969573659, -173.6562500020483810 ) ) ;
#29435=CARTESIAN_POINT ( 'NONE',  ( 10.00000000000000000, 5.773502691896255534, -44.25000000409676204 ) ) ;
#29437=CARTESIAN_POINT ( 'NONE',  ( 0.000000000000000000, 0.000000000000000000, -200.0000000000000000 ) ) ;
#29439=CARTESIAN_POINT ( 'NONE',  ( -4.999999999999996447, 8.660254037844387298, -156.0000000000000000 ) ) ;
#29440=CARTESIAN_POINT ( 'NONE',  ( 10.81189881249999907, 6.242252689847868297, -161.9062500020484094 ) ) ;
#29441=CARTESIAN_POINT ( 'NONE',  ( -10.81189881249999729, 6.242252689847871849, -144.7187500020483810 ) ) ;
#29445=CARTESIAN_POINT ( 'NONE',  ( -4.999999999999996447, 8.660254037844387298, -114.3750000040967763 ) ) ;
#29446=EDGE_CURVE ( 'NONE', #23818, #18552, #39002, .T. ) ;
#29447=CARTESIAN_POINT ( 'NONE',  ( 10.81189881249999907, 6.242252689847868297, -70.40625000204839523 ) ) ;
#29448=ORIENTED_EDGE ( 'NONE', *, *, #17109, .T. ) ;
#29450=CARTESIAN_POINT ( 'NONE',  ( 5.405949406249999534, 9.363379034771803333, -119.5937500020483810 ) ) ;
#29451=ORIENTED_EDGE ( 'NONE', *, *, #14281, .T. ) ;
#29452=ORIENTED_EDGE ( 'NONE', *, *, #35558, .T. ) ;
#29453=CARTESIAN_POINT ( 'NONE',  ( -5.405949406250003975, -9.363379034771801557, -18.34375000204835260 ) ) ;
#29454=CARTESIAN_POINT ( 'NONE',  ( -10.81189881249999729, 1.324075727343319199E-15, -0.7812500020483725827 ) ) ;
#29455=CARTESIAN_POINT ( 'NONE',  ( -10.81189881249999907, -6.242252689847864744, -48.46875000204837391 ) ) ;
#29458=CARTESIAN_POINT ( 'NONE',  ( -10.81189881249999729, 1.324075727343319199E-15, -185.0937500020483810 ) ) ;
#29459=CARTESIAN_POINT ( 'NONE',  ( -10.81189881249999729, 1.324075727343319199E-15, -165.5937500020484094 ) ) ;
#29462=CARTESIAN_POINT ( 'NONE',  ( 0.000000000000000000, 0.000000000000000000, -200.0000000000000000 ) ) ;
#29465=CARTESIAN_POINT ( 'NONE',  ( 10.81189881249999907, 6.242252689847868297, -95.71875000204838102 ) ) ;
#29466=CARTESIAN_POINT ( 'NONE',  ( 5.000000000000000000, 8.660254037844385522, -196.7500000000000000 ) ) ;
#29467=CARTESIAN_POINT ( 'NONE',  ( -10.81189881249999907, -6.242252689847864744, -77.15625000204836681 ) ) ;
#29468=CARTESIAN_POINT ( 'NONE',  ( 9.999999999999479527, 5.773502691896553074, -89.25000000409674783 ) ) ;
#29470=CARTESIAN_POINT ( 'NONE',  ( -10.81189881249999729, 1.324075727343319199E-15, -162.7812500020484094 ) ) ;
#29472=CARTESIAN_POINT ( 'NONE',  ( 9.999999999999996447, -5.773502691896262640, -140.5000000040967905 ) ) ;
#29474=VERTEX_POINT ( 'NONE', #17811 ) ;
#29477=CARTESIAN_POINT ( 'NONE',  ( 5.405949406249999534, 9.363379034771803333, -197.7812500020484094 ) ) ;
#29478=CARTESIAN_POINT ( 'NONE',  ( -9.999999999999998224, 1.224646799147353059E-15, -130.6250000040967620 ) ) ;
#29481=EDGE_LOOP ( 'NONE', ( #12015, #28080, #7685, #38614 ) ) ;
#29482=CARTESIAN_POINT ( 'NONE',  ( -4.999999999999996447, 8.660254037844387298, -53.99999999999996447 ) ) ;
#29484=CARTESIAN_POINT ( 'NONE',  ( 9.999999999999996447, -5.773502691896262640, -68.50000000409677625 ) ) ;
#29487=CARTESIAN_POINT ( 'NONE',  ( 7.071067811865472841, -7.071067811865472841, -200.0000000000000000 ) ) ;
#29489=CARTESIAN_POINT ( 'NONE',  ( -2.293366432827344421E-15, -12.48450537969573659, -69.40625000204839523 ) ) ;
#29492=DIRECTION ( 'NONE',  ( -0.000000000000000000, -0.000000000000000000, 1.000000000000000000 ) ) ;
#29493=CARTESIAN_POINT ( 'NONE',  ( 10.81189881249999907, 6.242252689847868297, -188.9062500020484379 ) ) ;
#29498=CARTESIAN_POINT ( 'NONE',  ( -4.999999999999996447, 8.660254037844387298, -168.0000000000000000 ) ) ;
#29499=CARTESIAN_POINT ( 'NONE',  ( 0.000000000000000000, 0.000000000000000000, -200.0000000000000000 ) ) ;
#29500=CARTESIAN_POINT ( 'NONE',  ( -10.81189881249999729, 6.242252689847871849, -95.40625000204838102 ) ) ;
#29501=ORIENTED_EDGE ( 'NONE', *, *, #6508, .F. ) ;
#29502=CARTESIAN_POINT ( 'NONE',  ( -2.121150477449813534E-15, -11.54700538379251284, -181.2500000040967905 ) ) ;
#29504=ORIENTED_EDGE ( 'NONE', *, *, #4339, .T. ) ;
#29506=CARTESIAN_POINT ( 'NONE',  ( 5.405949406249999534, 9.363379034771803333, -34.09375000204836681 ) ) ;
#29507=CARTESIAN_POINT ( 'NONE',  ( 5.405949406249999534, 9.363379034771803333, -25.28125000204836681 ) ) ;
#29509=CARTESIAN_POINT ( 'NONE',  ( -10.81189881249999729, 6.242252689847871849, -71.21875000204839523 ) ) ;
#29513=CARTESIAN_POINT ( 'NONE',  ( 5.405949406249992428, -9.363379034771808662, -193.5937500020484094 ) ) ;
#29514=( BOUNDED_CURVE ( )  B_SPLINE_CURVE ( 2, ( #22729, #35894, #16218, #26389, #9971, #23151, #36312 ),
 .UNSPECIFIED., .F., .F. ) 
 B_SPLINE_CURVE_WITH_KNOTS ( ( 3, 2, 2, 3 ),
 ( 0.1529850746268656692, 0.1542288557213930267, 0.1554726368159203842, 0.1567164179104477695 ),
 .UNSPECIFIED. ) 
 CURVE ( )  GEOMETRIC_REPRESENTATION_ITEM ( )  RATIONAL_B_SPLINE_CURVE ( ( 1.000000000000000000, 0.8660254037844387076, 1.000000000000000000, 0.8660254037844387076, 1.000000000000000000, 0.8660254037844387076, 1.000000000000000000 ) ) 
 REPRESENTATION_ITEM ( '' )  );
#29516=CARTESIAN_POINT ( 'NONE',  ( -9.999999999999998224, 1.224646799147353059E-15, -100.6250000040967905 ) ) ;
#29518=CARTESIAN_POINT ( 'NONE',  ( -10.00000000000000000, -5.773502691896251982, -4.500000004096765593 ) ) ;
#29520=CARTESIAN_POINT ( 'NONE',  ( -10.81189881249999907, -6.242252689847864744, -124.9687500020483810 ) ) ;
#29521=CARTESIAN_POINT ( 'NONE',  ( 5.405949406249999534, 9.363379034771803333, -97.28125000204839523 ) ) ;
#29522=CARTESIAN_POINT ( 'NONE',  ( -10.81189881249999729, 6.242252689847871849, -111.7187500020483810 ) ) ;
#29525=CARTESIAN_POINT ( 'NONE',  ( -10.00000000000000000, -5.773502691896251982, -162.0000000040967620 ) ) ;
#29526=CARTESIAN_POINT ( 'NONE',  ( -9.999999999999998224, 1.224646799147353059E-15, -200.0000000000000000 ) ) ;
#29530=CARTESIAN_POINT ( 'NONE',  ( -9.999999999999998224, 1.224646799147353059E-15, -157.2500000000000000 ) ) ;
#29532=CARTESIAN_POINT ( 'NONE',  ( -4.999999999999996447, 8.660254037844387298, -127.5000000000000000 ) ) ;
#29534=CARTESIAN_POINT ( 'NONE',  ( -2.121150477449813534E-15, -11.54700538379251284, -84.87500000000000000 ) ) ;
#29536=CARTESIAN_POINT ( 'NONE',  ( -2.121150477449813534E-15, -11.54700538379251284, -100.2500000040967905 ) ) ;
#29537=CARTESIAN_POINT ( 'NONE',  ( 7.070501591499376803E-16, 11.54700538379251284, -150.5000000040968189 ) ) ;
#29539=CARTESIAN_POINT ( 'NONE',  ( 7.644554776091147741E-16, 12.48450537969573659, -88.15625000204838102 ) ) ;
#29540=ORIENTED_EDGE ( 'NONE', *, *, #12511, .T. ) ;
#29542=CARTESIAN_POINT ( 'NONE',  ( -9.999999999999998224, 1.224646799147353059E-15, -47.74999999999998579 ) ) ;
#29544=ORIENTED_EDGE ( 'NONE', *, *, #37625, .T. ) ;
#29545=CARTESIAN_POINT ( 'NONE',  ( 9.999999999999996447, -5.773502691896262640, -8.124999999999975131 ) ) ;
#29546=CARTESIAN_POINT ( 'NONE',  ( -5.000000000000003553, -8.660254037844383745, -149.5000000000000000 ) ) ;
#29549=CARTESIAN_POINT ( 'NONE',  ( 7.070501591499377789E-16, 11.54700538379251284, -187.6250000000000284 ) ) ;
#29550=CARTESIAN_POINT ( 'NONE',  ( 10.81189881249999551, -6.242252689847874514, -114.1562500020483952 ) ) ;
#29552=CARTESIAN_POINT ( 'NONE',  ( 7.070501591499376803E-16, 11.54700538379251284, -13.62499999999996803 ) ) ;
#29553=ORIENTED_EDGE ( 'NONE', *, *, #34899, .T. ) ;
#29554=( BOUNDED_CURVE ( )  B_SPLINE_CURVE ( 2, ( #10683, #1210, #997, #37453, #40247, #13696, #8108 ),
 .UNSPECIFIED., .F., .F. ) 
 B_SPLINE_CURVE_WITH_KNOTS ( ( 3, 2, 2, 3 ),
 ( 0.2238805970149254365, 0.2251243781094527940, 0.2263681592039801793, 0.2276119402985075368 ),
 .UNSPECIFIED. ) 
 CURVE ( )  GEOMETRIC_REPRESENTATION_ITEM ( )  RATIONAL_B_SPLINE_CURVE ( ( 0.9999999999999940048, 0.8660254037844447028, 1.000000000000000000, 0.8660254037844387076, 1.000000000000000000, 0.8660254037844297148, 1.000000000000008882 ) ) 
 REPRESENTATION_ITEM ( '' )  );
#29555=CARTESIAN_POINT ( 'NONE',  ( -2.293366432827344421E-15, -12.48450537969573659, -46.90625000204836681 ) ) ;
#29557=CARTESIAN_POINT ( 'NONE',  ( 10.81189881249999729, 0.000000000000000000, -103.3437500020483668 ) ) ;
#29558=CARTESIAN_POINT ( 'NONE',  ( -10.81189881249999729, -6.242252689847864744, -122.1562500020483810 ) ) ;
#29559=ORIENTED_EDGE ( 'NONE', *, *, #37458, .F. ) ;
#29560=CARTESIAN_POINT ( 'NONE',  ( 10.00000000000102318, -5.773502691895667560, -83.12499999999992895 ) ) ;
#29561=DIRECTION ( 'NONE',  ( 1.000000000000000000, 0.000000000000000000, 0.000000000000000000 ) ) ;
#29562=( BOUNDED_CURVE ( )  B_SPLINE_CURVE ( 2, ( #27578, #24138, #30610, #28010, #14604, #1684, #8375 ),
 .UNSPECIFIED., .F., .F. ) 
 B_SPLINE_CURVE_WITH_KNOTS ( ( 3, 2, 2, 3 ),
 ( 0.4253731343283583266, 0.4266169154228856564, 0.4278606965174130417, 0.4291044776119404269 ),
 .UNSPECIFIED. ) 
 CURVE ( )  GEOMETRIC_REPRESENTATION_ITEM ( )  RATIONAL_B_SPLINE_CURVE ( ( 0.9999999999999880096, 0.8660254037844506980, 1.000000000000000000, 0.8660254037844387076, 1.000000000000000000, 0.8660254037844267172, 1.000000000000011990 ) ) 
 REPRESENTATION_ITEM ( '' )  );
#29564=CARTESIAN_POINT ( 'NONE',  ( 0.000000000000000000, 0.000000000000000000, -200.0000000000000000 ) ) ;
#29566=CARTESIAN_POINT ( 'NONE',  ( -10.81189881249999729, -6.242252689847864744, -130.9687500020483810 ) ) ;
#29571=CARTESIAN_POINT ( 'NONE',  ( 9.999999999999998224, 0.000000000000000000, -191.3750000040967905 ) ) ;
#29573=CARTESIAN_POINT ( 'NONE',  ( -2.293366432827344421E-15, -12.48450537969573659, -183.4062500020484094 ) ) ;
#29574=CARTESIAN_POINT ( 'NONE',  ( 10.00000000000102318, -5.773502691895667560, -47.12499999999992895 ) ) ;
#29575=LINE ( 'NONE', #25555, #13438 ) ;
#29578=CARTESIAN_POINT ( 'NONE',  ( -10.81189881249999729, -6.242252689847864744, -58.96875000204836681 ) ) ;
#29580=CARTESIAN_POINT ( 'NONE',  ( -10.81189881249999729, 1.324075727343319199E-15, -51.59375000204835260 ) ) ;
#29583=CARTESIAN_POINT ( 'NONE',  ( -10.81189881249999907, -6.242252689847864744, -15.65625000204837569 ) ) ;
#29587=CARTESIAN_POINT ( 'NONE',  ( -9.999999999999998224, 5.773502691896259087, -103.3750000000000000 ) ) ;
#29592=CARTESIAN_POINT ( 'NONE',  ( 10.81189881249999729, 0.000000000000000000, -115.5312500020483952 ) ) ;
#29594=VECTOR ( 'NONE', #16644, 1000.000000000000000 ) ;
#29599=ORIENTED_EDGE ( 'NONE', *, *, #32291, .T. ) ;
#29600=CARTESIAN_POINT ( 'NONE',  ( -9.999999999999998224, 5.773502691896259087, -31.37499999999995737 ) ) ;
#29601=CARTESIAN_POINT ( 'NONE',  ( 10.00000000000000000, 5.773502691896255534, -21.75000000409676559 ) ) ;
#29602=CARTESIAN_POINT ( 'NONE',  ( -5.405949406250003975, -9.363379034771801557, -47.03125000204838813 ) ) ;
#29605=CARTESIAN_POINT ( 'NONE',  ( -5.405949406249996869, 9.363379034771805109, -140.5312500020484094 ) ) ;
#29606=CARTESIAN_POINT ( 'NONE',  ( -5.405949406250003975, -9.363379034771801557, -143.0312500020483810 ) ) ;
#29609=VECTOR ( 'NONE', #41096, 1000.000000000000000 ) ;
#29610=ORIENTED_EDGE ( 'NONE', *, *, #33366, .F. ) ;
#29612=CARTESIAN_POINT ( 'NONE',  ( 4.999999999999992006, -8.660254037844389075, -121.1250000040967905 ) ) ;
#29613=CARTESIAN_POINT ( 'NONE',  ( 10.81189881249999729, 0.000000000000000000, -176.8437500020483810 ) ) ;
#29614=VECTOR ( 'NONE', #36421, 1000.000000000000000 ) ;
#29615=CARTESIAN_POINT ( 'NONE',  ( -2.293366432827344421E-15, -12.48450537969573659, -25.71875000204837391 ) ) ;
#29616=CARTESIAN_POINT ( 'NONE',  ( -9.999999999998969713, -5.773502691896847949, -61.50000000409675494 ) ) ;
#29617=EDGE_CURVE ( 'NONE', #25832, #37214, #16917, .T. ) ;
#29618=CARTESIAN_POINT ( 'NONE',  ( 7.644554776091147741E-16, 12.48450537969573659, -159.9687500020484094 ) ) ;
#29619=CARTESIAN_POINT ( 'NONE',  ( 7.644554776091147741E-16, 12.48450537969573659, -146.4687500020484094 ) ) ;
#29620=ADVANCED_FACE ( 'NONE', ( #31007 ), #37899, .T. ) ;
#29623=CARTESIAN_POINT ( 'NONE',  ( 10.81189881249999729, 0.000000000000000000, -17.84375000204835260 ) ) ;
#29625=ADVANCED_FACE ( 'NONE', ( #27331 ), #24532, .T. ) ;
#29626=FACE_OUTER_BOUND ( 'NONE', #32389, .T. ) ;
#29629=CARTESIAN_POINT ( 'NONE',  ( -9.999999999998456346, -5.773502691897145489, -17.62499999999993250 ) ) ;
#29630=CARTESIAN_POINT ( 'NONE',  ( 10.81189881249999907, 6.242252689847868297, -73.21875000204836681 ) ) ;
#29631=CARTESIAN_POINT ( 'NONE',  ( 10.81189881249999729, 0.000000000000000000, -40.53125000204838102 ) ) ;
#29635=CARTESIAN_POINT ( 'NONE',  ( -2.121150477449813534E-15, -11.54700538379251284, -131.3750000000000000 ) ) ;
#29636=CARTESIAN_POINT ( 'NONE',  ( -5.405949406249996869, 9.363379034771805109, -134.5312500020484094 ) ) ;
#29637=( BOUNDED_CURVE ( )  B_SPLINE_CURVE ( 2, ( #3310, #16655, #22737, #42567, #7178, #13415, #294 ),
 .UNSPECIFIED., .F., .F. ) 
 B_SPLINE_CURVE_WITH_KNOTS ( ( 3, 2, 2, 3 ),
 ( 0.2425373134328359381, 0.2437810945273632957, 0.2450248756218906532, 0.2462686567164180107 ),
 .UNSPECIFIED. ) 
 CURVE ( )  GEOMETRIC_REPRESENTATION_ITEM ( )  RATIONAL_B_SPLINE_CURVE ( ( 0.9999999999999880096, 0.8660254037844506980, 1.000000000000000000, 0.8660254037844387076, 1.000000000000000000, 0.8660254037844267172, 1.000000000000011990 ) ) 
 REPRESENTATION_ITEM ( '' )  );
#29639=CARTESIAN_POINT ( 'NONE',  ( -9.999999999999998224, 1.224646799147353059E-15, -114.1250000040967763 ) ) ;
#29645=VECTOR ( 'NONE', #23666, 1000.000000000000000 ) ;
#29646=CARTESIAN_POINT ( 'NONE',  ( 5.405949406249999534, 9.363379034771803333, -172.2812500020484094 ) ) ;
#29647=CARTESIAN_POINT ( 'NONE',  ( 10.00000000000000000, 5.773502691896255534, -38.25000000409676204 ) ) ;
#29649=FACE_OUTER_BOUND ( 'NONE', #10846, .T. ) ;
#29651=CARTESIAN_POINT ( 'NONE',  ( 5.000000000000000000, 8.660254037844385522, -101.1250000040967905 ) ) ;
#29652=CARTESIAN_POINT ( 'NONE',  ( 10.81189881249999729, 0.000000000000000000, -160.5312500020484094 ) ) ;
#29653=EDGE_CURVE ( 'NONE', #13705, #20043, #36485, .T. ) ;
#29654=CARTESIAN_POINT ( 'NONE',  ( 10.81189881249999551, -6.242252689847874514, -131.9687500020483810 ) ) ;
#29656=CARTESIAN_POINT ( 'NONE',  ( 7.070501591499376803E-16, 11.54700538379251284, -150.1250000000000000 ) ) ;
#29657=ADVANCED_FACE ( 'NONE', ( #8342 ), #34028, .T. ) ;
#29659=CARTESIAN_POINT ( 'NONE',  ( -9.999999999999479527, -5.773502691896549521, -79.12499999999997158 ) ) ;
#29660=CARTESIAN_POINT ( 'NONE',  ( 5.405949406249999534, 9.363379034771803333, -67.28125000204838102 ) ) ;
#29661=ORIENTED_EDGE ( 'NONE', *, *, #25421, .F. ) ;
#29662=CARTESIAN_POINT ( 'NONE',  ( 10.81189881249999551, -6.242252689847874514, -118.4687500020483810 ) ) ;
#29664=EDGE_CURVE ( 'NONE', #3284, #8850, #6990, .T. ) ;
#29666=VERTEX_POINT ( 'NONE', #42177 ) ;
#29667=CARTESIAN_POINT ( 'NONE',  ( -10.81189881249999729, 1.324075727343319199E-15, -21.59375000204835615 ) ) ;
#29668=CARTESIAN_POINT ( 'NONE',  ( 10.81189881249999907, 6.242252689847868297, 0.09374999795163654892 ) ) ;
#29669=AXIS2_PLACEMENT_3D ( 'NONE', #6669, #20036, #26319 ) ;
#29670=CARTESIAN_POINT ( 'NONE',  ( 10.81189881249999551, -6.242252689847874514, -50.96875000204836681 ) ) ;
#29671=CYLINDRICAL_SURFACE ( 'NONE', #23290, 9.999999999999998224 ) ;
#29673=CARTESIAN_POINT ( 'NONE',  ( -5.405949406250003975, -9.363379034771801557, -183.3437500020483810 ) ) ;
#29674=CARTESIAN_POINT ( 'NONE',  ( -2.293366432827344421E-15, -12.48450537969573659, -166.7187500020484094 ) ) ;
#29676=( BOUNDED_CURVE ( )  B_SPLINE_CURVE ( 2, ( #9247, #26299, #22417, #5596, #2786, #6237, #18749 ),
 .UNSPECIFIED., .F., .F. ) 
 B_SPLINE_CURVE_WITH_KNOTS ( ( 3, 2, 2, 3 ),
 ( 0.9626865671641793298, 0.9639303482587067151, 0.9651741293532341004, 0.9664179104477613746 ),
 .UNSPECIFIED. ) 
 CURVE ( )  GEOMETRIC_REPRESENTATION_ITEM ( )  RATIONAL_B_SPLINE_CURVE ( ( 0.9999999999999761302, 0.8660254037844625774, 1.000000000000000000, 0.8660254037844387076, 1.000000000000000000, 0.8660254037844148378, 1.000000000000023981 ) ) 
 REPRESENTATION_ITEM ( '' )  );
#29678=CARTESIAN_POINT ( 'NONE',  ( 9.999999999999998224, 0.000000000000000000, -5.375000004096769146 ) ) ;
#29679=CARTESIAN_POINT ( 'NONE',  ( 7.070501591499376803E-16, 11.54700538379251284, -20.00000000409677625 ) ) ;
#29681=CARTESIAN_POINT ( 'NONE',  ( -5.405949406250003975, -9.363379034771801557, -93.34375000204838102 ) ) ;
#29683=CARTESIAN_POINT ( 'NONE',  ( -10.81189881249999907, -6.242252689847864744, -69.65625000204839523 ) ) ;
#29684=CARTESIAN_POINT ( 'NONE',  ( -10.00000000000051337, 5.773502691895962435, -88.75000000409676204 ) ) ;
#29686=CARTESIAN_POINT ( 'NONE',  ( -10.81189881249999729, -6.242252689847864744, -162.6562500020483810 ) ) ;
#29688=CARTESIAN_POINT ( 'NONE',  ( 10.00000000000000000, 5.773502691896255534, -137.2500000040967905 ) ) ;
#29693=CARTESIAN_POINT ( 'NONE',  ( -10.81189881249999729, 6.242252689847871849, -195.9062500020484094 ) ) ;
#29694=CARTESIAN_POINT ( 'NONE',  ( 9.999999999999998224, 0.000000000000000000, -42.87500000409677625 ) ) ;
#29696=ORIENTED_EDGE ( 'NONE', *, *, #889, .F. ) ;
#29697=CARTESIAN_POINT ( 'NONE',  ( 9.999999999999996447, -5.773502691896262640, -60.62499999999998579 ) ) ;
#29699=CARTESIAN_POINT ( 'NONE',  ( 5.000000000000000000, 8.660254037844385522, -69.62500000409677625 ) ) ;
#29700=CARTESIAN_POINT ( 'NONE',  ( 9.999999999999998224, 0.000000000000000000, -102.5000000000000000 ) ) ;
#29701=CARTESIAN_POINT ( 'NONE',  ( 10.00000000000051159, -5.773502691895965988, -144.6250000000000000 ) ) ;
#29703=CARTESIAN_POINT ( 'NONE',  ( 7.644554776091147741E-16, 12.48450537969573659, -58.15625000204838102 ) ) ;
#29704=EDGE_CURVE ( 'NONE', #16918, #21964, #11387, .T. ) ;
#29707=FACE_OUTER_BOUND ( 'NONE', #30675, .T. ) ;
#29708=CARTESIAN_POINT ( 'NONE',  ( 5.405949406249992428, -9.363379034771808662, -184.7812500020484094 ) ) ;
#29711=CARTESIAN_POINT ( 'NONE',  ( -10.81189881249999729, -6.242252689847864744, -0.4687500020483501006 ) ) ;
#29714=CARTESIAN_POINT ( 'NONE',  ( -2.121150477449813534E-15, -11.54700538379251284, -62.75000000409679046 ) ) ;
#29716=CARTESIAN_POINT ( 'NONE',  ( -9.999999999999998224, 1.224646799147353059E-15, -169.2500000000000000 ) ) ;
#29717=CARTESIAN_POINT ( 'NONE',  ( 10.00000000000102318, -5.773502691895667560, -62.12499999999992895 ) ) ;
#29718=CARTESIAN_POINT ( 'NONE',  ( 7.644554776091147741E-16, 12.48450537969573659, -95.65625000204838102 ) ) ;
#29719=ORIENTED_EDGE ( 'NONE', *, *, #8536, .T. ) ;
#29720=CARTESIAN_POINT ( 'NONE',  ( -4.999999999999996447, 8.660254037844387298, -82.87500000409676204 ) ) ;
#29721=CARTESIAN_POINT ( 'NONE',  ( 9.999999999999872102, 5.773502691896329253, -162.3750000000000000 ) ) ;
#29722=ORIENTED_EDGE ( 'NONE', *, *, #41868, .F. ) ;
#29723=EDGE_LOOP ( 'NONE', ( #35861, #6177, #19807, #3991 ) ) ;
#29724=CARTESIAN_POINT ( 'NONE',  ( 10.81189881249999907, 6.242252689847868297, -35.71875000204835970 ) ) ;
#29725=CARTESIAN_POINT ( 'NONE',  ( -10.81189881249999907, -6.242252689847864744, -24.65625000204838457 ) ) ;
#29726=CARTESIAN_POINT ( 'NONE',  ( -10.81189881249999729, 6.242252689847871849, -72.71875000204835260 ) ) ;
#29728=CARTESIAN_POINT ( 'NONE',  ( -10.81189881249999729, 1.324075727343319199E-15, -192.5937500020484094 ) ) ;
#29729=CARTESIAN_POINT ( 'NONE',  ( 5.405949406249999534, 9.363379034771803333, -149.5937500020483810 ) ) ;
#29730=AXIS2_PLACEMENT_3D ( 'NONE', #42578, #39141, #39557 ) ;
#29734=CARTESIAN_POINT ( 'NONE',  ( -9.999999999999998224, 1.224646799147353059E-15, -0.1250000040967647053 ) ) ;
#29735=CYLINDRICAL_SURFACE ( 'NONE', #32932, 9.999999999999998224 ) ;
#29737=CARTESIAN_POINT ( 'NONE',  ( -10.81189881249999729, 1.324075727343319199E-15, -122.0937500020483952 ) ) ;
#29738=CARTESIAN_POINT ( 'NONE',  ( -10.81189881249999729, 1.324075727343319199E-15, -95.28125000204838102 ) ) ;
#29739=CARTESIAN_POINT ( 'NONE',  ( -10.81189881249999729, 1.324075727343319199E-15, -107.0937500020483810 ) ) ;
#29742=CARTESIAN_POINT ( 'NONE',  ( -2.121150477449813534E-15, -11.54700538379251284, -161.7500000040967620 ) ) ;
#29743=DIRECTION ( 'NONE',  ( -0.000000000000000000, -0.000000000000000000, 1.000000000000000000 ) ) ;
#29746=EDGE_CURVE ( 'NONE', #13020, #36434, #12189, .T. ) ;
#29748=CARTESIAN_POINT ( 'NONE',  ( 10.00000000000025402, -5.773502691896113426, -189.6250000000000000 ) ) ;
#29752=CARTESIAN_POINT ( 'NONE',  ( 9.999999999999998224, 0.000000000000000000, -82.99999999999997158 ) ) ;
#29754=CARTESIAN_POINT ( 'NONE',  ( 10.00000000000000000, 5.773502691896255534, -89.25000000409677625 ) ) ;
#29757=CARTESIAN_POINT ( 'NONE',  ( -10.81189881249999729, 6.242252689847871849, -87.90625000204838102 ) ) ;
#29758=ORIENTED_EDGE ( 'NONE', *, *, #25190, .F. ) ;
#29760=CARTESIAN_POINT ( 'NONE',  ( 9.999999999999998224, 0.000000000000000000, -200.0000000000000000 ) ) ;
#29762=EDGE_LOOP ( 'NONE', ( #3548, #33173, #1155, #29559 ) ) ;
#29763=CARTESIAN_POINT ( 'NONE',  ( -9.999999999999998224, 5.773502691896259087, -11.87499999999996092 ) ) ;
#29764=CARTESIAN_POINT ( 'NONE',  ( -10.00000000000000000, -5.773502691896251982, -142.1250000000000000 ) ) ;
#29765=CYLINDRICAL_SURFACE ( 'NONE', #31042, 9.999999999999998224 ) ;
#29770=CARTESIAN_POINT ( 'NONE',  ( 5.000000000000000000, 8.660254037844385522, -190.7500000000000000 ) ) ;
#29771=CARTESIAN_POINT ( 'NONE',  ( 9.999999999999998224, 0.000000000000000000, -183.8750000040967905 ) ) ;
#29773=CARTESIAN_POINT ( 'NONE',  ( -2.293366432827344421E-15, -12.48450537969573659, -115.9062500020483810 ) ) ;
#29775=CARTESIAN_POINT ( 'NONE',  ( -9.999999999999998224, 1.224646799147353059E-15, -200.0000000000000000 ) ) ;
#29776=( BOUNDED_CURVE ( )  B_SPLINE_CURVE ( 2, ( #4595, #8054, #30295, #21201, #10414, #34387, #4804 ),
 .UNSPECIFIED., .F., .F. ) 
 B_SPLINE_CURVE_WITH_KNOTS ( ( 3, 2, 2, 3 ),
 ( 0.04104477611940302029, 0.04228855721393039169, 0.04353233830845775615, 0.04477611940298512061 ),
 .UNSPECIFIED. ) 
 CURVE ( )  GEOMETRIC_REPRESENTATION_ITEM ( )  RATIONAL_B_SPLINE_CURVE ( ( 0.9999999999999963363, 0.8660254037844424824, 1.000000000000000000, 0.8660254037844387076, 1.000000000000000000, 0.8660254037844334896, 1.000000000000005329 ) ) 
 REPRESENTATION_ITEM ( '' )  );
#29777=ORIENTED_EDGE ( 'NONE', *, *, #21736, .F. ) ;
#29778=CARTESIAN_POINT ( 'NONE',  ( 5.405949406249992428, -9.363379034771808662, -49.78125000204838813 ) ) ;
#29780=AXIS2_PLACEMENT_3D ( 'NONE', #22117, #34867, #15195 ) ;
#29781=CARTESIAN_POINT ( 'NONE',  ( 10.81189881249999551, -6.242252689847874514, -92.96875000204838102 ) ) ;
#29782=CARTESIAN_POINT ( 'NONE',  ( 5.405949406249992428, -9.363379034771808662, -120.2812500020483952 ) ) ;
#29783=VERTEX_POINT ( 'NONE', #25591 ) ;
#29784=CARTESIAN_POINT ( 'NONE',  ( -9.999999999999998224, 1.224646799147353059E-15, -138.1250000040967620 ) ) ;
#29786=CARTESIAN_POINT ( 'NONE',  ( 0.000000000000000000, 0.000000000000000000, -200.0000000000000000 ) ) ;
#29787=CARTESIAN_POINT ( 'NONE',  ( -5.405949406250003975, -9.363379034771801557, -130.8437500020484094 ) ) ;
#29789=FACE_OUTER_BOUND ( 'NONE', #14486, .T. ) ;
#29791=CARTESIAN_POINT ( 'NONE',  ( 5.000000000000000000, 8.660254037844385522, -182.1250000040967905 ) ) ;
#29794=CARTESIAN_POINT ( 'NONE',  ( 5.405949406249999534, 9.363379034771803333, -182.7812500020484094 ) ) ;
#29795=ADVANCED_FACE ( 'NONE', ( #38746 ), #28833, .T. ) ;
#29796=CARTESIAN_POINT ( 'NONE',  ( 9.999999999999998224, 0.000000000000000000, -185.3750000040967905 ) ) ;
#29799=CARTESIAN_POINT ( 'NONE',  ( -5.405949406249996869, 9.363379034771805109, -59.34375000204835970 ) ) ;
#29800=CARTESIAN_POINT ( 'NONE',  ( -10.81189881249999729, 1.324075727343319199E-15, -47.09375000204838102 ) ) ;
#29802=CARTESIAN_POINT ( 'NONE',  ( -10.81189881249999907, -6.242252689847864744, -18.65625000204837036 ) ) ;
#29804=CARTESIAN_POINT ( 'NONE',  ( 5.000000000000000000, 8.660254037844385522, -145.7500000000000000 ) ) ;
#29806=CARTESIAN_POINT ( 'NONE',  ( 7.070501591499377789E-16, 11.54700538379251284, -102.1250000000000000 ) ) ;
#29808=CARTESIAN_POINT ( 'NONE',  ( 0.000000000000000000, 0.000000000000000000, -200.0000000000000000 ) ) ;
#29811=CARTESIAN_POINT ( 'NONE',  ( 10.81189881249999729, 6.242252689847867408, -112.4062500020483952 ) ) ;
#29812=ORIENTED_EDGE ( 'NONE', *, *, #28084, .T. ) ;
#29818=CARTESIAN_POINT ( 'NONE',  ( 9.999999999999998224, 0.000000000000000000, -33.49999999999997158 ) ) ;
#29819=AXIS2_PLACEMENT_3D ( 'NONE', #3059, #32211, #35864 ) ;
#29820=CARTESIAN_POINT ( 'NONE',  ( -4.999999999999996447, 8.660254037844387298, -16.87500000409675138 ) ) ;
#29821=CARTESIAN_POINT ( 'NONE',  ( -5.405949406249996869, 9.363379034771805109, -40.03125000204838102 ) ) ;
#29822=LINE ( 'NONE', #3703, #30419 ) ;
#29824=( BOUNDED_CURVE ( )  B_SPLINE_CURVE ( 2, ( #6792, #17123, #30326, #23200, #26434, #33354, #10652 ),
 .UNSPECIFIED., .F., .F. ) 
 B_SPLINE_CURVE_WITH_KNOTS ( ( 3, 2, 2, 3 ),
 ( 0.4888059701492538101, 0.4900497512437811398, 0.4912935323383085806, 0.4925373134328359104 ),
 .UNSPECIFIED. ) 
 CURVE ( )  GEOMETRIC_REPRESENTATION_ITEM ( )  RATIONAL_B_SPLINE_CURVE ( ( 0.9999999999999940048, 0.8660254037844447028, 1.000000000000000000, 0.8660254037844387076, 1.000000000000000000, 0.8660254037844267172, 1.000000000000011990 ) ) 
 REPRESENTATION_ITEM ( '' )  );
#29825=CARTESIAN_POINT ( 'NONE',  ( 9.999999999999742428, 5.773502691896404748, -156.7500000040967905 ) ) ;
#29826=CARTESIAN_POINT ( 'NONE',  ( 5.405949406249992428, -9.363379034771808662, -144.2812500020483810 ) ) ;
#29827=ADVANCED_FACE ( 'NONE', ( #9175 ), #25798, .T. ) ;
#29828=CARTESIAN_POINT ( 'NONE',  ( 9.999999999999998224, 0.000000000000000000, -15.49999999999995737 ) ) ;
#29829=VERTEX_POINT ( 'NONE', #21915 ) ;
#29833=CARTESIAN_POINT ( 'NONE',  ( -9.999999999999998224, 1.224646799147353059E-15, -200.0000000000000000 ) ) ;
#29834=CARTESIAN_POINT ( 'NONE',  ( 10.81189881249999551, -6.242252689847874514, -173.9687500020484094 ) ) ;
#29835=VECTOR ( 'NONE', #38352, 1000.000000000000000 ) ;
#29836=CARTESIAN_POINT ( 'NONE',  ( -5.405949406250003975, -9.363379034771801557, -24.34375000204835970 ) ) ;
#29838=CARTESIAN_POINT ( 'NONE',  ( 7.644554776091147741E-16, 12.48450537969573659, -152.4687500020484094 ) ) ;
#29839=CARTESIAN_POINT ( 'NONE',  ( 10.81189881249999551, -6.242252689847874514, -145.4687500020483810 ) ) ;
#29840=CARTESIAN_POINT ( 'NONE',  ( -7.071067811865477282, 7.071067811865471064, -200.0000000000000000 ) ) ;
#29843=CARTESIAN_POINT ( 'NONE',  ( -5.405949406249996869, 9.363379034771805109, -6.843750002048371250 ) ) ;
#29845=FACE_OUTER_BOUND ( 'NONE', #19146, .T. ) ;
#29846=CARTESIAN_POINT ( 'NONE',  ( 9.999999999999998224, 0.000000000000000000, -200.0000000000000000 ) ) ;
#29849=CARTESIAN_POINT ( 'NONE',  ( -10.81189881249999729, 1.324075727343319199E-15, -75.59375000204838102 ) ) ;
#29850=CARTESIAN_POINT ( 'NONE',  ( -10.81189881249999729, 1.324075727343319199E-15, -41.28125000204838102 ) ) ;
#29854=CARTESIAN_POINT ( 'NONE',  ( 9.999999999999996447, -5.773502691896262640, -126.6250000000000000 ) ) ;
#29855=CARTESIAN_POINT ( 'NONE',  ( 10.81189881249999551, -6.242252689847874514, -139.6562500020484094 ) ) ;
#29856=CARTESIAN_POINT ( 'NONE',  ( 9.999999999999998224, 0.000000000000000000, -23.37500000409675849 ) ) ;
#29857=CARTESIAN_POINT ( 'NONE',  ( -10.00000000000000000, -5.773502691896251982, -115.5000000040967905 ) ) ;
#29859=EDGE_LOOP ( 'NONE', ( #3074, #29023, #10690, #4016 ) ) ;
#29863=CARTESIAN_POINT ( 'NONE',  ( -2.293366432827344421E-15, -12.48450537969573659, -165.4062500020483810 ) ) ;
#29864=CARTESIAN_POINT ( 'NONE',  ( 7.070501591499377789E-16, 11.54700538379251284, -41.00000000409676204 ) ) ;
#29866=CARTESIAN_POINT ( 'NONE',  ( -10.81189881249999907, -6.242252689847864744, -164.1562500020484094 ) ) ;
#29867=CARTESIAN_POINT ( 'NONE',  ( -5.405949406249996869, 9.363379034771805109, -137.3437500020484094 ) ) ;
#29868=CARTESIAN_POINT ( 'NONE',  ( 7.070501591499376803E-16, 11.54700538379251284, -100.6250000000000000 ) ) ;
#29869=DIRECTION ( 'NONE',  ( 1.000000000000000000, 0.000000000000000000, 0.000000000000000000 ) ) ;
#29871=ORIENTED_EDGE ( 'NONE', *, *, #15271, .F. ) ;
#29874=CARTESIAN_POINT ( 'NONE',  ( -5.405949406250003975, -9.363379034771801557, -72.53125000204838102 ) ) ;
#29877=CARTESIAN_POINT ( 'NONE',  ( -10.81189881249999907, -6.242252689847864744, -118.9687500020483810 ) ) ;
#29878=ORIENTED_EDGE ( 'NONE', *, *, #25157, .T. ) ;
#29879=ORIENTED_EDGE ( 'NONE', *, *, #5615, .F. ) ;
#29880=CARTESIAN_POINT ( 'NONE',  ( 10.81189881249999729, 6.242252689847867408, -19.21875000204837747 ) ) ;
#29881=CARTESIAN_POINT ( 'NONE',  ( -2.293366432827344421E-15, -12.48450537969573659, -0.4062500020483658103 ) ) ;
#29882=CARTESIAN_POINT ( 'NONE',  ( -5.405949406250003975, -9.363379034771801557, -45.34375000204838102 ) ) ;
#29884=CARTESIAN_POINT ( 'NONE',  ( 0.000000000000000000, 0.000000000000000000, -200.0000000000000000 ) ) ;
#29885=CARTESIAN_POINT ( 'NONE',  ( 10.81189881249999551, -6.242252689847874514, -178.4687500020484094 ) ) ;
#29886=CARTESIAN_POINT ( 'NONE',  ( 10.81189881249999729, 0.000000000000000000, -169.3437500020484094 ) ) ;
#29887=( BOUNDED_CURVE ( )  B_SPLINE_CURVE ( 2, ( #25562, #41290, #1830, #22524, #35697, #11944, #5270 ),
 .UNSPECIFIED., .F., .F. ) 
 B_SPLINE_CURVE_WITH_KNOTS ( ( 3, 2, 2, 3 ),
 ( 0.9104477611940301474, 0.9116915422885575326, 0.9129353233830848069, 0.9141791044776121922 ),
 .UNSPECIFIED. ) 
 CURVE ( )  GEOMETRIC_REPRESENTATION_ITEM ( )  RATIONAL_B_SPLINE_CURVE ( ( 0.9999999999999641398, 0.8660254037844745678, 1.000000000000000000, 0.8660254037844387076, 1.000000000000000000, 0.8660254037844148378, 1.000000000000023981 ) ) 
 REPRESENTATION_ITEM ( '' )  );
#29893=CARTESIAN_POINT ( 'NONE',  ( 5.405949406249999534, 9.363379034771803333, -97.09375000204838102 ) ) ;
#29894=CARTESIAN_POINT ( 'NONE',  ( -4.999999999999996447, 8.660254037844387298, -34.49999999999997158 ) ) ;
#29895=CARTESIAN_POINT ( 'NONE',  ( 5.405949406249992428, -9.363379034771808662, -69.28125000204838102 ) ) ;
#29899=CARTESIAN_POINT ( 'NONE',  ( -10.81189881249999729, 1.324075727343319199E-15, -119.2812500020483952 ) ) ;
#29900=CARTESIAN_POINT ( 'NONE',  ( -10.81189881249999729, 6.242252689847871849, -165.9062500020483810 ) ) ;
#29902=CARTESIAN_POINT ( 'NONE',  ( -9.999999999999998224, 1.224646799147353059E-15, -141.1250000040967905 ) ) ;
#29904=ORIENTED_EDGE ( 'NONE', *, *, #23199, .T. ) ;
#29907=CARTESIAN_POINT ( 'NONE',  ( -10.81189881249999729, 6.242252689847871849, -185.4062500020484094 ) ) ;
#29908=CARTESIAN_POINT ( 'NONE',  ( 4.999999999999992006, -8.660254037844389075, -43.12500000409677625 ) ) ;
#29910=ORIENTED_EDGE ( 'NONE', *, *, #18589, .F. ) ;
#29911=CARTESIAN_POINT ( 'NONE',  ( 9.999999999999996447, -5.773502691896262640, -59.12499999999999289 ) ) ;
#29913=CARTESIAN_POINT ( 'NONE',  ( -9.999999999999998224, 5.773502691896259087, -67.75000000409677625 ) ) ;
#29917=CARTESIAN_POINT ( 'NONE',  ( 10.81189881249999729, 0.000000000000000000, -57.03125000204836681 ) ) ;
#29920=CYLINDRICAL_SURFACE ( 'NONE', #33841, 9.999999999999998224 ) ;
#29921=CARTESIAN_POINT ( 'NONE',  ( 7.644554776091147741E-16, 12.48450537969573659, -187.1562500020484094 ) ) ;
#29923=CARTESIAN_POINT ( 'NONE',  ( -5.405949406250003975, -9.363379034771801557, -0.3437500020483652552 ) ) ;
#29924=CARTESIAN_POINT ( 'NONE',  ( -9.999999999999742428, -5.773502691896402084, -118.1249999999999858 ) ) ;
#29926=CARTESIAN_POINT ( 'NONE',  ( -2.121150477449813534E-15, -11.54700538379251284, -45.87499999999996447 ) ) ;
#29928=EDGE_CURVE ( 'NONE', #30365, #12272, #9593, .T. ) ;
#29929=CARTESIAN_POINT ( 'NONE',  ( 9.999999999999998224, 0.000000000000000000, -168.5000000000000000 ) ) ;
#29930=CARTESIAN_POINT ( 'NONE',  ( -9.999999999999998224, 1.224646799147353059E-15, -200.0000000000000000 ) ) ;
#29931=EDGE_CURVE ( 'NONE', #6986, #3313, #26424, .T. ) ;
#29932=CARTESIAN_POINT ( 'NONE',  ( 10.81189881249999729, 0.000000000000000000, -94.53125000204838102 ) ) ;
#29933=EDGE_LOOP ( 'NONE', ( #12085, #13556, #38848, #21796 ) ) ;
#29934=CARTESIAN_POINT ( 'NONE',  ( 5.000000000000000000, 8.660254037844385522, -107.1250000040967763 ) ) ;
#29936=VERTEX_POINT ( 'NONE', #22767 ) ;
#29938=( BOUNDED_CURVE ( )  B_SPLINE_CURVE ( 2, ( #24015, #3734, #16864, #30067, #39969, #37156, #20121 ),
 .UNSPECIFIED., .F., .F. ) 
 B_SPLINE_CURVE_WITH_KNOTS ( ( 3, 2, 2, 3 ),
 ( 0.2947761194029852039, 0.2960199004975125336, 0.2972636815920398634, 0.2985074626865671932 ),
 .UNSPECIFIED. ) 
 CURVE ( )  GEOMETRIC_REPRESENTATION_ITEM ( )  RATIONAL_B_SPLINE_CURVE ( ( 0.9999999999999880096, 0.8660254037844506980, 1.000000000000000000, 0.8660254037844387076, 1.000000000000000000, 0.8660254037844327124, 1.000000000000005995 ) ) 
 REPRESENTATION_ITEM ( '' )  );
#29939=CARTESIAN_POINT ( 'NONE',  ( 10.81189881249999551, -6.242252689847874514, -35.96875000204835260 ) ) ;
#29940=CARTESIAN_POINT ( 'NONE',  ( -5.405949406250003975, -9.363379034771801557, -18.53125000204835970 ) ) ;
#29941=CARTESIAN_POINT ( 'NONE',  ( -10.81189881249999729, 1.324075727343319199E-15, -71.09375000204836681 ) ) ;
#29943=CARTESIAN_POINT ( 'NONE',  ( -10.81189881249999729, 6.242252689847871849, -192.7187500020483810 ) ) ;
#29944=CARTESIAN_POINT ( 'NONE',  ( 10.81189881249999551, -6.242252689847874514, -149.9687500020483810 ) ) ;
#29946=CARTESIAN_POINT ( 'NONE',  ( -9.999999999999998224, 1.224646799147353059E-15, -79.62500000409677625 ) ) ;
#29950=CARTESIAN_POINT ( 'NONE',  ( 7.070501591499377789E-16, 11.54700538379251284, -3.500000004096760264 ) ) ;
#29951=CARTESIAN_POINT ( 'NONE',  ( 4.999999999999992006, -8.660254037844389075, -103.1250000040967763 ) ) ;
#29952=CARTESIAN_POINT ( 'NONE',  ( -2.293366432827344421E-15, -12.48450537969573659, -117.2187500020483952 ) ) ;
#29953=CARTESIAN_POINT ( 'NONE',  ( -1.040834085586084257E-14, 20.00000000000000711, 32.49999999999999289 ) ) ;
#29954=CARTESIAN_POINT ( 'NONE',  ( -5.405949406250003975, -9.363379034771801557, -87.53125000204838102 ) ) ;
#29955=CARTESIAN_POINT ( 'NONE',  ( -10.81189881249999729, -6.242252689847864744, -111.4687500020483810 ) ) ;
#29958=CARTESIAN_POINT ( 'NONE',  ( -10.00000000000000000, -5.773502691896251982, -160.5000000040967905 ) ) ;
#29962=CARTESIAN_POINT ( 'NONE',  ( 9.999999999999998224, 0.000000000000000000, -129.5000000000000000 ) ) ;
#29964=CARTESIAN_POINT ( 'NONE',  ( -9.999999999999998224, 1.224646799147353059E-15, -109.2499999999999858 ) ) ;
#29966=CARTESIAN_POINT ( 'NONE',  ( -9.999999999999998224, 1.224646799147353059E-15, -83.74999999999997158 ) ) ;
#29968=CARTESIAN_POINT ( 'NONE',  ( 7.070501591499377789E-16, 11.54700538379251284, -87.50000000409677625 ) ) ;
#29969=CARTESIAN_POINT ( 'NONE',  ( -9.999999999999998224, 1.224646799147353059E-15, -115.2499999999999858 ) ) ;
#29971=CARTESIAN_POINT ( 'NONE',  ( 10.81189881249999551, -6.242252689847874514, -82.65625000204838102 ) ) ;
#29972=ORIENTED_EDGE ( 'NONE', *, *, #19620, .F. ) ;
#29974=CARTESIAN_POINT ( 'NONE',  ( -9.999999999999998224, 1.224646799147353059E-15, -121.6250000040967905 ) ) ;
#29976=ORIENTED_EDGE ( 'NONE', *, *, #8284, .T. ) ;
#29977=CARTESIAN_POINT ( 'NONE',  ( -2.121150477449813534E-15, -11.54700538379251284, -8.374999999999976907 ) ) ;
#29978=CARTESIAN_POINT ( 'NONE',  ( 10.00000000000000000, 5.773502691896255534, -142.8750000000000000 ) ) ;
#29979=CARTESIAN_POINT ( 'NONE',  ( 0.000000000000000000, 0.000000000000000000, -200.0000000000000000 ) ) ;
#29982=CARTESIAN_POINT ( 'NONE',  ( 5.000000000000000000, 8.660254037844385522, -193.7500000000000000 ) ) ;
#29984=CARTESIAN_POINT ( 'NONE',  ( 10.81189881249999551, -6.242252689847874514, -121.6562500020483952 ) ) ;
#29985=ORIENTED_EDGE ( 'NONE', *, *, #26372, .T. ) ;
#29986=VERTEX_POINT ( 'NONE', #3553 ) ;
#29987=CARTESIAN_POINT ( 'NONE',  ( -10.81189881249999729, 6.242252689847871849, -45.90625000204836681 ) ) ;
#29989=EDGE_CURVE ( 'NONE', #22184, #37944, #10220, .T. ) ;
#29990=CARTESIAN_POINT ( 'NONE',  ( -5.405949406250003975, -9.363379034771801557, -97.84375000204838102 ) ) ;
#29991=CARTESIAN_POINT ( 'NONE',  ( 10.81189881249999551, -6.242252689847874514, -124.6562500020483952 ) ) ;
#29992=ORIENTED_EDGE ( 'NONE', *, *, #36775, .T. ) ;
#29993=CARTESIAN_POINT ( 'NONE',  ( 9.999999999999998224, 0.000000000000000000, -111.4999999999999858 ) ) ;
#29994=CARTESIAN_POINT ( 'NONE',  ( -9.999999999999227285, -5.773502691896698735, -126.0000000040967478 ) ) ;
#29997=CARTESIAN_POINT ( 'NONE',  ( -10.81189881249999729, 1.324075727343319199E-15, -131.0937500020483810 ) ) ;
#30001=CARTESIAN_POINT ( 'NONE',  ( 9.999999999999996447, -5.773502691896262640, -184.0000000040968189 ) ) ;
#30003=CARTESIAN_POINT ( 'NONE',  ( 5.405949406249999534, 9.363379034771803333, -184.2812500020484094 ) ) ;
#30004=AXIS2_PLACEMENT_3D ( 'NONE', #41185, #28059, #31732 ) ;
#30008=CARTESIAN_POINT ( 'NONE',  ( -10.81189881249999729, 6.242252689847871849, -56.21875000204837391 ) ) ;
#30009=CARTESIAN_POINT ( 'NONE',  ( 5.405949406249992428, -9.363379034771808662, -40.59375000204837391 ) ) ;
#30011=CARTESIAN_POINT ( 'NONE',  ( 10.81189881249999551, -6.242252689847874514, -19.65625000204837747 ) ) ;
#30013=CARTESIAN_POINT ( 'NONE',  ( -9.999999999999998224, 1.224646799147353059E-15, -120.1250000040967905 ) ) ;
#30015=CARTESIAN_POINT ( 'NONE',  ( -4.999999999999996447, 8.660254037844387298, -109.4999999999999858 ) ) ;
#30020=CARTESIAN_POINT ( 'NONE',  ( -10.81189881249999729, 6.242252689847871849, -107.4062500020483668 ) ) ;
#30021=ORIENTED_EDGE ( 'NONE', *, *, #7149, .T. ) ;
#30022=DIRECTION ( 'NONE',  ( -0.000000000000000000, -0.000000000000000000, 1.000000000000000000 ) ) ;
#30024=MANIFOLD_SOLID_BREP ( 'Cut-Extrude1', #38410 ) ;
#30028=CARTESIAN_POINT ( 'NONE',  ( -2.121150477449813534E-15, -11.54700538379251284, -33.87499999999996447 ) ) ;
#30029=CARTESIAN_POINT ( 'NONE',  ( 10.00000000000000000, 5.773502691896255534, -18.75000000409676915 ) ) ;
#30030=CARTESIAN_POINT ( 'NONE',  ( -5.405949406249996869, 9.363379034771805109, -44.53125000204838102 ) ) ;
#30032=( BOUNDED_CURVE ( )  B_SPLINE_CURVE ( 2, ( #41369, #11806, #13806, #40149, #5139, #28018, #14012 ),
 .UNSPECIFIED., .F., .F. ) 
 B_SPLINE_CURVE_WITH_KNOTS ( ( 3, 2, 2, 3 ),
 ( 0.1865671641791045166, 0.1878109452736318741, 0.1890547263681592594, 0.1902985074626866169 ),
 .UNSPECIFIED. ) 
 CURVE ( )  GEOMETRIC_REPRESENTATION_ITEM ( )  RATIONAL_B_SPLINE_CURVE ( ( 0.9999999999999970024, 0.8660254037844417052, 1.000000000000000000, 0.8660254037844387076, 1.000000000000000000, 0.8660254037844327124, 1.000000000000005995 ) ) 
 REPRESENTATION_ITEM ( '' )  );
#30034=VECTOR ( 'NONE', #36167, 1000.000000000000000 ) ;
#30035=CARTESIAN_POINT ( 'NONE',  ( 9.999999999999998224, 0.000000000000000000, -57.87500000409676204 ) ) ;
#30036=CARTESIAN_POINT ( 'NONE',  ( -2.293366432827344421E-15, -12.48450537969573659, -141.4062500020483810 ) ) ;
#30039=ORIENTED_EDGE ( 'NONE', *, *, #33871, .F. ) ;
#30042=CARTESIAN_POINT ( 'NONE',  ( 10.81189881249999551, -6.242252689847874514, -170.9687500020483810 ) ) ;
#30044=CARTESIAN_POINT ( 'NONE',  ( 10.81189881249999729, 0.000000000000000000, -25.34375000204835970 ) ) ;
#30045=CARTESIAN_POINT ( 'NONE',  ( -9.999999999998969713, -5.773502691896847949, -33.00000000409673362 ) ) ;
#30046=CARTESIAN_POINT ( 'NONE',  ( 5.000000000000000000, 8.660254037844385522, -171.2500000000000000 ) ) ;
#30047=CARTESIAN_POINT ( 'NONE',  ( 7.644554776091147741E-16, 12.48450537969573659, -158.4687500020483810 ) ) ;
#30048=CARTESIAN_POINT ( 'NONE',  ( 10.81189881249999729, 0.000000000000000000, -133.3437500020484094 ) ) ;
#30050=CARTESIAN_POINT ( 'NONE',  ( 7.070501591499376803E-16, 11.54700538379251284, -173.0000000040967905 ) ) ;
#30053=VECTOR ( 'NONE', #38479, 1000.000000000000000 ) ;
#30055=( BOUNDED_CURVE ( )  B_SPLINE_CURVE ( 2, ( #37352, #1318, #4758, #31535, #27642, #15093, #11224 ),
 .UNSPECIFIED., .F., .F. ) 
 B_SPLINE_CURVE_WITH_KNOTS ( ( 3, 2, 2, 3 ),
 ( 0.7611940298507464675, 0.7624378109452738528, 0.7636815920398011270, 0.7649253731343285123 ),
 .UNSPECIFIED. ) 
 CURVE ( )  GEOMETRIC_REPRESENTATION_ITEM ( )  RATIONAL_B_SPLINE_CURVE ( ( 0.9999999999999761302, 0.8660254037844625774, 1.000000000000000000, 0.8660254037844387076, 1.000000000000000000, 0.8660254037844267172, 1.000000000000011990 ) ) 
 REPRESENTATION_ITEM ( '' )  );
#30056=CARTESIAN_POINT ( 'NONE',  ( 10.81189881249999729, 0.000000000000000000, -10.34375000204834549 ) ) ;
#30059=VECTOR ( 'NONE', #2547, 1000.000000000000000 ) ;
#30060=CARTESIAN_POINT ( 'NONE',  ( 5.000000000000000000, 8.660254037844385522, -25.74999999999996803 ) ) ;
#30062=DIRECTION ( 'NONE',  ( -0.000000000000000000, -0.000000000000000000, 1.000000000000000000 ) ) ;
#30063=CARTESIAN_POINT ( 'NONE',  ( -2.293366432827344421E-15, -12.48450537969573659, -84.21875000204835260 ) ) ;
#30064=CARTESIAN_POINT ( 'NONE',  ( 5.405949406249999534, 9.363379034771803333, -71.59375000204836681 ) ) ;
#30065=CARTESIAN_POINT ( 'NONE',  ( 5.405949406249992428, -9.363379034771808662, -45.28125000204838102 ) ) ;
#30067=CARTESIAN_POINT ( 'NONE',  ( -2.121150477449813534E-15, -11.54700538379251284, -139.2500000040967905 ) ) ;
#30069=CARTESIAN_POINT ( 'NONE',  ( 7.070501591499377789E-16, 11.54700538379251284, -130.6250000000000000 ) ) ;
#30070=CARTESIAN_POINT ( 'NONE',  ( 5.405949406249999534, 9.363379034771803333, -140.7812500020483810 ) ) ;
#30073=CARTESIAN_POINT ( 'NONE',  ( -10.81189881249999729, 1.324075727343319199E-15, -20.28125000204836326 ) ) ;
#30074=ORIENTED_EDGE ( 'NONE', *, *, #32848, .F. ) ;
#30075=( BOUNDED_CURVE ( )  B_SPLINE_CURVE ( 2, ( #29796, #452, #6692, #5482, #28794, #25341, #3679 ),
 .UNSPECIFIED., .F., .F. ) 
 B_SPLINE_CURVE_WITH_KNOTS ( ( 3, 2, 2, 3 ),
 ( 0.06716417910447768091, 0.06840796019900503844, 0.06965174129353240984, 0.07089552238805976736 ),
 .UNSPECIFIED. ) 
 CURVE ( )  GEOMETRIC_REPRESENTATION_ITEM ( )  RATIONAL_B_SPLINE_CURVE ( ( 0.9999999999999924505, 0.8660254037844461461, 1.000000000000000000, 0.8660254037844387076, 1.000000000000000000, 0.8660254037844312691, 1.000000000000007550 ) ) 
 REPRESENTATION_ITEM ( '' )  );
#30078=LINE ( 'NONE', #16661, #7792 ) ;
#30079=CARTESIAN_POINT ( 'NONE',  ( -10.81189881249999729, 6.242252689847871849, -167.4062500020483810 ) ) ;
#30080=CARTESIAN_POINT ( 'NONE',  ( 9.999999999999998224, 0.000000000000000000, -39.87500000409676915 ) ) ;
#30081=DIRECTION ( 'NONE',  ( -0.000000000000000000, -0.000000000000000000, 1.000000000000000000 ) ) ;
#30083=( BOUNDED_CURVE ( )  B_SPLINE_CURVE ( 2, ( #20984, #21409, #21196, #41031, #30924, #34383, #8479 ),
 .UNSPECIFIED., .F., .F. ) 
 B_SPLINE_CURVE_WITH_KNOTS ( ( 3, 2, 2, 3 ),
 ( 0.09328358208955218889, 0.09452736318407958804, 0.09577114427860700108, 0.09701492537313441411 ),
 .UNSPECIFIED. ) 
 CURVE ( )  GEOMETRIC_REPRESENTATION_ITEM ( )  RATIONAL_B_SPLINE_CURVE ( ( 1.000000000000005995, 0.8660254037844327124, 1.000000000000000000, 0.8660254037844387076, 1.000000000000000000, 0.8660254037844297148, 1.000000000000008882 ) ) 
 REPRESENTATION_ITEM ( '' )  );
#30084=CARTESIAN_POINT ( 'NONE',  ( 5.000000000000000000, 8.660254037844385522, -45.24999999999998579 ) ) ;
#30085=CARTESIAN_POINT ( 'NONE',  ( -10.81189881249999907, -6.242252689847864744, -161.1562500020484094 ) ) ;
#30086=CARTESIAN_POINT ( 'NONE',  ( -10.81189881249999729, 1.324075727343319199E-15, -135.5937500020483810 ) ) ;
#30087=DIRECTION ( 'NONE',  ( -0.000000000000000000, -0.000000000000000000, 1.000000000000000000 ) ) ;
#30088=CARTESIAN_POINT ( 'NONE',  ( -10.00000000000051337, 5.773502691895962435, -149.8750000000000000 ) ) ;
#30089=ORIENTED_EDGE ( 'NONE', *, *, #17764, .T. ) ;
#30091=VECTOR ( 'NONE', #605, 1000.000000000000000 ) ;
#30092=CARTESIAN_POINT ( 'NONE',  ( 7.644554776091147741E-16, 12.48450537969573659, -73.15625000204836681 ) ) ;
#30094=CARTESIAN_POINT ( 'NONE',  ( -10.81189881249999729, 6.242252689847871849, -117.7187500020483952 ) ) ;
#30095=EDGE_LOOP ( 'NONE', ( #39732, #1740, #12414, #32062 ) ) ;
#30096=CARTESIAN_POINT ( 'NONE',  ( -10.81189881249999729, 6.242252689847871849, -24.71875000204837036 ) ) ;
#30097=CARTESIAN_POINT ( 'NONE',  ( -10.81189881249999729, 6.242252689847871849, -197.2187500020484379 ) ) ;
#30098=CARTESIAN_POINT ( 'NONE',  ( -10.81189881249999907, -6.242252689847864744, -46.96875000204835970 ) ) ;
#30099=CYLINDRICAL_SURFACE ( 'NONE', #26066, 9.999999999999998224 ) ;
#30101=CARTESIAN_POINT ( 'NONE',  ( -2.293366432827344421E-15, -12.48450537969573659, -180.2187500020484094 ) ) ;
#30102=CARTESIAN_POINT ( 'NONE',  ( 10.81189881249999729, 0.000000000000000000, -172.3437500020484094 ) ) ;
#30105=DIRECTION ( 'NONE',  ( 1.000000000000000000, 0.000000000000000000, 0.000000000000000000 ) ) ;
#30108=CARTESIAN_POINT ( 'NONE',  ( -5.405949406249996869, 9.363379034771805109, -99.84375000204838102 ) ) ;
#30109=CYLINDRICAL_SURFACE ( 'NONE', #7252, 9.999999999999998224 ) ;
#30110=CARTESIAN_POINT ( 'NONE',  ( 5.405949406249992428, -9.363379034771808662, -66.28125000204838102 ) ) ;
#30112=EDGE_CURVE ( 'NONE', #31960, #24932, #3714, .T. ) ;
#30114=CARTESIAN_POINT ( 'NONE',  ( -10.81189881249999729, 6.242252689847871849, -125.4062500020483810 ) ) ;
#30115=CARTESIAN_POINT ( 'NONE',  ( -10.81189881249999729, 1.324075727343319199E-15, -161.2812500020484094 ) ) ;
#30117=CARTESIAN_POINT ( 'NONE',  ( -9.999999999999998224, 5.773502691896259087, -139.7500000040967905 ) ) ;
#30119=ORIENTED_EDGE ( 'NONE', *, *, #21426, .T. ) ;
#30122=CARTESIAN_POINT ( 'NONE',  ( -10.81189881249999907, -6.242252689847864744, -189.6562500020484094 ) ) ;
#30125=ORIENTED_EDGE ( 'NONE', *, *, #20022, .T. ) ;
#30126=CARTESIAN_POINT ( 'NONE',  ( -9.999999999999998224, 5.773502691896259087, -55.37499999999997868 ) ) ;
#30128=CARTESIAN_POINT ( 'NONE',  ( 4.999999999999992006, -8.660254037844389075, -68.62500000409677625 ) ) ;
#30129=DIRECTION ( 'NONE',  ( -0.000000000000000000, -0.000000000000000000, 1.000000000000000000 ) ) ;
#30132=CARTESIAN_POINT ( 'NONE',  ( 10.81189881249999729, 6.242252689847867408, -56.90625000204838102 ) ) ;
#30135=CARTESIAN_POINT ( 'NONE',  ( 10.00000000000051159, -5.773502691895965988, -151.0000000040967905 ) ) ;
#30136=CARTESIAN_POINT ( 'NONE',  ( -10.81189881249999907, -6.242252689847864744, -182.1562500020483810 ) ) ;
#30138=CARTESIAN_POINT ( 'NONE',  ( 9.999999999998969713, 5.773502691896851502, -85.87499999999995737 ) ) ;
#30139=DIRECTION ( 'NONE',  ( 1.000000000000000000, 0.000000000000000000, 0.000000000000000000 ) ) ;
#30140=CARTESIAN_POINT ( 'NONE',  ( -9.999999999999998224, 1.224646799147353059E-15, -57.12500000409676204 ) ) ;
#30142=DIRECTION ( 'NONE',  ( 1.000000000000000000, 0.000000000000000000, 0.000000000000000000 ) ) ;
#30143=CARTESIAN_POINT ( 'NONE',  ( -2.293366432827344421E-15, -12.48450537969573659, -93.40625000204839523 ) ) ;
#30144=ORIENTED_EDGE ( 'NONE', *, *, #13116, .F. ) ;
#30145=CARTESIAN_POINT ( 'NONE',  ( -9.999999999999998224, 1.224646799147353059E-15, -106.6250000040967763 ) ) ;
#30147=ORIENTED_EDGE ( 'NONE', *, *, #20349, .F. ) ;
#30148=( BOUNDED_CURVE ( )  B_SPLINE_CURVE ( 2, ( #9712, #19634, #13357, #32817, #33027, #3457, #16592 ),
 .UNSPECIFIED., .F., .F. ) 
 B_SPLINE_CURVE_WITH_KNOTS ( ( 3, 2, 2, 3 ),
 ( 0.9552238805970153512, 0.9564676616915426255, 0.9577114427860698997, 0.9589552238805971740 ),
 .UNSPECIFIED. ) 
 CURVE ( )  GEOMETRIC_REPRESENTATION_ITEM ( )  RATIONAL_B_SPLINE_CURVE ( ( 0.9999999999999521494, 0.8660254037844865582, 1.000000000000000000, 0.8660254037844387076, 1.000000000000000000, 0.8660254037844267172, 1.000000000000011990 ) ) 
 REPRESENTATION_ITEM ( '' )  );
#30149=VERTEX_POINT ( 'NONE', #36555 ) ;
#30150=CARTESIAN_POINT ( 'NONE',  ( 7.644554776091147741E-16, 12.48450537969573659, -23.46875000204836326 ) ) ;
#30151=CARTESIAN_POINT ( 'NONE',  ( 5.405949406249999534, 9.363379034771803333, -22.28125000204836326 ) ) ;
#30153=CARTESIAN_POINT ( 'NONE',  ( 7.644554776091147741E-16, 12.48450537969573659, -68.46875000204838102 ) ) ;
#30154=CARTESIAN_POINT ( 'NONE',  ( -5.000000000000003553, -8.660254037844383745, -173.8750000040968189 ) ) ;
#30156=CARTESIAN_POINT ( 'NONE',  ( -5.405949406250003975, -9.363379034771801557, -195.3437500020484094 ) ) ;
#30157=CARTESIAN_POINT ( 'NONE',  ( 10.81189881249999551, -6.242252689847874514, -148.4687500020484094 ) ) ;
#30158=CARTESIAN_POINT ( 'NONE',  ( -9.999999999999998224, 1.224646799147353059E-15, -72.12500000409677625 ) ) ;
#30161=CARTESIAN_POINT ( 'NONE',  ( -5.000000000000003553, -8.660254037844383745, -2.875000004096767370 ) ) ;
#30162=CARTESIAN_POINT ( 'NONE',  ( 9.999999999999998224, 0.000000000000000000, -89.37500000409677625 ) ) ;
#30163=CARTESIAN_POINT ( 'NONE',  ( 10.81189881249999907, 6.242252689847868297, -124.2187500020483952 ) ) ;
#30165=CARTESIAN_POINT ( 'NONE',  ( 10.81189881249999729, 0.000000000000000000, -88.53125000204838102 ) ) ;
#30166=ADVANCED_FACE ( 'NONE', ( #32907 ), #36349, .T. ) ;
#30167=CARTESIAN_POINT ( 'NONE',  ( -10.81189881249999729, -6.242252689847864744, -100.9687500020483668 ) ) ;
#30168=EDGE_CURVE ( 'NONE', #15363, #25538, #42599, .T. ) ;
#30171=CARTESIAN_POINT ( 'NONE',  ( -4.999999999999996447, 8.660254037844387298, -162.3750000040967905 ) ) ;
#30172=ADVANCED_FACE ( 'NONE', ( #16897 ), #29671, .T. ) ;
#30175=FACE_OUTER_BOUND ( 'NONE', #33600, .T. ) ;
#30179=CARTESIAN_POINT ( 'NONE',  ( -10.00000000000000000, -5.773502691896251982, -80.62499999999998579 ) ) ;
#30181=CARTESIAN_POINT ( 'NONE',  ( 4.999999999999992006, -8.660254037844389075, -88.12500000409677625 ) ) ;
#30185=CARTESIAN_POINT ( 'NONE',  ( 5.405949406249992428, -9.363379034771808662, -81.28125000204839523 ) ) ;
#30186=ORIENTED_EDGE ( 'NONE', *, *, #42537, .F. ) ;
#30190=ORIENTED_EDGE ( 'NONE', *, *, #34899, .F. ) ;
#30191=CARTESIAN_POINT ( 'NONE',  ( 7.070501591499377789E-16, 11.54700538379251284, -9.124999999999978684 ) ) ;
#30193=CARTESIAN_POINT ( 'NONE',  ( -2.121150477449813534E-15, -11.54700538379251284, -147.8750000000000000 ) ) ;
#30196=( BOUNDED_CURVE ( )  B_SPLINE_CURVE ( 2, ( #24916, #38271, #35686, #11933, #28995, #5478, #1821 ),
 .UNSPECIFIED., .F., .F. ) 
 B_SPLINE_CURVE_WITH_KNOTS ( ( 3, 2, 2, 3 ),
 ( 0.3208955223880597396, 0.3221393034825871804, 0.3233830845771145657, 0.3246268656716419510 ),
 .UNSPECIFIED. ) 
 CURVE ( )  GEOMETRIC_REPRESENTATION_ITEM ( )  RATIONAL_B_SPLINE_CURVE ( ( 0.9999999999999940048, 0.8660254037844447028, 1.000000000000000000, 0.8660254037844387076, 1.000000000000000000, 0.8660254037844207220, 1.000000000000017986 ) ) 
 REPRESENTATION_ITEM ( '' )  );
#30197=ADVANCED_FACE ( 'NONE', ( #6782 ), #30099, .T. ) ;
#30198=CARTESIAN_POINT ( 'NONE',  ( -10.00000000000000000, -5.773502691896251982, -190.1250000000000284 ) ) ;
#30200=CARTESIAN_POINT ( 'NONE',  ( 7.644554776091147741E-16, 12.48450537969573659, -118.1562500020483952 ) ) ;
#30204=ORIENTED_EDGE ( 'NONE', *, *, #36000, .T. ) ;
#30205=CARTESIAN_POINT ( 'NONE',  ( 5.405949406249999534, 9.363379034771803333, -43.28125000204838102 ) ) ;
#30207=CARTESIAN_POINT ( 'NONE',  ( 10.81189881249999551, -6.242252689847874514, -98.96875000204838102 ) ) ;
#30208=CARTESIAN_POINT ( 'NONE',  ( 10.81189881249999551, -6.242252689847874514, -120.1562500020483952 ) ) ;
#30209=ORIENTED_EDGE ( 'NONE', *, *, #31375, .F. ) ;
#30211=CARTESIAN_POINT ( 'NONE',  ( -9.999999999999998224, 1.224646799147353059E-15, -118.2500000000000000 ) ) ;
#30212=CARTESIAN_POINT ( 'NONE',  ( -5.405949406249996869, 9.363379034771805109, -198.8437500020484094 ) ) ;
#30214=CARTESIAN_POINT ( 'NONE',  ( -4.999999999999996447, 8.660254037844387298, -13.87500000409674961 ) ) ;
#30215=CARTESIAN_POINT ( 'NONE',  ( -5.405949406249996869, 9.363379034771805109, -134.3437500020484094 ) ) ;
#30219=CARTESIAN_POINT ( 'NONE',  ( 4.999999999999992006, -8.660254037844389075, -188.6250000040967905 ) ) ;
#30221=CARTESIAN_POINT ( 'NONE',  ( -10.81189881249999729, -6.242252689847864744, -176.1562500020484094 ) ) ;
#30222=CARTESIAN_POINT ( 'NONE',  ( 10.00000000000076916, -5.773502691895816774, -107.1249999999999574 ) ) ;
#30225=CARTESIAN_POINT ( 'NONE',  ( 10.81189881249999729, 0.000000000000000000, -59.84375000204835970 ) ) ;
#30226=CARTESIAN_POINT ( 'NONE',  ( -5.405949406249996869, 9.363379034771805109, -44.34375000204837391 ) ) ;
#30228=CARTESIAN_POINT ( 'NONE',  ( 10.81189881249999907, 6.242252689847868297, -16.40625000204838102 ) ) ;
#30232=CARTESIAN_POINT ( 'NONE',  ( 7.070501591499377789E-16, 11.54700538379251284, -108.1249999999999716 ) ) ;
#30234=AXIS2_PLACEMENT_3D ( 'NONE', #10600, #7383, #20530 ) ;
#30235=CARTESIAN_POINT ( 'NONE',  ( 9.999999999999998224, 0.000000000000000000, -164.0000000000000000 ) ) ;
#30238=CARTESIAN_POINT ( 'NONE',  ( 10.81189881249999551, -6.242252689847874514, -109.6562500020483810 ) ) ;
#30239=ORIENTED_EDGE ( 'NONE', *, *, #24757, .F. ) ;
#30240=DIRECTION ( 'NONE',  ( 1.000000000000000000, 0.000000000000000000, 0.000000000000000000 ) ) ;
#30245=CARTESIAN_POINT ( 'NONE',  ( 10.00000000000000000, 5.773502691896255534, -36.37499999999996447 ) ) ;
#30247=CARTESIAN_POINT ( 'NONE',  ( -10.81189881249999729, -6.242252689847864744, -39.65625000204835970 ) ) ;
#30248=CARTESIAN_POINT ( 'NONE',  ( 9.999999999999998224, 0.000000000000000000, -132.8750000040967905 ) ) ;
#30250=LINE ( 'NONE', #1907, #28680 ) ;
#30251=CARTESIAN_POINT ( 'NONE',  ( 7.644554776091147741E-16, 12.48450537969573659, -139.1562500020483810 ) ) ;
#30252=CARTESIAN_POINT ( 'NONE',  ( -10.00000000000012434, 5.773502691896184480, -162.2500000040967905 ) ) ;
#30253=ORIENTED_EDGE ( 'NONE', *, *, #13888, .F. ) ;
#30256=CARTESIAN_POINT ( 'NONE',  ( 9.999999999999227285, 5.773502691896701400, -108.3749999999999289 ) ) ;
#30257=DIRECTION ( 'NONE',  ( 1.000000000000000000, 0.000000000000000000, 0.000000000000000000 ) ) ;
#30258=CARTESIAN_POINT ( 'NONE',  ( 10.81189881249999551, -6.242252689847874514, -167.9687500020483810 ) ) ;
#30260=CARTESIAN_POINT ( 'NONE',  ( 10.81189881249999907, 6.242252689847868297, -16.21875000204836326 ) ) ;
#30261=CARTESIAN_POINT ( 'NONE',  ( -9.999999999999998224, 1.224646799147353059E-15, -170.7500000000000000 ) ) ;
#30262=CARTESIAN_POINT ( 'NONE',  ( 5.405949406249999534, 9.363379034771803333, -157.0937500020483810 ) ) ;
#30263=CARTESIAN_POINT ( 'NONE',  ( -10.81189881249999729, 1.324075727343319199E-15, -138.5937500020483810 ) ) ;
#30264=CARTESIAN_POINT ( 'NONE',  ( 5.000000000000000000, 8.660254037844385522, -67.74999999999997158 ) ) ;
#30268=CARTESIAN_POINT ( 'NONE',  ( 7.644554776091147741E-16, 12.48450537969573659, -8.468750002048357928 ) ) ;
#30270=DIRECTION ( 'NONE',  ( -0.000000000000000000, -0.000000000000000000, 1.000000000000000000 ) ) ;
#30271=VECTOR ( 'NONE', #18628, 1000.000000000000000 ) ;
#30272=CARTESIAN_POINT ( 'NONE',  ( -10.00000000000051337, 5.773502691895962435, -124.7500000040967620 ) ) ;
#30275=CARTESIAN_POINT ( 'NONE',  ( -2.293366432827344421E-15, -12.48450537969573659, -82.71875000204838102 ) ) ;
#30276=CARTESIAN_POINT ( 'NONE',  ( 10.81189881249999729, 0.000000000000000000, -64.34375000204836681 ) ) ;
#30277=CARTESIAN_POINT ( 'NONE',  ( 9.999999999999998224, 0.000000000000000000, -116.3750000040967905 ) ) ;
#30278=CARTESIAN_POINT ( 'NONE',  ( -10.81189881249999729, 6.242252689847871849, -42.90625000204838102 ) ) ;
#30282=CARTESIAN_POINT ( 'NONE',  ( -5.000000000000003553, -8.660254037844383745, -131.5000000000000000 ) ) ;
#30283=CARTESIAN_POINT ( 'NONE',  ( 5.405949406249992428, -9.363379034771808662, -138.2812500020483810 ) ) ;
#30284=DIRECTION ( 'NONE',  ( 1.000000000000000000, 0.000000000000000000, -0.000000000000000000 ) ) ;
#30286=CARTESIAN_POINT ( 'NONE',  ( -10.81189881249999729, 1.324075727343319199E-15, -18.78125000204835970 ) ) ;
#30290=CARTESIAN_POINT ( 'NONE',  ( -9.999999999999998224, 1.224646799147353059E-15, -142.2500000000000000 ) ) ;
#30292=CARTESIAN_POINT ( 'NONE',  ( 7.070501591499377789E-16, 11.54700538379251284, -45.50000000409676915 ) ) ;
#30295=CARTESIAN_POINT ( 'NONE',  ( -5.000000000000003553, -8.660254037844383745, -191.5000000000000000 ) ) ;
#30296=CARTESIAN_POINT ( 'NONE',  ( -10.81189881249999907, -6.242252689847864744, -156.6562500020483810 ) ) ;
#30297=VECTOR ( 'NONE', #8532, 1000.000000000000000 ) ;
#30298=CARTESIAN_POINT ( 'NONE',  ( 5.405949406249999534, 9.363379034771803333, -133.0937500020483810 ) ) ;
#30299=CARTESIAN_POINT ( 'NONE',  ( -9.999999999999479527, -5.773502691896549521, -115.5000000040967763 ) ) ;
#30301=DIRECTION ( 'NONE',  ( -0.000000000000000000, -0.000000000000000000, 1.000000000000000000 ) ) ;
#30304=CARTESIAN_POINT ( 'NONE',  ( 10.81189881249999551, -6.242252689847874514, -64.65625000204839523 ) ) ;
#30305=ORIENTED_EDGE ( 'NONE', *, *, #15852, .T. ) ;
#30307=CARTESIAN_POINT ( 'NONE',  ( -2.293366432827344421E-15, -12.48450537969573659, -111.2187500020483668 ) ) ;
#30309=( BOUNDED_CURVE ( )  B_SPLINE_CURVE ( 2, ( #35348, #42216, #41793, #12644, #25836, #5776, #3171 ),
 .UNSPECIFIED., .F., .F. ) 
 B_SPLINE_CURVE_WITH_KNOTS ( ( 3, 2, 2, 3 ),
 ( 0.4365671641791046276, 0.4378109452736320129, 0.4390547263681593981, 0.4402985074626867279 ),
 .UNSPECIFIED. ) 
 CURVE ( )  GEOMETRIC_REPRESENTATION_ITEM ( )  RATIONAL_B_SPLINE_CURVE ( ( 0.9999999999999820144, 0.8660254037844566932, 1.000000000000000000, 0.8660254037844387076, 1.000000000000000000, 0.8660254037844207220, 1.000000000000017986 ) ) 
 REPRESENTATION_ITEM ( '' )  );
#30310=CARTESIAN_POINT ( 'NONE',  ( 7.644554776091147741E-16, 12.48450537969573659, -21.96875000204837036 ) ) ;
#30311=CARTESIAN_POINT ( 'NONE',  ( -5.405949406249996869, 9.363379034771805109, -191.3437500020484094 ) ) ;
#30312=CARTESIAN_POINT ( 'NONE',  ( 5.405949406249992428, -9.363379034771808662, -46.59375000204838102 ) ) ;
#30313=CARTESIAN_POINT ( 'NONE',  ( -0.02412132759690014186, -10.44061561015125505, -5.090678961559005602E-15 ) ) ;
#30314=CARTESIAN_POINT ( 'NONE',  ( 7.070501591499376803E-16, 11.54700538379251284, -152.0000000040967905 ) ) ;
#30315=CARTESIAN_POINT ( 'NONE',  ( 10.81189881249999729, 6.242252689847867408, -181.2187500020484094 ) ) ;
#30316=CARTESIAN_POINT ( 'NONE',  ( -10.81189881249999907, -6.242252689847864744, -159.4687500020484094 ) ) ;
#30319=DIRECTION ( 'NONE',  ( 1.000000000000000000, 0.000000000000000000, 0.000000000000000000 ) ) ;
#30324=CARTESIAN_POINT ( 'NONE',  ( -5.405949406249996869, 9.363379034771805109, -89.34375000204838102 ) ) ;
#30325=EDGE_CURVE ( 'NONE', #18400, #33859, #20745, .T. ) ;
#30326=CARTESIAN_POINT ( 'NONE',  ( -5.000000000000003553, -8.660254037844383745, -101.5000000000000000 ) ) ;
#30327=CARTESIAN_POINT ( 'NONE',  ( -10.81189881249999729, 1.324075727343319199E-15, -66.78125000204838102 ) ) ;
#30330=CARTESIAN_POINT ( 'NONE',  ( 5.405949406249992428, -9.363379034771808662, -121.7812500020483952 ) ) ;
#30331=CARTESIAN_POINT ( 'NONE',  ( 5.405949406249992428, -9.363379034771808662, -165.2812500020484094 ) ) ;
#30333=CARTESIAN_POINT ( 'NONE',  ( -4.999999999999996447, 8.660254037844387298, -136.8750000040967905 ) ) ;
#30335=EDGE_CURVE ( 'NONE', #317, #2293, #5617, .T. ) ;
#30336=ORIENTED_EDGE ( 'NONE', *, *, #29272, .T. ) ;
#30339=CARTESIAN_POINT ( 'NONE',  ( -5.405949406250003975, -9.363379034771801557, -189.5312500020484094 ) ) ;
#30341=ORIENTED_EDGE ( 'NONE', *, *, #9425, .T. ) ;
#30342=CARTESIAN_POINT ( 'NONE',  ( 7.070501591499377789E-16, 11.54700538379251284, -48.12499999999997158 ) ) ;
#30344=CARTESIAN_POINT ( 'NONE',  ( 4.999999999999992006, -8.660254037844389075, -62.62500000409676204 ) ) ;
#30346=CARTESIAN_POINT ( 'NONE',  ( 9.999999999999998224, 0.000000000000000000, -165.5000000000000000 ) ) ;
#30348=CARTESIAN_POINT ( 'NONE',  ( 10.81189881249999729, 6.242252689847867408, -62.90625000204838813 ) ) ;
#30351=CARTESIAN_POINT ( 'NONE',  ( -9.999999999999998224, 1.224646799147353059E-15, -132.1250000040967620 ) ) ;
#30352=CARTESIAN_POINT ( 'NONE',  ( -10.81189881249999729, 1.324075727343319199E-15, -179.2812500020484094 ) ) ;
#30354=CARTESIAN_POINT ( 'NONE',  ( -9.999999999999998224, 1.224646799147353059E-15, -147.1250000040967905 ) ) ;
#30357=CARTESIAN_POINT ( 'NONE',  ( 0.000000000000000000, 0.000000000000000000, -200.0000000000000000 ) ) ;
#30359=CARTESIAN_POINT ( 'NONE',  ( 10.81189881249999907, 6.242252689847868297, -86.90625000204836681 ) ) ;
#30360=VERTEX_POINT ( 'NONE', #17326 ) ;
#30361=CARTESIAN_POINT ( 'NONE',  ( 9.999999999999227285, 5.773502691896701400, -107.2500000040967620 ) ) ;
#30362=EDGE_CURVE ( 'NONE', #6831, #22759, #40616, .T. ) ;
#30364=EDGE_LOOP ( 'NONE', ( #22855, #13336, #19125, #36531 ) ) ;
#30365=VERTEX_POINT ( 'NONE', #30529 ) ;
#30366=CARTESIAN_POINT ( 'NONE',  ( -10.81189881249999907, -6.242252689847864744, -27.46875000204838457 ) ) ;
#30367=CARTESIAN_POINT ( 'NONE',  ( 7.644554776091147741E-16, 12.48450537969573659, -25.15625000204838457 ) ) ;
#30369=CARTESIAN_POINT ( 'NONE',  ( -5.405949406250003975, -9.363379034771801557, -67.84375000204836681 ) ) ;
#30370=CARTESIAN_POINT ( 'NONE',  ( 10.00000000000102318, -5.773502691895667560, -17.50000000409673362 ) ) ;
#30372=CARTESIAN_POINT ( 'NONE',  ( -5.405949406249996869, 9.363379034771805109, -182.3437500020483810 ) ) ;
#30373=CARTESIAN_POINT ( 'NONE',  ( 9.999999999999998224, 0.000000000000000000, -25.99999999999996803 ) ) ;
#30374=CYLINDRICAL_SURFACE ( 'NONE', #2631, 9.999999999999998224 ) ;
#30375=CARTESIAN_POINT ( 'NONE',  ( -9.999999999999998224, 1.224646799147353059E-15, -70.62500000409677625 ) ) ;
#30376=CARTESIAN_POINT ( 'NONE',  ( -5.000000000000003553, -8.660254037844383745, -5.875000004096770034 ) ) ;
#30377=DIRECTION ( 'NONE',  ( 1.000000000000000000, 0.000000000000000000, 0.000000000000000000 ) ) ;
#30378=CARTESIAN_POINT ( 'NONE',  ( 10.81189881249999907, 6.242252689847868297, -118.2187500020483810 ) ) ;
#30379=CARTESIAN_POINT ( 'NONE',  ( -10.00000000000051337, 5.773502691895962435, -109.3749999999999858 ) ) ;
#30380=CARTESIAN_POINT ( 'NONE',  ( 5.405949406249992428, -9.363379034771808662, -90.28125000204838102 ) ) ;
#30381=CARTESIAN_POINT ( 'NONE',  ( -2.293366432827344421E-15, -12.48450537969573659, -103.7187500020483668 ) ) ;
#30384=CARTESIAN_POINT ( 'NONE',  ( 4.999999999999992006, -8.660254037844389075, -160.1250000040967905 ) ) ;
#30387=AXIS2_PLACEMENT_3D ( 'NONE', #37945, #15043, #1700 ) ;
#30389=LINE ( 'NONE', #23696, #9576 ) ;
#30391=CARTESIAN_POINT ( 'NONE',  ( -10.00000000000025580, 5.773502691896109873, -120.2500000040967905 ) ) ;
#30392=CARTESIAN_POINT ( 'NONE',  ( 7.070501591499377789E-16, 11.54700538379251284, -76.62499999999997158 ) ) ;
#30394=CARTESIAN_POINT ( 'NONE',  ( -10.00000000000000000, -5.773502691896251982, -90.00000000409677625 ) ) ;
#30395=VECTOR ( 'NONE', #39559, 1000.000000000000114 ) ;
#30396=FACE_OUTER_BOUND ( 'NONE', #5950, .T. ) ;
#30398=CARTESIAN_POINT ( 'NONE',  ( -10.81189881249999729, 6.242252689847871849, -83.40625000204838102 ) ) ;
#30400=CARTESIAN_POINT ( 'NONE',  ( -9.999999999999998224, 1.224646799147353059E-15, -20.74999999999996447 ) ) ;
#30402=ORIENTED_EDGE ( 'NONE', *, *, #8296, .F. ) ;
#30403=CARTESIAN_POINT ( 'NONE',  ( -9.999999999999998224, 5.773502691896259087, -7.374999999999970690 ) ) ;
#30405=CARTESIAN_POINT ( 'NONE',  ( 9.999999999999996447, -5.773502691896262640, -143.1250000000000000 ) ) ;
#30406=DIRECTION ( 'NONE',  ( 1.000000000000000000, 0.000000000000000000, 0.000000000000000000 ) ) ;
#30409=CARTESIAN_POINT ( 'NONE',  ( 10.81189881249999551, -6.242252689847874514, -135.1562500020484094 ) ) ;
#30410=CARTESIAN_POINT ( 'NONE',  ( -10.00000000000000000, -5.773502691896251982, -188.6250000000000284 ) ) ;
#30411=FACE_OUTER_BOUND ( 'NONE', #5738, .T. ) ;
#30412=CARTESIAN_POINT ( 'NONE',  ( -5.405949406249996869, 9.363379034771805109, -107.5312500020483810 ) ) ;
#30414=CARTESIAN_POINT ( 'NONE',  ( -9.999999999999998224, 1.224646799147353059E-15, -36.12500000409676915 ) ) ;
#30415=ADVANCED_FACE ( 'NONE', ( #12344 ), #38476, .T. ) ;
#30417=EDGE_CURVE ( 'NONE', #19501, #36017, #18840, .T. ) ;
#30418=ORIENTED_EDGE ( 'NONE', *, *, #2764, .T. ) ;
#30419=VECTOR ( 'NONE', #477, 1000.000000000000000 ) ;
#30420=CARTESIAN_POINT ( 'NONE',  ( -2.293366432827344421E-15, -12.48450537969573659, -45.40625000204837391 ) ) ;
#30422=CARTESIAN_POINT ( 'NONE',  ( -5.405949406250003975, -9.363379034771801557, -94.84375000204838102 ) ) ;
#30423=CARTESIAN_POINT ( 'NONE',  ( 10.81189881249999729, 6.242252689847867408, -125.9062500020483810 ) ) ;
#30424=ORIENTED_EDGE ( 'NONE', *, *, #3091, .T. ) ;
#30425=CARTESIAN_POINT ( 'NONE',  ( 9.999999999999994671, -5.773502691896262640, -132.6250000000000000 ) ) ;
#30426=CARTESIAN_POINT ( 'NONE',  ( 7.644554776091147741E-16, 12.48450537969573659, -195.9687500020484094 ) ) ;
#30428=CYLINDRICAL_SURFACE ( 'NONE', #35711, 9.999999999999998224 ) ;
#30430=CARTESIAN_POINT ( 'NONE',  ( 5.405949406249999534, 9.363379034771803333, -124.0937500020483952 ) ) ;
#30432=DIRECTION ( 'NONE',  ( -0.000000000000000000, -0.000000000000000000, 1.000000000000000000 ) ) ;
#30434=CARTESIAN_POINT ( 'NONE',  ( -10.00000000000000000, -5.773502691896251982, -187.5000000040967905 ) ) ;
#30436=CARTESIAN_POINT ( 'NONE',  ( 10.81189881249999729, 6.242252689847867408, -176.9062500020484094 ) ) ;
#30439=CARTESIAN_POINT ( 'NONE',  ( 10.81189881249999729, 0.000000000000000000, -50.84375000204835260 ) ) ;
#30440=CARTESIAN_POINT ( 'NONE',  ( 10.81189881249999551, -6.242252689847874514, -43.46875000204836681 ) ) ;
#30442=CARTESIAN_POINT ( 'NONE',  ( 5.405949406249999534, 9.363379034771803333, -7.281250002048378356 ) ) ;
#30446=CARTESIAN_POINT ( 'NONE',  ( -2.121150477449813534E-15, -11.54700538379251284, -102.8749999999999858 ) ) ;
#30449=LINE ( 'NONE', #20495, #42393 ) ;
#30452=CARTESIAN_POINT ( 'NONE',  ( 7.644554776091147741E-16, 12.48450537969573659, -106.1562500020483810 ) ) ;
#30453=VERTEX_POINT ( 'NONE', #2027 ) ;
#30454=AXIS2_PLACEMENT_3D ( 'NONE', #15330, #37795, #38012 ) ;
#30455=( BOUNDED_CURVE ( )  B_SPLINE_CURVE ( 2, ( #19570, #26696, #176, #36615, #13081, #805, #16745 ),
 .UNSPECIFIED., .F., .F. ) 
 B_SPLINE_CURVE_WITH_KNOTS ( ( 3, 2, 2, 3 ),
 ( 0.5000000000000001110, 0.5012437810945274963, 0.5024875621890548816, 0.5037313432835821558 ),
 .UNSPECIFIED. ) 
 CURVE ( )  GEOMETRIC_REPRESENTATION_ITEM ( )  RATIONAL_B_SPLINE_CURVE ( ( 0.9999999999999880096, 0.8660254037844506980, 1.000000000000000000, 0.8660254037844387076, 1.000000000000000000, 0.8660254037844267172, 1.000000000000011990 ) ) 
 REPRESENTATION_ITEM ( '' )  );
#30456=CARTESIAN_POINT ( 'NONE',  ( -5.000000000000003553, -8.660254037844383745, -6.999999999999978684 ) ) ;
#30458=DIRECTION ( 'NONE',  ( -0.000000000000000000, -0.000000000000000000, 1.000000000000000000 ) ) ;
#30460=ORIENTED_EDGE ( 'NONE', *, *, #30112, .F. ) ;
#30461=CARTESIAN_POINT ( 'NONE',  ( -5.000000000000003553, -8.660254037844383745, -30.99999999999997158 ) ) ;
#30463=CARTESIAN_POINT ( 'NONE',  ( 5.405949406249999534, 9.363379034771803333, -35.78125000204837391 ) ) ;
#30464=CARTESIAN_POINT ( 'NONE',  ( -5.000000000000003553, -8.660254037844383745, -90.99999999999998579 ) ) ;
#30466=DIRECTION ( 'NONE',  ( -0.000000000000000000, -0.000000000000000000, 1.000000000000000000 ) ) ;
#30467=AXIS2_PLACEMENT_3D ( 'NONE', #12706, #3026, #19831 ) ;
#30468=CARTESIAN_POINT ( 'NONE',  ( -10.81189881249999907, -6.242252689847864744, -138.6562500020484094 ) ) ;
#30469=CARTESIAN_POINT ( 'NONE',  ( -2.121150477449813534E-15, -11.54700538379251284, -119.7500000040967905 ) ) ;
#30470=VERTEX_POINT ( 'NONE', #9127 ) ;
#30471=EDGE_CURVE ( 'NONE', #31040, #9902, #9997, .T. ) ;
#30472=ADVANCED_FACE ( 'NONE', ( #35257 ), #25331, .T. ) ;
#30474=CARTESIAN_POINT ( 'NONE',  ( 4.999999999999992006, -8.660254037844389075, -106.1250000040967763 ) ) ;
#30475=DIRECTION ( 'NONE',  ( 1.000000000000000000, 0.000000000000000000, 0.000000000000000000 ) ) ;
#30476=CARTESIAN_POINT ( 'NONE',  ( 5.405949406249999534, 9.363379034771803333, -164.5937500020484094 ) ) ;
#30478=CARTESIAN_POINT ( 'NONE',  ( 7.644554776091147741E-16, 12.48450537969573659, -17.46875000204836681 ) ) ;
#30479=CARTESIAN_POINT ( 'NONE',  ( -2.121150477449813534E-15, -11.54700538379251284, -157.2500000040968189 ) ) ;
#30480=CARTESIAN_POINT ( 'NONE',  ( -10.81189881249999729, -6.242252689847864744, -144.4687500020484094 ) ) ;
#30481=CARTESIAN_POINT ( 'NONE',  ( 7.644554776091147741E-16, 12.48450537969573659, -134.4687500020483810 ) ) ;
#30482=CARTESIAN_POINT ( 'NONE',  ( -10.81189881249999907, -6.242252689847864744, -110.1562500020483952 ) ) ;
#30486=CARTESIAN_POINT ( 'NONE',  ( -5.405949406250003975, -9.363379034771801557, -13.84375000204834905 ) ) ;
#30488=EDGE_CURVE ( 'NONE', #8277, #42072, #15787, .T. ) ;
#30490=CARTESIAN_POINT ( 'NONE',  ( 4.999999999999992006, -8.660254037844389075, -96.74999999999998579 ) ) ;
#30494=CARTESIAN_POINT ( 'NONE',  ( 10.81189881249999551, -6.242252689847874514, -82.46875000204836681 ) ) ;
#30495=CARTESIAN_POINT ( 'NONE',  ( 5.405949406249992428, -9.363379034771808662, -63.09375000204836681 ) ) ;
#30497=CARTESIAN_POINT ( 'NONE',  ( 10.81189881249999729, 0.000000000000000000, -39.03125000204838102 ) ) ;
#30501=CARTESIAN_POINT ( 'NONE',  ( -5.000000000000003553, -8.660254037844383745, -128.5000000000000000 ) ) ;
#30502=CARTESIAN_POINT ( 'NONE',  ( -10.81189881249999729, 6.242252689847871849, -128.4062500020483810 ) ) ;
#30505=CARTESIAN_POINT ( 'NONE',  ( -10.81189881249999729, 6.242252689847871849, -18.90625000204837391 ) ) ;
#30506=ORIENTED_EDGE ( 'NONE', *, *, #22815, .T. ) ;
#30510=CARTESIAN_POINT ( 'NONE',  ( 10.00000000000000000, 5.773502691896255534, -35.25000000409675494 ) ) ;
#30513=AXIS2_PLACEMENT_3D ( 'NONE', #21761, #21968, #34939 ) ;
#30514=CARTESIAN_POINT ( 'NONE',  ( 5.000000000000000000, 8.660254037844385522, -76.74999999999998579 ) ) ;
#30515=CARTESIAN_POINT ( 'NONE',  ( 10.81189881249999729, 0.000000000000000000, -153.0312500020484094 ) ) ;
#30516=CARTESIAN_POINT ( 'NONE',  ( 10.81189881249999907, 6.242252689847868297, -131.7187500020483810 ) ) ;
#30517=CARTESIAN_POINT ( 'NONE',  ( -9.999999999999998224, 1.224646799147353059E-15, -143.7500000000000000 ) ) ;
#30518=VERTEX_POINT ( 'NONE', #15156 ) ;
#30519=CARTESIAN_POINT ( 'NONE',  ( 9.999999999999998224, 0.000000000000000000, -15.87500000409675138 ) ) ;
#30520=ORIENTED_EDGE ( 'NONE', *, *, #10764, .F. ) ;
#30523=CARTESIAN_POINT ( 'NONE',  ( -5.405949406249996869, 9.363379034771805109, -110.3437500020483810 ) ) ;
#30524=ORIENTED_EDGE ( 'NONE', *, *, #28347, .F. ) ;
#30526=CARTESIAN_POINT ( 'NONE',  ( -2.293366432827344421E-15, -12.48450537969573659, -190.7187500020484094 ) ) ;
#30527=CARTESIAN_POINT ( 'NONE',  ( -5.405949406249996869, 9.363379034771805109, -42.84375000204837391 ) ) ;
#30528=EDGE_CURVE ( 'NONE', #5068, #28118, #2448, .T. ) ;
#30529=CARTESIAN_POINT ( 'NONE',  ( -9.999999999999998224, 1.224646799147353059E-15, -94.62500000409677625 ) ) ;
#30530=CARTESIAN_POINT ( 'NONE',  ( -2.121150477449813534E-15, -11.54700538379251284, -31.25000000409674783 ) ) ;
#30531=CARTESIAN_POINT ( 'NONE',  ( 5.405949406249992428, -9.363379034771808662, -181.5937500020483810 ) ) ;
#30532=CARTESIAN_POINT ( 'NONE',  ( -2.293366432827344421E-15, -12.48450537969573659, -159.2187500020483810 ) ) ;
#30533=CARTESIAN_POINT ( 'NONE',  ( -9.999999999999479527, -5.773502691896549521, -123.0000000040967763 ) ) ;
#30536=CARTESIAN_POINT ( 'NONE',  ( -10.00000000000076916, 5.773502691895813221, -133.7500000040967905 ) ) ;
#30537=CARTESIAN_POINT ( 'NONE',  ( 7.070501591499376803E-16, 11.54700538379251284, -36.12499999999996447 ) ) ;
#30539=CARTESIAN_POINT ( 'NONE',  ( -10.81189881249999729, 6.242252689847871849, -87.71875000204838102 ) ) ;
#30541=CARTESIAN_POINT ( 'NONE',  ( -10.81189881249999729, 6.242252689847871849, -63.90625000204836681 ) ) ;
#30543=CARTESIAN_POINT ( 'NONE',  ( 10.81189881249999729, 0.000000000000000000, -121.5312500020483952 ) ) ;
#30544=CARTESIAN_POINT ( 'NONE',  ( 10.81189881249999729, 6.242252689847867408, -157.4062500020483810 ) ) ;
#30546=CARTESIAN_POINT ( 'NONE',  ( -4.999999999999996447, 8.660254037844387298, -133.8750000040967905 ) ) ;
#30548=EDGE_CURVE ( 'NONE', #14006, #30625, #8710, .T. ) ;
#30549=EDGE_LOOP ( 'NONE', ( #9224, #20348, #31479, #22713 ) ) ;
#30553=CARTESIAN_POINT ( 'NONE',  ( -5.405949406250003975, -9.363379034771801557, -185.0312500020484094 ) ) ;
#30555=ORIENTED_EDGE ( 'NONE', *, *, #4854, .T. ) ;
#30556=CARTESIAN_POINT ( 'NONE',  ( 4.999999999999992006, -8.660254037844389075, -47.24999999999998579 ) ) ;
#30558=CARTESIAN_POINT ( 'NONE',  ( 5.000000000000000000, 8.660254037844385522, -57.62500000409676204 ) ) ;
#30560=CARTESIAN_POINT ( 'NONE',  ( 5.405949406249992428, -9.363379034771808662, -61.78125000204837391 ) ) ;
#30563=DIRECTION ( 'NONE',  ( -0.000000000000000000, -0.000000000000000000, 1.000000000000000000 ) ) ;
#30564=CARTESIAN_POINT ( 'NONE',  ( -5.405949406250003975, -9.363379034771801557, -174.5312500020484094 ) ) ;
#30566=CARTESIAN_POINT ( 'NONE',  ( -9.999999999999998224, 1.224646799147353059E-15, -73.62500000409677625 ) ) ;
#30567=CARTESIAN_POINT ( 'NONE',  ( -9.999999999999998224, 1.224646799147353059E-15, -67.62500000409676204 ) ) ;
#30570=FACE_OUTER_BOUND ( 'NONE', #19909, .T. ) ;
#30571=CARTESIAN_POINT ( 'NONE',  ( -10.81189881249999729, 1.324075727343319199E-15, -84.78125000204838102 ) ) ;
#30573=CARTESIAN_POINT ( 'NONE',  ( 5.000000000000000000, 8.660254037844385522, -81.24999999999998579 ) ) ;
#30574=VERTEX_POINT ( 'NONE', #15581 ) ;
#30575=ORIENTED_EDGE ( 'NONE', *, *, #41499, .F. ) ;
#30576=EDGE_CURVE ( 'NONE', #14677, #21458, #8393, .T. ) ;
#30577=CARTESIAN_POINT ( 'NONE',  ( 10.81189881249999907, 6.242252689847868297, -26.71875000204838102 ) ) ;
#30578=CARTESIAN_POINT ( 'NONE',  ( 5.405949406249992428, -9.363379034771808662, -13.78125000204835615 ) ) ;
#30579=CARTESIAN_POINT ( 'NONE',  ( 5.405949406249999534, 9.363379034771803333, -64.09375000204836681 ) ) ;
#30582=CARTESIAN_POINT ( 'NONE',  ( -10.81189881249999907, -6.242252689847864744, -186.4687500020484094 ) ) ;
#30584=CARTESIAN_POINT ( 'NONE',  ( 9.999999999999479527, 5.773502691896553074, -175.8749999999999716 ) ) ;
#30585=CARTESIAN_POINT ( 'NONE',  ( -4.999999999999996447, 8.660254037844387298, -132.0000000000000000 ) ) ;
#30586=CARTESIAN_POINT ( 'NONE',  ( 5.000000000000000000, 8.660254037844385522, -71.12500000409677625 ) ) ;
#30588=CARTESIAN_POINT ( 'NONE',  ( 10.81189881249999907, 6.242252689847868297, -115.2187500020483810 ) ) ;
#30589=CARTESIAN_POINT ( 'NONE',  ( 9.999999999999998224, 0.000000000000000000, -63.49999999999997158 ) ) ;
#30590=CARTESIAN_POINT ( 'NONE',  ( -2.293366432827344421E-15, -12.48450537969573659, -88.90625000204838102 ) ) ;
#30591=CARTESIAN_POINT ( 'NONE',  ( -10.81189881249999729, 1.324075727343319199E-15, -101.0937500020483810 ) ) ;
#30595=CARTESIAN_POINT ( 'NONE',  ( 4.999999999999992006, -8.660254037844389075, -151.1250000040967905 ) ) ;
#30600=DIRECTION ( 'NONE',  ( -0.000000000000000000, -0.000000000000000000, 1.000000000000000000 ) ) ;
#30602=CARTESIAN_POINT ( 'NONE',  ( 9.999999999999998224, 0.000000000000000000, -176.0000000000000000 ) ) ;
#30603=CARTESIAN_POINT ( 'NONE',  ( 7.070501591499377789E-16, 11.54700538379251284, -75.12500000000000000 ) ) ;
#30605=CARTESIAN_POINT ( 'NONE',  ( -9.999999999999998224, 5.773502691896259087, -90.25000000409676204 ) ) ;
#30608=CARTESIAN_POINT ( 'NONE',  ( -10.81189881249999729, 6.242252689847871849, -81.90625000204839523 ) ) ;
#30610=CARTESIAN_POINT ( 'NONE',  ( 5.000000000000000000, 8.660254037844385522, -113.1250000040967763 ) ) ;
#30613=CARTESIAN_POINT ( 'NONE',  ( 5.000000000000000000, 8.660254037844385522, -3.249999999999975131 ) ) ;
#30615=CARTESIAN_POINT ( 'NONE',  ( 10.81189881249999729, 6.242252689847867408, -13.21875000204836326 ) ) ;
#30616=FACE_OUTER_BOUND ( 'NONE', #39157, .T. ) ;
#30618=CARTESIAN_POINT ( 'NONE',  ( -10.81189881249999729, 1.324075727343319199E-15, -128.2812500020483810 ) ) ;
#30619=CARTESIAN_POINT ( 'NONE',  ( 9.999999999999998224, 0.000000000000000000, -179.0000000000000000 ) ) ;
#30620=CARTESIAN_POINT ( 'NONE',  ( -9.999999999999678479, -5.773502691896439387, -184.5000000040968189 ) ) ;
#30621=CARTESIAN_POINT ( 'NONE',  ( -5.405949406250003975, -9.363379034771801557, -107.0312500020483810 ) ) ;
#30623=CYLINDRICAL_SURFACE ( 'NONE', #30387, 9.999999999999998224 ) ;
#30625=VERTEX_POINT ( 'NONE', #14940 ) ;
#30626=CARTESIAN_POINT ( 'NONE',  ( 5.405949406249999534, 9.363379034771803333, -34.28125000204837391 ) ) ;
#30628=CARTESIAN_POINT ( 'NONE',  ( -5.405949406250003975, -9.363379034771801557, -96.34375000204838102 ) ) ;
#30629=FACE_OUTER_BOUND ( 'NONE', #31400, .T. ) ;
#30631=CARTESIAN_POINT ( 'NONE',  ( 5.405949406249999534, 9.363379034771803333, -196.0937500020484094 ) ) ;
#30633=CARTESIAN_POINT ( 'NONE',  ( -2.121150477449813534E-15, -11.54700538379251284, -138.8750000000000000 ) ) ;
#30634=CARTESIAN_POINT ( 'NONE',  ( 7.644554776091147741E-16, 12.48450537969573659, -125.4687500020483952 ) ) ;
#30638=CARTESIAN_POINT ( 'NONE',  ( 10.00000000000000000, 5.773502691896255534, -188.2500000040968189 ) ) ;
#30640=CARTESIAN_POINT ( 'NONE',  ( 10.81189881249999551, -6.242252689847874514, -181.6562500020484379 ) ) ;
#30641=CARTESIAN_POINT ( 'NONE',  ( -9.999999999999998224, 1.224646799147353059E-15, -1.625000004096766038 ) ) ;
#30644=CARTESIAN_POINT ( 'NONE',  ( 10.81189881249999551, -6.242252689847874514, -49.46875000204835970 ) ) ;
#30645=CARTESIAN_POINT ( 'NONE',  ( 10.81189881249999729, 0.000000000000000000, -44.84375000204837391 ) ) ;
#30647=CARTESIAN_POINT ( 'NONE',  ( 10.81189881249999551, -6.242252689847874514, -9.156250002048375691 ) ) ;
#30649=CARTESIAN_POINT ( 'NONE',  ( 9.999999999999998224, 0.000000000000000000, -10.99999999999995381 ) ) ;
#30652=CARTESIAN_POINT ( 'NONE',  ( -9.999999999999998224, 1.224646799147353059E-15, -98.74999999999998579 ) ) ;
#30654=CARTESIAN_POINT ( 'NONE',  ( -9.999999999999998224, 5.773502691896259087, -111.2500000040967763 ) ) ;
#30660=CARTESIAN_POINT ( 'NONE',  ( 10.81189881249999729, 0.000000000000000000, -105.0312500020483810 ) ) ;
#30661=ORIENTED_EDGE ( 'NONE', *, *, #21376, .F. ) ;
#30662=LINE ( 'NONE', #22164, #41704 ) ;
#30667=CARTESIAN_POINT ( 'NONE',  ( 4.999999999999992006, -8.660254037844389075, -23.24999999999996447 ) ) ;
#30668=CARTESIAN_POINT ( 'NONE',  ( 5.405949406249999534, 9.363379034771803333, -38.78125000204838102 ) ) ;
#30669=CARTESIAN_POINT ( 'NONE',  ( 7.070501591499377789E-16, 11.54700538379251284, -163.6250000000000000 ) ) ;
#30670=CARTESIAN_POINT ( 'NONE',  ( -9.999999999999998224, 1.224646799147353059E-15, -103.2500000000000000 ) ) ;
#30672=CARTESIAN_POINT ( 'NONE',  ( -5.405949406249996869, 9.363379034771805109, -136.0312500020484094 ) ) ;
#30673=CARTESIAN_POINT ( 'NONE',  ( 7.070501591499376803E-16, 11.54700538379251284, -167.0000000040967905 ) ) ;
#30674=VERTEX_POINT ( 'NONE', #36302 ) ;
#30675=EDGE_LOOP ( 'NONE', ( #14962, #25097, #38157, #41246 ) ) ;
#30676=ORIENTED_EDGE ( 'NONE', *, *, #3288, .T. ) ;
#30679=CARTESIAN_POINT ( 'NONE',  ( -10.81189881249999907, -6.242252689847864744, -168.4687500020483526 ) ) ;
#30682=CARTESIAN_POINT ( 'NONE',  ( -10.81189881249999907, -6.242252689847864744, -13.96875000204836681 ) ) ;
#30684=CARTESIAN_POINT ( 'NONE',  ( -2.293366432827344421E-15, -12.48450537969573659, -148.7187500020484094 ) ) ;
#30685=CARTESIAN_POINT ( 'NONE',  ( -10.81189881249999907, -6.242252689847864744, -133.9687500020483810 ) ) ;
#30686=CARTESIAN_POINT ( 'NONE',  ( 5.405949406249999534, 9.363379034771803333, -106.2812500020483810 ) ) ;
#30690=CARTESIAN_POINT ( 'NONE',  ( 10.81189881249999907, 6.242252689847868297, -8.718750002048356151 ) ) ;
#30692=CARTESIAN_POINT ( 'NONE',  ( 10.81189881249999729, 0.000000000000000000, -199.5312500020484094 ) ) ;
#30693=( BOUNDED_CURVE ( )  B_SPLINE_CURVE ( 2, ( #7915, #40687, #11344, #14576, #30585, #41111, #14786 ),
 .UNSPECIFIED., .F., .F. ) 
 B_SPLINE_CURVE_WITH_KNOTS ( ( 3, 2, 2, 3 ),
 ( 0.3358208955223880854, 0.3370646766169154707, 0.3383084577114429670, 0.3395522388059703522 ),
 .UNSPECIFIED. ) 
 CURVE ( )  GEOMETRIC_REPRESENTATION_ITEM ( )  RATIONAL_B_SPLINE_CURVE ( ( 1.000000000000000000, 0.8660254037844387076, 1.000000000000000000, 0.8660254037844387076, 1.000000000000000000, 0.8660254037844148378, 1.000000000000023981 ) ) 
 REPRESENTATION_ITEM ( '' )  );
#30697=CARTESIAN_POINT ( 'NONE',  ( -2.293366432827344421E-15, -12.48450537969573659, -79.71875000204838102 ) ) ;
#30698=CARTESIAN_POINT ( 'NONE',  ( -5.405949406250003975, -9.363379034771801557, -61.84375000204836681 ) ) ;
#30699=CARTESIAN_POINT ( 'NONE',  ( -9.999999999999872102, -5.773502691896326589, -167.6250000000000000 ) ) ;
#30700=CARTESIAN_POINT ( 'NONE',  ( 5.405949406249992428, -9.363379034771808662, -33.28125000204837391 ) ) ;
#30702=DIRECTION ( 'NONE',  ( 1.000000000000000000, 0.000000000000000000, 0.000000000000000000 ) ) ;
#30704=EDGE_CURVE ( 'NONE', #18780, #12159, #25752, .T. ) ;
#30705=CARTESIAN_POINT ( 'NONE',  ( 9.999999999999998224, 0.000000000000000000, -123.5000000000000000 ) ) ;
#30706=CARTESIAN_POINT ( 'NONE',  ( -2.293366432827344421E-15, -12.48450537969573659, -132.4062500020483810 ) ) ;
#30710=CARTESIAN_POINT ( 'NONE',  ( -5.405949406250003975, -9.363379034771801557, -15.53125000204835793 ) ) ;
#30711=EDGE_CURVE ( 'NONE', #22759, #16098, #24657, .T. ) ;
#30712=ORIENTED_EDGE ( 'NONE', *, *, #29653, .T. ) ;
#30713=( BOUNDED_CURVE ( )  B_SPLINE_CURVE ( 2, ( #6248, #2168, #15506, #35395, #5819, #15303, #38405 ),
 .UNSPECIFIED., .F., .F. ) 
 B_SPLINE_CURVE_WITH_KNOTS ( ( 3, 2, 2, 3 ),
 ( 0.6343283582089553896, 0.6355721393034826638, 0.6368159203980100491, 0.6380597014925374344 ),
 .UNSPECIFIED. ) 
 CURVE ( )  GEOMETRIC_REPRESENTATION_ITEM ( )  RATIONAL_B_SPLINE_CURVE ( ( 0.9999999999999880096, 0.8660254037844506980, 1.000000000000000000, 0.8660254037844387076, 1.000000000000000000, 0.8660254037844267172, 1.000000000000011990 ) ) 
 REPRESENTATION_ITEM ( '' )  );
#30716=CARTESIAN_POINT ( 'NONE',  ( 7.070501591499376803E-16, 11.54700538379251284, -9.124999999999978684 ) ) ;
#30717=EDGE_CURVE ( 'NONE', #6996, #37716, #26278, .T. ) ;
#30718=CARTESIAN_POINT ( 'NONE',  ( -9.999999999999998224, 5.773502691896259087, -33.25000000409676204 ) ) ;
#30719=CARTESIAN_POINT ( 'NONE',  ( -9.999999999999998224, 1.224646799147353059E-15, -200.0000000000000000 ) ) ;
#30722=CARTESIAN_POINT ( 'NONE',  ( 0.000000000000000000, 0.000000000000000000, -200.0000000000000000 ) ) ;
#30723=CARTESIAN_POINT ( 'NONE',  ( -2.293366432827344421E-15, -12.48450537969573659, -153.4062500020483810 ) ) ;
#30724=CARTESIAN_POINT ( 'NONE',  ( -10.81189881249999729, 1.324075727343319199E-15, -123.5937500020483952 ) ) ;
#30726=EDGE_LOOP ( 'NONE', ( #29812, #3815, #24583, #37568 ) ) ;
#30729=EDGE_CURVE ( 'NONE', #20886, #12962, #12765, .T. ) ;
#30730=VERTEX_POINT ( 'NONE', #6523 ) ;
#30731=CARTESIAN_POINT ( 'NONE',  ( -5.405949406249996869, 9.363379034771805109, -111.8437500020483810 ) ) ;
#30732=ORIENTED_EDGE ( 'NONE', *, *, #9216, .F. ) ;
#30733=CARTESIAN_POINT ( 'NONE',  ( 10.81189881249999907, 6.242252689847868297, -187.2187500020484094 ) ) ;
#30734=CARTESIAN_POINT ( 'NONE',  ( 7.644554776091147741E-16, 12.48450537969573659, -39.96875000204835970 ) ) ;
#30735=CARTESIAN_POINT ( 'NONE',  ( -9.999999999999742428, -5.773502691896402084, -156.0000000040968473 ) ) ;
#30736=CARTESIAN_POINT ( 'NONE',  ( -2.121150477449813534E-15, -11.54700538379251284, -10.25000000409676026 ) ) ;
#30737=CARTESIAN_POINT ( 'NONE',  ( -2.293366432827344421E-15, -12.48450537969573659, -174.2187500020483810 ) ) ;
#30738=AXIS2_PLACEMENT_3D ( 'NONE', #13177, #22493, #6100 ) ;
#30739=CARTESIAN_POINT ( 'NONE',  ( 5.405949406249992428, -9.363379034771808662, -157.5937500020483810 ) ) ;
#30740=CARTESIAN_POINT ( 'NONE',  ( 9.999999999999998224, 0.000000000000000000, -179.0000000000000000 ) ) ;
#30743=CARTESIAN_POINT ( 'NONE',  ( 10.00000000000051159, -5.773502691895965988, -42.62499999999996447 ) ) ;
#30744=CARTESIAN_POINT ( 'NONE',  ( -9.999999999999998224, 1.224646799147353059E-15, -36.12500000409676915 ) ) ;
#30746=CARTESIAN_POINT ( 'NONE',  ( 10.81189881249999907, 6.242252689847868297, -88.21875000204838102 ) ) ;
#30748=CARTESIAN_POINT ( 'NONE',  ( -10.81189881249999729, 6.242252689847871849, -54.90625000204836681 ) ) ;
#30750=CARTESIAN_POINT ( 'NONE',  ( -5.405949406249996869, 9.363379034771805109, -124.0312500020483952 ) ) ;
#30751=CARTESIAN_POINT ( 'NONE',  ( 5.405949406249999534, 9.363379034771803333, -157.2812500020484094 ) ) ;
#30754=CARTESIAN_POINT ( 'NONE',  ( 9.999999999999996447, -5.773502691896262640, -130.0000000040967905 ) ) ;
#30756=ORIENTED_EDGE ( 'NONE', *, *, #27372, .F. ) ;
#30760=CARTESIAN_POINT ( 'NONE',  ( 5.405949406249999534, 9.363379034771803333, -188.7812500020484094 ) ) ;
#30762=CARTESIAN_POINT ( 'NONE',  ( -9.999999999999998224, 5.773502691896259087, -46.37499999999995737 ) ) ;
#30764=CARTESIAN_POINT ( 'NONE',  ( -4.999999999999996447, 8.660254037844387298, -57.37500000409676204 ) ) ;
#30765=CARTESIAN_POINT ( 'NONE',  ( -9.999999999999998224, 1.224646799147353059E-15, -152.7500000000000000 ) ) ;
#30768=AXIS2_PLACEMENT_3D ( 'NONE', #34895, #24542, #21504 ) ;
#30769=CARTESIAN_POINT ( 'NONE',  ( 10.81189881249999729, 0.000000000000000000, -49.53125000204838813 ) ) ;
#30773=CARTESIAN_POINT ( 'NONE',  ( 7.644554776091147741E-16, 12.48450537969573659, -175.1562500020484094 ) ) ;
#30779=CARTESIAN_POINT ( 'NONE',  ( -4.999999999999996447, 8.660254037844387298, -39.37500000409676915 ) ) ;
#30780=CARTESIAN_POINT ( 'NONE',  ( -10.81189881249999907, -6.242252689847864744, -87.65625000204836681 ) ) ;
#30781=ORIENTED_EDGE ( 'NONE', *, *, #1444, .F. ) ;
#30784=VERTEX_POINT ( 'NONE', #19673 ) ;
#30786=CARTESIAN_POINT ( 'NONE',  ( 5.405949406249992428, -9.363379034771808662, -36.09375000204836681 ) ) ;
#30787=CARTESIAN_POINT ( 'NONE',  ( 10.81189881249999729, 0.000000000000000000, -26.84375000204835970 ) ) ;
#30788=CARTESIAN_POINT ( 'NONE',  ( 10.81189881249999729, 0.000000000000000000, -15.03125000204835793 ) ) ;
#30789=CARTESIAN_POINT ( 'NONE',  ( -2.293366432827344421E-15, -12.48450537969573659, -64.71875000204838102 ) ) ;
#30790=CARTESIAN_POINT ( 'NONE',  ( 0.000000000000000000, 0.000000000000000000, -200.0000000000000000 ) ) ;
#30792=CARTESIAN_POINT ( 'NONE',  ( -10.81189881249999729, 6.242252689847871849, -183.7187500020484379 ) ) ;
#30794=CARTESIAN_POINT ( 'NONE',  ( -10.00000000000102496, 5.773502691895664007, -43.37499999999993605 ) ) ;
#30795=LINE ( 'NONE', #27765, #7444 ) ;
#30797=CARTESIAN_POINT ( 'NONE',  ( 10.81189881249999729, 0.000000000000000000, -109.3437500020483810 ) ) ;
#30799=CARTESIAN_POINT ( 'NONE',  ( -2.293366432827344421E-15, -12.48450537969573659, -82.90625000204838102 ) ) ;
#30800=CARTESIAN_POINT ( 'NONE',  ( 10.81189881249999729, 0.000000000000000000, -103.3437500020483668 ) ) ;
#30803=CARTESIAN_POINT ( 'NONE',  ( 10.00000000000000000, 5.773502691896255534, -152.2500000040967620 ) ) ;
#30807=CARTESIAN_POINT ( 'NONE',  ( 7.070501591499376803E-16, 11.54700538379251284, -153.5000000040967905 ) ) ;
#30808=CARTESIAN_POINT ( 'NONE',  ( 4.999999999999992006, -8.660254037844389075, -197.2500000000000000 ) ) ;
#30811=CARTESIAN_POINT ( 'NONE',  ( -9.999999999999998224, 5.773502691896259087, -74.87499999999997158 ) ) ;
#30813=CARTESIAN_POINT ( 'NONE',  ( -4.999999999999996447, 8.660254037844387298, -84.37500000409677625 ) ) ;
#30814=CYLINDRICAL_SURFACE ( 'NONE', #36864, 9.999999999999998224 ) ;
#30816=CARTESIAN_POINT ( 'NONE',  ( -10.81189881249999729, 1.324075727343319199E-15, -74.28125000204838102 ) ) ;
#30822=CARTESIAN_POINT ( 'NONE',  ( 10.00000000000000000, 5.773502691896255534, -4.874999999999959144 ) ) ;
#30824=CARTESIAN_POINT ( 'NONE',  ( -5.405949406250003975, -9.363379034771801557, -10.84375000204834727 ) ) ;
#30825=DIRECTION ( 'NONE',  ( 1.000000000000000000, 0.000000000000000000, 0.000000000000000000 ) ) ;
#30827=CARTESIAN_POINT ( 'NONE',  ( 5.405949406249999534, 9.363379034771803333, -131.7812500020483810 ) ) ;
#30828=CARTESIAN_POINT ( 'NONE',  ( 9.999999999999996447, -5.773502691896262640, -186.6250000000000284 ) ) ;
#30830=CARTESIAN_POINT ( 'NONE',  ( 7.644554776091147741E-16, 12.48450537969573659, -107.6562500020483810 ) ) ;
#30832=CARTESIAN_POINT ( 'NONE',  ( 7.070501591499376803E-16, 11.54700538379251284, -138.5000000040967905 ) ) ;
#30833=ORIENTED_EDGE ( 'NONE', *, *, #23858, .F. ) ;
#30834=ORIENTED_EDGE ( 'NONE', *, *, #10646, .T. ) ;
#30835=EDGE_CURVE ( 'NONE', #33047, #32122, #26587, .T. ) ;
#30836=CARTESIAN_POINT ( 'NONE',  ( 10.81189881249999551, -6.242252689847874514, -39.15625000204835260 ) ) ;
#30838=CARTESIAN_POINT ( 'NONE',  ( -10.81189881249999907, -6.242252689847864744, -90.46875000204836681 ) ) ;
#30840=CARTESIAN_POINT ( 'NONE',  ( -9.999999999999996447, 5.773502691896259975, -173.8750000000000000 ) ) ;
#30843=LINE ( 'NONE', #7324, #20506 ) ;
#30844=CARTESIAN_POINT ( 'NONE',  ( -10.81189881249999729, -6.242252689847864744, -121.9687500020484237 ) ) ;
#30846=CARTESIAN_POINT ( 'NONE',  ( -10.81189881249999729, 1.324075727343319199E-15, -0.7812500020483725827 ) ) ;
#30847=DIRECTION ( 'NONE',  ( 1.000000000000000000, 0.000000000000000000, 0.000000000000000000 ) ) ;
#30849=CARTESIAN_POINT ( 'NONE',  ( -9.999999999999998224, 1.224646799147353059E-15, -175.6250000040968189 ) ) ;
#30851=CARTESIAN_POINT ( 'NONE',  ( 10.81189881249999729, 0.000000000000000000, -180.0312500020483810 ) ) ;
#30854=CARTESIAN_POINT ( 'NONE',  ( -10.81189881249999729, 6.242252689847871849, -48.71875000204834549 ) ) ;
#30855=ADVANCED_FACE ( 'NONE', ( #10172 ), #29407, .T. ) ;
#30857=CARTESIAN_POINT ( 'NONE',  ( -10.81189881249999907, -6.242252689847864744, -14.15625000204836859 ) ) ;
#30859=CYLINDRICAL_SURFACE ( 'NONE', #37831, 9.999999999999998224 ) ;
#30861=CARTESIAN_POINT ( 'NONE',  ( -4.999999999999996447, 8.660254037844387298, -95.99999999999998579 ) ) ;
#30863=CARTESIAN_POINT ( 'NONE',  ( 10.00000000000000000, 5.773502691896255534, -102.7500000040967905 ) ) ;
#30864=CARTESIAN_POINT ( 'NONE',  ( 4.999999999999992006, -8.660254037844389075, -168.7500000000000000 ) ) ;
#30867=CARTESIAN_POINT ( 'NONE',  ( -2.293366432827344421E-15, -12.48450537969573659, -106.9062500020483810 ) ) ;
#30868=VERTEX_POINT ( 'NONE', #42126 ) ;
#30872=CARTESIAN_POINT ( 'NONE',  ( -5.405949406249996869, 9.363379034771805109, -163.0312500020484094 ) ) ;
#30875=CARTESIAN_POINT ( 'NONE',  ( -9.999999999999998224, 1.224646799147353059E-15, -25.24999999999996803 ) ) ;
#30876=VECTOR ( 'NONE', #12248, 1000.000000000000000 ) ;
#30877=CARTESIAN_POINT ( 'NONE',  ( 10.81189881249999551, -6.242252689847874514, -34.65625000204836681 ) ) ;
#30878=CARTESIAN_POINT ( 'NONE',  ( 5.000000000000000000, 8.660254037844385522, -160.7500000000000000 ) ) ;
#30880=CARTESIAN_POINT ( 'NONE',  ( -9.999999999999998224, 1.224646799147353059E-15, -200.0000000000000000 ) ) ;
#30882=CARTESIAN_POINT ( 'NONE',  ( -10.81189881249999729, 1.324075727343319199E-15, -131.2812500020483810 ) ) ;
#30884=ORIENTED_EDGE ( 'NONE', *, *, #12475, .T. ) ;
#30886=ORIENTED_EDGE ( 'NONE', *, *, #26939, .T. ) ;
#30888=CARTESIAN_POINT ( 'NONE',  ( -9.999999999999998224, 1.224646799147353059E-15, -46.62500000409677625 ) ) ;
#30889=CARTESIAN_POINT ( 'NONE',  ( -9.999999999999479527, -5.773502691896549521, -147.0000000040967620 ) ) ;
#30890=CARTESIAN_POINT ( 'NONE',  ( -5.405949406249996869, 9.363379034771805109, -162.8437500020484094 ) ) ;
#30892=CARTESIAN_POINT ( 'NONE',  ( -5.405949406250003975, -9.363379034771801557, -13.84375000204834905 ) ) ;
#30893=DIRECTION ( 'NONE',  ( -0.6123724356957964687, 0.3535533905932747301, 0.7071067811865454633 ) ) ;
#30895=CARTESIAN_POINT ( 'NONE',  ( -10.81189881249999729, -6.242252689847864744, -151.9687500020484094 ) ) ;
#30896=VECTOR ( 'NONE', #35316, 1000.000000000000000 ) ;
#30897=CARTESIAN_POINT ( 'NONE',  ( 10.81189881249999907, 6.242252689847868297, -134.7187500020484094 ) ) ;
#30898=( BOUNDED_CURVE ( )  B_SPLINE_CURVE ( 2, ( #19475, #3090, #19898, #23370, #3509, #3302, #13407 ),
 .UNSPECIFIED., .F., .F. ) 
 B_SPLINE_CURVE_WITH_KNOTS ( ( 3, 2, 2, 3 ),
 ( 0.4925373134328359104, 0.4937810945273632957, 0.4950248756218906809, 0.4962686567164180107 ),
 .UNSPECIFIED. ) 
 CURVE ( )  GEOMETRIC_REPRESENTATION_ITEM ( )  RATIONAL_B_SPLINE_CURVE ( ( 0.9999999999999880096, 0.8660254037844506980, 1.000000000000000000, 0.8660254037844387076, 1.000000000000000000, 0.8660254037844267172, 1.000000000000011990 ) ) 
 REPRESENTATION_ITEM ( '' )  );
#30899=CARTESIAN_POINT ( 'NONE',  ( -5.405949406249996869, 9.363379034771805109, -109.0312500020483810 ) ) ;
#30903=CARTESIAN_POINT ( 'NONE',  ( -9.999999999999998224, 5.773502691896259087, -198.2500000040968189 ) ) ;
#30905=CARTESIAN_POINT ( 'NONE',  ( 10.00000000000154010, -5.773502691895370020, -54.62499999999992895 ) ) ;
#30909=CARTESIAN_POINT ( 'NONE',  ( -10.81189881249999729, 6.242252689847871849, -75.71875000204838102 ) ) ;
#30910=CARTESIAN_POINT ( 'NONE',  ( 10.81189881249999551, -6.242252689847874514, -68.96875000204839523 ) ) ;
#30911=CARTESIAN_POINT ( 'NONE',  ( 4.999999999999992006, -8.660254037844389075, -19.12500000409675494 ) ) ;
#30912=CARTESIAN_POINT ( 'NONE',  ( -5.405949406250003975, -9.363379034771801557, -32.03125000204837391 ) ) ;
#30916=CARTESIAN_POINT ( 'NONE',  ( -4.999999999999996447, 8.660254037844387298, -120.0000000000000000 ) ) ;
#30917=CARTESIAN_POINT ( 'NONE',  ( 7.644554776091147741E-16, 12.48450537969573659, -128.6562500020483810 ) ) ;
#30920=CARTESIAN_POINT ( 'NONE',  ( -5.405949406249996869, 9.363379034771805109, -17.53125000204835970 ) ) ;
#30921=VERTEX_POINT ( 'NONE', #9544 ) ;
#30924=CARTESIAN_POINT ( 'NONE',  ( 4.999999999999992006, -8.660254037844389075, -179.6250000040968189 ) ) ;
#30925=CARTESIAN_POINT ( 'NONE',  ( 9.999999999999996447, -5.773502691896262640, -34.00000000409674783 ) ) ;
#30926=DIRECTION ( 'NONE',  ( 1.000000000000000000, 0.000000000000000000, 0.000000000000000000 ) ) ;
#30928=CARTESIAN_POINT ( 'NONE',  ( 9.999999999999998224, 0.000000000000000000, -147.5000000000000000 ) ) ;
#30929=CARTESIAN_POINT ( 'NONE',  ( 5.405949406249992428, -9.363379034771808662, -153.2812500020484094 ) ) ;
#30930=CARTESIAN_POINT ( 'NONE',  ( -10.81189881249999729, 6.242252689847871849, -125.2187500020483810 ) ) ;
#30931=CARTESIAN_POINT ( 'NONE',  ( 7.070501591499376803E-16, 11.54700538379251284, -190.6250000000000284 ) ) ;
#30934=CARTESIAN_POINT ( 'NONE',  ( -10.00000000000102496, 5.773502691895664007, -22.37499999999994671 ) ) ;
#30935=ORIENTED_EDGE ( 'NONE', *, *, #24533, .T. ) ;
#30937=EDGE_CURVE ( 'NONE', #2019, #12962, #17173, .T. ) ;
#30938=CARTESIAN_POINT ( 'NONE',  ( -10.81189881249999729, 6.242252689847871849, -108.7187500020483810 ) ) ;
#30940=EDGE_CURVE ( 'NONE', #7682, #10798, #1278, .T. ) ;
#30942=LINE ( 'NONE', #20999, #36187 ) ;
#30943=( BOUNDED_CURVE ( )  B_SPLINE_CURVE ( 2, ( #26065, #36191, #36405, #16530, #13503, #3615, #13711 ),
 .UNSPECIFIED., .F., .F. ) 
 B_SPLINE_CURVE_WITH_KNOTS ( ( 3, 2, 2, 3 ),
 ( 0.4701492537313434195, 0.4713930348258707492, 0.4726368159203981900, 0.4738805970149255198 ),
 .UNSPECIFIED. ) 
 CURVE ( )  GEOMETRIC_REPRESENTATION_ITEM ( )  RATIONAL_B_SPLINE_CURVE ( ( 0.9999999999999880096, 0.8660254037844506980, 1.000000000000000000, 0.8660254037844387076, 1.000000000000000000, 0.8660254037844207220, 1.000000000000017986 ) ) 
 REPRESENTATION_ITEM ( '' )  );
#30944=CARTESIAN_POINT ( 'NONE',  ( -5.405949406249996869, 9.363379034771805109, -186.8437500020483810 ) ) ;
#30945=CARTESIAN_POINT ( 'NONE',  ( -5.405949406249996869, 9.363379034771805109, -38.34375000204837391 ) ) ;
#30946=CARTESIAN_POINT ( 'NONE',  ( 6.419290871637174156, -8.565826599455219181, 3.494387113477268989E-15 ) ) ;
#30947=CARTESIAN_POINT ( 'NONE',  ( -9.999999999999479527, -5.773502691896549521, -74.62499999999994316 ) ) ;
#30948=CARTESIAN_POINT ( 'NONE',  ( -10.81189881249999729, 1.324075727343319199E-15, -168.5937500020484094 ) ) ;
#30949=CARTESIAN_POINT ( 'NONE',  ( -10.81189881249999729, 6.242252689847871849, -162.7187500020483810 ) ) ;
#30951=CARTESIAN_POINT ( 'NONE',  ( 9.999999999999479527, 5.773502691896553074, -178.8749999999999716 ) ) ;
#30955=CARTESIAN_POINT ( 'NONE',  ( -9.999999999999998224, 1.224646799147353059E-15, -58.24999999999997158 ) ) ;
#30956=( BOUNDED_CURVE ( )  B_SPLINE_CURVE ( 2, ( #21160, #4343, #41435, #8229, #24428, #14890, #17914 ),
 .UNSPECIFIED., .F., .F. ) 
 B_SPLINE_CURVE_WITH_KNOTS ( ( 3, 2, 2, 3 ),
 ( 0.3917910447761194792, 0.3930348258706468090, 0.3942786069651742498, 0.3955223880597015795 ),
 .UNSPECIFIED. ) 
 CURVE ( )  GEOMETRIC_REPRESENTATION_ITEM ( )  RATIONAL_B_SPLINE_CURVE ( ( 0.9999999999999940048, 0.8660254037844447028, 1.000000000000000000, 0.8660254037844387076, 1.000000000000000000, 0.8660254037844267172, 1.000000000000011990 ) ) 
 REPRESENTATION_ITEM ( '' )  );
#30959=CARTESIAN_POINT ( 'NONE',  ( 10.81189881249999907, 6.242252689847868297, -85.21875000204836681 ) ) ;
#30960=CARTESIAN_POINT ( 'NONE',  ( 9.999999999999998224, 0.000000000000000000, -135.5000000000000000 ) ) ;
#30961=CARTESIAN_POINT ( 'NONE',  ( 5.405949406249999534, 9.363379034771803333, -59.78125000204836681 ) ) ;
#30964=EDGE_CURVE ( 'NONE', #5198, #5513, #1711, .T. ) ;
#30965=CARTESIAN_POINT ( 'NONE',  ( -2.293366432827344421E-15, -12.48450537969573659, -117.4062500020483952 ) ) ;
#30966=VECTOR ( 'NONE', #26218, 1000.000000000000000 ) ;
#30967=CARTESIAN_POINT ( 'NONE',  ( 10.81189881249999729, 0.000000000000000000, -157.5312500020484094 ) ) ;
#30970=CARTESIAN_POINT ( 'NONE',  ( 9.999999999999998224, 0.000000000000000000, -129.8750000040967905 ) ) ;
#30975=CARTESIAN_POINT ( 'NONE',  ( -9.999999999999998224, 1.224646799147353059E-15, -200.0000000000000000 ) ) ;
#30976=EDGE_CURVE ( 'NONE', #24961, #9954, #21613, .T. ) ;
#30977=CARTESIAN_POINT ( 'NONE',  ( -2.293366432827344421E-15, -12.48450537969573659, -183.4062500020483810 ) ) ;
#30978=ORIENTED_EDGE ( 'NONE', *, *, #41370, .F. ) ;
#30979=CARTESIAN_POINT ( 'NONE',  ( 5.000000000000000000, 8.660254037844385522, -52.74999999999996447 ) ) ;
#30981=CARTESIAN_POINT ( 'NONE',  ( -2.121150477449813534E-15, -11.54700538379251284, -55.25000000409678336 ) ) ;
#30984=CARTESIAN_POINT ( 'NONE',  ( -9.999999999999998224, 1.224646799147353059E-15, -171.1250000040968189 ) ) ;
#30986=CARTESIAN_POINT ( 'NONE',  ( 10.81189881249999551, -6.242252689847874514, -52.65625000204836681 ) ) ;
#30988=AXIS2_PLACEMENT_3D ( 'NONE', #23099, #36261, #2827 ) ;
#30990=CARTESIAN_POINT ( 'NONE',  ( 10.00000000000154010, -5.773502691895370020, -29.50000000409671586 ) ) ;
#30991=CARTESIAN_POINT ( 'NONE',  ( -10.81189881249999729, 1.324075727343319199E-15, -177.7812500020484094 ) ) ;
#30992=CARTESIAN_POINT ( 'NONE',  ( -9.999999999999998224, 1.224646799147353059E-15, -200.0000000000000000 ) ) ;
#30993=CARTESIAN_POINT ( 'NONE',  ( 9.999999999999966249, 5.773502691896273298, -198.3750000000000284 ) ) ;
#30994=ADVANCED_FACE ( 'NONE', ( #40741 ), #28035, .T. ) ;
#30997=CARTESIAN_POINT ( 'NONE',  ( -10.81189881249999729, 1.324075727343319199E-15, -89.28125000204838102 ) ) ;
#30999=CARTESIAN_POINT ( 'NONE',  ( -4.999999999999996447, 8.660254037844387298, -91.87500000409677625 ) ) ;
#31000=ORIENTED_EDGE ( 'NONE', *, *, #8579, .F. ) ;
#31002=EDGE_CURVE ( 'NONE', #19501, #3609, #25781, .T. ) ;
#31003=CARTESIAN_POINT ( 'NONE',  ( 5.405949406249999534, 9.363379034771803333, -34.09375000204836681 ) ) ;
#31004=CARTESIAN_POINT ( 'NONE',  ( -10.81189881249999729, 6.242252689847871849, -26.21875000204837391 ) ) ;
#31005=CARTESIAN_POINT ( 'NONE',  ( 10.81189881249999729, 0.000000000000000000, -13.53125000204835615 ) ) ;
#31006=CARTESIAN_POINT ( 'NONE',  ( -10.81189881249999729, 1.324075727343319199E-15, -62.09375000204836681 ) ) ;
#31007=FACE_OUTER_BOUND ( 'NONE', #26873, .T. ) ;
#31009=CARTESIAN_POINT ( 'NONE',  ( -2.293366432827344421E-15, -12.48450537969573659, -183.2187500020484094 ) ) ;
#31013=FACE_OUTER_BOUND ( 'NONE', #17626, .T. ) ;
#31014=CARTESIAN_POINT ( 'NONE',  ( 0.000000000000000000, 0.000000000000000000, -200.0000000000000000 ) ) ;
#31015=CYLINDRICAL_SURFACE ( 'NONE', #17743, 9.999999999999998224 ) ;
#31016=CARTESIAN_POINT ( 'NONE',  ( 10.81189881249999729, 0.000000000000000000, -110.8437500020483810 ) ) ;
#31017=CARTESIAN_POINT ( 'NONE',  ( -9.999999999999998224, 1.224646799147353059E-15, -191.7500000000000000 ) ) ;
#31018=CARTESIAN_POINT ( 'NONE',  ( 10.81189881249999729, 0.000000000000000000, -85.53125000204838102 ) ) ;
#31019=CARTESIAN_POINT ( 'NONE',  ( 10.81189881249999729, 0.000000000000000000, -97.34375000204838102 ) ) ;
#31022=CARTESIAN_POINT ( 'NONE',  ( -9.999999999999998224, 5.773502691896259087, -156.2500000040967905 ) ) ;
#31027=PLANE ( 'NONE',  #2020 ) ;
#31030=CARTESIAN_POINT ( 'NONE',  ( -5.000000000000003553, -8.660254037844383745, -74.49999999999998579 ) ) ;
#31032=CARTESIAN_POINT ( 'NONE',  ( 7.070501591499377789E-16, 11.54700538379251284, -83.00000000409677625 ) ) ;
#31033=( BOUNDED_CURVE ( )  B_SPLINE_CURVE ( 2, ( #36219, #6028, #2791, #29537, #22422, #12682, #6867 ),
 .UNSPECIFIED., .F., .F. ) 
 B_SPLINE_CURVE_WITH_KNOTS ( ( 3, 2, 2, 3 ),
 ( 0.2388059701492538378, 0.2400497512437811953, 0.2412935323383085806, 0.2425373134328359381 ),
 .UNSPECIFIED. ) 
 CURVE ( )  GEOMETRIC_REPRESENTATION_ITEM ( )  RATIONAL_B_SPLINE_CURVE ( ( 0.9999999999999880096, 0.8660254037844506980, 1.000000000000000000, 0.8660254037844387076, 1.000000000000000000, 0.8660254037844267172, 1.000000000000011990 ) ) 
 REPRESENTATION_ITEM ( '' )  );
#31034=CARTESIAN_POINT ( 'NONE',  ( 9.999999999999998224, 0.000000000000000000, -26.37500000409676204 ) ) ;
#31036=CARTESIAN_POINT ( 'NONE',  ( 5.405949406249999534, 9.363379034771803333, -74.78125000204838102 ) ) ;
#31038=CARTESIAN_POINT ( 'NONE',  ( -10.00000000000154188, 5.773502691895366468, -19.37499999999993960 ) ) ;
#31040=VERTEX_POINT ( 'NONE', #41385 ) ;
#31041=CARTESIAN_POINT ( 'NONE',  ( 10.81189881249999907, 6.242252689847868297, -199.4062500020484094 ) ) ;
#31042=AXIS2_PLACEMENT_3D ( 'NONE', #3652, #27368, #26937 ) ;
#31044=CARTESIAN_POINT ( 'NONE',  ( -5.405949406249996869, 9.363379034771805109, -11.34375000204834727 ) ) ;
#31045=CARTESIAN_POINT ( 'NONE',  ( -10.00000000000019185, -5.773502691896140071, -177.0000000040967620 ) ) ;
#31047=CARTESIAN_POINT ( 'NONE',  ( 10.81189881249999551, -6.242252689847874514, -127.6562500020483952 ) ) ;
#31048=CARTESIAN_POINT ( 'NONE',  ( -4.999999999999996447, 8.660254037844387298, -183.0000000000000000 ) ) ;
#31049=CARTESIAN_POINT ( 'NONE',  ( 9.999999999999998224, 0.000000000000000000, -1.999999999999974021 ) ) ;
#31050=CARTESIAN_POINT ( 'NONE',  ( 10.81189881249999907, 6.242252689847868297, -112.4062500020483952 ) ) ;
#31051=ORIENTED_EDGE ( 'NONE', *, *, #22754, .F. ) ;
#31053=VERTEX_POINT ( 'NONE', #4716 ) ;
#31054=VERTEX_POINT ( 'NONE', #11821 ) ;
#31055=CARTESIAN_POINT ( 'NONE',  ( -5.405949406250003975, -9.363379034771801557, -38.03125000204838102 ) ) ;
#31057=CARTESIAN_POINT ( 'NONE',  ( -2.293366432827344421E-15, -12.48450537969573659, -84.21875000204835260 ) ) ;
#31061=CARTESIAN_POINT ( 'NONE',  ( 9.999999999998456346, 5.773502691897149042, -54.75000000409674783 ) ) ;
#31062=VECTOR ( 'NONE', #17372, 1000.000000000000000 ) ;
#31064=CARTESIAN_POINT ( 'NONE',  ( 10.81189881249999729, 0.000000000000000000, -124.3437500020483952 ) ) ;
#31066=CARTESIAN_POINT ( 'NONE',  ( 10.81189881249999729, 0.000000000000000000, -1.531250002048373249 ) ) ;
#31069=CARTESIAN_POINT ( 'NONE',  ( -4.999999999999996447, 8.660254037844387298, -177.3750000040967905 ) ) ;
#31071=CARTESIAN_POINT ( 'NONE',  ( 5.405949406249999534, 9.363379034771803333, -167.7812500020484094 ) ) ;
#31073=CARTESIAN_POINT ( 'NONE',  ( 10.00000000000102318, -5.773502691895667560, -1.000000004096722739 ) ) ;
#31076=CARTESIAN_POINT ( 'NONE',  ( -10.81189881249999729, 6.242252689847871849, -54.71875000204838813 ) ) ;
#31078=CARTESIAN_POINT ( 'NONE',  ( -5.405949406249996869, 9.363379034771805109, -13.03125000204835615 ) ) ;
#31080=CARTESIAN_POINT ( 'NONE',  ( 9.999999999999998224, 0.000000000000000000, -146.0000000000000000 ) ) ;
#31082=CARTESIAN_POINT ( 'NONE',  ( 5.000000000000000000, 8.660254037844385522, -94.74999999999998579 ) ) ;
#31084=CARTESIAN_POINT ( 'NONE',  ( -9.999999999999998224, 5.773502691896259087, -108.2500000040967763 ) ) ;
#31085=CARTESIAN_POINT ( 'NONE',  ( -2.121150477449813534E-15, -11.54700538379251284, -26.75000000409677270 ) ) ;
#31088=CARTESIAN_POINT ( 'NONE',  ( -5.405949406250003975, -9.363379034771801557, -101.0312500020483952 ) ) ;
#31090=ORIENTED_EDGE ( 'NONE', *, *, #8670, .T. ) ;
#31092=CARTESIAN_POINT ( 'NONE',  ( -9.999999999999998224, 1.224646799147353059E-15, -200.0000000000000000 ) ) ;
#31093=CARTESIAN_POINT ( 'NONE',  ( -5.405949406250003975, -9.363379034771801557, -164.0312500020484094 ) ) ;
#31096=CARTESIAN_POINT ( 'NONE',  ( -2.121150477449813534E-15, -11.54700538379251284, -23.37499999999998224 ) ) ;
#31097=CARTESIAN_POINT ( 'NONE',  ( -10.81189881249999729, -6.242252689847864744, -32.15625000204835970 ) ) ;
#31098=CARTESIAN_POINT ( 'NONE',  ( 7.070501591499377789E-16, 11.54700538379251284, -159.1250000000000000 ) ) ;
#31099=CARTESIAN_POINT ( 'NONE',  ( 9.999999999999998224, 0.000000000000000000, -91.99999999999998579 ) ) ;
#31102=CARTESIAN_POINT ( 'NONE',  ( -2.121150477449813534E-15, -11.54700538379251284, -33.87499999999996447 ) ) ;
#31103=CARTESIAN_POINT ( 'NONE',  ( 7.644554776091147741E-16, 12.48450537969573659, -133.1562500020483810 ) ) ;
#31104=CARTESIAN_POINT ( 'NONE',  ( 0.2267623460602178065, 10.23228579648178638, -4.586030929915087727E-15 ) ) ;
#31107=CARTESIAN_POINT ( 'NONE',  ( -5.405949406250003975, -9.363379034771801557, -63.53125000204837391 ) ) ;
#31108=VERTEX_POINT ( 'NONE', #29299 ) ;
#31111=DIRECTION ( 'NONE',  ( 1.000000000000000000, 0.000000000000000000, 0.000000000000000000 ) ) ;
#31112=CARTESIAN_POINT ( 'NONE',  ( -5.405949406250003975, -9.363379034771801557, -169.8437500020484094 ) ) ;
#31115=CARTESIAN_POINT ( 'NONE',  ( 10.81189881249999551, -6.242252689847874514, -13.46875000204836503 ) ) ;
#31117=CARTESIAN_POINT ( 'NONE',  ( -2.293366432827344421E-15, -12.48450537969573659, -151.7187500020483810 ) ) ;
#31118=CARTESIAN_POINT ( 'NONE',  ( -10.81189881249999907, -6.242252689847864744, -132.4687500020483810 ) ) ;
#31119=CARTESIAN_POINT ( 'NONE',  ( 10.81189881249999729, 0.000000000000000000, -105.0312500020483810 ) ) ;
#31121=CARTESIAN_POINT ( 'NONE',  ( 5.000000000000000000, 8.660254037844385522, -191.1250000040967905 ) ) ;
#31123=CARTESIAN_POINT ( 'NONE',  ( -2.293366432827344421E-15, -12.48450537969573659, -1.718750002048355929 ) ) ;
#31127=FACE_OUTER_BOUND ( 'NONE', #8011, .T. ) ;
#31131=CARTESIAN_POINT ( 'NONE',  ( -10.81189881249999729, 6.242252689847871849, -78.71875000204838102 ) ) ;
#31132=CARTESIAN_POINT ( 'NONE',  ( 7.644554776091147741E-16, 12.48450537969573659, -68.46875000204838102 ) ) ;
#31133=CARTESIAN_POINT ( 'NONE',  ( 9.999999999999998224, 0.000000000000000000, -18.87500000409675494 ) ) ;
#31134=CARTESIAN_POINT ( 'NONE',  ( 10.81189881249999551, -6.242252689847874514, -34.65625000204836681 ) ) ;
#31136=CARTESIAN_POINT ( 'NONE',  ( 0.000000000000000000, 0.000000000000000000, -200.0000000000000000 ) ) ;
#31138=CARTESIAN_POINT ( 'NONE',  ( 7.070501591499377789E-16, 11.54700538379251284, -123.1249999999999858 ) ) ;
#31139=CARTESIAN_POINT ( 'NONE',  ( 7.644554776091147741E-16, 12.48450537969573659, -131.6562500020483810 ) ) ;
#31140=CARTESIAN_POINT ( 'NONE',  ( -4.999999999999996447, 8.660254037844387298, -94.49999999999998579 ) ) ;
#31142=CARTESIAN_POINT ( 'NONE',  ( 10.81189881249999551, -6.242252689847874514, -7.656250002048368586 ) ) ;
#31143=ORIENTED_EDGE ( 'NONE', *, *, #29039, .T. ) ;
#31146=CARTESIAN_POINT ( 'NONE',  ( 9.999999999999998224, 0.000000000000000000, -56.37500000409676204 ) ) ;
#31147=VECTOR ( 'NONE', #6892, 1000.000000000000000 ) ;
#31148=CARTESIAN_POINT ( 'NONE',  ( -9.999999999999998224, 1.224646799147353059E-15, -33.12500000409676915 ) ) ;
#31152=CARTESIAN_POINT ( 'NONE',  ( -9.999999999998969713, -5.773502691896847949, -40.50000000409674072 ) ) ;
#31153=CARTESIAN_POINT ( 'NONE',  ( -5.405949406250003975, -9.363379034771801557, -155.0312500020484094 ) ) ;
#31154=CARTESIAN_POINT ( 'NONE',  ( 7.644554776091147741E-16, 12.48450537969573659, -126.9687500020483668 ) ) ;
#31155=CARTESIAN_POINT ( 'NONE',  ( 7.070501591499376803E-16, 11.54700538379251284, -3.500000004096760264 ) ) ;
#31156=ORIENTED_EDGE ( 'NONE', *, *, #35064, .T. ) ;
#31160=ORIENTED_EDGE ( 'NONE', *, *, #34683, .T. ) ;
#31161=ORIENTED_EDGE ( 'NONE', *, *, #26996, .T. ) ;
#31162=( BOUNDED_CURVE ( )  B_SPLINE_CURVE ( 2, ( #39151, #36338, #36760, #13431, #6770, #35919, #3117 ),
 .UNSPECIFIED., .F., .F. ) 
 B_SPLINE_CURVE_WITH_KNOTS ( ( 3, 2, 2, 3 ),
 ( 0.8395522388059704078, 0.8407960199004976820, 0.8420398009950251783, 0.8432835820895525636 ),
 .UNSPECIFIED. ) 
 CURVE ( )  GEOMETRIC_REPRESENTATION_ITEM ( )  RATIONAL_B_SPLINE_CURVE ( ( 0.9999999999999761302, 0.8660254037844625774, 1.000000000000000000, 0.8660254037844387076, 1.000000000000000000, 0.8660254037844028474, 1.000000000000035971 ) ) 
 REPRESENTATION_ITEM ( '' )  );
#31163=CARTESIAN_POINT ( 'NONE',  ( 9.999999999999742428, 5.773502691896404748, -189.3749999999999716 ) ) ;
#31164=CARTESIAN_POINT ( 'NONE',  ( 7.644554776091147741E-16, 12.48450537969573659, -192.9687500020483810 ) ) ;
#31166=CARTESIAN_POINT ( 'NONE',  ( 7.644554776091147741E-16, 12.48450537969573659, -36.96875000204835970 ) ) ;
#31167=CARTESIAN_POINT ( 'NONE',  ( 1.679738968335770632, -10.37593646986413276, 1.566949817559348910E-14 ) ) ;
#31168=CARTESIAN_POINT ( 'NONE',  ( 5.000000000000000000, 8.660254037844385522, -139.7499999999999716 ) ) ;
#31169=CARTESIAN_POINT ( 'NONE',  ( 5.405949406249999534, 9.363379034771803333, -170.5937500020484094 ) ) ;
#31170=CARTESIAN_POINT ( 'NONE',  ( -10.81189881249999729, 1.324075727343319199E-15, -162.5937500020484094 ) ) ;
#31175=CARTESIAN_POINT ( 'NONE',  ( -9.999999999999612754, -5.773502691896474914, -155.6249999999999716 ) ) ;
#31176=FACE_OUTER_BOUND ( 'NONE', #3265, .T. ) ;
#31178=CARTESIAN_POINT ( 'NONE',  ( -5.405949406249996869, 9.363379034771805109, -90.84375000204838102 ) ) ;
#31180=CARTESIAN_POINT ( 'NONE',  ( -5.405949406250003975, -9.363379034771801557, -62.03125000204837391 ) ) ;
#31183=CARTESIAN_POINT ( 'NONE',  ( -10.81189881249999907, -6.242252689847864744, -111.6562500020483952 ) ) ;
#31184=CARTESIAN_POINT ( 'NONE',  ( -5.405949406250003975, -9.363379034771801557, -156.5312500020484094 ) ) ;
#31187=CARTESIAN_POINT ( 'NONE',  ( 7.070501591499377789E-16, 11.54700538379251284, -134.0000000040967905 ) ) ;
#31189=ORIENTED_EDGE ( 'NONE', *, *, #36252, .F. ) ;
#31192=CARTESIAN_POINT ( 'NONE',  ( -4.999999999999996447, 8.660254037844387298, -67.87500000409677625 ) ) ;
#31193=CARTESIAN_POINT ( 'NONE',  ( -10.81189881249999729, 6.242252689847871849, -180.9062500020484094 ) ) ;
#31194=ORIENTED_EDGE ( 'NONE', *, *, #431, .F. ) ;
#31196=CARTESIAN_POINT ( 'NONE',  ( 7.070501591499377789E-16, 11.54700538379251284, -54.50000000409677625 ) ) ;
#31197=EDGE_CURVE ( 'NONE', #4760, #26724, #37875, .T. ) ;
#31199=DIRECTION ( 'NONE',  ( -0.000000000000000000, -0.000000000000000000, 1.000000000000000000 ) ) ;
#31200=EDGE_CURVE ( 'NONE', #28824, #19402, #42268, .T. ) ;
#31202=CARTESIAN_POINT ( 'NONE',  ( -10.81189881249999729, -6.242252689847864744, -54.65625000204838813 ) ) ;
#31206=CARTESIAN_POINT ( 'NONE',  ( -10.81189881249999729, 1.324075727343319199E-15, -174.7812500020484094 ) ) ;
#31207=VECTOR ( 'NONE', #3908, 1000.000000000000000 ) ;
#31210=VERTEX_POINT ( 'NONE', #21973 ) ;
#31211=CARTESIAN_POINT ( 'NONE',  ( 23.09401076758504345, 1.040834085586084257E-14, 0.000000000000000000 ) ) ;
#31214=FACE_OUTER_BOUND ( 'NONE', #11386, .T. ) ;
#31215=CARTESIAN_POINT ( 'NONE',  ( 5.405949406249999534, 9.363379034771803333, -83.78125000204838102 ) ) ;
#31216=ORIENTED_EDGE ( 'NONE', *, *, #13341, .F. ) ;
#31219=CARTESIAN_POINT ( 'NONE',  ( -10.81189881249999729, 1.324075727343319199E-15, -33.59375000204836681 ) ) ;
#31221=CARTESIAN_POINT ( 'NONE',  ( -5.405949406249996869, 9.363379034771805109, -17.53125000204835970 ) ) ;
#31222=( BOUNDED_CURVE ( )  B_SPLINE_CURVE ( 2, ( #10207, #32893, #33326, #23172, #23393, #6354, #25996 ),
 .UNSPECIFIED., .F., .F. ) 
 B_SPLINE_CURVE_WITH_KNOTS ( ( 3, 2, 2, 3 ),
 ( 0.7350746268656719318, 0.7363184079601993171, 0.7375621890547265913, 0.7388059701492539766 ),
 .UNSPECIFIED. ) 
 CURVE ( )  GEOMETRIC_REPRESENTATION_ITEM ( )  RATIONAL_B_SPLINE_CURVE ( ( 0.9999999999999641398, 0.8660254037844745678, 1.000000000000000000, 0.8660254037844387076, 1.000000000000000000, 0.8660254037844148378, 1.000000000000023981 ) ) 
 REPRESENTATION_ITEM ( '' )  );
#31223=CARTESIAN_POINT ( 'NONE',  ( 10.81189881249999729, 0.000000000000000000, -64.34375000204836681 ) ) ;
#31224=ORIENTED_EDGE ( 'NONE', *, *, #13771, .F. ) ;
#31225=CARTESIAN_POINT ( 'NONE',  ( -9.999999999999998224, 1.224646799147353059E-15, -131.7499999999999716 ) ) ;
#31227=EDGE_CURVE ( 'NONE', #23672, #3711, #39218, .T. ) ;
#31228=CARTESIAN_POINT ( 'NONE',  ( 10.81189881249999551, -6.242252689847874514, -182.9687500020484094 ) ) ;
#31230=CARTESIAN_POINT ( 'NONE',  ( -9.999999999999998224, 1.224646799147353059E-15, -200.0000000000000000 ) ) ;
#31231=CARTESIAN_POINT ( 'NONE',  ( 7.070501591499376803E-16, 11.54700538379251284, -59.00000000409676915 ) ) ;
#31232=CARTESIAN_POINT ( 'NONE',  ( 7.070501591499376803E-16, 11.54700538379251284, -141.1250000000000000 ) ) ;
#31233=DIRECTION ( 'NONE',  ( -0.000000000000000000, -0.000000000000000000, 1.000000000000000000 ) ) ;
#31235=CARTESIAN_POINT ( 'NONE',  ( 7.644554776091147741E-16, 12.48450537969573659, -113.4687500020483952 ) ) ;
#31236=CYLINDRICAL_SURFACE ( 'NONE', #25955, 9.999999999999998224 ) ;
#31237=CARTESIAN_POINT ( 'NONE',  ( -10.81189881249999729, 6.242252689847871849, -80.40625000204839523 ) ) ;
#31238=CARTESIAN_POINT ( 'NONE',  ( -5.405949406250003975, -9.363379034771801557, -94.84375000204838102 ) ) ;
#31241=CARTESIAN_POINT ( 'NONE',  ( -4.999999999999996447, 8.660254037844387298, -153.3750000040967905 ) ) ;
#31245=CARTESIAN_POINT ( 'NONE',  ( -9.999999999998969713, -5.773502691896847949, -13.50000000409673540 ) ) ;
#31246=CARTESIAN_POINT ( 'NONE',  ( -9.999999999999998224, 1.224646799147353059E-15, -172.2500000000000000 ) ) ;
#31248=CARTESIAN_POINT ( 'NONE',  ( 5.000000000000000000, 8.660254037844385522, -63.24999999999997158 ) ) ;
#31249=CARTESIAN_POINT ( 'NONE',  ( 7.070501591499377789E-16, 11.54700538379251284, -72.12499999999995737 ) ) ;
#31251=CARTESIAN_POINT ( 'NONE',  ( 9.999999999999996447, -5.773502691896262640, -85.00000000409677625 ) ) ;
#31255=CARTESIAN_POINT ( 'NONE',  ( 7.644554776091147741E-16, 12.48450537969573659, -74.65625000204838102 ) ) ;
#31260=ORIENTED_EDGE ( 'NONE', *, *, #15933, .T. ) ;
#31261=CARTESIAN_POINT ( 'NONE',  ( -2.121150477449813534E-15, -11.54700538379251284, -2.374999999999946709 ) ) ;
#31264=CARTESIAN_POINT ( 'NONE',  ( -10.81189881249999729, 6.242252689847871849, -14.21875000204836681 ) ) ;
#31265=CARTESIAN_POINT ( 'NONE',  ( 9.999999999999998224, 0.000000000000000000, -93.87500000409677625 ) ) ;
#31267=CARTESIAN_POINT ( 'NONE',  ( -9.999999999999998224, 1.224646799147353059E-15, -200.0000000000000000 ) ) ;
#31268=CARTESIAN_POINT ( 'NONE',  ( 7.644554776091147741E-16, 12.48450537969573659, -131.6562500020483810 ) ) ;
#31269=CARTESIAN_POINT ( 'NONE',  ( 10.00000000000000000, 5.773502691896255534, -186.3750000000000284 ) ) ;
#31270=CARTESIAN_POINT ( 'NONE',  ( -5.405949406249996869, 9.363379034771805109, -106.0312500020483810 ) ) ;
#31271=ORIENTED_EDGE ( 'NONE', *, *, #375, .T. ) ;
#31273=VERTEX_POINT ( 'NONE', #22613 ) ;
#31274=VERTEX_POINT ( 'NONE', #32131 ) ;
#31275=ADVANCED_FACE ( 'NONE', ( #28472 ), #6219, .T. ) ;
#31276=CARTESIAN_POINT ( 'NONE',  ( 10.81189881249999551, -6.242252689847874514, -40.65625000204835970 ) ) ;
#31278=CARTESIAN_POINT ( 'NONE',  ( 5.405949406249999534, 9.363379034771803333, -88.09375000204836681 ) ) ;
#31279=CYLINDRICAL_SURFACE ( 'NONE', #10482, 9.999999999999998224 ) ;
#31283=CARTESIAN_POINT ( 'NONE',  ( -5.000000000000003553, -8.660254037844383745, -139.0000000000000000 ) ) ;
#31284=CARTESIAN_POINT ( 'NONE',  ( 5.405949406249999534, 9.363379034771803333, -121.0937500020483952 ) ) ;
#31285=( BOUNDED_CURVE ( )  B_SPLINE_CURVE ( 2, ( #18967, #32154, #14652, #27841, #40973, #11417, #24611 ),
 .UNSPECIFIED., .F., .F. ) 
 B_SPLINE_CURVE_WITH_KNOTS ( ( 3, 2, 2, 3 ),
 ( 0.04104477611940302029, 0.04228855721393039169, 0.04353233830845775615, 0.04477611940298512061 ),
 .UNSPECIFIED. ) 
 CURVE ( )  GEOMETRIC_REPRESENTATION_ITEM ( )  RATIONAL_B_SPLINE_CURVE ( ( 0.9999999999999963363, 0.8660254037844424824, 1.000000000000000000, 0.8660254037844387076, 1.000000000000000000, 0.8660254037844334896, 1.000000000000005329 ) ) 
 REPRESENTATION_ITEM ( '' )  );
#31287=CARTESIAN_POINT ( 'NONE',  ( 9.999999999999998224, 0.000000000000000000, -200.0000000000000000 ) ) ;
#31290=CARTESIAN_POINT ( 'NONE',  ( -5.000000000000003553, -8.660254037844383745, -176.8750000040967905 ) ) ;
#31291=CARTESIAN_POINT ( 'NONE',  ( -5.405949406249996869, 9.363379034771805109, -173.5312500020484094 ) ) ;
#31292=CARTESIAN_POINT ( 'NONE',  ( 9.999999999998969713, 5.773502691896851502, -103.8750000000000000 ) ) ;
#31295=CARTESIAN_POINT ( 'NONE',  ( -10.81189881249999729, 1.324075727343319199E-15, -51.59375000204835260 ) ) ;
#31297=CARTESIAN_POINT ( 'NONE',  ( -5.405949406250003975, -9.363379034771801557, -12.53125000204835615 ) ) ;
#31299=CARTESIAN_POINT ( 'NONE',  ( 9.999999999998456346, 5.773502691897149042, -54.37499999999994316 ) ) ;
#31301=CARTESIAN_POINT ( 'NONE',  ( 5.000000000000000000, 8.660254037844385522, -99.24999999999998579 ) ) ;
#31303=CARTESIAN_POINT ( 'NONE',  ( 7.070501591499377789E-16, 11.54700538379251284, -108.5000000040967763 ) ) ;
#31304=FACE_OUTER_BOUND ( 'NONE', #21268, .T. ) ;
#31307=CARTESIAN_POINT ( 'NONE',  ( -5.405949406249996869, 9.363379034771805109, -100.0312500020483952 ) ) ;
#31311=CARTESIAN_POINT ( 'NONE',  ( 10.81189881249999551, -6.242252689847874514, -168.1562500020484094 ) ) ;
#31314=CARTESIAN_POINT ( 'NONE',  ( 7.070501591499377789E-16, 11.54700538379251284, -24.12499999999998934 ) ) ;
#31315=CARTESIAN_POINT ( 'NONE',  ( -10.81189881249999729, 6.242252689847871849, -24.90625000204838813 ) ) ;
#31316=CARTESIAN_POINT ( 'NONE',  ( -2.121150477449813534E-15, -11.54700538379251284, -164.3750000000000000 ) ) ;
#31317=CARTESIAN_POINT ( 'NONE',  ( 4.999999999999992006, -8.660254037844389075, -102.7500000000000000 ) ) ;
#31320=EDGE_CURVE ( 'NONE', #25539, #39040, #2980, .T. ) ;
#31321=CARTESIAN_POINT ( 'NONE',  ( -5.405949406250003975, -9.363379034771801557, -137.0312500020484094 ) ) ;
#31322=CARTESIAN_POINT ( 'NONE',  ( -1.040834085586084257E-14, -20.00000000000000355, 32.49999999999999289 ) ) ;
#31323=CARTESIAN_POINT ( 'NONE',  ( -9.999999999999998224, 1.224646799147353059E-15, -69.12500000409677625 ) ) ;
#31324=ORIENTED_EDGE ( 'NONE', *, *, #1662, .F. ) ;
#31325=CARTESIAN_POINT ( 'NONE',  ( 5.405949406249999534, 9.363379034771803333, -61.28125000204837391 ) ) ;
#31329=CARTESIAN_POINT ( 'NONE',  ( -9.999999999999998224, 1.224646799147353059E-15, -181.6250000040967905 ) ) ;
#31330=CARTESIAN_POINT ( 'NONE',  ( -2.253471898105756789E-15, 15.00000000000011013, 49.99999999999998579 ) ) ;
#31331=( BOUNDED_CURVE ( )  B_SPLINE_CURVE ( 2, ( #36783, #16910, #27287, #40637, #1181, #7219, #14524 ),
 .UNSPECIFIED., .F., .F. ) 
 B_SPLINE_CURVE_WITH_KNOTS ( ( 3, 2, 2, 3 ),
 ( 0.2611940298507463565, 0.2624378109452737418, 0.2636815920398011270, 0.2649253731343284568 ),
 .UNSPECIFIED. ) 
 CURVE ( )  GEOMETRIC_REPRESENTATION_ITEM ( )  RATIONAL_B_SPLINE_CURVE ( ( 0.9999999999999880096, 0.8660254037844506980, 1.000000000000000000, 0.8660254037844387076, 1.000000000000000000, 0.8660254037844267172, 1.000000000000011990 ) ) 
 REPRESENTATION_ITEM ( '' )  );
#31332=CARTESIAN_POINT ( 'NONE',  ( -5.405949406249996869, 9.363379034771805109, -159.8437500020484094 ) ) ;
#31334=CARTESIAN_POINT ( 'NONE',  ( -10.81189881249999729, 6.242252689847871849, -8.218750002048354375 ) ) ;
#31335=CARTESIAN_POINT ( 'NONE',  ( -9.999999999999998224, 1.224646799147353059E-15, -129.1250000040967620 ) ) ;
#31336=CARTESIAN_POINT ( 'NONE',  ( -5.405949406250003975, -9.363379034771801557, -147.3437500020483810 ) ) ;
#31337=CARTESIAN_POINT ( 'NONE',  ( 10.81189881249999551, -6.242252689847874514, -106.6562500020483952 ) ) ;
#31339=CARTESIAN_POINT ( 'NONE',  ( 10.00000000000012257, -5.773502691896187144, -161.1250000000000568 ) ) ;
#31341=CARTESIAN_POINT ( 'NONE',  ( 10.81189881249999551, -6.242252689847874514, -1.468750002048354819 ) ) ;
#31343=CARTESIAN_POINT ( 'NONE',  ( -10.81189881249999729, -6.242252689847864744, -195.6562500020484094 ) ) ;
#31344=DIRECTION ( 'NONE',  ( -0.000000000000000000, -0.000000000000000000, 1.000000000000000000 ) ) ;
#31347=CARTESIAN_POINT ( 'NONE',  ( 10.81189881249999551, -6.242252689847874514, -74.96875000204839523 ) ) ;
#31348=CARTESIAN_POINT ( 'NONE',  ( -10.81189881249999729, 1.324075727343319199E-15, -59.09375000204835970 ) ) ;
#31350=CARTESIAN_POINT ( 'NONE',  ( -10.81189881249999729, 1.324075727343319199E-15, -33.78125000204837391 ) ) ;
#31354=CARTESIAN_POINT ( 'NONE',  ( -10.00000000000000000, -5.773502691896251982, -124.1250000000000000 ) ) ;
#31357=CARTESIAN_POINT ( 'NONE',  ( -5.405949406250003975, -9.363379034771801557, -6.531250002048377468 ) ) ;
#31359=DIRECTION ( 'NONE',  ( -0.000000000000000000, -0.000000000000000000, 1.000000000000000000 ) ) ;
#31363=CARTESIAN_POINT ( 'NONE',  ( 9.999999999999996447, -5.773502691896262640, -37.00000000409676204 ) ) ;
#31364=CARTESIAN_POINT ( 'NONE',  ( -10.00000000000102496, 5.773502691895664007, -61.37499999999995737 ) ) ;
#31366=CYLINDRICAL_SURFACE ( 'NONE', #4871, 9.999999999999998224 ) ;
#31367=CARTESIAN_POINT ( 'NONE',  ( 10.81189881249999907, 6.242252689847868297, -146.9062500020484094 ) ) ;
#31368=CARTESIAN_POINT ( 'NONE',  ( -5.405949406250003975, -9.363379034771801557, -123.3437500020483952 ) ) ;
#31369=CARTESIAN_POINT ( 'NONE',  ( -9.999999999999998224, 1.224646799147353059E-15, -200.0000000000000000 ) ) ;
#31370=CYLINDRICAL_SURFACE ( 'NONE', #33491, 9.999999999999998224 ) ;
#31371=ORIENTED_EDGE ( 'NONE', *, *, #19616, .F. ) ;
#31372=AXIS2_PLACEMENT_3D ( 'NONE', #23865, #30129, #774 ) ;
#31373=ORIENTED_EDGE ( 'NONE', *, *, #7944, .T. ) ;
#31375=EDGE_CURVE ( 'NONE', #468, #13705, #5366, .T. ) ;
#31377=CARTESIAN_POINT ( 'NONE',  ( -2.293366432827344421E-15, -12.48450537969573659, -181.7187500020484094 ) ) ;
#31378=CARTESIAN_POINT ( 'NONE',  ( 7.644554776091147741E-16, 12.48450537969573659, -38.46875000204835260 ) ) ;
#31379=CARTESIAN_POINT ( 'NONE',  ( 9.999999999999227285, 5.773502691896701400, -110.2500000040967478 ) ) ;
#31380=CARTESIAN_POINT ( 'NONE',  ( 5.405949406249992428, -9.363379034771808662, -174.0937500020484094 ) ) ;
#31381=CARTESIAN_POINT ( 'NONE',  ( -2.293366432827344421E-15, -12.48450537969573659, -156.2187500020483810 ) ) ;
#31382=CARTESIAN_POINT ( 'NONE',  ( 4.999999999999992006, -8.660254037844389075, -76.12500000409677625 ) ) ;
#31387=CARTESIAN_POINT ( 'NONE',  ( -9.999999999999996447, 5.773502691896259975, -169.3750000000000000 ) ) ;
#31389=CARTESIAN_POINT ( 'NONE',  ( 5.405949406249992428, -9.363379034771808662, -78.09375000204838102 ) ) ;
#31390=DIRECTION ( 'NONE',  ( 1.000000000000000000, 0.000000000000000000, 0.000000000000000000 ) ) ;
#31391=CARTESIAN_POINT ( 'NONE',  ( 10.81189881249999551, -6.242252689847874514, -60.15625000204839523 ) ) ;
#31394=CARTESIAN_POINT ( 'NONE',  ( -10.81189881249999729, 6.242252689847871849, -117.9062500020483952 ) ) ;
#31395=CARTESIAN_POINT ( 'NONE',  ( 5.405949406249999534, 9.363379034771803333, -154.2812500020484094 ) ) ;
#31396=LINE ( 'NONE', #8304, #24112 ) ;
#31398=CARTESIAN_POINT ( 'NONE',  ( 10.00000000000000000, 5.773502691896255534, -128.2500000040967620 ) ) ;
#31400=EDGE_LOOP ( 'NONE', ( #27906, #9777, #19119, #8313 ) ) ;
#31401=AXIS2_PLACEMENT_3D ( 'NONE', #13842, #24236, #34163 ) ;
#31404=CARTESIAN_POINT ( 'NONE',  ( 9.999999999999998224, 0.000000000000000000, -192.8750000040967905 ) ) ;
#31405=CARTESIAN_POINT ( 'NONE',  ( 10.81189881249999551, -6.242252689847874514, -180.1562500020484379 ) ) ;
#31406=ORIENTED_EDGE ( 'NONE', *, *, #19513, .F. ) ;
#31408=CARTESIAN_POINT ( 'NONE',  ( 4.999999999999992006, -8.660254037844389075, -61.12500000409676204 ) ) ;
#31410=CARTESIAN_POINT ( 'NONE',  ( -4.999999999999996447, 8.660254037844387298, -171.3750000040968189 ) ) ;
#31414=CARTESIAN_POINT ( 'NONE',  ( -10.81189881249999907, -6.242252689847864744, -165.6562500020483810 ) ) ;
#31415=FACE_OUTER_BOUND ( 'NONE', #12387, .T. ) ;
#31417=ORIENTED_EDGE ( 'NONE', *, *, #23199, .F. ) ;
#31418=CARTESIAN_POINT ( 'NONE',  ( 10.00000000000102318, -5.773502691895667560, -0.6249999999999450440 ) ) ;
#31419=CARTESIAN_POINT ( 'NONE',  ( -9.999999999999612754, -5.773502691896474914, -154.1249999999999716 ) ) ;
#31421=CARTESIAN_POINT ( 'NONE',  ( -2.121150477449813534E-15, -11.54700538379251284, -163.2500000040968189 ) ) ;
#31422=CARTESIAN_POINT ( 'NONE',  ( -5.405949406249996869, 9.363379034771805109, -79.03125000204838102 ) ) ;
#31424=CARTESIAN_POINT ( 'NONE',  ( 10.81189881249999729, 0.000000000000000000, -199.4375000020484094 ) ) ;
#31425=CARTESIAN_POINT ( 'NONE',  ( -9.999999999999998224, 1.224646799147353059E-15, -200.0000000000000000 ) ) ;
#31426=ORIENTED_EDGE ( 'NONE', *, *, #27004, .T. ) ;
#31428=CARTESIAN_POINT ( 'NONE',  ( -5.405949406249996869, 9.363379034771805109, -39.84375000204837391 ) ) ;
#31429=CARTESIAN_POINT ( 'NONE',  ( -2.121150477449813534E-15, -11.54700538379251284, -186.8750000000000000 ) ) ;
#31430=CARTESIAN_POINT ( 'NONE',  ( -10.81189881249999729, 1.324075727343319199E-15, -15.78125000204835793 ) ) ;
#31431=CARTESIAN_POINT ( 'NONE',  ( -10.81189881249999907, -6.242252689847864744, -64.96875000204838102 ) ) ;
#31432=ORIENTED_EDGE ( 'NONE', *, *, #26353, .T. ) ;
#31434=EDGE_CURVE ( 'NONE', #26359, #468, #31846, .T. ) ;
#31436=CARTESIAN_POINT ( 'NONE',  ( -10.81189881249999729, 6.242252689847871849, -197.2187500020484379 ) ) ;
#31437=CARTESIAN_POINT ( 'NONE',  ( 10.81189881249999729, 0.000000000000000000, -175.3437500020483810 ) ) ;
#31443=CARTESIAN_POINT ( 'NONE',  ( -10.81189881249999729, 1.324075727343319199E-15, -111.5937500020483810 ) ) ;
#31444=LINE ( 'NONE', #15224, #9403 ) ;
#31445=CARTESIAN_POINT ( 'NONE',  ( -10.81189881249999729, 6.242252689847871849, -84.90625000204838102 ) ) ;
#31446=CARTESIAN_POINT ( 'NONE',  ( -2.293366432827344421E-15, -12.48450537969573659, -94.71875000204838102 ) ) ;
#31449=CARTESIAN_POINT ( 'NONE',  ( 5.000000000000000000, 8.660254037844385522, -152.1250000040967905 ) ) ;
#31454=CARTESIAN_POINT ( 'NONE',  ( 10.70731569305672615, 1.500182182589836044, 0.000000000000000000 ) ) ;
#31457=CARTESIAN_POINT ( 'NONE',  ( 10.00000000000000000, 5.773502691896255534, -61.87499999999998579 ) ) ;
#31459=CARTESIAN_POINT ( 'NONE',  ( -9.999999999999998224, 5.773502691896259087, -85.75000000409676204 ) ) ;
#31460=CARTESIAN_POINT ( 'NONE',  ( -9.999999999999479527, -5.773502691896549521, -142.5000000040967620 ) ) ;
#31462=CARTESIAN_POINT ( 'NONE',  ( 10.81189881249999551, -6.242252689847874514, -76.65625000204838102 ) ) ;
#31465=CARTESIAN_POINT ( 'NONE',  ( -9.999999999999998224, 1.224646799147353059E-15, -69.12500000409677625 ) ) ;
#31467=ORIENTED_EDGE ( 'NONE', *, *, #13116, .T. ) ;
#31468=CARTESIAN_POINT ( 'NONE',  ( 7.070501591499377789E-16, 11.54700538379251284, -3.124999999999951150 ) ) ;
#31470=CARTESIAN_POINT ( 'NONE',  ( 10.81189881249999729, 6.242252689847867408, -14.71875000204836859 ) ) ;
#31471=CARTESIAN_POINT ( 'NONE',  ( 5.000000000000000000, 8.660254037844385522, -142.7500000000000000 ) ) ;
#31472=CARTESIAN_POINT ( 'NONE',  ( -2.293366432827344421E-15, -12.48450537969573659, -139.7187500020483810 ) ) ;
#31473=CARTESIAN_POINT ( 'NONE',  ( 9.999999999999998224, 0.000000000000000000, -123.5000000000000000 ) ) ;
#31474=CARTESIAN_POINT ( 'NONE',  ( 10.81189881249999729, 0.000000000000000000, -129.0312500020484094 ) ) ;
#31475=( BOUNDED_CURVE ( )  B_SPLINE_CURVE ( 2, ( #40865, #8092, #2052, #41521, #31192, #15183, #28379 ),
 .UNSPECIFIED., .F., .F. ) 
 B_SPLINE_CURVE_WITH_KNOTS ( ( 3, 2, 2, 3 ),
 ( 0.6492537313432837909, 0.6504975124378111762, 0.6517412935323385614, 0.6529850746268659467 ),
 .UNSPECIFIED. ) 
 CURVE ( )  GEOMETRIC_REPRESENTATION_ITEM ( )  RATIONAL_B_SPLINE_CURVE ( ( 0.9999999999999761302, 0.8660254037844625774, 1.000000000000000000, 0.8660254037844387076, 1.000000000000000000, 0.8660254037844148378, 1.000000000000023981 ) ) 
 REPRESENTATION_ITEM ( '' )  );
#31476=CARTESIAN_POINT ( 'NONE',  ( 4.999999999999992006, -8.660254037844389075, -182.2500000000000000 ) ) ;
#31478=CARTESIAN_POINT ( 'NONE',  ( -5.405949406249996869, 9.363379034771805109, -101.5312500020483952 ) ) ;
#31479=ORIENTED_EDGE ( 'NONE', *, *, #25981, .F. ) ;
#31481=ORIENTED_EDGE ( 'NONE', *, *, #35386, .T. ) ;
#31484=CARTESIAN_POINT ( 'NONE',  ( -10.81189881249999907, -6.242252689847864744, -38.15625000204835260 ) ) ;
#31486=CARTESIAN_POINT ( 'NONE',  ( 10.81189881249999551, -6.242252689847874514, -83.96875000204838102 ) ) ;
#31487=CARTESIAN_POINT ( 'NONE',  ( 9.999999999999742428, 5.773502691896404748, -128.2500000040967905 ) ) ;
#31488=EDGE_CURVE ( 'NONE', #17896, #37898, #30455, .T. ) ;
#31490=EDGE_CURVE ( 'NONE', #32484, #40773, #16533, .T. ) ;
#31493=CARTESIAN_POINT ( 'NONE',  ( 0.000000000000000000, 0.000000000000000000, -200.0000000000000000 ) ) ;
#31495=CARTESIAN_POINT ( 'NONE',  ( 9.999999999999998224, 0.000000000000000000, -85.99999999999998579 ) ) ;
#31496=CARTESIAN_POINT ( 'NONE',  ( -10.81189881249999729, 6.242252689847871849, -116.2187500020483810 ) ) ;
#31500=DIRECTION ( 'NONE',  ( 1.000000000000000000, 0.000000000000000000, 0.000000000000000000 ) ) ;
#31503=CARTESIAN_POINT ( 'NONE',  ( -9.999999999999998224, 1.224646799147353059E-15, -178.6250000040968189 ) ) ;
#31504=CARTESIAN_POINT ( 'NONE',  ( 10.81189881249999729, 0.000000000000000000, -174.0312500020484094 ) ) ;
#31505=CARTESIAN_POINT ( 'NONE',  ( -5.000000000000003553, -8.660254037844383745, -70.37500000409677625 ) ) ;
#31508=CARTESIAN_POINT ( 'NONE',  ( 5.405949406249992428, -9.363379034771808662, -43.59375000204837391 ) ) ;
#31510=CARTESIAN_POINT ( 'NONE',  ( -10.81189881249999907, -6.242252689847864744, -2.156250002048373915 ) ) ;
#31512=CARTESIAN_POINT ( 'NONE',  ( -9.999999999999998224, 1.224646799147353059E-15, -61.24999999999997158 ) ) ;
#31514=CARTESIAN_POINT ( 'NONE',  ( 9.999999999999996447, -5.773502691896262640, -99.62500000000000000 ) ) ;
#31516=CARTESIAN_POINT ( 'NONE',  ( 5.000000000000000000, 8.660254037844385522, -102.6250000040967905 ) ) ;
#31517=EDGE_CURVE ( 'NONE', #16629, #33917, #34863, .T. ) ;
#31518=CARTESIAN_POINT ( 'NONE',  ( 7.070501591499376803E-16, 11.54700538379251284, -82.62500000000000000 ) ) ;
#31521=CARTESIAN_POINT ( 'NONE',  ( -5.405949406250003975, -9.363379034771801557, -99.53125000204839523 ) ) ;
#31522=EDGE_LOOP ( 'NONE', ( #30209, #21423, #20809, #23617 ) ) ;
#31524=CARTESIAN_POINT ( 'NONE',  ( 5.000000000000000000, 8.660254037844385522, -91.74999999999998579 ) ) ;
#31525=CARTESIAN_POINT ( 'NONE',  ( -5.405949406249996869, 9.363379034771805109, -155.5312500020484094 ) ) ;
#31527=ORIENTED_EDGE ( 'NONE', *, *, #38238, .T. ) ;
#31529=CARTESIAN_POINT ( 'NONE',  ( 10.00000000000000000, 5.773502691896255534, -24.37499999999998579 ) ) ;
#31530=CARTESIAN_POINT ( 'NONE',  ( -5.405949406249996869, 9.363379034771805109, -26.53125000204836681 ) ) ;
#31531=CARTESIAN_POINT ( 'NONE',  ( -9.999999999999998224, 1.224646799147353059E-15, -160.2500000000000000 ) ) ;
#31533=CARTESIAN_POINT ( 'NONE',  ( 9.999999999999998224, 0.000000000000000000, -200.0000000000000000 ) ) ;
#31534=CARTESIAN_POINT ( 'NONE',  ( -5.405949406250003975, -9.363379034771801557, -132.5312500020484094 ) ) ;
#31535=CARTESIAN_POINT ( 'NONE',  ( 7.070501591499376803E-16, 11.54700538379251284, -46.62499999999996447 ) ) ;
#31536=ADVANCED_FACE ( 'NONE', ( #7270 ), #27123, .T. ) ;
#31539=CARTESIAN_POINT ( 'NONE',  ( -2.293366432827344421E-15, -12.48450537969573659, -60.40625000204839523 ) ) ;
#31541=ORIENTED_EDGE ( 'NONE', *, *, #38726, .T. ) ;
#31542=ORIENTED_EDGE ( 'NONE', *, *, #32567, .T. ) ;
#31543=( BOUNDED_CURVE ( )  B_SPLINE_CURVE ( 2, ( #4728, #21561, #31505, #34742, #18742, #11404, #38388 ),
 .UNSPECIFIED., .F., .F. ) 
 B_SPLINE_CURVE_WITH_KNOTS ( ( 3, 2, 2, 3 ),
 ( 0.6380597014925374344, 0.6393034825870648197, 0.6405472636815923160, 0.6417910447761195902 ),
 .UNSPECIFIED. ) 
 CURVE ( )  GEOMETRIC_REPRESENTATION_ITEM ( )  RATIONAL_B_SPLINE_CURVE ( ( 0.9999999999999880096, 0.8660254037844506980, 1.000000000000000000, 0.8660254037844387076, 1.000000000000000000, 0.8660254037844148378, 1.000000000000023981 ) ) 
 REPRESENTATION_ITEM ( '' )  );
#31545=CARTESIAN_POINT ( 'NONE',  ( 7.070501591499376803E-16, 11.54700538379251284, -144.5000000040967905 ) ) ;
#31546=CARTESIAN_POINT ( 'NONE',  ( -5.405949406250003975, -9.363379034771801557, -154.8437500020483810 ) ) ;
#31548=CARTESIAN_POINT ( 'NONE',  ( 7.644554776091147741E-16, 12.48450537969573659, -9.968750002048363257 ) ) ;
#31549=CARTESIAN_POINT ( 'NONE',  ( 10.81189881249999551, -6.242252689847874514, -140.9687500020483810 ) ) ;
#31550=CARTESIAN_POINT ( 'NONE',  ( -10.81189881249999907, -6.242252689847864744, -96.65625000204839523 ) ) ;
#31552=CARTESIAN_POINT ( 'NONE',  ( -10.00000000000015987, 5.773502691896167605, -190.7500000040968757 ) ) ;
#31554=CARTESIAN_POINT ( 'NONE',  ( 10.81189881249999551, -6.242252689847874514, -2.968750002048361925 ) ) ;
#31556=CARTESIAN_POINT ( 'NONE',  ( 7.644554776091147741E-16, 12.48450537969573659, -194.6562500020484094 ) ) ;
#31560=EDGE_CURVE ( 'NONE', #6937, #31960, #39254, .T. ) ;
#31561=CARTESIAN_POINT ( 'NONE',  ( -2.293366432827344421E-15, -12.48450537969573659, -76.71875000204838102 ) ) ;
#31562=CARTESIAN_POINT ( 'NONE',  ( 10.81189881249999907, 6.242252689847868297, -58.21875000204836681 ) ) ;
#31564=CARTESIAN_POINT ( 'NONE',  ( 10.81189881249999551, -6.242252689847874514, -24.15625000204838102 ) ) ;
#31566=CARTESIAN_POINT ( 'NONE',  ( 9.999999999999998224, 0.000000000000000000, -171.8750000040968189 ) ) ;
#31568=CARTESIAN_POINT ( 'NONE',  ( 9.999999999999998224, 0.000000000000000000, -122.0000000000000000 ) ) ;
#31572=CARTESIAN_POINT ( 'NONE',  ( -10.81189881249999729, 1.324075727343319199E-15, -11.28125000204835438 ) ) ;
#31573=ORIENTED_EDGE ( 'NONE', *, *, #40425, .F. ) ;
#31578=CARTESIAN_POINT ( 'NONE',  ( -10.00000000000000000, -5.773502691896251982, -30.00000000409675494 ) ) ;
#31579=CARTESIAN_POINT ( 'NONE',  ( 10.00000000000051159, -5.773502691895965988, -2.500000004096743833 ) ) ;
#31581=DIRECTION ( 'NONE',  ( 0.000000000000000000, 0.000000000000000000, -1.000000000000000000 ) ) ;
#31582=CARTESIAN_POINT ( 'NONE',  ( 7.644554776091147741E-16, 12.48450537969573659, -143.6562500020484094 ) ) ;
#31583=CARTESIAN_POINT ( 'NONE',  ( 5.405949406249999534, 9.363379034771803333, -128.5937500020483810 ) ) ;
#31584=LINE ( 'NONE', #34820, #15817 ) ;
#31586=ORIENTED_EDGE ( 'NONE', *, *, #40946, .F. ) ;
#31587=( BOUNDED_CURVE ( )  B_SPLINE_CURVE ( 2, ( #34268, #5328, #8146, #18051, #4684, #18483, #31246 ),
 .UNSPECIFIED., .F., .F. ) 
 B_SPLINE_CURVE_WITH_KNOTS ( ( 3, 2, 2, 3 ),
 ( 0.1343283582089551953, 0.1355721393034825528, 0.1368159203980099381, 0.1380597014925373234 ),
 .UNSPECIFIED. ) 
 CURVE ( )  GEOMETRIC_REPRESENTATION_ITEM ( )  RATIONAL_B_SPLINE_CURVE ( ( 1.000000000000003109, 0.8660254037844358210, 1.000000000000000000, 0.8660254037844387076, 1.000000000000000000, 0.8660254037844387076, 1.000000000000000000 ) ) 
 REPRESENTATION_ITEM ( '' )  );
#31588=ORIENTED_EDGE ( 'NONE', *, *, #30717, .F. ) ;
#31589=VECTOR ( 'NONE', #41972, 1000.000000000000000 ) ;
#31590=ORIENTED_EDGE ( 'NONE', *, *, #14281, .F. ) ;
#31591=DIRECTION ( 'NONE',  ( -0.000000000000000000, -0.000000000000000000, 1.000000000000000000 ) ) ;
#31592=CARTESIAN_POINT ( 'NONE',  ( -10.81189881249999907, -6.242252689847864744, -183.4687500020484379 ) ) ;
#31593=CARTESIAN_POINT ( 'NONE',  ( 5.405949406249999534, 9.363379034771803333, -32.59375000204836681 ) ) ;
#31594=CARTESIAN_POINT ( 'NONE',  ( -2.121150477449813534E-15, -11.54700538379251284, -41.37499999999997158 ) ) ;
#31595=CARTESIAN_POINT ( 'NONE',  ( 10.81189881249999551, -6.242252689847874514, -175.4687500020484094 ) ) ;
#31596=CARTESIAN_POINT ( 'NONE',  ( 10.81189881249999907, 6.242252689847868297, -155.7187500020483810 ) ) ;
#31597=CYLINDRICAL_SURFACE ( 'NONE', #10712, 9.999999999999998224 ) ;
#31601=LINE ( 'NONE', #31823, #11593 ) ;
#31602=CARTESIAN_POINT ( 'NONE',  ( 5.000000000000000000, 8.660254037844385522, -169.7500000000000000 ) ) ;
#31604=ADVANCED_FACE ( 'NONE', ( #36828 ), #30374, .T. ) ;
#31605=CARTESIAN_POINT ( 'NONE',  ( 10.81189881249999729, 0.000000000000000000, -82.34375000204836681 ) ) ;
#31607=CARTESIAN_POINT ( 'NONE',  ( 5.405949406249999534, 9.363379034771803333, -56.78125000204836681 ) ) ;
#31610=CARTESIAN_POINT ( 'NONE',  ( -2.293366432827344421E-15, -12.48450537969573659, -114.4062500020483952 ) ) ;
#31611=CARTESIAN_POINT ( 'NONE',  ( -5.405949406249996869, 9.363379034771805109, -145.0312500020483810 ) ) ;
#31612=CARTESIAN_POINT ( 'NONE',  ( 5.000000000000000000, 8.660254037844385522, -143.1250000040967905 ) ) ;
#31614=CARTESIAN_POINT ( 'NONE',  ( 4.999999999999992006, -8.660254037844389075, -122.6250000040967905 ) ) ;
#31619=CARTESIAN_POINT ( 'NONE',  ( -4.999999999999996447, 8.660254037844387298, -192.3750000040967905 ) ) ;
#31620=CARTESIAN_POINT ( 'NONE',  ( 10.81189881249999907, 6.242252689847868297, -176.9062500020484094 ) ) ;
#31623=CARTESIAN_POINT ( 'NONE',  ( 4.999999999999992006, -8.660254037844389075, -47.62500000409677625 ) ) ;
#31624=AXIS2_PLACEMENT_3D ( 'NONE', #40746, #27606, #31500 ) ;
#31625=CARTESIAN_POINT ( 'NONE',  ( 0.000000000000000000, 0.000000000000000000, -200.0000000000000000 ) ) ;
#31628=EDGE_CURVE ( 'NONE', #30921, #2425, #40265, .T. ) ;
#31632=CARTESIAN_POINT ( 'NONE',  ( 10.81189881249999907, 6.242252689847868297, -170.9062500020484094 ) ) ;
#31633=DIRECTION ( 'NONE',  ( -0.4999999999999997224, -0.8660254037844388186, 0.000000000000000000 ) ) ;
#31634=CARTESIAN_POINT ( 'NONE',  ( 5.000000000000000000, 8.660254037844385522, -64.74999999999997158 ) ) ;
#31636=CARTESIAN_POINT ( 'NONE',  ( -9.999999999999998224, 1.224646799147353059E-15, -1.249999999999973355 ) ) ;
#31637=CARTESIAN_POINT ( 'NONE',  ( 9.999999999999742428, 5.773502691896404748, -123.7500000040967763 ) ) ;
#31638=CARTESIAN_POINT ( 'NONE',  ( 5.405949406249992428, -9.363379034771808662, -76.78125000204838102 ) ) ;
#31641=CARTESIAN_POINT ( 'NONE',  ( -5.000000000000003553, -8.660254037844383745, -188.8750000040967905 ) ) ;
#31642=EDGE_LOOP ( 'NONE', ( #3581, #14918, #30336, #30186 ) ) ;
#31643=VERTEX_POINT ( 'NONE', #3827 ) ;
#31644=CARTESIAN_POINT ( 'NONE',  ( -5.405949406250003975, -9.363379034771801557, -25.84375000204835970 ) ) ;
#31646=CARTESIAN_POINT ( 'NONE',  ( 10.81189881249999729, 0.000000000000000000, -7.531250002048350822 ) ) ;
#31647=CARTESIAN_POINT ( 'NONE',  ( -2.293366432827344421E-15, -12.48450537969573659, -55.71875000204837391 ) ) ;
#31648=ORIENTED_EDGE ( 'NONE', *, *, #28081, .F. ) ;
#31650=AXIS2_PLACEMENT_3D ( 'NONE', #17719, #20757, #30702 ) ;
#31651=CARTESIAN_POINT ( 'NONE',  ( -5.405949406249996869, 9.363379034771805109, -195.8437500020484094 ) ) ;
#31652=CARTESIAN_POINT ( 'NONE',  ( 10.81189881249999729, 0.000000000000000000, -179.8437500020483810 ) ) ;
#31656=LINE ( 'NONE', #28629, #12965 ) ;
#31659=CARTESIAN_POINT ( 'NONE',  ( 10.81189881249999729, 0.000000000000000000, -106.3437500020483810 ) ) ;
#31660=CARTESIAN_POINT ( 'NONE',  ( 9.999999999999998224, 0.000000000000000000, -191.3750000040967905 ) ) ;
#31661=CARTESIAN_POINT ( 'NONE',  ( -10.81189881249999729, 1.324075727343319199E-15, -80.28125000204838102 ) ) ;
#31662=CARTESIAN_POINT ( 'NONE',  ( -10.81189881249999729, 6.242252689847871849, -93.71875000204838102 ) ) ;
#31664=CARTESIAN_POINT ( 'NONE',  ( -10.00000000000000000, -5.773502691896251982, -142.5000000040967905 ) ) ;
#31667=AXIS2_PLACEMENT_3D ( 'NONE', #22727, #35892, #6329 ) ;
#31670=CARTESIAN_POINT ( 'NONE',  ( 4.999999999999992006, -8.660254037844389075, -39.74999999999997868 ) ) ;
#31671=CYLINDRICAL_SURFACE ( 'NONE', #17137, 9.999999999999998224 ) ;
#31673=ORIENTED_EDGE ( 'NONE', *, *, #14492, .T. ) ;
#31674=CARTESIAN_POINT ( 'NONE',  ( 9.999999999999998224, 0.000000000000000000, -67.99999999999997158 ) ) ;
#31676=CARTESIAN_POINT ( 'NONE',  ( -10.00000000000000000, -5.773502691896251982, -79.50000000409679046 ) ) ;
#31678=CARTESIAN_POINT ( 'NONE',  ( 0.000000000000000000, 0.000000000000000000, -200.0000000000000000 ) ) ;
#31680=CARTESIAN_POINT ( 'NONE',  ( -10.81189881249999729, 6.242252689847871849, -78.90625000204838102 ) ) ;
#31682=CYLINDRICAL_SURFACE ( 'NONE', #36917, 9.999999999999998224 ) ;
#31684=ORIENTED_EDGE ( 'NONE', *, *, #25451, .F. ) ;
#31685=CARTESIAN_POINT ( 'NONE',  ( -10.81189881249999729, 6.242252689847871849, -194.4062500020484094 ) ) ;
#31688=CARTESIAN_POINT ( 'NONE',  ( 10.81189881249999729, 6.242252689847867408, -4.218750002048367698 ) ) ;
#31689=CARTESIAN_POINT ( 'NONE',  ( 4.999999999999992006, -8.660254037844389075, -64.12500000409676204 ) ) ;
#31690=CARTESIAN_POINT ( 'NONE',  ( -5.405949406249996869, 9.363379034771805109, -144.8437500020483810 ) ) ;
#31691=CARTESIAN_POINT ( 'NONE',  ( -2.121150477449813534E-15, -11.54700538379251284, -180.8749999999999432 ) ) ;
#31692=CARTESIAN_POINT ( 'NONE',  ( 9.999999999999994671, -5.773502691896262640, -137.1250000000000000 ) ) ;
#31693=CARTESIAN_POINT ( 'NONE',  ( 4.999999999999992006, -8.660254037844389075, -171.7500000000000000 ) ) ;
#31694=CARTESIAN_POINT ( 'NONE',  ( -9.999999999999998224, 1.224646799147353059E-15, -157.6250000040967905 ) ) ;
#31695=AXIS2_PLACEMENT_3D ( 'NONE', #11749, #8106, #996 ) ;
#31696=CARTESIAN_POINT ( 'NONE',  ( 7.644554776091147741E-16, 12.48450537969573659, -100.1562500020483952 ) ) ;
#31699=ORIENTED_EDGE ( 'NONE', *, *, #15901, .T. ) ;
#31700=ORIENTED_EDGE ( 'NONE', *, *, #27310, .F. ) ;
#31702=CARTESIAN_POINT ( 'NONE',  ( -10.81189881249999907, -6.242252689847864744, -29.15625000204835970 ) ) ;
#31704=CARTESIAN_POINT ( 'NONE',  ( 5.405949406249999534, 9.363379034771803333, -91.09375000204838102 ) ) ;
#31705=CYLINDRICAL_SURFACE ( 'NONE', #37358, 9.999999999999998224 ) ;
#31707=( BOUNDED_CURVE ( )  B_SPLINE_CURVE ( 2, ( #9218, #6204, #2338, #42641, #41797, #12860, #15467 ),
 .UNSPECIFIED., .F., .F. ) 
 B_SPLINE_CURVE_WITH_KNOTS ( ( 3, 2, 2, 3 ),
 ( 0.9850746268656718208, 0.9863184079601992060, 0.9875621890547265913, 0.9888059701492539766 ),
 .UNSPECIFIED. ) 
 CURVE ( )  GEOMETRIC_REPRESENTATION_ITEM ( )  RATIONAL_B_SPLINE_CURVE ( ( 0.9999999999999761302, 0.8660254037844625774, 1.000000000000000000, 0.8660254037844387076, 1.000000000000000000, 0.8660254037844148378, 1.000000000000023981 ) ) 
 REPRESENTATION_ITEM ( '' )  );
#31710=CARTESIAN_POINT ( 'NONE',  ( -5.000000000000003553, -8.660254037844383745, -10.37500000409674605 ) ) ;
#31712=CARTESIAN_POINT ( 'NONE',  ( 10.81189881249999729, 0.000000000000000000, -113.8437500020483810 ) ) ;
#31716=CARTESIAN_POINT ( 'NONE',  ( 9.999999999999998224, 0.000000000000000000, -179.3750000040967905 ) ) ;
#31717=CARTESIAN_POINT ( 'NONE',  ( 5.405949406249992428, -9.363379034771808662, -171.2812500020484094 ) ) ;
#31718=( BOUNDED_CURVE ( )  B_SPLINE_CURVE ( 2, ( #34467, #17388, #7917, #33823, #17819, #37690, #24761 ),
 .UNSPECIFIED., .F., .F. ) 
 B_SPLINE_CURVE_WITH_KNOTS ( ( 3, 2, 2, 3 ),
 ( 0.4738805970149255198, 0.4751243781094529051, 0.4763681592039803459, 0.4776119402985076756 ),
 .UNSPECIFIED. ) 
 CURVE ( )  GEOMETRIC_REPRESENTATION_ITEM ( )  RATIONAL_B_SPLINE_CURVE ( ( 0.9999999999999820144, 0.8660254037844566932, 1.000000000000000000, 0.8660254037844387076, 1.000000000000000000, 0.8660254037844148378, 1.000000000000023981 ) ) 
 REPRESENTATION_ITEM ( '' )  );
#31722=CARTESIAN_POINT ( 'NONE',  ( -5.405949406250003975, -9.363379034771801557, -43.84375000204837391 ) ) ;
#31723=VECTOR ( 'NONE', #36442, 1000.000000000000000 ) ;
#31725=CARTESIAN_POINT ( 'NONE',  ( -5.405949406249996869, 9.363379034771805109, -2.531250002048373915 ) ) ;
#31727=CARTESIAN_POINT ( 'NONE',  ( -9.999999999999998224, 1.224646799147353059E-15, -200.0000000000000000 ) ) ;
#31729=CARTESIAN_POINT ( 'NONE',  ( 7.070501591499377789E-16, 11.54700538379251284, -91.62500000000000000 ) ) ;
#31731=CARTESIAN_POINT ( 'NONE',  ( -10.00000000000000000, -5.773502691896251982, -108.0000000040967763 ) ) ;
#31732=DIRECTION ( 'NONE',  ( 1.000000000000000000, 0.000000000000000000, 0.000000000000000000 ) ) ;
#31735=CARTESIAN_POINT ( 'NONE',  ( 7.644554776091147741E-16, 12.48450537969573659, -98.65625000204838102 ) ) ;
#31736=ORIENTED_EDGE ( 'NONE', *, *, #20349, .T. ) ;
#31740=CARTESIAN_POINT ( 'NONE',  ( 5.405949406249992428, -9.363379034771808662, -154.7812500020484094 ) ) ;
#31742=ORIENTED_EDGE ( 'NONE', *, *, #31227, .T. ) ;
#31743=CARTESIAN_POINT ( 'NONE',  ( 9.999999999999996447, -5.773502691896262640, -20.12499999999996803 ) ) ;
#31744=EDGE_CURVE ( 'NONE', #25635, #1542, #37249, .T. ) ;
#31745=CARTESIAN_POINT ( 'NONE',  ( 10.81189881249999551, -6.242252689847874514, -28.65625000204838813 ) ) ;
#31746=CARTESIAN_POINT ( 'NONE',  ( 9.999999999999998224, 0.000000000000000000, -155.0000000000000000 ) ) ;
#31748=EDGE_CURVE ( 'NONE', #18719, #38940, #28815, .T. ) ;
#31749=CARTESIAN_POINT ( 'NONE',  ( -9.999999999998969713, -5.773502691896847949, -34.12499999999995026 ) ) ;
#31750=CARTESIAN_POINT ( 'NONE',  ( 10.81189881249999551, -6.242252689847874514, -124.6562500020483952 ) ) ;
#31751=CARTESIAN_POINT ( 'NONE',  ( -4.999999999999996447, 8.660254037844387298, -117.3750000040967905 ) ) ;
#31752=CARTESIAN_POINT ( 'NONE',  ( 23.09401076758504345, 1.040834085586084257E-14, 45.00000000000009237 ) ) ;
#31753=ORIENTED_EDGE ( 'NONE', *, *, #4039, .F. ) ;
#31754=CARTESIAN_POINT ( 'NONE',  ( -5.405949406250003975, -9.363379034771801557, -53.03125000204836681 ) ) ;
#31756=CARTESIAN_POINT ( 'NONE',  ( -10.81189881249999907, -6.242252689847864744, -108.4687500020483810 ) ) ;
#31760=DIRECTION ( 'NONE',  ( -0.000000000000000000, -0.000000000000000000, 1.000000000000000000 ) ) ;
#31762=CARTESIAN_POINT ( 'NONE',  ( -5.405949406249996869, 9.363379034771805109, -158.3437500020483810 ) ) ;
#31764=CARTESIAN_POINT ( 'NONE',  ( 5.405949406249992428, -9.363379034771808662, -6.093750002048370362 ) ) ;
#31765=EDGE_CURVE ( 'NONE', #40867, #13705, #30693, .T. ) ;
#31766=CARTESIAN_POINT ( 'NONE',  ( -10.81189881249999729, 6.242252689847871849, -138.7187500020483810 ) ) ;
#31770=CARTESIAN_POINT ( 'NONE',  ( 10.81189881249999907, 6.242252689847868297, -1.218750002048353709 ) ) ;
#31772=CARTESIAN_POINT ( 'NONE',  ( -2.293366432827344421E-15, -12.48450537969573659, -193.9062500020484094 ) ) ;
#31773=CARTESIAN_POINT ( 'NONE',  ( 9.999999999998969713, 5.773502691896851502, -12.37499999999993783 ) ) ;
#31776=CARTESIAN_POINT ( 'NONE',  ( -10.81189881249999729, 1.324075727343319199E-15, -71.09375000204836681 ) ) ;
#31777=CARTESIAN_POINT ( 'NONE',  ( 5.405949406249999534, 9.363379034771803333, -53.59375000204835970 ) ) ;
#31779=CARTESIAN_POINT ( 'NONE',  ( -2.293366432827344421E-15, -12.48450537969573659, -28.90625000204835615 ) ) ;
#31781=CARTESIAN_POINT ( 'NONE',  ( 5.000000000000000000, 8.660254037844385522, -32.12500000409676204 ) ) ;
#31783=CARTESIAN_POINT ( 'NONE',  ( 5.000000000000000000, 8.660254037844385522, -111.2499999999999858 ) ) ;
#31784=CARTESIAN_POINT ( 'NONE',  ( -9.999999999999998224, 1.224646799147353059E-15, -170.7500000000000000 ) ) ;
#31787=CARTESIAN_POINT ( 'NONE',  ( -2.293366432827344421E-15, -12.48450537969573659, -9.406250002048377468 ) ) ;
#31788=EDGE_LOOP ( 'NONE', ( #31736, #19071, #4870, #11486 ) ) ;
#31789=CARTESIAN_POINT ( 'NONE',  ( 9.999999999999742428, 5.773502691896404748, -121.8750000000000142 ) ) ;
#31793=CARTESIAN_POINT ( 'NONE',  ( -2.121150477449813534E-15, -11.54700538379251284, -47.37499999999997158 ) ) ;
#31795=CARTESIAN_POINT ( 'NONE',  ( 4.999999999999992006, -8.660254037844389075, -23.62500000409675849 ) ) ;
#31796=ADVANCED_FACE ( 'NONE', ( #1441 ), #11127, .T. ) ;
#31797=AXIS2_PLACEMENT_3D ( 'NONE', #8952, #19080, #22115 ) ;
#31800=EDGE_CURVE ( 'NONE', #42167, #35094, #947, .T. ) ;
#31801=CARTESIAN_POINT ( 'NONE',  ( 0.000000000000000000, 0.000000000000000000, -200.0000000000000000 ) ) ;
#31802=CARTESIAN_POINT ( 'NONE',  ( -2.293366432827344421E-15, -12.48450537969573659, -145.9062500020484094 ) ) ;
#31803=EDGE_CURVE ( 'NONE', #15042, #4157, #39507, .T. ) ;
#31804=CARTESIAN_POINT ( 'NONE',  ( -5.405949406250003975, -9.363379034771801557, -152.0312500020484094 ) ) ;
#31805=CARTESIAN_POINT ( 'NONE',  ( -10.00000000000051337, 5.773502691895962435, -78.25000000409677625 ) ) ;
#31808=ORIENTED_EDGE ( 'NONE', *, *, #10072, .F. ) ;
#31811=EDGE_CURVE ( 'NONE', #2913, #6874, #2345, .T. ) ;
#31813=CARTESIAN_POINT ( 'NONE',  ( 9.999999999999998224, 0.000000000000000000, -6.875000004096742501 ) ) ;
#31814=CARTESIAN_POINT ( 'NONE',  ( 10.81189881249999551, -6.242252689847874514, -178.4687500020484094 ) ) ;
#31816=CARTESIAN_POINT ( 'NONE',  ( 7.644554776091147741E-16, 12.48450537969573659, -27.96875000204838457 ) ) ;
#31817=CARTESIAN_POINT ( 'NONE',  ( -5.405949406250003975, -9.363379034771801557, -166.8437500020484094 ) ) ;
#31818=CARTESIAN_POINT ( 'NONE',  ( 7.644554776091147741E-16, 12.48450537969573659, -149.4687500020484094 ) ) ;
#31819=CARTESIAN_POINT ( 'NONE',  ( 0.000000000000000000, 0.000000000000000000, -200.0000000000000000 ) ) ;
#31823=CARTESIAN_POINT ( 'NONE',  ( -9.999999999999998224, 1.224646799147353059E-15, -200.0000000000000000 ) ) ;
#31825=CARTESIAN_POINT ( 'NONE',  ( -5.405949406250003975, -9.363379034771801557, -81.34375000204838102 ) ) ;
#31826=DIRECTION ( 'NONE',  ( 1.000000000000000000, 0.000000000000000000, 0.000000000000000000 ) ) ;
#31827=CARTESIAN_POINT ( 'NONE',  ( -5.405949406250003975, -9.363379034771801557, -51.53125000204835970 ) ) ;
#31828=CARTESIAN_POINT ( 'NONE',  ( -9.999999999999998224, 1.224646799147353059E-15, -37.62500000409676915 ) ) ;
#31830=CARTESIAN_POINT ( 'NONE',  ( -5.405949406249996869, 9.363379034771805109, -115.0312500020483952 ) ) ;
#31831=CARTESIAN_POINT ( 'NONE',  ( -10.81189881249999729, 1.324075727343319199E-15, -147.7812500020483810 ) ) ;
#31834=CARTESIAN_POINT ( 'NONE',  ( -5.000000000000003553, -8.660254037844383745, -124.3750000040967763 ) ) ;
#31836=VERTEX_POINT ( 'NONE', #28201 ) ;
#31839=CARTESIAN_POINT ( 'NONE',  ( -4.999999999999996447, 8.660254037844387298, -184.5000000000000000 ) ) ;
#31840=CARTESIAN_POINT ( 'NONE',  ( 10.81189881249999907, 6.242252689847868297, -181.4062500020484379 ) ) ;
#31841=ORIENTED_EDGE ( 'NONE', *, *, #25690, .T. ) ;
#31842=CARTESIAN_POINT ( 'NONE',  ( -9.999999999999998224, 5.773502691896259087, -52.75000000409676915 ) ) ;
#31843=CARTESIAN_POINT ( 'NONE',  ( 9.999999999999998224, 0.000000000000000000, -87.87500000409677625 ) ) ;
#31845=AXIS2_PLACEMENT_3D ( 'NONE', #1284, #20478, #37314 ) ;
#31846=( BOUNDED_CURVE ( )  B_SPLINE_CURVE ( 2, ( #32969, #23468, #388, #33611, #19996, #599, #19782 ),
 .UNSPECIFIED., .F., .F. ) 
 B_SPLINE_CURVE_WITH_KNOTS ( ( 3, 2, 2, 3 ),
 ( 0.3283582089552238847, 0.3296019900497513255, 0.3308457711442787108, 0.3320895522388061516 ),
 .UNSPECIFIED. ) 
 CURVE ( )  GEOMETRIC_REPRESENTATION_ITEM ( )  RATIONAL_B_SPLINE_CURVE ( ( 1.000000000000000000, 0.8660254037844387076, 1.000000000000000000, 0.8660254037844387076, 1.000000000000000000, 0.8660254037844207220, 1.000000000000017986 ) ) 
 REPRESENTATION_ITEM ( '' )  );
#31848=CARTESIAN_POINT ( 'NONE',  ( 10.81189881249999907, 6.242252689847868297, -167.9062500020484094 ) ) ;
#31849=CARTESIAN_POINT ( 'NONE',  ( 10.81189881249999729, 0.000000000000000000, -114.0312500020483952 ) ) ;
#31851=CARTESIAN_POINT ( 'NONE',  ( -9.999999999999998224, 1.224646799147353059E-15, -56.74999999999996447 ) ) ;
#31852=ORIENTED_EDGE ( 'NONE', *, *, #11564, .F. ) ;
#31853=CARTESIAN_POINT ( 'NONE',  ( 9.999999999999998224, 0.000000000000000000, -17.37500000409675138 ) ) ;
#31855=CARTESIAN_POINT ( 'NONE',  ( 0.000000000000000000, 0.000000000000000000, -200.0000000000000000 ) ) ;
#31856=VECTOR ( 'NONE', #11736, 1000.000000000000000 ) ;
#31857=EDGE_CURVE ( 'NONE', #8912, #6661, #41335, .T. ) ;
#31858=CARTESIAN_POINT ( 'NONE',  ( -10.81189881249999729, 1.324075727343319199E-15, -77.28125000204838102 ) ) ;
#31860=CARTESIAN_POINT ( 'NONE',  ( 9.999999999999998224, 0.000000000000000000, -39.49999999999997868 ) ) ;
#31862=ORIENTED_EDGE ( 'NONE', *, *, #6705, .F. ) ;
#31863=CARTESIAN_POINT ( 'NONE',  ( -10.81189881249999729, 1.324075727343319199E-15, -32.09375000204836681 ) ) ;
#31864=CARTESIAN_POINT ( 'NONE',  ( 9.999999999999479527, 5.773502691896553074, -77.25000000409676204 ) ) ;
#31865=CARTESIAN_POINT ( 'NONE',  ( 10.81189881249999551, -6.242252689847874514, -3.156250002048346381 ) ) ;
#31866=CARTESIAN_POINT ( 'NONE',  ( -5.405949406250003975, -9.363379034771801557, -58.84375000204835970 ) ) ;
#31867=ORIENTED_EDGE ( 'NONE', *, *, #35558, .F. ) ;
#31870=CARTESIAN_POINT ( 'NONE',  ( 5.405949406249999534, 9.363379034771803333, -191.5937500020484094 ) ) ;
#31871=CARTESIAN_POINT ( 'NONE',  ( 10.81189881249999729, 0.000000000000000000, -176.8437500020483810 ) ) ;
#31875=CARTESIAN_POINT ( 'NONE',  ( 5.000000000000000000, 8.660254037844385522, -18.62500000409675494 ) ) ;
#31876=CARTESIAN_POINT ( 'NONE',  ( -5.000000000000003553, -8.660254037844383745, -24.99999999999996803 ) ) ;
#31878=CARTESIAN_POINT ( 'NONE',  ( 10.81189881249999729, 0.000000000000000000, -104.8437500020483810 ) ) ;
#31879=CARTESIAN_POINT ( 'NONE',  ( -4.999999999999996447, 8.660254037844387298, -17.99999999999996092 ) ) ;
#31880=CARTESIAN_POINT ( 'NONE',  ( -2.293366432827344421E-15, -12.48450537969573659, -70.90625000204839523 ) ) ;
#31881=CARTESIAN_POINT ( 'NONE',  ( -10.81189881249999729, -6.242252689847864744, -93.46875000204838102 ) ) ;
#31883=CARTESIAN_POINT ( 'NONE',  ( -5.000000000000003553, -8.660254037844383745, -142.3750000040967905 ) ) ;
#31889=CARTESIAN_POINT ( 'NONE',  ( -2.121150477449813534E-15, -11.54700538379251284, -13.25000000409675849 ) ) ;
#31892=ORIENTED_EDGE ( 'NONE', *, *, #24647, .T. ) ;
#31893=CARTESIAN_POINT ( 'NONE',  ( -4.999999999999996447, 8.660254037844387298, -68.99999999999997158 ) ) ;
#31895=CARTESIAN_POINT ( 'NONE',  ( 7.070501591499377789E-16, 11.54700538379251284, -75.50000000409677625 ) ) ;
#31897=CARTESIAN_POINT ( 'NONE',  ( 9.999999999999998224, 0.000000000000000000, -200.0000000000000000 ) ) ;
#31899=CARTESIAN_POINT ( 'NONE',  ( -2.293366432827344421E-15, -12.48450537969573659, -66.40625000204839523 ) ) ;
#31902=VERTEX_POINT ( 'NONE', #32289 ) ;
#31903=CARTESIAN_POINT ( 'NONE',  ( 10.81189881249999551, -6.242252689847874514, -196.6562500020484379 ) ) ;
#31905=CARTESIAN_POINT ( 'NONE',  ( -5.405949406249996869, 9.363379034771805109, -5.343750002048369474 ) ) ;
#31907=CARTESIAN_POINT ( 'NONE',  ( -9.999999999999998224, 1.224646799147353059E-15, -191.7500000000000000 ) ) ;
#31908=CARTESIAN_POINT ( 'NONE',  ( 9.999999999999866773, -5.773502691896336358, -173.1250000000000000 ) ) ;
#31909=EDGE_CURVE ( 'NONE', #17345, #16464, #15637, .T. ) ;
#31910=CARTESIAN_POINT ( 'NONE',  ( 5.000000000000000000, 8.660254037844385522, -177.2500000000000284 ) ) ;
#31911=CARTESIAN_POINT ( 'NONE',  ( 10.00000000000051159, -5.773502691895965988, -36.62499999999995026 ) ) ;
#31912=CARTESIAN_POINT ( 'NONE',  ( -10.81189881249999729, 6.242252689847871849, -104.4062500020483810 ) ) ;
#31913=VERTEX_POINT ( 'NONE', #34891 ) ;
#31914=ORIENTED_EDGE ( 'NONE', *, *, #25479, .T. ) ;
#31915=ORIENTED_EDGE ( 'NONE', *, *, #20645, .T. ) ;
#31916=CARTESIAN_POINT ( 'NONE',  ( -10.81189881249999729, 6.242252689847871849, -32.40625000204835970 ) ) ;
#31919=CARTESIAN_POINT ( 'NONE',  ( 10.81189881249999729, 0.000000000000000000, -76.34375000204838102 ) ) ;
#31920=DIRECTION ( 'NONE',  ( 1.000000000000000000, 0.000000000000000000, 0.000000000000000000 ) ) ;
#31921=EDGE_CURVE ( 'NONE', #29474, #20834, #22559, .T. ) ;
#31925=CARTESIAN_POINT ( 'NONE',  ( -9.999999999999998224, 5.773502691896259087, -10.75000000409676204 ) ) ;
#31926=CARTESIAN_POINT ( 'NONE',  ( 10.00000000000003020, -5.773502691896243988, -198.6250000000000284 ) ) ;
#31927=CARTESIAN_POINT ( 'NONE',  ( -5.405949406250003975, -9.363379034771801557, -130.8437500020484094 ) ) ;
#31928=CARTESIAN_POINT ( 'NONE',  ( 5.405949406249992428, -9.363379034771808662, -114.0937500020483810 ) ) ;
#31932=CARTESIAN_POINT ( 'NONE',  ( -2.121150477449813534E-15, -11.54700538379251284, -169.2500000040967620 ) ) ;
#31933=CARTESIAN_POINT ( 'NONE',  ( -10.81189881249999729, -6.242252689847864744, -170.1562500020484094 ) ) ;
#31934=CARTESIAN_POINT ( 'NONE',  ( -4.999999999999996447, 8.660254037844387298, -68.99999999999997158 ) ) ;
#31937=CARTESIAN_POINT ( 'NONE',  ( 5.405949406249999534, 9.363379034771803333, -46.09375000204838102 ) ) ;
#31939=CARTESIAN_POINT ( 'NONE',  ( 5.405949406249999534, 9.363379034771803333, 0.2187499979516283055 ) ) ;
#31942=CARTESIAN_POINT ( 'NONE',  ( 9.999999999999998224, 0.000000000000000000, -85.99999999999998579 ) ) ;
#31944=CARTESIAN_POINT ( 'NONE',  ( 4.999999999999992006, -8.660254037844389075, -98.62500000409677625 ) ) ;
#31945=CARTESIAN_POINT ( 'NONE',  ( 10.00000000000051159, -5.773502691895965988, -149.5000000040967905 ) ) ;
#31947=CARTESIAN_POINT ( 'NONE',  ( 7.644554776091147741E-16, 12.48450537969573659, -101.6562500020483952 ) ) ;
#31951=CARTESIAN_POINT ( 'NONE',  ( -5.405949406250003975, -9.363379034771801557, -156.5312500020484094 ) ) ;
#31953=ORIENTED_EDGE ( 'NONE', *, *, #27778, .T. ) ;
#31954=CARTESIAN_POINT ( 'NONE',  ( 10.00000000000000000, 5.773502691896255534, -16.87499999999996803 ) ) ;
#31955=CARTESIAN_POINT ( 'NONE',  ( -10.81189881249999729, 1.324075727343319199E-15, -26.28125000204836681 ) ) ;
#31956=CARTESIAN_POINT ( 'NONE',  ( 7.070501591499377789E-16, 11.54700538379251284, -154.6250000000000284 ) ) ;
#31959=CARTESIAN_POINT ( 'NONE',  ( -10.81189881249999729, 6.242252689847871849, -129.9062500020483810 ) ) ;
#31960=VERTEX_POINT ( 'NONE', #38533 ) ;
#31961=CARTESIAN_POINT ( 'NONE',  ( -10.00000000000102496, 5.773502691895664007, -64.75000000409674783 ) ) ;
#31962=CARTESIAN_POINT ( 'NONE',  ( 9.999999999999998224, 0.000000000000000000, -188.0000000000000000 ) ) ;
#31963=VERTEX_POINT ( 'NONE', #2713 ) ;
#31964=SHAPE_REPRESENTATION ( 'thrust bolt', ( #39998 ), #15874 ) ;
#31965=CARTESIAN_POINT ( 'NONE',  ( -2.293366432827344421E-15, -12.48450537969573659, -55.90625000204837391 ) ) ;
#31967=CARTESIAN_POINT ( 'NONE',  ( 10.81189881249999551, -6.242252689847874514, -101.9687500020483810 ) ) ;
#31969=ORIENTED_EDGE ( 'NONE', *, *, #42334, .T. ) ;
#31970=CARTESIAN_POINT ( 'NONE',  ( 4.999999999999992006, -8.660254037844389075, -175.1250000040968189 ) ) ;
#31971=CARTESIAN_POINT ( 'NONE',  ( 10.81189881249999907, 6.242252689847868297, -158.7187500020483810 ) ) ;
#31973=CARTESIAN_POINT ( 'NONE',  ( -5.405949406249996869, 9.363379034771805109, -8.343750002048345493 ) ) ;
#31974=CARTESIAN_POINT ( 'NONE',  ( 0.000000000000000000, 0.000000000000000000, -200.0000000000000000 ) ) ;
#31975=EDGE_CURVE ( 'NONE', #39731, #1094, #36233, .T. ) ;
#31976=CARTESIAN_POINT ( 'NONE',  ( 7.644554776091147741E-16, 12.48450537969573659, -138.9687500020483810 ) ) ;
#31977=EDGE_CURVE ( 'NONE', #2291, #30470, #18898, .T. ) ;
#31981=CARTESIAN_POINT ( 'NONE',  ( 10.00000000000000000, 5.773502691896255534, -192.7500000040968189 ) ) ;
#31983=CARTESIAN_POINT ( 'NONE',  ( 5.405949406249999534, 9.363379034771803333, -193.2812500020484094 ) ) ;
#31987=CARTESIAN_POINT ( 'NONE',  ( -10.81189881249999729, 1.324075727343319199E-15, -66.59375000204836681 ) ) ;
#31988=CARTESIAN_POINT ( 'NONE',  ( -10.81189881249999907, -6.242252689847864744, -58.96875000204836681 ) ) ;
#31990=CARTESIAN_POINT ( 'NONE',  ( 10.81189881249999907, 6.242252689847868297, -23.90625000204838102 ) ) ;
#31992=CARTESIAN_POINT ( 'NONE',  ( -10.00000000000051337, 5.773502691895962435, -31.75000000409674072 ) ) ;
#31994=CARTESIAN_POINT ( 'NONE',  ( -9.999999999999998224, 5.773502691896259087, -115.3749999999999858 ) ) ;
#31998=CARTESIAN_POINT ( 'NONE',  ( -10.81189881249999729, 1.324075727343319199E-15, -9.781250002048352599 ) ) ;
#31999=ORIENTED_EDGE ( 'NONE', *, *, #41978, .F. ) ;
#32000=CARTESIAN_POINT ( 'NONE',  ( 9.999999999999998224, 0.000000000000000000, -200.0000000000000000 ) ) ;
#32002=CARTESIAN_POINT ( 'NONE',  ( 10.00000000000102318, -5.773502691895667560, -38.50000000409673362 ) ) ;
#32004=CARTESIAN_POINT ( 'NONE',  ( 5.000000000000000000, 8.660254037844385522, -40.74999999999997868 ) ) ;
#32005=CARTESIAN_POINT ( 'NONE',  ( 4.999999999999992006, -8.660254037844389075, -26.62500000409676204 ) ) ;
#32006=CARTESIAN_POINT ( 'NONE',  ( 7.644554776091147741E-16, 12.48450537969573659, -49.15625000204837391 ) ) ;
#32009=CARTESIAN_POINT ( 'NONE',  ( 9.999999999999998224, 0.000000000000000000, -105.4999999999999858 ) ) ;
#32010=CARTESIAN_POINT ( 'NONE',  ( -10.81189881249999907, -6.242252689847864744, -146.1562500020484094 ) ) ;
#32011=CARTESIAN_POINT ( 'NONE',  ( 7.644554776091147741E-16, 12.48450537969573659, -151.1562500020484094 ) ) ;
#32012=CARTESIAN_POINT ( 'NONE',  ( 9.999999999998969713, 5.773502691896851502, -60.37499999999996447 ) ) ;
#32013=CARTESIAN_POINT ( 'NONE',  ( 0.000000000000000000, 0.000000000000000000, -200.0000000000000000 ) ) ;
#32015=ORIENTED_EDGE ( 'NONE', *, *, #37295, .T. ) ;
#32017=CYLINDRICAL_SURFACE ( 'NONE', #8636, 9.999999999999998224 ) ;
#32018=CARTESIAN_POINT ( 'NONE',  ( -2.293366432827344421E-15, -12.48450537969573659, -184.7187500020484094 ) ) ;
#32019=CARTESIAN_POINT ( 'NONE',  ( 5.405949406249992428, -9.363379034771808662, -30.09375000204836326 ) ) ;
#32020=CARTESIAN_POINT ( 'NONE',  ( 9.999999999999998224, 0.000000000000000000, -40.99999999999997868 ) ) ;
#32021=EDGE_CURVE ( 'NONE', #22494, #4750, #5356, .T. ) ;
#32022=CARTESIAN_POINT ( 'NONE',  ( -10.81189881249999729, -6.242252689847864744, -162.4687500020483526 ) ) ;
#32023=CARTESIAN_POINT ( 'NONE',  ( 10.81189881249999907, 6.242252689847868297, -154.2187500020483810 ) ) ;
#32024=LINE ( 'NONE', #38266, #12112 ) ;
#32029=EDGE_CURVE ( 'NONE', #31210, #28982, #12195, .T. ) ;
#32030=CARTESIAN_POINT ( 'NONE',  ( -9.999999999999998224, 1.224646799147353059E-15, -176.7500000000000284 ) ) ;
#32031=CARTESIAN_POINT ( 'NONE',  ( -4.999999999999996447, 8.660254037844387298, -157.5000000000000000 ) ) ;
#32033=CARTESIAN_POINT ( 'NONE',  ( -10.81189881249999907, -6.242252689847864744, -81.46875000204838102 ) ) ;
#32034=DIRECTION ( 'NONE',  ( -0.000000000000000000, -0.000000000000000000, 1.000000000000000000 ) ) ;
#32035=CARTESIAN_POINT ( 'NONE',  ( -5.405949406249996869, 9.363379034771805109, -49.03125000204838813 ) ) ;
#32038=CARTESIAN_POINT ( 'NONE',  ( -5.000000000000003553, -8.660254037844383745, -139.0000000000000000 ) ) ;
#32039=CARTESIAN_POINT ( 'NONE',  ( 5.405949406249999534, 9.363379034771803333, -148.2812500020483810 ) ) ;
#32041=CARTESIAN_POINT ( 'NONE',  ( -9.999999999999998224, 1.224646799147353059E-15, -24.12500000409675849 ) ) ;
#32043=CARTESIAN_POINT ( 'NONE',  ( 9.999999999999998224, 0.000000000000000000, -123.8750000040967905 ) ) ;
#32048=CYLINDRICAL_SURFACE ( 'NONE', #42198, 9.999999999999998224 ) ;
#32049=CARTESIAN_POINT ( 'NONE',  ( -5.405949406249996869, 9.363379034771805109, -172.0312500020484094 ) ) ;
#32050=CARTESIAN_POINT ( 'NONE',  ( 9.999999999999998224, 0.000000000000000000, -48.87500000409678336 ) ) ;
#32051=( BOUNDED_CURVE ( )  B_SPLINE_CURVE ( 2, ( #38684, #28775, #11702, #41903, #9118, #41482, #25110 ),
 .UNSPECIFIED., .F., .F. ) 
 B_SPLINE_CURVE_WITH_KNOTS ( ( 3, 2, 2, 3 ),
 ( 0.7052238805970151292, 0.7064676616915425145, 0.7077114427860698997, 0.7089552238805972850 ),
 .UNSPECIFIED. ) 
 CURVE ( )  GEOMETRIC_REPRESENTATION_ITEM ( )  RATIONAL_B_SPLINE_CURVE ( ( 0.9999999999999761302, 0.8660254037844625774, 1.000000000000000000, 0.8660254037844387076, 1.000000000000000000, 0.8660254037844148378, 1.000000000000023981 ) ) 
 REPRESENTATION_ITEM ( '' )  );
#32052=CARTESIAN_POINT ( 'NONE',  ( -9.999999999999479527, -5.773502691896549521, -98.62499999999998579 ) ) ;
#32054=CARTESIAN_POINT ( 'NONE',  ( 7.644554776091147741E-16, 12.48450537969573659, -167.6562500020483810 ) ) ;
#32055=EDGE_CURVE ( 'NONE', #26056, #31902, #11988, .T. ) ;
#32056=CARTESIAN_POINT ( 'NONE',  ( 7.423074889580959734, 12.85714285714296423, 52.14285714285716011 ) ) ;
#32057=LINE ( 'NONE', #15196, #23416 ) ;
#32060=CARTESIAN_POINT ( 'NONE',  ( 9.999999999999998224, 0.000000000000000000, -162.8750000040967905 ) ) ;
#32061=CARTESIAN_POINT ( 'NONE',  ( 10.81189881249999551, -6.242252689847874514, -76.65625000204838102 ) ) ;
#32062=ORIENTED_EDGE ( 'NONE', *, *, #26529, .F. ) ;
#32066=ORIENTED_EDGE ( 'NONE', *, *, #19280, .F. ) ;
#32067=CARTESIAN_POINT ( 'NONE',  ( 5.405949406249999534, 9.363379034771803333, -28.09375000204836326 ) ) ;
#32068=CARTESIAN_POINT ( 'NONE',  ( 9.999999999999479527, 5.773502691896553074, -74.25000000409676204 ) ) ;
#32069=CARTESIAN_POINT ( 'NONE',  ( -10.81189881249999729, 1.324075727343319199E-15, -2.281250002048373915 ) ) ;
#32070=CARTESIAN_POINT ( 'NONE',  ( -10.81189881249999907, -6.242252689847864744, -57.46875000204835970 ) ) ;
#32072=CARTESIAN_POINT ( 'NONE',  ( 10.00000000000051159, -5.773502691895965988, -3.624999999999940492 ) ) ;
#32074=CARTESIAN_POINT ( 'NONE',  ( -2.293366432827344421E-15, -12.48450537969573659, -189.2187500020484094 ) ) ;
#32075=CARTESIAN_POINT ( 'NONE',  ( -10.81189881249999729, 6.242252689847871849, -174.7187500020483810 ) ) ;
#32078=CARTESIAN_POINT ( 'NONE',  ( -9.999999999999998224, 1.224646799147353059E-15, -76.24999999999998579 ) ) ;
#32082=CARTESIAN_POINT ( 'NONE',  ( -10.81189881249999729, 6.242252689847871849, -102.7187500020483810 ) ) ;
#32083=CARTESIAN_POINT ( 'NONE',  ( -10.00000000000007994, 5.773502691896212013, -196.3750000000000000 ) ) ;
#32084=CARTESIAN_POINT ( 'NONE',  ( 5.405949406249992428, -9.363379034771808662, -76.78125000204838102 ) ) ;
#32085=CARTESIAN_POINT ( 'NONE',  ( 10.81189881249999729, 6.242252689847867408, -89.71875000204838102 ) ) ;
#32087=CARTESIAN_POINT ( 'NONE',  ( -9.999999999999998224, 1.224646799147353059E-15, -144.1250000040967905 ) ) ;
#32089=( BOUNDED_CURVE ( )  B_SPLINE_CURVE ( 2, ( #20208, #33397, #16957, #14569, #37682, #30370, #1224 ),
 .UNSPECIFIED., .F., .F. ) 
 B_SPLINE_CURVE_WITH_KNOTS ( ( 3, 2, 2, 3 ),
 ( 0.8992537313432839019, 0.9004975124378112872, 0.9017412935323385614, 0.9029850746268659467 ),
 .UNSPECIFIED. ) 
 CURVE ( )  GEOMETRIC_REPRESENTATION_ITEM ( )  RATIONAL_B_SPLINE_CURVE ( ( 0.9999999999999641398, 0.8660254037844745678, 1.000000000000000000, 0.8660254037844387076, 1.000000000000000000, 0.8660254037844148378, 1.000000000000023981 ) ) 
 REPRESENTATION_ITEM ( '' )  );
#32094=CARTESIAN_POINT ( 'NONE',  ( 5.405949406249999534, 9.363379034771803333, -194.7812500020484094 ) ) ;
#32095=DIRECTION ( 'NONE',  ( -0.000000000000000000, -0.000000000000000000, 1.000000000000000000 ) ) ;
#32097=ORIENTED_EDGE ( 'NONE', *, *, #7449, .F. ) ;
#32098=CARTESIAN_POINT ( 'NONE',  ( 7.070501591499377789E-16, 11.54700538379251284, -69.12500000000000000 ) ) ;
#32100=CARTESIAN_POINT ( 'NONE',  ( -4.999999999999996447, 8.660254037844387298, -70.87500000409677625 ) ) ;
#32104=AXIS2_PLACEMENT_3D ( 'NONE', #39490, #16375, #31826 ) ;
#32105=CARTESIAN_POINT ( 'NONE',  ( 10.81189881249999551, -6.242252689847874514, -64.65625000204838102 ) ) ;
#32107=CARTESIAN_POINT ( 'NONE',  ( 5.000000000000000000, 8.660254037844385522, -93.62500000409677625 ) ) ;
#32109=ORIENTED_EDGE ( 'NONE', *, *, #11683, .F. ) ;
#32110=CARTESIAN_POINT ( 'NONE',  ( -5.405949406250003975, -9.363379034771801557, -189.5312500020484094 ) ) ;
#32112=CARTESIAN_POINT ( 'NONE',  ( -10.81189881249999729, 6.242252689847871849, -5.218750002048341052 ) ) ;
#32113=CYLINDRICAL_SURFACE ( 'NONE', #3486, 9.999999999999998224 ) ;
#32114=AXIS2_PLACEMENT_3D ( 'NONE', #17959, #11272, #8059 ) ;
#32115=CARTESIAN_POINT ( 'NONE',  ( 4.999999999999992006, -8.660254037844389075, -180.7500000000000284 ) ) ;
#32116=CARTESIAN_POINT ( 'NONE',  ( 9.999999999999998224, 0.000000000000000000, -137.0000000000000000 ) ) ;
#32117=CARTESIAN_POINT ( 'NONE',  ( -10.00000000000000000, -5.773502691896251982, -172.1250000000000284 ) ) ;
#32118=CYLINDRICAL_SURFACE ( 'NONE', #28976, 9.999999999999998224 ) ;
#32119=CARTESIAN_POINT ( 'NONE',  ( 5.405949406249992428, -9.363379034771808662, -99.28125000204839523 ) ) ;
#32120=ORIENTED_EDGE ( 'NONE', *, *, #31490, .T. ) ;
#32121=DIRECTION ( 'NONE',  ( 1.000000000000000000, 0.000000000000000000, 0.000000000000000000 ) ) ;
#32122=VERTEX_POINT ( 'NONE', #15431 ) ;
#32123=ORIENTED_EDGE ( 'NONE', *, *, #37545, .F. ) ;
#32124=CARTESIAN_POINT ( 'NONE',  ( 10.81189881249999729, 0.000000000000000000, -27.03125000204836681 ) ) ;
#32126=CARTESIAN_POINT ( 'NONE',  ( -10.81189881249999907, -6.242252689847864744, -82.96875000204836681 ) ) ;
#32128=CARTESIAN_POINT ( 'NONE',  ( -10.81189881249999729, 6.242252689847871849, -197.2187500020484379 ) ) ;
#32129=VECTOR ( 'NONE', #3929, 1000.000000000000000 ) ;
#32130=VECTOR ( 'NONE', #26468, 1000.000000000000000 ) ;
#32131=CARTESIAN_POINT ( 'NONE',  ( -9.999999999999998224, 1.224646799147353059E-15, -170.7500000000000000 ) ) ;
#32132=CARTESIAN_POINT ( 'NONE',  ( -9.999999999999998224, 1.224646799147353059E-15, -30.12500000409676204 ) ) ;
#32134=CARTESIAN_POINT ( 'NONE',  ( -9.999999999999998224, 1.224646799147353059E-15, -15.12500000409674961 ) ) ;
#32136=CARTESIAN_POINT ( 'NONE',  ( 5.405949406249999534, 9.363379034771803333, -128.5937500020483810 ) ) ;
#32137=CARTESIAN_POINT ( 'NONE',  ( 10.81189881249999729, 6.242252689847867408, -116.7187500020483810 ) ) ;
#32138=AXIS2_PLACEMENT_3D ( 'NONE', #29564, #17016, #33018 ) ;
#32141=CARTESIAN_POINT ( 'NONE',  ( 7.070501591499377789E-16, 11.54700538379251284, -170.0000000040967905 ) ) ;
#32142=CARTESIAN_POINT ( 'NONE',  ( -2.121150477449813534E-15, -11.54700538379251284, -133.2500000040967905 ) ) ;
#32145=CARTESIAN_POINT ( 'NONE',  ( -10.81189881249999729, -6.242252689847864744, -46.96875000204837391 ) ) ;
#32147=CARTESIAN_POINT ( 'NONE',  ( -10.81189881249999907, -6.242252689847864744, -5.156250002048356151 ) ) ;
#32149=CARTESIAN_POINT ( 'NONE',  ( 7.070501591499376803E-16, 11.54700538379251284, -127.6249999999999858 ) ) ;
#32151=CARTESIAN_POINT ( 'NONE',  ( -10.00000000000000000, -5.773502691896251982, -92.62499999999998579 ) ) ;
#32153=CARTESIAN_POINT ( 'NONE',  ( -9.999999999999998224, 1.224646799147353059E-15, -97.62500000409677625 ) ) ;
#32154=CARTESIAN_POINT ( 'NONE',  ( -9.999999999999834799, -5.773502691896343464, -190.5000000040967905 ) ) ;
#32156=CARTESIAN_POINT ( 'NONE',  ( 7.644554776091147741E-16, 12.48450537969573659, -94.15625000204839523 ) ) ;
#32159=CARTESIAN_POINT ( 'NONE',  ( 7.070501591499376803E-16, 11.54700538379251284, -4.624999999999958256 ) ) ;
#32160=CARTESIAN_POINT ( 'NONE',  ( -10.81189881249999907, -6.242252689847864744, -156.6562500020483810 ) ) ;
#32162=ORIENTED_EDGE ( 'NONE', *, *, #24644, .F. ) ;
#32163=CARTESIAN_POINT ( 'NONE',  ( -5.000000000000003553, -8.660254037844383745, -18.99999999999996092 ) ) ;
#32164=CARTESIAN_POINT ( 'NONE',  ( -10.81189881249999729, 6.242252689847871849, -23.40625000204837747 ) ) ;
#32165=CARTESIAN_POINT ( 'NONE',  ( -9.999999999999998224, 5.773502691896259087, -154.3749999999999716 ) ) ;
#32167=AXIS2_PLACEMENT_3D ( 'NONE', #21111, #7531, #1493 ) ;
#32169=CARTESIAN_POINT ( 'NONE',  ( -2.121150477449813534E-15, -11.54700538379251284, -197.3750000000000284 ) ) ;
#32170=CARTESIAN_POINT ( 'NONE',  ( -10.81189881249999907, -6.242252689847864744, -125.1562500020483810 ) ) ;
#32174=CARTESIAN_POINT ( 'NONE',  ( 7.644554776091147741E-16, 12.48450537969573659, -50.65625000204838102 ) ) ;
#32176=CARTESIAN_POINT ( 'NONE',  ( -2.293366432827344421E-15, -12.48450537969573659, -105.2187500020483952 ) ) ;
#32178=ORIENTED_EDGE ( 'NONE', *, *, #713, .F. ) ;
#32179=FACE_OUTER_BOUND ( 'NONE', #17555, .T. ) ;
#32180=DIRECTION ( 'NONE',  ( -0.000000000000000000, -0.000000000000000000, 1.000000000000000000 ) ) ;
#32181=CARTESIAN_POINT ( 'NONE',  ( 5.405949406249992428, -9.363379034771808662, -156.0937500020483810 ) ) ;
#32183=CARTESIAN_POINT ( 'NONE',  ( 7.644554776091147741E-16, 12.48450537969573659, -5.468750002048341941 ) ) ;
#32185=EDGE_CURVE ( 'NONE', #28503, #6727, #9750, .T. ) ;
#32186=CARTESIAN_POINT ( 'NONE',  ( 10.81189881249999729, 0.000000000000000000, -142.3437500020483810 ) ) ;
#32190=CARTESIAN_POINT ( 'NONE',  ( -10.00000000000000000, -5.773502691896251982, -192.0000000040968189 ) ) ;
#32192=CARTESIAN_POINT ( 'NONE',  ( 5.405949406249999534, 9.363379034771803333, -196.2812500020484094 ) ) ;
#32193=CARTESIAN_POINT ( 'NONE',  ( 5.000000000000000000, 8.660254037844385522, -149.1250000040967905 ) ) ;
#32196=CARTESIAN_POINT ( 'NONE',  ( -10.81189881249999729, -6.242252689847864744, -66.46875000204838102 ) ) ;
#32197=CARTESIAN_POINT ( 'NONE',  ( -10.81189881249999729, 6.242252689847871849, -59.21875000204837391 ) ) ;
#32199=CARTESIAN_POINT ( 'NONE',  ( 5.405949406249999534, 9.363379034771803333, -28.28125000204837036 ) ) ;
#32203=CARTESIAN_POINT ( 'NONE',  ( 7.070501591499377789E-16, 11.54700538379251284, -112.6249999999999858 ) ) ;
#32207=CARTESIAN_POINT ( 'NONE',  ( 10.81189881249999729, 6.242252689847867408, -116.9062500020483952 ) ) ;
#32208=ORIENTED_EDGE ( 'NONE', *, *, #31921, .F. ) ;
#32209=CARTESIAN_POINT ( 'NONE',  ( 9.999999999999998224, 0.000000000000000000, -200.0000000000000000 ) ) ;
#32211=DIRECTION ( 'NONE',  ( 0.6123724356957960246, 0.3535533905932753962, 0.7071067811865453523 ) ) ;
#32213=CARTESIAN_POINT ( 'NONE',  ( 9.999999999999998224, 0.000000000000000000, -42.49999999999998579 ) ) ;
#32214=CARTESIAN_POINT ( 'NONE',  ( 10.00000000000000000, 5.773502691896255534, -29.25000000409675494 ) ) ;
#32215=CARTESIAN_POINT ( 'NONE',  ( -5.405949406249996869, 9.363379034771805109, -52.03125000204835970 ) ) ;
#32218=( BOUNDED_CURVE ( )  B_SPLINE_CURVE ( 2, ( #9913, #10917, #9, #26329, #23089, #19206, #30373 ),
 .UNSPECIFIED., .F., .F. ) 
 B_SPLINE_CURVE_WITH_KNOTS ( ( 3, 2, 2, 3 ),
 ( 0.8619402985074630097, 0.8631840796019903950, 0.8644278606965177802, 0.8656716417910450545 ),
 .UNSPECIFIED. ) 
 CURVE ( )  GEOMETRIC_REPRESENTATION_ITEM ( )  RATIONAL_B_SPLINE_CURVE ( ( 0.9999999999999641398, 0.8660254037844745678, 1.000000000000000000, 0.8660254037844387076, 1.000000000000000000, 0.8660254037844028474, 1.000000000000035971 ) ) 
 REPRESENTATION_ITEM ( '' )  );
#32219=CARTESIAN_POINT ( 'NONE',  ( 7.070501591499376803E-16, 11.54700538379251284, -24.12499999999998224 ) ) ;
#32220=CARTESIAN_POINT ( 'NONE',  ( -10.81189881249999729, 1.324075727343319199E-15, -143.2812500020483810 ) ) ;
#32221=CARTESIAN_POINT ( 'NONE',  ( 7.644554776091147741E-16, 12.48450537969573659, -152.6562500020484094 ) ) ;
#32223=EDGE_CURVE ( 'NONE', #34698, #9647, #31656, .T. ) ;
#32224=LINE ( 'NONE', #5885, #10726 ) ;
#32225=ORIENTED_EDGE ( 'NONE', *, *, #41203, .F. ) ;
#32226=EDGE_LOOP ( 'NONE', ( #16283, #32267, #31742, #10850 ) ) ;
#32227=EDGE_LOOP ( 'NONE', ( #28068, #13390, #39468, #25585 ) ) ;
#32228=DIRECTION ( 'NONE',  ( 1.000000000000000000, 0.000000000000000000, 0.000000000000000000 ) ) ;
#32229=CARTESIAN_POINT ( 'NONE',  ( -10.81189881249999729, 6.242252689847871849, -183.7187500020484379 ) ) ;
#32230=CARTESIAN_POINT ( 'NONE',  ( 5.405949406249992428, -9.363379034771808662, -28.59375000204836326 ) ) ;
#32231=CARTESIAN_POINT ( 'NONE',  ( -9.999999999999998224, 1.224646799147353059E-15, -200.0000000000000000 ) ) ;
#32232=CARTESIAN_POINT ( 'NONE',  ( -5.405949406249996869, 9.363379034771805109, -165.8437500020484094 ) ) ;
#32233=CARTESIAN_POINT ( 'NONE',  ( 10.81189881249999729, 0.000000000000000000, -143.8437500020483810 ) ) ;
#32234=CARTESIAN_POINT ( 'NONE',  ( -9.999999999999998224, 1.224646799147353059E-15, -200.0000000000000000 ) ) ;
#32237=CARTESIAN_POINT ( 'NONE',  ( -5.405949406250003975, -9.363379034771801557, -21.34375000204835615 ) ) ;
#32239=CARTESIAN_POINT ( 'NONE',  ( 7.070501591499376803E-16, 11.54700538379251284, -157.6250000000000284 ) ) ;
#32241=CARTESIAN_POINT ( 'NONE',  ( 5.405949406249992428, -9.363379034771808662, -84.09375000204836681 ) ) ;
#32243=CARTESIAN_POINT ( 'NONE',  ( -10.81189881249999729, 6.242252689847871849, -53.40625000204837391 ) ) ;
#32247=CARTESIAN_POINT ( 'NONE',  ( -10.00000000000000000, -5.773502691896251982, -134.6250000000000000 ) ) ;
#32248=CARTESIAN_POINT ( 'NONE',  ( -2.293366432827344421E-15, -12.48450537969573659, -142.9062500020484094 ) ) ;
#32249=FACE_OUTER_BOUND ( 'NONE', #40645, .T. ) ;
#32250=CARTESIAN_POINT ( 'NONE',  ( 4.999999999999992006, -8.660254037844389075, -125.6250000040967620 ) ) ;
#32252=ORIENTED_EDGE ( 'NONE', *, *, #14608, .T. ) ;
#32255=CARTESIAN_POINT ( 'NONE',  ( 10.00000000000154010, -5.773502691895370020, -22.00000000409673007 ) ) ;
#32256=CARTESIAN_POINT ( 'NONE',  ( 10.81189881249999551, -6.242252689847874514, -171.1562500020484094 ) ) ;
#32257=CARTESIAN_POINT ( 'NONE',  ( -5.000000000000003553, -8.660254037844383745, -52.37500000409675494 ) ) ;
#32258=CARTESIAN_POINT ( 'NONE',  ( -2.121150477449813534E-15, -11.54700538379251284, -98.37500000000000000 ) ) ;
#32260=CARTESIAN_POINT ( 'NONE',  ( -4.999999999999996447, 8.660254037844387298, -9.375000004096744277 ) ) ;
#32261=CARTESIAN_POINT ( 'NONE',  ( 7.644554776091147741E-16, 12.48450537969573659, -166.1562500020483810 ) ) ;
#32262=EDGE_CURVE ( 'NONE', #26141, #32541, #18585, .T. ) ;
#32263=CARTESIAN_POINT ( 'NONE',  ( -10.00000000000051337, 5.773502691895962435, -7.374999999999958256 ) ) ;
#32264=CARTESIAN_POINT ( 'NONE',  ( -9.999999999998969713, -5.773502691896847949, -56.62499999999995737 ) ) ;
#32267=ORIENTED_EDGE ( 'NONE', *, *, #9949, .T. ) ;
#32268=ADVANCED_FACE ( 'NONE', ( #10439 ), #16263, .T. ) ;
#32269=CARTESIAN_POINT ( 'NONE',  ( -9.999999999999998224, 1.224646799147353059E-15, -79.24999999999998579 ) ) ;
#32271=CARTESIAN_POINT ( 'NONE',  ( 7.070501591499376803E-16, 11.54700538379251284, -137.0000000040967905 ) ) ;
#32272=CARTESIAN_POINT ( 'NONE',  ( 10.81189881249999729, 0.000000000000000000, -76.53125000204838102 ) ) ;
#32273=ORIENTED_EDGE ( 'NONE', *, *, #22707, .F. ) ;
#32274=CARTESIAN_POINT ( 'NONE',  ( -4.999999999999996447, 8.660254037844387298, -29.99999999999997158 ) ) ;
#32276=ORIENTED_EDGE ( 'NONE', *, *, #39156, .T. ) ;
#32277=CARTESIAN_POINT ( 'NONE',  ( 10.81189881249999551, -6.242252689847874514, -32.96875000204834549 ) ) ;
#32278=CARTESIAN_POINT ( 'NONE',  ( 10.00000000000076916, -5.773502691895816774, -106.0000000040967763 ) ) ;
#32279=CARTESIAN_POINT ( 'NONE',  ( -10.81189881249999907, -6.242252689847864744, -8.156250002048370362 ) ) ;
#32280=CARTESIAN_POINT ( 'NONE',  ( 10.81189881249999551, -6.242252689847874514, -52.46875000204837391 ) ) ;
#32281=ORIENTED_EDGE ( 'NONE', *, *, #28864, .T. ) ;
#32285=CARTESIAN_POINT ( 'NONE',  ( -10.81189881249999729, 1.324075727343319199E-15, -189.5937500020483810 ) ) ;
#32286=CARTESIAN_POINT ( 'NONE',  ( 5.405949406249999534, 9.363379034771803333, -178.0937500020484094 ) ) ;
#32289=CARTESIAN_POINT ( 'NONE',  ( 9.999999999999998224, 0.000000000000000000, -168.5000000000000000 ) ) ;
#32291=EDGE_CURVE ( 'NONE', #2592, #7682, #33224, .T. ) ;
#32293=CARTESIAN_POINT ( 'NONE',  ( -5.405949406249996869, 9.363379034771805109, -107.3437500020483810 ) ) ;
#32294=CARTESIAN_POINT ( 'NONE',  ( 9.999999999999998224, 0.000000000000000000, -197.0000000000000000 ) ) ;
#32295=CARTESIAN_POINT ( 'NONE',  ( -10.81189881249999729, 6.242252689847871849, -77.40625000204838102 ) ) ;
#32296=CARTESIAN_POINT ( 'NONE',  ( 10.81189881249999729, 0.000000000000000000, -6.031250002048377468 ) ) ;
#32297=CARTESIAN_POINT ( 'NONE',  ( -10.81189881249999729, 6.242252689847871849, -80.21875000204838102 ) ) ;
#32299=AXIS2_PLACEMENT_3D ( 'NONE', #2034, #38061, #15799 ) ;
#32300=( BOUNDED_CURVE ( )  B_SPLINE_CURVE ( 2, ( #37842, #38854, #31168, #4821, #22247, #15742, #19000 ),
 .UNSPECIFIED., .F., .F. ) 
 B_SPLINE_CURVE_WITH_KNOTS ( ( 3, 2, 2, 3 ),
 ( 0.2985074626865671932, 0.2997512437810946340, 0.3009950248756220192, 0.3022388059701494045 ),
 .UNSPECIFIED. ) 
 CURVE ( )  GEOMETRIC_REPRESENTATION_ITEM ( )  RATIONAL_B_SPLINE_CURVE ( ( 0.9999999999999940048, 0.8660254037844447028, 1.000000000000000000, 0.8660254037844387076, 1.000000000000000000, 0.8660254037844207220, 1.000000000000017986 ) ) 
 REPRESENTATION_ITEM ( '' )  );
#32302=CARTESIAN_POINT ( 'NONE',  ( 5.000000000000000000, 8.660254037844385522, -146.1250000040967905 ) ) ;
#32307=CARTESIAN_POINT ( 'NONE',  ( 7.644554776091147741E-16, 12.48450537969573659, -193.1562500020484094 ) ) ;
#32308=CARTESIAN_POINT ( 'NONE',  ( 9.999999999999998224, 0.000000000000000000, -51.49999999999996447 ) ) ;
#32310=ORIENTED_EDGE ( 'NONE', *, *, #30576, .F. ) ;
#32311=CARTESIAN_POINT ( 'NONE',  ( 9.999999999999996447, -5.773502691896262640, -63.62499999999999289 ) ) ;
#32313=CARTESIAN_POINT ( 'NONE',  ( 9.999999999999996447, -5.773502691896262640, -74.50000000409677625 ) ) ;
#32317=CARTESIAN_POINT ( 'NONE',  ( 10.81189881249999729, 6.242252689847867408, -67.40625000204839523 ) ) ;
#32320=ORIENTED_EDGE ( 'NONE', *, *, #34357, .F. ) ;
#32321=CARTESIAN_POINT ( 'NONE',  ( -2.293366432827344421E-15, -12.48450537969573659, -192.4062500020484094 ) ) ;
#32323=CARTESIAN_POINT ( 'NONE',  ( -2.293366432827344421E-15, -12.48450537969573659, -7.718750002048352599 ) ) ;
#32326=CARTESIAN_POINT ( 'NONE',  ( -9.999999999999998224, 1.224646799147353059E-15, -133.2499999999999716 ) ) ;
#32327=EDGE_CURVE ( 'NONE', #28547, #41040, #37617, .T. ) ;
#32328=CARTESIAN_POINT ( 'NONE',  ( -5.000000000000003553, -8.660254037844383745, -178.0000000000000000 ) ) ;
#32329=CARTESIAN_POINT ( 'NONE',  ( -10.00000000000051337, 5.773502691895962435, -97.37499999999998579 ) ) ;
#32331=CARTESIAN_POINT ( 'NONE',  ( -10.81189881249999729, 1.324075727343319199E-15, -102.7812500020483952 ) ) ;
#32332=ORIENTED_EDGE ( 'NONE', *, *, #26453, .T. ) ;
#32334=VECTOR ( 'NONE', #26604, 1000.000000000000000 ) ;
#32335=EDGE_LOOP ( 'NONE', ( #1863, #6623, #9537, #6938 ) ) ;
#32336=VERTEX_POINT ( 'NONE', #12824 ) ;
#32337=CARTESIAN_POINT ( 'NONE',  ( -10.81189881249999907, -6.242252689847864744, -27.65625000204838457 ) ) ;
#32339=CARTESIAN_POINT ( 'NONE',  ( 7.644554776091147741E-16, 12.48450537969573659, -78.96875000204839523 ) ) ;
#32340=FACE_OUTER_BOUND ( 'NONE', #17002, .T. ) ;
#32343=( BOUNDED_CURVE ( )  B_SPLINE_CURVE ( 2, ( #23556, #7143, #46, #20296, #10792, #13170, #27204 ),
 .UNSPECIFIED., .F., .F. ) 
 B_SPLINE_CURVE_WITH_KNOTS ( ( 3, 2, 2, 3 ),
 ( 0.4328358208955225273, 0.4340796019900499125, 0.4353233830845772978, 0.4365671641791046276 ),
 .UNSPECIFIED. ) 
 CURVE ( )  GEOMETRIC_REPRESENTATION_ITEM ( )  RATIONAL_B_SPLINE_CURVE ( ( 0.9999999999999820144, 0.8660254037844566932, 1.000000000000000000, 0.8660254037844387076, 1.000000000000000000, 0.8660254037844207220, 1.000000000000017986 ) ) 
 REPRESENTATION_ITEM ( '' )  );
#32344=CARTESIAN_POINT ( 'NONE',  ( 9.999999999999998224, 0.000000000000000000, -129.8750000040967905 ) ) ;
#32345=LINE ( 'NONE', #4030, #35012 ) ;
#32347=CARTESIAN_POINT ( 'NONE',  ( -9.999999999999998224, 1.224646799147353059E-15, -12.12500000409674783 ) ) ;
#32348=CARTESIAN_POINT ( 'NONE',  ( -5.000000000000003553, -8.660254037844383745, -125.5000000000000000 ) ) ;
#32349=CARTESIAN_POINT ( 'NONE',  ( 5.405949406249999534, 9.363379034771803333, -127.0937500020483668 ) ) ;
#32350=CARTESIAN_POINT ( 'NONE',  ( -10.81189881249999729, 1.324075727343319199E-15, -101.2812500020483952 ) ) ;
#32351=CARTESIAN_POINT ( 'NONE',  ( -10.81189881249999729, 1.324075727343319199E-15, -113.0937500020483810 ) ) ;
#32354=CARTESIAN_POINT ( 'NONE',  ( -5.000000000000003553, -8.660254037844383745, -166.3750000040967905 ) ) ;
#32356=FACE_OUTER_BOUND ( 'NONE', #28928, .T. ) ;
#32360=CARTESIAN_POINT ( 'NONE',  ( 10.81189881249999907, 6.242252689847868297, 0.09374999795163654892 ) ) ;
#32362=LINE ( 'NONE', #42252, #6135 ) ;
#32364=CARTESIAN_POINT ( 'NONE',  ( -9.999999999999998224, 5.773502691896259087, -89.87499999999998579 ) ) ;
#32366=CARTESIAN_POINT ( 'NONE',  ( -10.00000000000000000, -5.773502691896251982, -97.50000000409679046 ) ) ;
#32369=CARTESIAN_POINT ( 'NONE',  ( 10.81189881249999729, 6.242252689847867408, -89.90625000204839523 ) ) ;
#32370=ORIENTED_EDGE ( 'NONE', *, *, #39145, .T. ) ;
#32372=CARTESIAN_POINT ( 'NONE',  ( 0.000000000000000000, 0.000000000000000000, -200.0000000000000000 ) ) ;
#32374=ORIENTED_EDGE ( 'NONE', *, *, #25954, .F. ) ;
#32375=CARTESIAN_POINT ( 'NONE',  ( -9.999999999999998224, 5.773502691896259087, -16.37499999999998224 ) ) ;
#32376=VECTOR ( 'NONE', #41555, 1000.000000000000000 ) ;
#32377=CARTESIAN_POINT ( 'NONE',  ( -9.999999999999998224, 1.224646799147353059E-15, -157.2500000000000000 ) ) ;
#32379=AXIS2_PLACEMENT_3D ( 'NONE', #7766, #1073, #16806 ) ;
#32380=CARTESIAN_POINT ( 'NONE',  ( -9.999999999999998224, 5.773502691896259087, -194.8750000000000000 ) ) ;
#32381=CARTESIAN_POINT ( 'NONE',  ( -2.293366432827344421E-15, -12.48450537969573659, -129.4062500020483810 ) ) ;
#32382=ORIENTED_EDGE ( 'NONE', *, *, #8003, .F. ) ;
#32383=CARTESIAN_POINT ( 'NONE',  ( 9.999999999999998224, 0.000000000000000000, -12.49999999999995559 ) ) ;
#32385=CARTESIAN_POINT ( 'NONE',  ( -5.405949406250003975, -9.363379034771801557, -57.53125000204836681 ) ) ;
#32388=CARTESIAN_POINT ( 'NONE',  ( -10.81189881249999729, 1.324075727343319199E-15, -102.5937500020483810 ) ) ;
#32389=EDGE_LOOP ( 'NONE', ( #10667, #20780, #28382, #11055 ) ) ;
#32390=VERTEX_POINT ( 'NONE', #29678 ) ;
#32391=CARTESIAN_POINT ( 'NONE',  ( 9.999999999999998224, 0.000000000000000000, -49.99999999999998579 ) ) ;
#32392=CARTESIAN_POINT ( 'NONE',  ( 5.000000000000000000, 8.660254037844385522, -33.24999999999997158 ) ) ;
#32395=CARTESIAN_POINT ( 'NONE',  ( -23.09401076758503280, 0.000000000000000000, 0.000000000000000000 ) ) ;
#32396=VECTOR ( 'NONE', #27751, 1000.000000000000114 ) ;
#32397=CARTESIAN_POINT ( 'NONE',  ( 7.644554776091147741E-16, 12.48450537969573659, -140.4687500020483810 ) ) ;
#32399=FACE_OUTER_BOUND ( 'NONE', #24937, .T. ) ;
#32401=CARTESIAN_POINT ( 'NONE',  ( 10.00000000000000000, 5.773502691896255534, -191.2500000040968189 ) ) ;
#32403=EDGE_CURVE ( 'NONE', #2293, #10098, #10017, .T. ) ;
#32404=CARTESIAN_POINT ( 'NONE',  ( 10.81189881249999729, 6.242252689847867408, -188.9062500020484094 ) ) ;
#32405=DIRECTION ( 'NONE',  ( -0.000000000000000000, -0.000000000000000000, 1.000000000000000000 ) ) ;
#32408=CARTESIAN_POINT ( 'NONE',  ( -2.293366432827344421E-15, -12.48450537969573659, -67.71875000204838102 ) ) ;
#32409=CARTESIAN_POINT ( 'NONE',  ( 10.81189881249999551, -6.242252689847874514, -46.46875000204837391 ) ) ;
#32411=CARTESIAN_POINT ( 'NONE',  ( -10.81189881249999907, -6.242252689847864744, -27.65625000204838457 ) ) ;
#32415=CARTESIAN_POINT ( 'NONE',  ( -5.000000000000003553, -8.660254037844383745, -110.4999999999999858 ) ) ;
#32416=CARTESIAN_POINT ( 'NONE',  ( -10.00000000000051337, 5.773502691895962435, -118.7500000040967763 ) ) ;
#32419=CARTESIAN_POINT ( 'NONE',  ( 7.644554776091147741E-16, 12.48450537969573659, -112.1562500020483952 ) ) ;
#32420=ORIENTED_EDGE ( 'NONE', *, *, #29617, .F. ) ;
#32424=CARTESIAN_POINT ( 'NONE',  ( 9.999999999999996447, -5.773502691896262640, -42.62499999999997868 ) ) ;
#32425=CARTESIAN_POINT ( 'NONE',  ( -10.00000000000000000, -5.773502691896251982, -25.50000000409676915 ) ) ;
#32426=CARTESIAN_POINT ( 'NONE',  ( 10.81189881249999729, 0.000000000000000000, -42.03125000204838102 ) ) ;
#32428=DIRECTION ( 'NONE',  ( 1.000000000000000000, 0.000000000000000000, 0.000000000000000000 ) ) ;
#32432=CARTESIAN_POINT ( 'NONE',  ( 10.81189881249999907, 6.242252689847868297, -133.4062500020483810 ) ) ;
#32433=VECTOR ( 'NONE', #38792, 1000.000000000000000 ) ;
#32434=CARTESIAN_POINT ( 'NONE',  ( -10.81189881249999729, 6.242252689847871849, -147.9062500020483810 ) ) ;
#32435=CARTESIAN_POINT ( 'NONE',  ( 9.999999999998969713, 5.773502691896851502, -51.37499999999997158 ) ) ;
#32436=VERTEX_POINT ( 'NONE', #3770 ) ;
#32437=EDGE_CURVE ( 'NONE', #1269, #30921, #23001, .T. ) ;
#32439=ORIENTED_EDGE ( 'NONE', *, *, #9016, .F. ) ;
#32440=CARTESIAN_POINT ( 'NONE',  ( 0.000000000000000000, 0.000000000000000000, -200.0000000000000000 ) ) ;
#32441=CARTESIAN_POINT ( 'NONE',  ( 5.405949406249992428, -9.363379034771808662, -177.0937500020484094 ) ) ;
#32442=CARTESIAN_POINT ( 'NONE',  ( -10.81189881249999729, 6.242252689847871849, -33.71875000204835260 ) ) ;
#32444=CARTESIAN_POINT ( 'NONE',  ( 10.81189881249999729, 6.242252689847867408, -161.7187500020483810 ) ) ;
#32445=CARTESIAN_POINT ( 'NONE',  ( 10.81189881249999551, -6.242252689847874514, -146.9687500020484094 ) ) ;
#32446=EDGE_CURVE ( 'NONE', #14499, #10098, #42017, .T. ) ;
#32447=CARTESIAN_POINT ( 'NONE',  ( 10.70731569305672615, 1.500182182589836044, 0.000000000000000000 ) ) ;
#32450=CARTESIAN_POINT ( 'NONE',  ( 10.81189881249999907, 6.242252689847868297, -16.21875000204836326 ) ) ;
#32452=CARTESIAN_POINT ( 'NONE',  ( 0.000000000000000000, 0.000000000000000000, -200.0000000000000000 ) ) ;
#32456=CARTESIAN_POINT ( 'NONE',  ( 7.644554776091147741E-16, 12.48450537969573659, -72.96875000204835260 ) ) ;
#32457=CARTESIAN_POINT ( 'NONE',  ( 10.81189881249999551, -6.242252689847874514, -52.65625000204837391 ) ) ;
#32462=CARTESIAN_POINT ( 'NONE',  ( 5.000000000000000000, 8.660254037844385522, -133.7499999999999716 ) ) ;
#32463=CARTESIAN_POINT ( 'NONE',  ( -10.81189881249999729, 6.242252689847871849, -147.9062500020484094 ) ) ;
#32465=CARTESIAN_POINT ( 'NONE',  ( -10.00000000000000000, -5.773502691896251982, -120.0000000040967905 ) ) ;
#32468=VERTEX_POINT ( 'NONE', #30955 ) ;
#32471=CARTESIAN_POINT ( 'NONE',  ( -10.00000000000154188, 5.773502691895366468, -52.37499999999992895 ) ) ;
#32472=CARTESIAN_POINT ( 'NONE',  ( -10.81189881249999907, -6.242252689847864744, -174.6562500020483810 ) ) ;
#32473=CARTESIAN_POINT ( 'NONE',  ( -10.00000000000000000, -5.773502691896251982, -48.00000000409676204 ) ) ;
#32474=CARTESIAN_POINT ( 'NONE',  ( 9.999999999999998224, 0.000000000000000000, -97.99999999999998579 ) ) ;
#32476=LINE ( 'NONE', #16668, #30395 ) ;
#32477=CARTESIAN_POINT ( 'NONE',  ( -5.405949406250003975, -9.363379034771801557, -158.0312500020484094 ) ) ;
#32478=CARTESIAN_POINT ( 'NONE',  ( 5.405949406249999534, 9.363379034771803333, -143.5937500020483810 ) ) ;
#32480=CARTESIAN_POINT ( 'NONE',  ( -4.999999999999996447, 8.660254037844387298, -79.87500000409677625 ) ) ;
#32482=CARTESIAN_POINT ( 'NONE',  ( 0.000000000000000000, 0.000000000000000000, -200.0000000000000000 ) ) ;
#32483=CARTESIAN_POINT ( 'NONE',  ( 7.644554776091147741E-16, 12.48450537969573659, -67.15625000204838102 ) ) ;
#32484=VERTEX_POINT ( 'NONE', #21224 ) ;
#32486=CARTESIAN_POINT ( 'NONE',  ( -2.121150477449813534E-15, -11.54700538379251284, -188.7500000040967905 ) ) ;
#32487=VERTEX_POINT ( 'NONE', #17761 ) ;
#32488=ORIENTED_EDGE ( 'NONE', *, *, #2344, .T. ) ;
#32489=CARTESIAN_POINT ( 'NONE',  ( -5.405949406249996869, 9.363379034771805109, -29.34375000204836326 ) ) ;
#32491=CARTESIAN_POINT ( 'NONE',  ( 7.644554776091147741E-16, 12.48450537969573659, -194.4687500020484094 ) ) ;
#32492=CARTESIAN_POINT ( 'NONE',  ( 5.405949406249999534, 9.363379034771803333, -52.09375000204835260 ) ) ;
#32493=CARTESIAN_POINT ( 'NONE',  ( -9.999999999999479527, -5.773502691896549521, -72.00000000409676204 ) ) ;
#32495=CARTESIAN_POINT ( 'NONE',  ( 5.405949406249992428, -9.363379034771808662, -192.0937500020484094 ) ) ;
#32496=CARTESIAN_POINT ( 'NONE',  ( -2.293366432827344421E-15, -12.48450537969573659, -168.2187500020483810 ) ) ;
#32501=CARTESIAN_POINT ( 'NONE',  ( -10.81189881249999729, 1.324075727343319199E-15, -107.0937500020483810 ) ) ;
#32502=CARTESIAN_POINT ( 'NONE',  ( 7.070501591499376803E-16, 11.54700538379251284, -196.6250000000000284 ) ) ;
#32503=CARTESIAN_POINT ( 'NONE',  ( -5.405949406250003975, -9.363379034771801557, -77.03125000204838102 ) ) ;
#32506=CARTESIAN_POINT ( 'NONE',  ( 5.405949406249999534, 9.363379034771803333, -85.09375000204836681 ) ) ;
#32507=ADVANCED_FACE ( 'NONE', ( #34200 ), #754, .T. ) ;
#32509=CARTESIAN_POINT ( 'NONE',  ( 10.00000000000000000, 5.773502691896255534, -149.2500000040968189 ) ) ;
#32515=CARTESIAN_POINT ( 'NONE',  ( -10.81189881249999729, 1.324075727343319199E-15, -197.2812500020484094 ) ) ;
#32519=CARTESIAN_POINT ( 'NONE',  ( 5.000000000000000000, 8.660254037844385522, -55.74999999999996447 ) ) ;
#32521=CARTESIAN_POINT ( 'NONE',  ( 5.000000000000000000, 8.660254037844385522, -72.62500000409677625 ) ) ;
#32523=CARTESIAN_POINT ( 'NONE',  ( 9.999999999999998224, 0.000000000000000000, -159.8750000040967905 ) ) ;
#32525=CARTESIAN_POINT ( 'NONE',  ( 5.405949406249992428, -9.363379034771808662, -66.28125000204838102 ) ) ;
#32529=CARTESIAN_POINT ( 'NONE',  ( 10.81189881249999729, 0.000000000000000000, -192.0312500020484094 ) ) ;
#32530=AXIS2_PLACEMENT_3D ( 'NONE', #23990, #14019, #1326 ) ;
#32532=CARTESIAN_POINT ( 'NONE',  ( 5.405949406249992428, -9.363379034771808662, -0.09375000204836503315 ) ) ;
#32533=DIRECTION ( 'NONE',  ( -0.000000000000000000, -0.000000000000000000, 1.000000000000000000 ) ) ;
#32534=CARTESIAN_POINT ( 'NONE',  ( -9.439719357620422358, -3.412429525893140525, -0.000000000000000000 ) ) ;
#32535=CARTESIAN_POINT ( 'NONE',  ( 5.000000000000000000, 8.660254037844385522, -159.6250000040967905 ) ) ;
#32536=CARTESIAN_POINT ( 'NONE',  ( -2.121150477449813534E-15, -11.54700538379251284, -176.3750000000000000 ) ) ;
#32537=CARTESIAN_POINT ( 'NONE',  ( 10.00000000000000000, 5.773502691896255534, -166.8750000000000000 ) ) ;
#32538=CARTESIAN_POINT ( 'NONE',  ( 5.405949406249999534, 9.363379034771803333, -94.28125000204838102 ) ) ;
#32539=VERTEX_POINT ( 'NONE', #1387 ) ;
#32540=CARTESIAN_POINT ( 'NONE',  ( 4.999999999999992006, -8.660254037844389075, -161.6250000040967905 ) ) ;
#32541=VERTEX_POINT ( 'NONE', #34622 ) ;
#32543=CARTESIAN_POINT ( 'NONE',  ( 10.81189881249999551, -6.242252689847874514, -34.46875000204835260 ) ) ;
#32544=CARTESIAN_POINT ( 'NONE',  ( -5.405949406250003975, -9.363379034771801557, -30.53125000204837036 ) ) ;
#32546=CARTESIAN_POINT ( 'NONE',  ( 7.644554776091147741E-16, 12.48450537969573659, -75.96875000204838102 ) ) ;
#32548=CARTESIAN_POINT ( 'NONE',  ( -10.81189881249999729, 1.324075727343319199E-15, -191.0937500020484094 ) ) ;
#32549=( BOUNDED_CURVE ( )  B_SPLINE_CURVE ( 2, ( #42157, #41946, #11960, #24946, #34650, #21684, #25150 ),
 .UNSPECIFIED., .F., .F. ) 
 B_SPLINE_CURVE_WITH_KNOTS ( ( 3, 2, 2, 3 ),
 ( 0.2500000000000001110, 0.2512437810945274963, 0.2524875621890548261, 0.2537313432835822113 ),
 .UNSPECIFIED. ) 
 CURVE ( )  GEOMETRIC_REPRESENTATION_ITEM ( )  RATIONAL_B_SPLINE_CURVE ( ( 0.9999999999999880096, 0.8660254037844506980, 1.000000000000000000, 0.8660254037844387076, 1.000000000000000000, 0.8660254037844267172, 1.000000000000011990 ) ) 
 REPRESENTATION_ITEM ( '' )  );
#32551=DIRECTION ( 'NONE',  ( -0.000000000000000000, -0.000000000000000000, 1.000000000000000000 ) ) ;
#32553=CARTESIAN_POINT ( 'NONE',  ( 5.000000000000000000, 8.660254037844385522, -11.12500000409674605 ) ) ;
#32555=CARTESIAN_POINT ( 'NONE',  ( 9.999999999999998224, 0.000000000000000000, -50.37500000409675494 ) ) ;
#32556=CARTESIAN_POINT ( 'NONE',  ( 10.81189881249999729, 0.000000000000000000, -130.3437500020484094 ) ) ;
#32557=CARTESIAN_POINT ( 'NONE',  ( 10.81189881249999729, 0.000000000000000000, -102.0312500020483952 ) ) ;
#32558=EDGE_CURVE ( 'NONE', #12272, #25832, #27415, .T. ) ;
#32559=CARTESIAN_POINT ( 'NONE',  ( 5.405949406249992428, -9.363379034771808662, -108.0937500020483810 ) ) ;
#32562=CARTESIAN_POINT ( 'NONE',  ( 7.070501591499377789E-16, 11.54700538379251284, -171.5000000040967905 ) ) ;
#32563=EDGE_CURVE ( 'NONE', #1542, #3313, #6729, .T. ) ;
#32564=CARTESIAN_POINT ( 'NONE',  ( 4.999999999999992006, -8.660254037844389075, -133.1250000040967620 ) ) ;
#32567=EDGE_CURVE ( 'NONE', #15830, #29288, #8127, .T. ) ;
#32569=CARTESIAN_POINT ( 'NONE',  ( -9.999999999999998224, 1.224646799147353059E-15, -4.249999999999976019 ) ) ;
#32571=CARTESIAN_POINT ( 'NONE',  ( -9.999999999999998224, 1.224646799147353059E-15, -172.2500000000000000 ) ) ;
#32573=CARTESIAN_POINT ( 'NONE',  ( 4.999999999999992006, -8.660254037844389075, -89.24999999999998579 ) ) ;
#32575=CARTESIAN_POINT ( 'NONE',  ( 5.000000000000000000, 8.660254037844385522, -101.1250000040967905 ) ) ;
#32576=DIRECTION ( 'NONE',  ( 1.000000000000000000, 0.000000000000000000, 0.000000000000000000 ) ) ;
#32579=CARTESIAN_POINT ( 'NONE',  ( -10.81189881249999729, 1.324075727343319199E-15, -89.28125000204838102 ) ) ;
#32581=AXIS2_PLACEMENT_3D ( 'NONE', #14184, #17433, #37519 ) ;
#32585=ORIENTED_EDGE ( 'NONE', *, *, #9473, .T. ) ;
#32586=CARTESIAN_POINT ( 'NONE',  ( -2.121150477449813534E-15, -11.54700538379251284, -15.87499999999998046 ) ) ;
#32587=CARTESIAN_POINT ( 'NONE',  ( -9.999999999999998224, 5.773502691896259087, -152.8749999999999716 ) ) ;
#32590=CARTESIAN_POINT ( 'NONE',  ( 9.999999999999998224, 0.000000000000000000, -200.0000000000000000 ) ) ;
#32591=CARTESIAN_POINT ( 'NONE',  ( -10.81189881249999729, 6.242252689847871849, -125.4062500020483810 ) ) ;
#32592=ORIENTED_EDGE ( 'NONE', *, *, #5401, .T. ) ;
#32593=CARTESIAN_POINT ( 'NONE',  ( -4.999999999999996447, 8.660254037844387298, -89.99999999999998579 ) ) ;
#32594=ORIENTED_EDGE ( 'NONE', *, *, #20835, .F. ) ;
#32596=CARTESIAN_POINT ( 'NONE',  ( 5.405949406249999534, 9.363379034771803333, -53.78125000204836681 ) ) ;
#32598=CARTESIAN_POINT ( 'NONE',  ( -5.405949406250003975, -9.363379034771801557, -105.3437500020483810 ) ) ;
#32600=ORIENTED_EDGE ( 'NONE', *, *, #6144, .T. ) ;
#32601=CARTESIAN_POINT ( 'NONE',  ( 0.000000000000000000, 0.000000000000000000, -200.0000000000000000 ) ) ;
#32602=CARTESIAN_POINT ( 'NONE',  ( -2.121150477449813534E-15, -11.54700538379251284, -125.7500000040967763 ) ) ;
#32603=( BOUNDED_CURVE ( )  B_SPLINE_CURVE ( 2, ( #417, #16774, #26309, #10100, #6659, #13537, #29542 ),
 .UNSPECIFIED., .F., .F. ) 
 B_SPLINE_CURVE_WITH_KNOTS ( ( 3, 2, 2, 3 ),
 ( 0.7537313432835822669, 0.7549751243781096521, 0.7562189054726369264, 0.7574626865671643117 ),
 .UNSPECIFIED. ) 
 CURVE ( )  GEOMETRIC_REPRESENTATION_ITEM ( )  RATIONAL_B_SPLINE_CURVE ( ( 0.9999999999999761302, 0.8660254037844625774, 1.000000000000000000, 0.8660254037844387076, 1.000000000000000000, 0.8660254037844267172, 1.000000000000011990 ) ) 
 REPRESENTATION_ITEM ( '' )  );
#32605=CARTESIAN_POINT ( 'NONE',  ( 10.81189881249999729, 0.000000000000000000, -2.843750002048367698 ) ) ;
#32607=CARTESIAN_POINT ( 'NONE',  ( -2.293366432827344421E-15, -12.48450537969573659, -132.2187500020483810 ) ) ;
#32609=CARTESIAN_POINT ( 'NONE',  ( -9.999999999999998224, 1.224646799147353059E-15, -148.2500000000000000 ) ) ;
#32611=CARTESIAN_POINT ( 'NONE',  ( -4.999999999999996447, 8.660254037844387298, -193.8750000040967905 ) ) ;
#32613=CARTESIAN_POINT ( 'NONE',  ( 10.81189881249999551, -6.242252689847874514, -184.6562500020484094 ) ) ;
#32614=CARTESIAN_POINT ( 'NONE',  ( -4.999999999999996447, 8.660254037844387298, -148.8750000040967905 ) ) ;
#32617=CARTESIAN_POINT ( 'NONE',  ( -5.405949406249996869, 9.363379034771805109, -65.34375000204836681 ) ) ;
#32618=CARTESIAN_POINT ( 'NONE',  ( -10.81189881249999907, -6.242252689847864744, -49.96875000204835970 ) ) ;
#32620=CARTESIAN_POINT ( 'NONE',  ( -5.405949406249996869, 9.363379034771805109, -16.03125000204835970 ) ) ;
#32624=CARTESIAN_POINT ( 'NONE',  ( -5.000000000000003553, -8.660254037844383745, -113.4999999999999858 ) ) ;
#32628=CARTESIAN_POINT ( 'NONE',  ( 10.81189881249999729, 0.000000000000000000, -118.5312500020483952 ) ) ;
#32630=FACE_OUTER_BOUND ( 'NONE', #23348, .T. ) ;
#32634=ORIENTED_EDGE ( 'NONE', *, *, #4523, .F. ) ;
#32635=CARTESIAN_POINT ( 'NONE',  ( -2.121150477449813534E-15, -11.54700538379251284, -44.37499999999997158 ) ) ;
#32636=EDGE_CURVE ( 'NONE', #35567, #23620, #12519, .T. ) ;
#32637=CARTESIAN_POINT ( 'NONE',  ( -9.999999999999998224, 5.773502691896259087, -19.75000000409677270 ) ) ;
#32638=CARTESIAN_POINT ( 'NONE',  ( -10.81189881249999729, -6.242252689847864744, -41.15625000204836681 ) ) ;
#32641=DIRECTION ( 'NONE',  ( 1.000000000000000000, 0.000000000000000000, 0.000000000000000000 ) ) ;
#32642=CARTESIAN_POINT ( 'NONE',  ( -10.81189881249999729, 6.242252689847871849, -140.4062500020484094 ) ) ;
#32643=CARTESIAN_POINT ( 'NONE',  ( -10.81189881249999729, 1.324075727343319199E-15, -149.2812500020483810 ) ) ;
#32645=ORIENTED_EDGE ( 'NONE', *, *, #11274, .F. ) ;
#32647=ORIENTED_EDGE ( 'NONE', *, *, #22279, .T. ) ;
#32648=CARTESIAN_POINT ( 'NONE',  ( -5.405949406250003975, -9.363379034771801557, -175.8437500020483810 ) ) ;
#32649=CARTESIAN_POINT ( 'NONE',  ( -5.405949406250003975, -9.363379034771801557, -19.84375000204835615 ) ) ;
#32651=CARTESIAN_POINT ( 'NONE',  ( -2.293366432827344421E-15, -12.48450537969573659, -160.7187500020483810 ) ) ;
#32652=CARTESIAN_POINT ( 'NONE',  ( -10.81189881249999729, 6.242252689847871849, -141.7187500020483810 ) ) ;
#32656=CARTESIAN_POINT ( 'NONE',  ( 10.81189881249999729, 0.000000000000000000, -14.84375000204835082 ) ) ;
#32662=CARTESIAN_POINT ( 'NONE',  ( 10.81189881249999907, 6.242252689847868297, -71.71875000204838102 ) ) ;
#32663=CARTESIAN_POINT ( 'NONE',  ( 5.405949406249999534, 9.363379034771803333, -53.78125000204836681 ) ) ;
#32665=CARTESIAN_POINT ( 'NONE',  ( -10.00000000000051337, 5.773502691895962435, -90.25000000409679046 ) ) ;
#32667=CARTESIAN_POINT ( 'NONE',  ( -9.999999999999998224, 1.224646799147353059E-15, -139.2499999999999716 ) ) ;
#32668=CARTESIAN_POINT ( 'NONE',  ( 10.81189881249999729, 0.000000000000000000, -139.5312500020484094 ) ) ;
#32669=( BOUNDED_CURVE ( )  B_SPLINE_CURVE ( 2, ( #8064, #27486, #11061, #24262, #37409, #27699, #7851 ),
 .UNSPECIFIED., .F., .F. ) 
 B_SPLINE_CURVE_WITH_KNOTS ( ( 3, 2, 2, 3 ),
 ( 0.7798507462686569136, 0.7810945273631842989, 0.7823383084577115731, 0.7835820895522389584 ),
 .UNSPECIFIED. ) 
 CURVE ( )  GEOMETRIC_REPRESENTATION_ITEM ( )  RATIONAL_B_SPLINE_CURVE ( ( 0.9999999999999761302, 0.8660254037844625774, 1.000000000000000000, 0.8660254037844387076, 1.000000000000000000, 0.8660254037844267172, 1.000000000000011990 ) ) 
 REPRESENTATION_ITEM ( '' )  );
#32670=CARTESIAN_POINT ( 'NONE',  ( -2.121150477449813534E-15, -11.54700538379251284, -98.75000000409677625 ) ) ;
#32671=CARTESIAN_POINT ( 'NONE',  ( -4.999999999999996447, 8.660254037844387298, -114.3750000040967763 ) ) ;
#32676=CARTESIAN_POINT ( 'NONE',  ( -5.000000000000003553, -8.660254037844383745, -22.37500000409675494 ) ) ;
#32677=CARTESIAN_POINT ( 'NONE',  ( -10.81189881249999729, 6.242252689847871849, -176.4062500020484094 ) ) ;
#32678=CARTESIAN_POINT ( 'NONE',  ( -4.999999999999996447, 8.660254037844387298, -43.87500000409677625 ) ) ;
#32679=CARTESIAN_POINT ( 'NONE',  ( 0.000000000000000000, 0.000000000000000000, -200.0000000000000000 ) ) ;
#32681=CARTESIAN_POINT ( 'NONE',  ( 9.999999999999612754, 5.773502691896477579, -156.3750000000000000 ) ) ;
#32682=CARTESIAN_POINT ( 'NONE',  ( -2.293366432827344421E-15, -12.48450537969573659, -163.9062500020483810 ) ) ;
#32683=CARTESIAN_POINT ( 'NONE',  ( -10.81189881249999729, 1.324075727343319199E-15, -140.0937500020483810 ) ) ;
#32684=CARTESIAN_POINT ( 'NONE',  ( 5.000000000000000000, 8.660254037844385522, -100.7499999999999858 ) ) ;
#32685=VERTEX_POINT ( 'NONE', #41500 ) ;
#32686=DIRECTION ( 'NONE',  ( -0.000000000000000000, -0.000000000000000000, 1.000000000000000000 ) ) ;
#32687=ADVANCED_FACE ( 'NONE', ( #2665 ), #5904, .T. ) ;
#32688=CARTESIAN_POINT ( 'NONE',  ( 10.81189881249999907, 6.242252689847868297, -71.90625000204836681 ) ) ;
#32689=ORIENTED_EDGE ( 'NONE', *, *, #9324, .T. ) ;
#32691=CARTESIAN_POINT ( 'NONE',  ( -2.293366432827344421E-15, -12.48450537969573659, -118.7187500020483952 ) ) ;
#32692=ORIENTED_EDGE ( 'NONE', *, *, #34286, .F. ) ;
#32693=ORIENTED_EDGE ( 'NONE', *, *, #42683, .T. ) ;
#32694=CARTESIAN_POINT ( 'NONE',  ( -5.405949406250003975, -9.363379034771801557, -24.34375000204835970 ) ) ;
#32695=CARTESIAN_POINT ( 'NONE',  ( -5.405949406249996869, 9.363379034771805109, -197.3437500020484094 ) ) ;
#32696=CARTESIAN_POINT ( 'NONE',  ( -5.405949406249996869, 9.363379034771805109, -45.84375000204838102 ) ) ;
#32697=DIRECTION ( 'NONE',  ( 1.000000000000000000, 0.000000000000000000, 0.000000000000000000 ) ) ;
#32699=CARTESIAN_POINT ( 'NONE',  ( -10.81189881249999729, -6.242252689847864744, -187.9687500020484094 ) ) ;
#32700=CARTESIAN_POINT ( 'NONE',  ( -10.81189881249999729, 1.324075727343319199E-15, -168.5937500020484094 ) ) ;
#32704=DIRECTION ( 'NONE',  ( -0.000000000000000000, -0.000000000000000000, 1.000000000000000000 ) ) ;
#32706=CARTESIAN_POINT ( 'NONE',  ( -5.405949406250003975, -9.363379034771801557, -99.34375000204838102 ) ) ;
#32707=CARTESIAN_POINT ( 'NONE',  ( 9.999999999999998224, 0.000000000000000000, -108.8750000040967763 ) ) ;
#32708=CARTESIAN_POINT ( 'NONE',  ( -5.405949406250003975, -9.363379034771801557, -75.53125000204838102 ) ) ;
#32709=CARTESIAN_POINT ( 'NONE',  ( -9.999999999999998224, 1.224646799147353059E-15, -200.0000000000000000 ) ) ;
#32711=CARTESIAN_POINT ( 'NONE',  ( 10.81189881249999729, 6.242252689847867408, -158.9062500020483810 ) ) ;
#32713=CARTESIAN_POINT ( 'NONE',  ( 9.999999999999998224, 0.000000000000000000, -134.3750000040967905 ) ) ;
#32715=ORIENTED_EDGE ( 'NONE', *, *, #29931, .F. ) ;
#32718=CARTESIAN_POINT ( 'NONE',  ( 7.644554776091147741E-16, 12.48450537969573659, -194.6562500020484094 ) ) ;
#32721=ORIENTED_EDGE ( 'NONE', *, *, #41568, .F. ) ;
#32722=CARTESIAN_POINT ( 'NONE',  ( 5.000000000000000000, 8.660254037844385522, -54.24999999999996447 ) ) ;
#32724=CARTESIAN_POINT ( 'NONE',  ( 9.999999999999996447, -5.773502691896262640, -76.00000000409677625 ) ) ;
#32725=LINE ( 'NONE', #9625, #22393 ) ;
#32726=CARTESIAN_POINT ( 'NONE',  ( 4.999999999999992006, -8.660254037844389075, -160.1250000040967905 ) ) ;
#32728=CARTESIAN_POINT ( 'NONE',  ( -10.81189881249999729, 1.324075727343319199E-15, -68.28125000204838102 ) ) ;
#32731=DIRECTION ( 'NONE',  ( -0.000000000000000000, -0.000000000000000000, 1.000000000000000000 ) ) ;
#32732=CARTESIAN_POINT ( 'NONE',  ( -10.81189881249999729, 1.324075727343319199E-15, -185.2812500020484094 ) ) ;
#32734=CARTESIAN_POINT ( 'NONE',  ( -9.999999999999998224, 1.224646799147353059E-15, -85.24999999999997158 ) ) ;
#32735=CARTESIAN_POINT ( 'NONE',  ( 9.999999999999998224, 0.000000000000000000, -149.0000000000000000 ) ) ;
#32736=CARTESIAN_POINT ( 'NONE',  ( 10.00000000000154010, -5.773502691895370020, -62.50000000409673362 ) ) ;
#32737=CARTESIAN_POINT ( 'NONE',  ( -5.755749739768639017, 8.223921721521577410, 0.000000000000000000 ) ) ;
#32738=CARTESIAN_POINT ( 'NONE',  ( 9.999999999999996447, -5.773502691896262640, -167.1250000000000000 ) ) ;
#32739=DIRECTION ( 'NONE',  ( 1.000000000000000000, 0.000000000000000000, 0.000000000000000000 ) ) ;
#32740=CARTESIAN_POINT ( 'NONE',  ( -10.81189881249999729, 1.324075727343319199E-15, -92.28125000204838102 ) ) ;
#32742=CARTESIAN_POINT ( 'NONE',  ( 10.00000000000012257, -5.773502691896188921, -162.6250000000000568 ) ) ;
#32743=EDGE_CURVE ( 'NONE', #4341, #18779, #30196, .T. ) ;
#32747=CARTESIAN_POINT ( 'NONE',  ( -10.81189881249999907, -6.242252689847864744, -33.46875000204834549 ) ) ;
#32748=AXIS2_PLACEMENT_3D ( 'NONE', #12341, #35466, #9122 ) ;
#32749=CARTESIAN_POINT ( 'NONE',  ( -2.293366432827344421E-15, -12.48450537969573659, -25.90625000204838813 ) ) ;
#32750=CARTESIAN_POINT ( 'NONE',  ( 10.81189881249999907, 6.242252689847868297, -82.21875000204836681 ) ) ;
#32751=DIRECTION ( 'NONE',  ( 1.000000000000000000, 0.000000000000000000, 0.000000000000000000 ) ) ;
#32752=CARTESIAN_POINT ( 'NONE',  ( -10.81189881249999907, -6.242252689847864744, -192.4687500020484094 ) ) ;
#32756=CARTESIAN_POINT ( 'NONE',  ( 4.999999999999992006, -8.660254037844389075, 0.3749999959032357388 ) ) ;
#32758=CARTESIAN_POINT ( 'NONE',  ( -10.81189881249999907, -6.242252689847864744, -120.4687500020483810 ) ) ;
#32759=CARTESIAN_POINT ( 'NONE',  ( 10.81189881249999729, 0.000000000000000000, -97.53125000204839523 ) ) ;
#32760=CARTESIAN_POINT ( 'NONE',  ( -10.81189881249999729, 6.242252689847871849, -104.2187500020483810 ) ) ;
#32762=VECTOR ( 'NONE', #30022, 1000.000000000000000 ) ;
#32764=CARTESIAN_POINT ( 'NONE',  ( 5.000000000000000000, 8.660254037844385522, -168.6250000040967905 ) ) ;
#32765=DIRECTION ( 'NONE',  ( 1.000000000000000000, 0.000000000000000000, 0.000000000000000000 ) ) ;
#32769=CARTESIAN_POINT ( 'NONE',  ( -9.999999999999998224, 1.224646799147353059E-15, -79.62500000409677625 ) ) ;
#32773=CARTESIAN_POINT ( 'NONE',  ( 4.999999999999992006, -8.660254037844389075, -84.74999999999997158 ) ) ;
#32775=CARTESIAN_POINT ( 'NONE',  ( 7.070501591499377789E-16, 11.54700538379251284, -95.00000000409677625 ) ) ;
#32776=CYLINDRICAL_SURFACE ( 'NONE', #15504, 9.999999999999998224 ) ;
#32778=CARTESIAN_POINT ( 'NONE',  ( 10.81189881249999729, 6.242252689847867408, -88.40625000204836681 ) ) ;
#32781=LINE ( 'NONE', #29760, #18769 ) ;
#32784=CARTESIAN_POINT ( 'NONE',  ( 10.00000000000000000, 5.773502691896255534, -10.87499999999995381 ) ) ;
#32785=CARTESIAN_POINT ( 'NONE',  ( 9.999999999999996447, -5.773502691896262640, -146.1250000000000000 ) ) ;
#32787=CARTESIAN_POINT ( 'NONE',  ( -4.999999999999996447, 8.660254037844387298, -196.5000000000000000 ) ) ;
#32788=CARTESIAN_POINT ( 'NONE',  ( -2.293366432827344421E-15, -12.48450537969573659, -114.4062500020483952 ) ) ;
#32789=ORIENTED_EDGE ( 'NONE', *, *, #19490, .F. ) ;
#32791=EDGE_CURVE ( 'NONE', #8276, #13430, #31601, .T. ) ;
#32792=( BOUNDED_CURVE ( )  B_SPLINE_CURVE ( 2, ( #37019, #7459, #7892, #4645, #11318, #37664, #24085 ),
 .UNSPECIFIED., .F., .F. ) 
 B_SPLINE_CURVE_WITH_KNOTS ( ( 3, 2, 2, 3 ),
 ( 0.2014925373134328901, 0.2027363184079602476, 0.2039800995024875774, 0.2052238805970149627 ),
 .UNSPECIFIED. ) 
 CURVE ( )  GEOMETRIC_REPRESENTATION_ITEM ( )  RATIONAL_B_SPLINE_CURVE ( ( 0.9999999999999940048, 0.8660254037844447028, 1.000000000000000000, 0.8660254037844387076, 1.000000000000000000, 0.8660254037844357100, 1.000000000000002887 ) ) 
 REPRESENTATION_ITEM ( '' )  );
#32795=ORIENTED_EDGE ( 'NONE', *, *, #27856, .T. ) ;
#32797=CARTESIAN_POINT ( 'NONE',  ( 10.81189881249999729, 0.000000000000000000, -48.03125000204838813 ) ) ;
#32799=CARTESIAN_POINT ( 'NONE',  ( -10.81189881249999907, -6.242252689847864744, -99.46875000204838102 ) ) ;
#32800=CARTESIAN_POINT ( 'NONE',  ( -10.81189881249999729, -6.242252689847864744, -123.6562500020484094 ) ) ;
#32801=VERTEX_POINT ( 'NONE', #28362 ) ;
#32807=CARTESIAN_POINT ( 'NONE',  ( 10.81189881249999551, -6.242252689847874514, -1.468750002048354819 ) ) ;
#32808=FACE_OUTER_BOUND ( 'NONE', #40731, .T. ) ;
#32809=ADVANCED_FACE ( 'NONE', ( #25125 ), #8717, .T. ) ;
#32810=CARTESIAN_POINT ( 'NONE',  ( -5.405949406249996869, 9.363379034771805109, -135.8437500020484094 ) ) ;
#32812=CARTESIAN_POINT ( 'NONE',  ( 9.999999999999998224, 0.000000000000000000, -116.3750000040967905 ) ) ;
#32814=CARTESIAN_POINT ( 'NONE',  ( 4.999999999999992006, -8.660254037844389075, -191.6250000040967905 ) ) ;
#32816=CARTESIAN_POINT ( 'NONE',  ( -10.81189881249999729, 6.242252689847871849, -186.9062500020484094 ) ) ;
#32817=CARTESIAN_POINT ( 'NONE',  ( 7.070501591499376803E-16, 11.54700538379251284, -6.500000004096742501 ) ) ;
#32820=EDGE_CURVE ( 'NONE', #16786, #8228, #15541, .T. ) ;
#32821=CARTESIAN_POINT ( 'NONE',  ( -5.405949406249996869, 9.363379034771805109, -60.84375000204836681 ) ) ;
#32822=CARTESIAN_POINT ( 'NONE',  ( -10.81189881249999907, -6.242252689847864744, -52.96875000204838102 ) ) ;
#32824=CARTESIAN_POINT ( 'NONE',  ( 5.405949406249992428, -9.363379034771808662, -19.78125000204836326 ) ) ;
#32826=CARTESIAN_POINT ( 'NONE',  ( -4.999999999999996447, 8.660254037844387298, -27.37500000409676204 ) ) ;
#32828=CARTESIAN_POINT ( 'NONE',  ( -10.00000000000000000, -5.773502691896251982, -106.1249999999999858 ) ) ;
#32830=EDGE_CURVE ( 'NONE', #33229, #27592, #19957, .T. ) ;
#32831=CARTESIAN_POINT ( 'NONE',  ( -4.999999999999996447, 8.660254037844387298, -163.5000000000000000 ) ) ;
#32835=CARTESIAN_POINT ( 'NONE',  ( -5.405949406250003975, -9.363379034771801557, -114.5312500020483952 ) ) ;
#32842=CARTESIAN_POINT ( 'NONE',  ( 10.00000000000000000, 5.773502691896255534, -39.37499999999996447 ) ) ;
#32843=CARTESIAN_POINT ( 'NONE',  ( -9.999999999999998224, 1.224646799147353059E-15, -18.12500000409675138 ) ) ;
#32844=CARTESIAN_POINT ( 'NONE',  ( 5.405949406249999534, 9.363379034771803333, -44.78125000204838102 ) ) ;
#32848=EDGE_CURVE ( 'NONE', #21106, #37675, #38484, .T. ) ;
#32849=( BOUNDED_CURVE ( )  B_SPLINE_CURVE ( 2, ( #8506, #21229, #24278, #21660, #4833, #34840, #5264 ),
 .UNSPECIFIED., .F., .F. ) 
 B_SPLINE_CURVE_WITH_KNOTS ( ( 3, 2, 2, 3 ),
 ( 0.5783582089552241623, 0.5796019900497515476, 0.5808457711442788218, 0.5820895522388062071 ),
 .UNSPECIFIED. ) 
 CURVE ( )  GEOMETRIC_REPRESENTATION_ITEM ( )  RATIONAL_B_SPLINE_CURVE ( ( 0.9999999999999641398, 0.8660254037844745678, 1.000000000000000000, 0.8660254037844387076, 1.000000000000000000, 0.8660254037844148378, 1.000000000000023981 ) ) 
 REPRESENTATION_ITEM ( '' )  );
#32851=CARTESIAN_POINT ( 'NONE',  ( -10.81189881249999729, 1.324075727343319199E-15, -137.2812500020483810 ) ) ;
#32852=CARTESIAN_POINT ( 'NONE',  ( 10.81189881249999551, -6.242252689847874514, -144.1562500020484094 ) ) ;
#32853=EDGE_LOOP ( 'NONE', ( #27864, #32958, #16870, #24522 ) ) ;
#32855=EDGE_LOOP ( 'NONE', ( #32208, #34290, #2910, #20149 ) ) ;
#32856=VERTEX_POINT ( 'NONE', #32030 ) ;
#32857=CARTESIAN_POINT ( 'NONE',  ( -9.999999999999998224, 1.224646799147353059E-15, -130.2499999999999716 ) ) ;
#32858=CARTESIAN_POINT ( 'NONE',  ( -5.405949406250003975, -9.363379034771801557, -172.8437500020484094 ) ) ;
#32859=CARTESIAN_POINT ( 'NONE',  ( -10.81189881249999729, 6.242252689847871849, -26.21875000204837391 ) ) ;
#32860=CARTESIAN_POINT ( 'NONE',  ( 9.999999999999998224, 0.000000000000000000, -200.0000000000000000 ) ) ;
#32861=CARTESIAN_POINT ( 'NONE',  ( -10.81189881249999729, 6.242252689847871849, -153.7187500020483810 ) ) ;
#32862=CARTESIAN_POINT ( 'NONE',  ( -10.81189881249999729, 1.324075727343319199E-15, -143.0937500020483810 ) ) ;
#32863=CARTESIAN_POINT ( 'NONE',  ( -9.999999999999998224, 1.224646799147353059E-15, -10.24999999999995381 ) ) ;
#32866=CARTESIAN_POINT ( 'NONE',  ( -10.81189881249999729, 1.324075727343319199E-15, -21.59375000204835615 ) ) ;
#32868=CYLINDRICAL_SURFACE ( 'NONE', #3326, 9.999999999999998224 ) ;
#32872=CARTESIAN_POINT ( 'NONE',  ( -2.293366432827344421E-15, -12.48450537969573659, -70.71875000204839523 ) ) ;
#32873=CARTESIAN_POINT ( 'NONE',  ( 5.405949406249992428, -9.363379034771808662, -42.28125000204838102 ) ) ;
#32877=CARTESIAN_POINT ( 'NONE',  ( -9.999999999999998224, 5.773502691896259087, -128.8749999999999716 ) ) ;
#32878=CARTESIAN_POINT ( 'NONE',  ( 5.405949406249999534, 9.363379034771803333, -134.7812500020483810 ) ) ;
#32880=CARTESIAN_POINT ( 'NONE',  ( -2.121150477449813534E-15, -11.54700538379251284, -116.7500000040967905 ) ) ;
#32886=CARTESIAN_POINT ( 'NONE',  ( 10.81189881249999907, 6.242252689847868297, -173.9062500020484094 ) ) ;
#32887=CARTESIAN_POINT ( 'NONE',  ( -2.121150477449813534E-15, -11.54700538379251284, -40.25000000409676204 ) ) ;
#32888=CARTESIAN_POINT ( 'NONE',  ( 4.999999999999992006, -8.660254037844389075, -91.12500000409677625 ) ) ;
#32890=CARTESIAN_POINT ( 'NONE',  ( -10.00000000000038547, 5.773502691896036154, -155.8749999999999432 ) ) ;
#32891=CARTESIAN_POINT ( 'NONE',  ( 10.81189881249999907, 6.242252689847868297, -157.4062500020483810 ) ) ;
#32892=CARTESIAN_POINT ( 'NONE',  ( 10.81189881249999729, 0.000000000000000000, -146.8437500020483810 ) ) ;
#32893=CARTESIAN_POINT ( 'NONE',  ( -9.999999999998456346, -5.773502691897145489, -51.00000000409671941 ) ) ;
#32894=CARTESIAN_POINT ( 'NONE',  ( -9.999999999999998224, 1.224646799147353059E-15, -200.0000000000000000 ) ) ;
#32895=EDGE_LOOP ( 'NONE', ( #29137, #2637, #17962, #32957 ) ) ;
#32897=CARTESIAN_POINT ( 'NONE',  ( 10.81189881249999729, 0.000000000000000000, -67.53125000204838102 ) ) ;
#32900=CARTESIAN_POINT ( 'NONE',  ( 7.644554776091147741E-16, 12.48450537969573659, -116.4687500020483952 ) ) ;
#32903=CARTESIAN_POINT ( 'NONE',  ( -5.405949406249996869, 9.363379034771805109, -20.34375000204835615 ) ) ;
#32904=CARTESIAN_POINT ( 'NONE',  ( 5.405949406249992428, -9.363379034771808662, -1.781250002048373471 ) ) ;
#32905=CARTESIAN_POINT ( 'NONE',  ( 10.81189881249999551, -6.242252689847874514, -44.96875000204836681 ) ) ;
#32907=FACE_OUTER_BOUND ( 'NONE', #29762, .T. ) ;
#32909=CARTESIAN_POINT ( 'NONE',  ( -10.81189881249999729, 1.324075727343319199E-15, -177.5937500020484094 ) ) ;
#32910=CARTESIAN_POINT ( 'NONE',  ( 10.81189881249999551, -6.242252689847874514, -170.9687500020483810 ) ) ;
#32911=( BOUNDED_CURVE ( )  B_SPLINE_CURVE ( 2, ( #9877, #13092, #23050, #42246, #36207, #18955, #22625 ),
 .UNSPECIFIED., .F., .F. ) 
 B_SPLINE_CURVE_WITH_KNOTS ( ( 3, 2, 2, 3 ),
 ( 0.6604477611940301474, 0.6616915422885575326, 0.6629353233830848069, 0.6641791044776121922 ),
 .UNSPECIFIED. ) 
 CURVE ( )  GEOMETRIC_REPRESENTATION_ITEM ( )  RATIONAL_B_SPLINE_CURVE ( ( 0.9999999999999641398, 0.8660254037844745678, 1.000000000000000000, 0.8660254037844387076, 1.000000000000000000, 0.8660254037844148378, 1.000000000000023981 ) ) 
 REPRESENTATION_ITEM ( '' )  );
#32916=CARTESIAN_POINT ( 'NONE',  ( -5.405949406250003975, -9.363379034771801557, -100.8437500020483810 ) ) ;
#32917=CARTESIAN_POINT ( 'NONE',  ( 10.00000000000000000, 5.773502691896255534, -198.7500000040968189 ) ) ;
#32918=CARTESIAN_POINT ( 'NONE',  ( 10.81189881249999907, 6.242252689847868297, -62.90625000204838813 ) ) ;
#32919=CARTESIAN_POINT ( 'NONE',  ( -9.999999999999998224, 1.224646799147353059E-15, -132.1250000040967620 ) ) ;
#32921=CARTESIAN_POINT ( 'NONE',  ( -10.81189881249999729, -6.242252689847864744, -164.1562500020483810 ) ) ;
#32923=CARTESIAN_POINT ( 'NONE',  ( -9.999999999999998224, 5.773502691896259087, -138.2500000040967905 ) ) ;
#32925=ADVANCED_FACE ( 'NONE', ( #29845 ), #32868, .T. ) ;
#32926=ORIENTED_EDGE ( 'NONE', *, *, #12742, .T. ) ;
#32929=CARTESIAN_POINT ( 'NONE',  ( 7.644554776091147741E-16, 12.48450537969573659, -196.1562500020484379 ) ) ;
#32932=AXIS2_PLACEMENT_3D ( 'NONE', #26491, #33614, #7484 ) ;
#32934=CARTESIAN_POINT ( 'NONE',  ( -5.000000000000003553, -8.660254037844383745, -57.99999999999997158 ) ) ;
#32936=CARTESIAN_POINT ( 'NONE',  ( 7.070501591499377789E-16, 11.54700538379251284, -63.50000000409679046 ) ) ;
#32937=VECTOR ( 'NONE', #23897, 1000.000000000000000 ) ;
#32938=CARTESIAN_POINT ( 'NONE',  ( 7.070501591499376803E-16, 11.54700538379251284, -66.12499999999998579 ) ) ;
#32939=CARTESIAN_POINT ( 'NONE',  ( -2.121150477449813534E-15, -11.54700538379251284, -144.8750000000000000 ) ) ;
#32941=CARTESIAN_POINT ( 'NONE',  ( -10.81189881249999729, -6.242252689847864744, -57.65625000204838102 ) ) ;
#32944=CARTESIAN_POINT ( 'NONE',  ( -9.999999999999998224, 1.224646799147353059E-15, -37.62500000409676915 ) ) ;
#32945=CARTESIAN_POINT ( 'NONE',  ( -5.405949406249996869, 9.363379034771805109, -187.0312500020484094 ) ) ;
#32947=CARTESIAN_POINT ( 'NONE',  ( 7.070501591499376803E-16, 11.54700538379251284, -85.62500000000000000 ) ) ;
#32948=DIRECTION ( 'NONE',  ( -0.000000000000000000, -0.000000000000000000, 1.000000000000000000 ) ) ;
#32949=CARTESIAN_POINT ( 'NONE',  ( 9.999999999999998224, 0.000000000000000000, -62.37500000409676204 ) ) ;
#32951=CARTESIAN_POINT ( 'NONE',  ( 4.999999999999992006, -8.660254037844389075, -165.7500000000000000 ) ) ;
#32952=CARTESIAN_POINT ( 'NONE',  ( -9.999999999999227285, -5.773502691896698735, -138.0000000040967620 ) ) ;
#32953=CARTESIAN_POINT ( 'NONE',  ( -10.81189881249999729, 6.242252689847871849, -93.90625000204839523 ) ) ;
#32955=CARTESIAN_POINT ( 'NONE',  ( -5.000000000000003553, -8.660254037844383745, -163.0000000000000000 ) ) ;
#32957=ORIENTED_EDGE ( 'NONE', *, *, #13792, .F. ) ;
#32958=ORIENTED_EDGE ( 'NONE', *, *, #27310, .T. ) ;
#32959=( BOUNDED_CURVE ( )  B_SPLINE_CURVE ( 2, ( #6794, #16269, #9401, #6171, #19312, #2934, #6382 ),
 .UNSPECIFIED., .F., .F. ) 
 B_SPLINE_CURVE_WITH_KNOTS ( ( 3, 2, 2, 3 ),
 ( 0.5074626865671643117, 0.5087064676616916969, 0.5099502487562189712, 0.5111940298507463565 ),
 .UNSPECIFIED. ) 
 CURVE ( )  GEOMETRIC_REPRESENTATION_ITEM ( )  RATIONAL_B_SPLINE_CURVE ( ( 0.9999999999999880096, 0.8660254037844506980, 1.000000000000000000, 0.8660254037844387076, 1.000000000000000000, 0.8660254037844267172, 1.000000000000011990 ) ) 
 REPRESENTATION_ITEM ( '' )  );
#32961=CARTESIAN_POINT ( 'NONE',  ( 10.81189881249999551, -6.242252689847874514, -31.46875000204835260 ) ) ;
#32962=CARTESIAN_POINT ( 'NONE',  ( 5.405949406249992428, -9.363379034771808662, -22.78125000204836326 ) ) ;
#32963=CARTESIAN_POINT ( 'NONE',  ( 7.644554776091147741E-16, 12.48450537969573659, -72.96875000204835260 ) ) ;
#32964=CARTESIAN_POINT ( 'NONE',  ( -9.999999999999998224, 1.224646799147353059E-15, -200.0000000000000000 ) ) ;
#32967=CARTESIAN_POINT ( 'NONE',  ( -5.405949406250003975, -9.363379034771801557, -190.8437500020484094 ) ) ;
#32968=CARTESIAN_POINT ( 'NONE',  ( -10.81189881249999729, 1.324075727343319199E-15, -149.0937500020483810 ) ) ;
#32969=CARTESIAN_POINT ( 'NONE',  ( 9.999999999999998224, 0.000000000000000000, -132.8750000040967905 ) ) ;
#32972=CARTESIAN_POINT ( 'NONE',  ( 9.999999999999996447, -5.773502691896262640, -7.000000004096744277 ) ) ;
#32973=CARTESIAN_POINT ( 'NONE',  ( -2.121150477449813534E-15, -11.54700538379251284, -80.37499999999997158 ) ) ;
#32974=CARTESIAN_POINT ( 'NONE',  ( -10.81189881249999729, 6.242252689847871849, -120.7187500020483952 ) ) ;
#32975=CARTESIAN_POINT ( 'NONE',  ( 10.81189881249999907, 6.242252689847868297, -95.90625000204839523 ) ) ;
#32976=CARTESIAN_POINT ( 'NONE',  ( -10.81189881249999729, 6.242252689847871849, -107.2187500020483810 ) ) ;
#32979=CARTESIAN_POINT ( 'NONE',  ( -9.999999999999998224, 1.224646799147353059E-15, -163.6250000040967905 ) ) ;
#32980=CARTESIAN_POINT ( 'NONE',  ( 5.000000000000000000, 8.660254037844385522, -81.62500000409676204 ) ) ;
#32989=CARTESIAN_POINT ( 'NONE',  ( 4.999999999999992006, -8.660254037844389075, -80.24999999999998579 ) ) ;
#32991=CARTESIAN_POINT ( 'NONE',  ( -2.121150477449813534E-15, -11.54700538379251284, -86.75000000409677625 ) ) ;
#32994=CARTESIAN_POINT ( 'NONE',  ( -5.405949406250003975, -9.363379034771801557, -90.53125000204838102 ) ) ;
#32997=FACE_OUTER_BOUND ( 'NONE', #29933, .T. ) ;
#32999=VERTEX_POINT ( 'NONE', #42555 ) ;
#33000=CARTESIAN_POINT ( 'NONE',  ( -10.00000000000000000, -5.773502691896251982, -13.12499999999996625 ) ) ;
#33001=CARTESIAN_POINT ( 'NONE',  ( -9.999999999999998224, 1.224646799147353059E-15, -145.2500000000000000 ) ) ;
#33002=FACE_OUTER_BOUND ( 'NONE', #30095, .T. ) ;
#33003=AXIS2_PLACEMENT_3D ( 'NONE', #10654, #27717, #40423 ) ;
#33005=CARTESIAN_POINT ( 'NONE',  ( -5.000000000000003553, -8.660254037844383745, -188.5000000000000000 ) ) ;
#33006=CARTESIAN_POINT ( 'NONE',  ( 5.405949406249992428, -9.363379034771808662, -120.2812500020483952 ) ) ;
#33008=CARTESIAN_POINT ( 'NONE',  ( 0.000000000000000000, 0.000000000000000000, -200.0000000000000000 ) ) ;
#33009=ORIENTED_EDGE ( 'NONE', *, *, #13755, .F. ) ;
#33010=CARTESIAN_POINT ( 'NONE',  ( 5.405949406249999534, 9.363379034771803333, -47.78125000204838813 ) ) ;
#33012=CARTESIAN_POINT ( 'NONE',  ( 7.644554776091147741E-16, 12.48450537969573659, -96.96875000204838102 ) ) ;
#33013=CARTESIAN_POINT ( 'NONE',  ( -2.293366432827344421E-15, -12.48450537969573659, -121.9062500020483952 ) ) ;
#33015=CARTESIAN_POINT ( 'NONE',  ( 4.999999999999992006, -8.660254037844389075, -85.12500000409677625 ) ) ;
#33016=PLANE ( 'NONE',  #30467 ) ;
#33018=DIRECTION ( 'NONE',  ( 1.000000000000000000, 0.000000000000000000, 0.000000000000000000 ) ) ;
#33019=CARTESIAN_POINT ( 'NONE',  ( 10.81189881249999729, 0.000000000000000000, -130.3437500020484094 ) ) ;
#33020=VECTOR ( 'NONE', #537, 1000.000000000000000 ) ;
#33022=LINE ( 'NONE', #5848, #2900 ) ;
#33024=CARTESIAN_POINT ( 'NONE',  ( 10.00000000000000000, 5.773502691896255534, -182.2500000040968189 ) ) ;
#33026=CARTESIAN_POINT ( 'NONE',  ( 10.81189881249999729, 6.242252689847867408, -182.9062500020484094 ) ) ;
#33027=CARTESIAN_POINT ( 'NONE',  ( -4.999999999999996447, 8.660254037844387298, -6.375000004096770034 ) ) ;
#33028=CARTESIAN_POINT ( 'NONE',  ( 0.000000000000000000, 0.000000000000000000, -200.0000000000000000 ) ) ;
#33031=CARTESIAN_POINT ( 'NONE',  ( 5.405949406249999534, 9.363379034771803333, -56.59375000204835970 ) ) ;
#33033=CARTESIAN_POINT ( 'NONE',  ( 5.405949406249999534, 9.363379034771803333, -46.09375000204838102 ) ) ;
#33035=CARTESIAN_POINT ( 'NONE',  ( -10.81189881249999729, 6.242252689847871849, -21.90625000204837036 ) ) ;
#33040=CARTESIAN_POINT ( 'NONE',  ( -4.999999999999996447, 8.660254037844387298, -104.9999999999999858 ) ) ;
#33043=ADVANCED_FACE ( 'NONE', ( #29626 ), #36097, .T. ) ;
#33046=CARTESIAN_POINT ( 'NONE',  ( -5.405949406249996869, 9.363379034771805109, -113.5312500020483952 ) ) ;
#33047=VERTEX_POINT ( 'NONE', #26809 ) ;
#33051=CARTESIAN_POINT ( 'NONE',  ( -5.000000000000003553, -8.660254037844383745, -194.8750000040967905 ) ) ;
#33054=CARTESIAN_POINT ( 'NONE',  ( 7.070501591499377789E-16, 11.54700538379251284, -33.12499999999996447 ) ) ;
#33055=CARTESIAN_POINT ( 'NONE',  ( -9.999999999999998224, 5.773502691896259087, -18.25000000409676559 ) ) ;
#33056=CARTESIAN_POINT ( 'NONE',  ( -2.293366432827344421E-15, -12.48450537969573659, -46.90625000204836681 ) ) ;
#33057=CARTESIAN_POINT ( 'NONE',  ( -2.121150477449813534E-15, -11.54700538379251284, -2.374999999999946709 ) ) ;
#33060=CARTESIAN_POINT ( 'NONE',  ( 10.81189881249999907, 6.242252689847868297, -145.4062500020484094 ) ) ;
#33062=CYLINDRICAL_SURFACE ( 'NONE', #18994, 9.999999999999998224 ) ;
#33063=ORIENTED_EDGE ( 'NONE', *, *, #5029, .F. ) ;
#33065=VERTEX_POINT ( 'NONE', #10391 ) ;
#33067=CARTESIAN_POINT ( 'NONE',  ( 9.999999999999998224, 0.000000000000000000, -129.5000000000000000 ) ) ;
#33068=CARTESIAN_POINT ( 'NONE',  ( -10.81189881249999729, 6.242252689847871849, -171.7187500020483810 ) ) ;
#33069=CARTESIAN_POINT ( 'NONE',  ( 10.81189881249999907, 6.242252689847868297, -26.71875000204838102 ) ) ;
#33071=CARTESIAN_POINT ( 'NONE',  ( -10.81189881249999729, 1.324075727343319199E-15, -158.0937500020483810 ) ) ;
#33072=CARTESIAN_POINT ( 'NONE',  ( 5.405949406249999534, 9.363379034771803333, -148.0937500020483810 ) ) ;
#33073=CARTESIAN_POINT ( 'NONE',  ( 9.999999999999998224, 0.000000000000000000, -9.499999999999953815 ) ) ;
#33076=( BOUNDED_CURVE ( )  B_SPLINE_CURVE ( 2, ( #25636, #38795, #9222, #22390, #15884, #12652, #38999 ),
 .UNSPECIFIED., .F., .F. ) 
 B_SPLINE_CURVE_WITH_KNOTS ( ( 3, 2, 2, 3 ),
 ( 0.8059701492537315604, 0.8072139303482589456, 0.8084577114427863309, 0.8097014925373136052 ),
 .UNSPECIFIED. ) 
 CURVE ( )  GEOMETRIC_REPRESENTATION_ITEM ( )  RATIONAL_B_SPLINE_CURVE ( ( 0.9999999999999761302, 0.8660254037844625774, 1.000000000000000000, 0.8660254037844387076, 1.000000000000000000, 0.8660254037844148378, 1.000000000000023981 ) ) 
 REPRESENTATION_ITEM ( '' )  );
#33077=CARTESIAN_POINT ( 'NONE',  ( 10.81189881249999551, -6.242252689847874514, -10.46875000204836503 ) ) ;
#33079=LINE ( 'NONE', #20965, #37111 ) ;
#33080=CARTESIAN_POINT ( 'NONE',  ( -10.00000000000038547, 5.773502691896036154, -182.8750000000000000 ) ) ;
#33083=CARTESIAN_POINT ( 'NONE',  ( -10.81189881249999729, 1.324075727343319199E-15, -74.09375000204838102 ) ) ;
#33084=CARTESIAN_POINT ( 'NONE',  ( -10.81189881249999729, 6.242252689847871849, -41.40625000204836681 ) ) ;
#33088=ADVANCED_FACE ( 'NONE', ( #9762 ), #16643, .T. ) ;
#33089=CARTESIAN_POINT ( 'NONE',  ( -9.999999999999998224, 1.224646799147353059E-15, -131.7499999999999716 ) ) ;
#33090=CARTESIAN_POINT ( 'NONE',  ( -10.81189881249999729, 1.324075727343319199E-15, -141.7812500020483810 ) ) ;
#33091=CYLINDRICAL_SURFACE ( 'NONE', #2062, 9.999999999999998224 ) ;
#33092=CARTESIAN_POINT ( 'NONE',  ( -9.999999999999998224, 1.224646799147353059E-15, -115.6250000040967905 ) ) ;
#33095=VERTEX_POINT ( 'NONE', #19895 ) ;
#33099=CARTESIAN_POINT ( 'NONE',  ( 23.09401076758504345, 1.040834085586084257E-14, 0.000000000000000000 ) ) ;
#33100=AXIS2_PLACEMENT_3D ( 'NONE', #29979, #10526, #14169 ) ;
#33101=EDGE_CURVE ( 'NONE', #35132, #36368, #33079, .T. ) ;
#33102=CARTESIAN_POINT ( 'NONE',  ( -5.405949406250003975, -9.363379034771801557, -162.5312500020484094 ) ) ;
#33103=CARTESIAN_POINT ( 'NONE',  ( 10.00000000000000000, 5.773502691896255534, -42.75000000409675494 ) ) ;
#33104=CARTESIAN_POINT ( 'NONE',  ( 9.999999999999998224, 0.000000000000000000, -200.0000000000000000 ) ) ;
#33107=( BOUNDED_CURVE ( )  B_SPLINE_CURVE ( 2, ( #40451, #7895, #20397, #27959, #11320, #10895, #13909 ),
 .UNSPECIFIED., .F., .F. ) 
 B_SPLINE_CURVE_WITH_KNOTS ( ( 3, 2, 2, 3 ),
 ( 0.5559701492537315604, 0.5572139303482589456, 0.5584577114427863309, 0.5597014925373136052 ),
 .UNSPECIFIED. ) 
 CURVE ( )  GEOMETRIC_REPRESENTATION_ITEM ( )  RATIONAL_B_SPLINE_CURVE ( ( 0.9999999999999761302, 0.8660254037844625774, 1.000000000000000000, 0.8660254037844387076, 1.000000000000000000, 0.8660254037844148378, 1.000000000000023981 ) ) 
 REPRESENTATION_ITEM ( '' )  );
#33109=CARTESIAN_POINT ( 'NONE',  ( 10.81189881249999551, -6.242252689847874514, -163.6562500020484094 ) ) ;
#33110=CARTESIAN_POINT ( 'NONE',  ( 5.405949406249999534, 9.363379034771803333, -137.5937500020483810 ) ) ;
#33111=DIRECTION ( 'NONE',  ( -0.000000000000000000, -0.000000000000000000, 1.000000000000000000 ) ) ;
#33112=DIRECTION ( 'NONE',  ( -0.000000000000000000, -0.000000000000000000, 1.000000000000000000 ) ) ;
#33116=CARTESIAN_POINT ( 'NONE',  ( -5.405949406249996869, 9.363379034771805109, -68.53125000204838102 ) ) ;
#33117=ORIENTED_EDGE ( 'NONE', *, *, #31227, .F. ) ;
#33119=CARTESIAN_POINT ( 'NONE',  ( -10.81189881249999907, -6.242252689847864744, -117.4687500020483952 ) ) ;
#33122=CARTESIAN_POINT ( 'NONE',  ( -5.405949406249996869, 9.363379034771805109, -23.34375000204835970 ) ) ;
#33123=CARTESIAN_POINT ( 'NONE',  ( 5.405949406249999534, 9.363379034771803333, 0.2187499979516283055 ) ) ;
#33124=VECTOR ( 'NONE', #42644, 1000.000000000000000 ) ;
#33125=CARTESIAN_POINT ( 'NONE',  ( -10.81189881249999729, 6.242252689847871849, -45.71875000204837391 ) ) ;
#33126=CARTESIAN_POINT ( 'NONE',  ( 4.999999999999992006, -8.660254037844389075, -71.62500000409677625 ) ) ;
#33128=CARTESIAN_POINT ( 'NONE',  ( -10.81189881249999729, -6.242252689847864744, -181.9687500020484094 ) ) ;
#33129=CARTESIAN_POINT ( 'NONE',  ( -10.81189881249999907, -6.242252689847864744, -169.9687500020484094 ) ) ;
#33132=CARTESIAN_POINT ( 'NONE',  ( 9.999999999999998224, 0.000000000000000000, -200.0000000000000000 ) ) ;
#33133=CARTESIAN_POINT ( 'NONE',  ( 5.000000000000000000, 8.660254037844385522, -188.1250000040967905 ) ) ;
#33135=CARTESIAN_POINT ( 'NONE',  ( -10.81189881249999907, -6.242252689847864744, -94.96875000204838102 ) ) ;
#33137=CARTESIAN_POINT ( 'NONE',  ( -10.81189881249999907, -6.242252689847864744, -66.65625000204839523 ) ) ;
#33138=CARTESIAN_POINT ( 'NONE',  ( -9.999999999999742428, -5.773502691896402084, -160.1250000000000284 ) ) ;
#33140=CARTESIAN_POINT ( 'NONE',  ( 7.644554776091147741E-16, 12.48450537969573659, -125.6562500020483810 ) ) ;
#33141=CARTESIAN_POINT ( 'NONE',  ( -5.405949406250003975, -9.363379034771801557, -161.0312500020484094 ) ) ;
#33143=CARTESIAN_POINT ( 'NONE',  ( 10.00000000000000000, 5.773502691896255534, -134.2500000040967905 ) ) ;
#33148=CARTESIAN_POINT ( 'NONE',  ( 10.81189881249999729, 0.000000000000000000, -186.0312500020484094 ) ) ;
#33149=CARTESIAN_POINT ( 'NONE',  ( 9.999999999999998224, 0.000000000000000000, -131.3750000040967905 ) ) ;
#33152=CARTESIAN_POINT ( 'NONE',  ( 4.999999999999992006, -8.660254037844389075, -60.74999999999997158 ) ) ;
#33154=CARTESIAN_POINT ( 'NONE',  ( 10.00000000000000000, 5.773502691896255534, -65.25000000409677625 ) ) ;
#33155=CARTESIAN_POINT ( 'NONE',  ( -10.00000000000102496, 5.773502691895664007, -21.25000000409673362 ) ) ;
#33156=DIRECTION ( 'NONE',  ( -0.000000000000000000, -0.000000000000000000, 1.000000000000000000 ) ) ;
#33158=CARTESIAN_POINT ( 'NONE',  ( -5.405949406249996869, 9.363379034771805109, -56.53125000204836681 ) ) ;
#33161=LINE ( 'NONE', #152, #78 ) ;
#33162=CARTESIAN_POINT ( 'NONE',  ( 5.405949406249999534, 9.363379034771803333, -185.7812500020484094 ) ) ;
#33164=ADVANCED_FACE ( 'NONE', ( #11243 ), #27451, .T. ) ;
#33166=DIRECTION ( 'NONE',  ( 0.000000000000000000, 0.000000000000000000, -1.000000000000000000 ) ) ;
#33170=CARTESIAN_POINT ( 'NONE',  ( -10.00000000000000000, -5.773502691896251982, -169.1249999999999716 ) ) ;
#33171=CARTESIAN_POINT ( 'NONE',  ( -2.121150477449813534E-15, -11.54700538379251284, -137.7500000040967905 ) ) ;
#33172=CARTESIAN_POINT ( 'NONE',  ( 10.81189881249999551, -6.242252689847874514, -96.15625000204838102 ) ) ;
#33173=ORIENTED_EDGE ( 'NONE', *, *, #9863, .T. ) ;
#33174=DIRECTION ( 'NONE',  ( -0.000000000000000000, -0.000000000000000000, -1.000000000000000000 ) ) ;
#33177=( BOUNDED_CURVE ( )  B_SPLINE_CURVE ( 2, ( #39633, #12874, #20214, #36829, #6844, #26697, #36410 ),
 .UNSPECIFIED., .F., .F. ) 
 B_SPLINE_CURVE_WITH_KNOTS ( ( 3, 2, 2, 3 ),
 ( 0.4328358208955225273, 0.4340796019900499125, 0.4353233830845772978, 0.4365671641791046276 ),
 .UNSPECIFIED. ) 
 CURVE ( )  GEOMETRIC_REPRESENTATION_ITEM ( )  RATIONAL_B_SPLINE_CURVE ( ( 0.9999999999999820144, 0.8660254037844566932, 1.000000000000000000, 0.8660254037844387076, 1.000000000000000000, 0.8660254037844207220, 1.000000000000017986 ) ) 
 REPRESENTATION_ITEM ( '' )  );
#33179=CARTESIAN_POINT ( 'NONE',  ( 5.405949406249992428, -9.363379034771808662, -36.09375000204836681 ) ) ;
#33180=CARTESIAN_POINT ( 'NONE',  ( -10.81189881249999729, 6.242252689847871849, -18.90625000204837391 ) ) ;
#33182=CARTESIAN_POINT ( 'NONE',  ( 5.405949406249992428, -9.363379034771808662, -69.09375000204836681 ) ) ;
#33184=CARTESIAN_POINT ( 'NONE',  ( -2.293366432827344421E-15, -12.48450537969573659, -189.2187500020484094 ) ) ;
#33185=CARTESIAN_POINT ( 'NONE',  ( -10.81189881249999907, -6.242252689847864744, -153.4687500020484094 ) ) ;
#33186=AXIS2_PLACEMENT_3D ( 'NONE', #32679, #13001, #9784 ) ;
#33187=CARTESIAN_POINT ( 'NONE',  ( 0.000000000000000000, 0.000000000000000000, -200.0000000000000000 ) ) ;
#33190=CARTESIAN_POINT ( 'NONE',  ( 5.000000000000000000, 8.660254037844385522, -5.125000004096769146 ) ) ;
#33193=CARTESIAN_POINT ( 'NONE',  ( -5.405949406250003975, -9.363379034771801557, -124.8437500020483810 ) ) ;
#33194=CARTESIAN_POINT ( 'NONE',  ( -4.999999999999996447, 8.660254037844387298, -14.99999999999995737 ) ) ;
#33195=CARTESIAN_POINT ( 'NONE',  ( -5.405949406250003975, -9.363379034771801557, -92.03125000204838102 ) ) ;
#33196=CARTESIAN_POINT ( 'NONE',  ( -2.293366432827344421E-15, -12.48450537969573659, -109.7187500020483668 ) ) ;
#33199=CARTESIAN_POINT ( 'NONE',  ( -2.121150477449813534E-15, -11.54700538379251284, -160.2500000040967620 ) ) ;
#33203=VECTOR ( 'NONE', #22714, 1000.000000000000000 ) ;
#33208=CARTESIAN_POINT ( 'NONE',  ( 4.999999999999992006, -8.660254037844389075, -83.24999999999997158 ) ) ;
#33210=CARTESIAN_POINT ( 'NONE',  ( -9.999999999999998224, 1.224646799147353059E-15, -91.62500000409677625 ) ) ;
#33211=CARTESIAN_POINT ( 'NONE',  ( 0.000000000000000000, 0.000000000000000000, -200.0000000000000000 ) ) ;
#33213=CARTESIAN_POINT ( 'NONE',  ( 5.405949406249992428, -9.363379034771808662, -82.78125000204838102 ) ) ;
#33218=ORIENTED_EDGE ( 'NONE', *, *, #17476, .T. ) ;
#33219=CARTESIAN_POINT ( 'NONE',  ( -9.999999999999998224, 1.224646799147353059E-15, -8.749999999999952038 ) ) ;
#33220=CARTESIAN_POINT ( 'NONE',  ( -4.999999999999996447, 8.660254037844387298, -145.5000000000000000 ) ) ;
#33221=CARTESIAN_POINT ( 'NONE',  ( -9.999999999999479527, -5.773502691896549521, -32.62499999999994316 ) ) ;
#33223=AXIS2_PLACEMENT_3D ( 'NONE', #23448, #13065, #16729 ) ;
#33224=( BOUNDED_CURVE ( )  B_SPLINE_CURVE ( 2, ( #329, #10226, #544, #36145, #17119, #6576, #33554 ),
 .UNSPECIFIED., .F., .F. ) 
 B_SPLINE_CURVE_WITH_KNOTS ( ( 3, 2, 2, 3 ),
 ( 0.4664179104477613191, 0.4676616915422886489, 0.4689054726368160342, 0.4701492537313434195 ),
 .UNSPECIFIED. ) 
 CURVE ( )  GEOMETRIC_REPRESENTATION_ITEM ( )  RATIONAL_B_SPLINE_CURVE ( ( 0.9999999999999880096, 0.8660254037844506980, 1.000000000000000000, 0.8660254037844387076, 1.000000000000000000, 0.8660254037844267172, 1.000000000000011990 ) ) 
 REPRESENTATION_ITEM ( '' )  );
#33226=CARTESIAN_POINT ( 'NONE',  ( -10.00000000000000000, -5.773502691896251982, -193.1250000000000284 ) ) ;
#33227=LINE ( 'NONE', #36447, #16481 ) ;
#33228=CARTESIAN_POINT ( 'NONE',  ( -5.405949406249996869, 9.363379034771805109, -121.0312500020483952 ) ) ;
#33229=VERTEX_POINT ( 'NONE', #4568 ) ;
#33230=DIRECTION ( 'NONE',  ( 1.000000000000000000, 0.000000000000000000, 0.000000000000000000 ) ) ;
#33233=CARTESIAN_POINT ( 'NONE',  ( -10.81189881249999729, 6.242252689847871849, -47.40625000204835970 ) ) ;
#33236=CARTESIAN_POINT ( 'NONE',  ( -5.405949406249996869, 9.363379034771805109, -95.34375000204838102 ) ) ;
#33237=CARTESIAN_POINT ( 'NONE',  ( 10.81189881249999729, 0.000000000000000000, -123.0312500020483952 ) ) ;
#33238=EDGE_LOOP ( 'NONE', ( #26373, #11276, #31953, #28729 ) ) ;
#33243=CARTESIAN_POINT ( 'NONE',  ( -10.81189881249999729, 1.324075727343319199E-15, -134.0937500020483810 ) ) ;
#33247=CARTESIAN_POINT ( 'NONE',  ( 10.00000000000000000, 5.773502691896255534, -185.2500000040967905 ) ) ;
#33249=AXIS2_PLACEMENT_3D ( 'NONE', #33814, #27759, #21274 ) ;
#33250=CARTESIAN_POINT ( 'NONE',  ( -10.81189881249999729, 1.324075727343319199E-15, -185.2812500020484094 ) ) ;
#33252=FACE_OUTER_BOUND ( 'NONE', #24207, .T. ) ;
#33255=CARTESIAN_POINT ( 'NONE',  ( -2.293366432827344421E-15, -12.48450537969573659, -58.71875000204836681 ) ) ;
#33256=CARTESIAN_POINT ( 'NONE',  ( -10.81189881249999729, 6.242252689847871849, -45.71875000204837391 ) ) ;
#33258=CARTESIAN_POINT ( 'NONE',  ( -5.405949406250003975, -9.363379034771801557, -15.53125000204835793 ) ) ;
#33260=CARTESIAN_POINT ( 'NONE',  ( 4.999999999999992006, -8.660254037844389075, -124.1250000040967905 ) ) ;
#33262=CARTESIAN_POINT ( 'NONE',  ( 9.999999999999996447, -5.773502691896262640, -104.1249999999999858 ) ) ;
#33264=CARTESIAN_POINT ( 'NONE',  ( -2.121150477449813534E-15, -11.54700538379251284, -114.8749999999999716 ) ) ;
#33267=CARTESIAN_POINT ( 'NONE',  ( -5.405949406250003975, -9.363379034771801557, -105.5312500020483810 ) ) ;
#33268=VERTEX_POINT ( 'NONE', #40802 ) ;
#33271=CARTESIAN_POINT ( 'NONE',  ( -2.121150477449813534E-15, -11.54700538379251284, -136.2500000040967905 ) ) ;
#33274=CARTESIAN_POINT ( 'NONE',  ( -9.999999999999998224, 1.224646799147353059E-15, -31.24999999999997158 ) ) ;
#33276=CARTESIAN_POINT ( 'NONE',  ( -5.000000000000003553, -8.660254037844383745, -16.37500000409675138 ) ) ;
#33277=CARTESIAN_POINT ( 'NONE',  ( -10.81189881249999729, -6.242252689847864744, -47.15625000204836681 ) ) ;
#33278=DIRECTION ( 'NONE',  ( -0.000000000000000000, -0.000000000000000000, 1.000000000000000000 ) ) ;
#33280=LINE ( 'NONE', #31267, #40350 ) ;
#33281=CARTESIAN_POINT ( 'NONE',  ( 5.405949406249992428, -9.363379034771808662, -141.2812500020483810 ) ) ;
#33282=CARTESIAN_POINT ( 'NONE',  ( 0.000000000000000000, 0.000000000000000000, -200.0000000000000000 ) ) ;
#33283=ORIENTED_EDGE ( 'NONE', *, *, #32262, .F. ) ;
#33284=ORIENTED_EDGE ( 'NONE', *, *, #7477, .F. ) ;
#33288=EDGE_CURVE ( 'NONE', #18350, #15045, #10623, .T. ) ;
#33289=CARTESIAN_POINT ( 'NONE',  ( -2.121150477449813534E-15, -11.54700538379251284, -121.2500000040967905 ) ) ;
#33290=CARTESIAN_POINT ( 'NONE',  ( -5.405949406249996869, 9.363379034771805109, -174.8437500020484094 ) ) ;
#33291=CARTESIAN_POINT ( 'NONE',  ( 5.405949406249999534, 9.363379034771803333, -20.59375000204835615 ) ) ;
#33293=DIRECTION ( 'NONE',  ( -0.000000000000000000, -0.000000000000000000, 1.000000000000000000 ) ) ;
#33294=CARTESIAN_POINT ( 'NONE',  ( -2.293366432827344421E-15, -12.48450537969573659, -156.2187500020483810 ) ) ;
#33295=CARTESIAN_POINT ( 'NONE',  ( 5.405949406249992428, -9.363379034771808662, -138.0937500020483810 ) ) ;
#33299=CARTESIAN_POINT ( 'NONE',  ( -5.405949406249996869, 9.363379034771805109, -14.34375000204834905 ) ) ;
#33302=CARTESIAN_POINT ( 'NONE',  ( 9.999999999999998224, 0.000000000000000000, -120.5000000000000000 ) ) ;
#33304=CARTESIAN_POINT ( 'NONE',  ( -9.999999999999998224, 1.224646799147353059E-15, -67.24999999999997158 ) ) ;
#33305=CARTESIAN_POINT ( 'NONE',  ( -10.81189881249999729, 1.324075727343319199E-15, -83.09375000204836681 ) ) ;
#33306=CARTESIAN_POINT ( 'NONE',  ( -10.81189881249999729, 6.242252689847871849, -69.71875000204838102 ) ) ;
#33307=CARTESIAN_POINT ( 'NONE',  ( 10.81189881249999907, 6.242252689847868297, -43.40625000204837391 ) ) ;
#33309=LINE ( 'NONE', #27460, #17813 ) ;
#33311=CARTESIAN_POINT ( 'NONE',  ( 10.00000000000000000, 5.773502691896255534, -126.3749999999999858 ) ) ;
#33312=CARTESIAN_POINT ( 'NONE',  ( -10.81189881249999729, 1.324075727343319199E-15, -135.7812500020483810 ) ) ;
#33313=DIRECTION ( 'NONE',  ( 1.000000000000000000, 0.000000000000000000, 0.000000000000000000 ) ) ;
#33319=CARTESIAN_POINT ( 'NONE',  ( 5.405949406249992428, -9.363379034771808662, -168.2812500020484094 ) ) ;
#33320=CARTESIAN_POINT ( 'NONE',  ( 9.999999999999996447, -5.773502691896262640, -40.00000000409676204 ) ) ;
#33321=CARTESIAN_POINT ( 'NONE',  ( 0.000000000000000000, 0.000000000000000000, -200.0000000000000000 ) ) ;
#33323=CARTESIAN_POINT ( 'NONE',  ( -5.000000000000003553, -8.660254037844383745, -63.99999999999997158 ) ) ;
#33324=CARTESIAN_POINT ( 'NONE',  ( -5.405949406250003975, -9.363379034771801557, -159.5312500020484094 ) ) ;
#33325=CARTESIAN_POINT ( 'NONE',  ( 10.81189881249999907, 6.242252689847868297, -136.2187500020483810 ) ) ;
#33326=CARTESIAN_POINT ( 'NONE',  ( -5.000000000000003553, -8.660254037844383745, -50.87500000409675494 ) ) ;
#33327=CARTESIAN_POINT ( 'NONE',  ( -9.999999999999998224, 1.224646799147353059E-15, -79.62500000409677625 ) ) ;
#33329=DIRECTION ( 'NONE',  ( -0.5000000000000003331, 0.8660254037844383745, 0.000000000000000000 ) ) ;
#33330=CARTESIAN_POINT ( 'NONE',  ( -5.405949406250003975, -9.363379034771801557, -66.53125000204838102 ) ) ;
#33333=EDGE_CURVE ( 'NONE', #12734, #982, #20318, .T. ) ;
#33334=CARTESIAN_POINT ( 'NONE',  ( 10.81189881249999551, -6.242252689847874514, -119.9687500020483952 ) ) ;
#33336=EDGE_CURVE ( 'NONE', #31054, #27322, #15038, .T. ) ;
#33337=( BOUNDED_CURVE ( )  B_SPLINE_CURVE ( 2, ( #1858, #34017, #21045, #31421, #38096, #7680, #4651 ),
 .UNSPECIFIED., .F., .F. ) 
 B_SPLINE_CURVE_WITH_KNOTS ( ( 3, 2, 2, 3 ),
 ( 0.1753731343283582433, 0.1766169154228856009, 0.1778606965174129861, 0.1791044776119403437 ),
 .UNSPECIFIED. ) 
 CURVE ( )  GEOMETRIC_REPRESENTATION_ITEM ( )  RATIONAL_B_SPLINE_CURVE ( ( 0.9999999999999970024, 0.8660254037844417052, 1.000000000000000000, 0.8660254037844387076, 1.000000000000000000, 0.8660254037844327124, 1.000000000000005995 ) ) 
 REPRESENTATION_ITEM ( '' )  );
#33339=CARTESIAN_POINT ( 'NONE',  ( -2.293366432827344421E-15, -12.48450537969573659, -18.21875000204837036 ) ) ;
#33341=CARTESIAN_POINT ( 'NONE',  ( -2.293366432827344421E-15, -12.48450537969573659, -195.2187500020484094 ) ) ;
#33342=CARTESIAN_POINT ( 'NONE',  ( -2.293366432827344421E-15, -12.48450537969573659, -51.21875000204836681 ) ) ;
#33344=DIRECTION ( 'NONE',  ( -0.000000000000000000, -0.000000000000000000, 1.000000000000000000 ) ) ;
#33345=CARTESIAN_POINT ( 'NONE',  ( 5.405949406249999534, 9.363379034771803333, -176.5937500020484094 ) ) ;
#33346=CARTESIAN_POINT ( 'NONE',  ( -10.81189881249999907, -6.242252689847864744, -172.9687500020484094 ) ) ;
#33353=CARTESIAN_POINT ( 'NONE',  ( -10.81189881249999907, -6.242252689847864744, -99.46875000204838102 ) ) ;
#33354=CARTESIAN_POINT ( 'NONE',  ( 10.00000000000051159, -5.773502691895965988, -101.1249999999999858 ) ) ;
#33355=CARTESIAN_POINT ( 'NONE',  ( 10.81189881249999551, -6.242252689847874514, -64.65625000204839523 ) ) ;
#33356=FACE_OUTER_BOUND ( 'NONE', #25002, .T. ) ;
#33358=CARTESIAN_POINT ( 'NONE',  ( 10.81189881249999551, -6.242252689847874514, -123.1562500020483952 ) ) ;
#33359=CARTESIAN_POINT ( 'NONE',  ( -10.81189881249999729, -6.242252689847864744, -159.6562500020484094 ) ) ;
#33361=CARTESIAN_POINT ( 'NONE',  ( 4.999999999999992006, -8.660254037844389075, -139.1250000040967905 ) ) ;
#33366=EDGE_CURVE ( 'NONE', #21484, #36111, #7618, .T. ) ;
#33367=CARTESIAN_POINT ( 'NONE',  ( 5.405949406249999534, 9.363379034771803333, -187.2812500020484094 ) ) ;
#33368=CARTESIAN_POINT ( 'NONE',  ( 0.000000000000000000, -5.321294541346989426, -220.0000000000000000 ) ) ;
#33370=VERTEX_POINT ( 'NONE', #37742 ) ;
#33371=CARTESIAN_POINT ( 'NONE',  ( -10.00000000000000000, -5.773502691896251982, -59.62500000000000000 ) ) ;
#33373=CARTESIAN_POINT ( 'NONE',  ( -9.999999999999998224, 5.773502691896259087, -64.75000000409677625 ) ) ;
#33375=DIRECTION ( 'NONE',  ( -1.000000000000000000, 0.000000000000000000, -0.000000000000000000 ) ) ;
#33377=CARTESIAN_POINT ( 'NONE',  ( 5.405949406249999534, 9.363379034771803333, -58.28125000204836681 ) ) ;
#33380=FACE_OUTER_BOUND ( 'NONE', #7625, .T. ) ;
#33381=CARTESIAN_POINT ( 'NONE',  ( -10.81189881249999907, -6.242252689847864744, -185.1562500020484094 ) ) ;
#33383=CARTESIAN_POINT ( 'NONE',  ( 9.999999999998969713, 5.773502691896851502, -40.87499999999994316 ) ) ;
#33384=CARTESIAN_POINT ( 'NONE',  ( 9.999999999999998224, 0.000000000000000000, -117.5000000000000000 ) ) ;
#33385=CYLINDRICAL_SURFACE ( 'NONE', #33223, 9.999999999999998224 ) ;
#33386=DIRECTION ( 'NONE',  ( 0.000000000000000000, 1.000000000000000000, 0.000000000000000000 ) ) ;
#33387=CARTESIAN_POINT ( 'NONE',  ( -9.999999999999998224, 1.224646799147353059E-15, -62.74999999999997158 ) ) ;
#33388=CARTESIAN_POINT ( 'NONE',  ( 5.405949406249999534, 9.363379034771803333, -91.28125000204838102 ) ) ;
#33392=EDGE_LOOP ( 'NONE', ( #40927, #19984, #31432, #34183 ) ) ;
#33394=CARTESIAN_POINT ( 'NONE',  ( 10.81189881249999551, -6.242252689847874514, -32.96875000204834549 ) ) ;
#33395=CARTESIAN_POINT ( 'NONE',  ( -5.405949406249996869, 9.363379034771805109, -23.53125000204836681 ) ) ;
#33396=CARTESIAN_POINT ( 'NONE',  ( -10.81189881249999907, -6.242252689847864744, -69.46875000204838102 ) ) ;
#33397=CARTESIAN_POINT ( 'NONE',  ( -9.999999999998456346, -5.773502691897145489, -18.00000000409673007 ) ) ;
#33399=CARTESIAN_POINT ( 'NONE',  ( 7.644554776091147741E-16, 12.48450537969573659, -194.4687500020484094 ) ) ;
#33400=CARTESIAN_POINT ( 'NONE',  ( -2.293366432827344421E-15, -12.48450537969573659, -148.7187500020484094 ) ) ;
#33401=CARTESIAN_POINT ( 'NONE',  ( 9.999999999999998224, 0.000000000000000000, -72.87500000409677625 ) ) ;
#33404=CARTESIAN_POINT ( 'NONE',  ( 9.999999999999998224, 0.000000000000000000, -0.8750000040967653714 ) ) ;
#33405=CARTESIAN_POINT ( 'NONE',  ( 10.00000000000102318, -5.773502691895667560, -103.0000000040967194 ) ) ;
#33406=EDGE_CURVE ( 'NONE', #3605, #26657, #18092, .T. ) ;
#33407=CARTESIAN_POINT ( 'NONE',  ( 10.81189881249999729, 0.000000000000000000, -119.8437500020483810 ) ) ;
#33409=CARTESIAN_POINT ( 'NONE',  ( 10.81189881249999551, -6.242252689847874514, -90.15625000204836681 ) ) ;
#33410=CARTESIAN_POINT ( 'NONE',  ( 7.644554776091147741E-16, 12.48450537969573659, -110.4687500020483668 ) ) ;
#33413=CARTESIAN_POINT ( 'NONE',  ( -5.000000000000003553, -8.660254037844383745, -161.8750000040967905 ) ) ;
#33420=CARTESIAN_POINT ( 'NONE',  ( -5.000000000000003553, -8.660254037844383745, -83.49999999999997158 ) ) ;
#33422=CARTESIAN_POINT ( 'NONE',  ( 5.000000000000000000, 8.660254037844385522, -90.62500000409677625 ) ) ;
#33423=DIRECTION ( 'NONE',  ( -0.8660254037844388186, 0.4999999999999997224, 0.000000000000000000 ) ) ;
#33425=CARTESIAN_POINT ( 'NONE',  ( 10.81189881249999729, 0.000000000000000000, -81.03125000204839523 ) ) ;
#33426=ORIENTED_EDGE ( 'NONE', *, *, #15257, .F. ) ;
#33428=CARTESIAN_POINT ( 'NONE',  ( 9.999999999999998224, 0.000000000000000000, -200.0000000000000000 ) ) ;
#33430=VERTEX_POINT ( 'NONE', #1716 ) ;
#33431=CARTESIAN_POINT ( 'NONE',  ( 10.00000000000000000, 5.773502691896255534, -9.374999999999980460 ) ) ;
#33433=CARTESIAN_POINT ( 'NONE',  ( 7.070501591499377789E-16, 11.54700538379251284, -144.1250000000000000 ) ) ;
#33434=DIRECTION ( 'NONE',  ( -0.000000000000000000, -0.000000000000000000, 1.000000000000000000 ) ) ;
#33435=( BOUNDED_CURVE ( )  B_SPLINE_CURVE ( 2, ( #35668, #26789, #15992, #51, #29398, #6516, #36295 ),
 .UNSPECIFIED., .F., .F. ) 
 B_SPLINE_CURVE_WITH_KNOTS ( ( 3, 2, 2, 3 ),
 ( 0.3768656716417911334, 0.3781094527363185187, 0.3793532338308459040, 0.3805970149253732338 ),
 .UNSPECIFIED. ) 
 CURVE ( )  GEOMETRIC_REPRESENTATION_ITEM ( )  RATIONAL_B_SPLINE_CURVE ( ( 0.9999999999999880096, 0.8660254037844506980, 1.000000000000000000, 0.8660254037844387076, 1.000000000000000000, 0.8660254037844267172, 1.000000000000011990 ) ) 
 REPRESENTATION_ITEM ( '' )  );
#33437=CARTESIAN_POINT ( 'NONE',  ( 9.999999999999996447, -5.773502691896262640, -189.6250000000000000 ) ) ;
#33438=CARTESIAN_POINT ( 'NONE',  ( -9.999999999999998224, 1.224646799147353059E-15, -200.0000000000000000 ) ) ;
#33439=CARTESIAN_POINT ( 'NONE',  ( -2.293366432827344421E-15, -12.48450537969573659, -120.4062500020483952 ) ) ;
#33441=CARTESIAN_POINT ( 'NONE',  ( 9.999999999998456346, 5.773502691897149042, -23.25000000409674072 ) ) ;
#33443=EDGE_LOOP ( 'NONE', ( #18164, #18696, #27432, #17427 ) ) ;
#33444=CARTESIAN_POINT ( 'NONE',  ( -10.81189881249999729, 1.324075727343319199E-15, -47.28125000204838813 ) ) ;
#33446=CARTESIAN_POINT ( 'NONE',  ( -2.293366432827344421E-15, -12.48450537969573659, -93.21875000204838102 ) ) ;
#33447=CARTESIAN_POINT ( 'NONE',  ( -5.405949406250003975, -9.363379034771801557, -125.0312500020483952 ) ) ;
#33448=EDGE_LOOP ( 'NONE', ( #32281, #12205, #693, #36133 ) ) ;
#33449=CARTESIAN_POINT ( 'NONE',  ( -5.000000000000003553, -8.660254037844383745, -83.49999999999997158 ) ) ;
#33450=VECTOR ( 'NONE', #22991, 1000.000000000000000 ) ;
#33451=CARTESIAN_POINT ( 'NONE',  ( -5.405949406250003975, -9.363379034771801557, -196.8437500020484094 ) ) ;
#33454=CARTESIAN_POINT ( 'NONE',  ( 10.81189881249999729, 6.242252689847867408, -130.2187500020483810 ) ) ;
#33456=DIRECTION ( 'NONE',  ( -0.000000000000000000, -0.000000000000000000, 1.000000000000000000 ) ) ;
#33458=CARTESIAN_POINT ( 'NONE',  ( -9.999999999999998224, 5.773502691896259087, -187.7500000040967905 ) ) ;
#33460=CARTESIAN_POINT ( 'NONE',  ( -2.293366432827344421E-15, -12.48450537969573659, -177.4062500020484379 ) ) ;
#33461=VECTOR ( 'NONE', #34105, 1000.000000000000000 ) ;
#33462=CARTESIAN_POINT ( 'NONE',  ( -5.000000000000003553, -8.660254037844383745, -107.4999999999999858 ) ) ;
#33465=CARTESIAN_POINT ( 'NONE',  ( 7.644554776091147741E-16, 12.48450537969573659, -62.46875000204839523 ) ) ;
#33466=CARTESIAN_POINT ( 'NONE',  ( 5.405949406249999534, 9.363379034771803333, -41.59375000204837391 ) ) ;
#33468=CARTESIAN_POINT ( 'NONE',  ( -2.293366432827344421E-15, -12.48450537969573659, -21.40625000204837036 ) ) ;
#33470=CARTESIAN_POINT ( 'NONE',  ( 0.000000000000000000, 0.000000000000000000, -200.0000000000000000 ) ) ;
#33472=CARTESIAN_POINT ( 'NONE',  ( 10.00000000000000000, 5.773502691896255534, -106.8749999999999716 ) ) ;
#33476=CARTESIAN_POINT ( 'NONE',  ( -5.405949406250003975, -9.363379034771801557, -108.5312500020483810 ) ) ;
#33477=ADVANCED_FACE ( 'NONE', ( #34736 ), #5158, .T. ) ;
#33478=ORIENTED_EDGE ( 'NONE', *, *, #15107, .T. ) ;
#33482=CARTESIAN_POINT ( 'NONE',  ( -9.999999999999918288, -5.773502691896298167, -195.0000000040968189 ) ) ;
#33484=ORIENTED_EDGE ( 'NONE', *, *, #13750, .T. ) ;
#33485=CARTESIAN_POINT ( 'NONE',  ( 10.00000000000000000, 5.773502691896255534, -30.37499999999995381 ) ) ;
#33486=CARTESIAN_POINT ( 'NONE',  ( 10.81189881249999551, -6.242252689847874514, -39.15625000204835970 ) ) ;
#33490=CARTESIAN_POINT ( 'NONE',  ( 5.405949406249999534, 9.363379034771803333, -139.2812500020483810 ) ) ;
#33491=AXIS2_PLACEMENT_3D ( 'NONE', #2438, #22289, #19038 ) ;
#33492=CARTESIAN_POINT ( 'NONE',  ( 5.000000000000000000, 8.660254037844385522, -174.6250000040968189 ) ) ;
#33496=CARTESIAN_POINT ( 'NONE',  ( -9.999999999999998224, 1.224646799147353059E-15, -107.7499999999999858 ) ) ;
#33497=CARTESIAN_POINT ( 'NONE',  ( 10.00000000000025402, -5.773502691896113426, -129.6250000000000000 ) ) ;
#33498=CARTESIAN_POINT ( 'NONE',  ( 10.81189881249999729, 0.000000000000000000, -164.8437500020484094 ) ) ;
#33499=EDGE_CURVE ( 'NONE', #15077, #11765, #13890, .T. ) ;
#33501=CARTESIAN_POINT ( 'NONE',  ( 10.81189881249999729, 0.000000000000000000, -20.84375000204835615 ) ) ;
#33503=CARTESIAN_POINT ( 'NONE',  ( 10.81189881249999551, -6.242252689847874514, -155.9687500020484094 ) ) ;
#33504=CARTESIAN_POINT ( 'NONE',  ( 10.81189881249999729, 0.000000000000000000, -137.8437500020484094 ) ) ;
#33505=CARTESIAN_POINT ( 'NONE',  ( -9.999999999999998224, 1.224646799147353059E-15, -9.125000004096744277 ) ) ;
#33510=CARTESIAN_POINT ( 'NONE',  ( 10.81189881249999729, 0.000000000000000000, -8.843750002048345493 ) ) ;
#33512=CARTESIAN_POINT ( 'NONE',  ( 7.070501591499376803E-16, 11.54700538379251284, -63.50000000409679046 ) ) ;
#33516=CARTESIAN_POINT ( 'NONE',  ( -5.405949406250003975, -9.363379034771801557, -85.84375000204836681 ) ) ;
#33517=CARTESIAN_POINT ( 'NONE',  ( 5.405949406249999534, 9.363379034771803333, -68.59375000204836681 ) ) ;
#33518=CARTESIAN_POINT ( 'NONE',  ( -5.405949406249996869, 9.363379034771805109, -41.53125000204838102 ) ) ;
#33520=DIRECTION ( 'NONE',  ( -0.000000000000000000, -0.000000000000000000, 1.000000000000000000 ) ) ;
#33522=CARTESIAN_POINT ( 'NONE',  ( -10.00000000000000000, -5.773502691896251982, -125.6249999999999858 ) ) ;
#33523=CARTESIAN_POINT ( 'NONE',  ( 10.81189881249999729, 0.000000000000000000, -141.0312500020483810 ) ) ;
#33524=CARTESIAN_POINT ( 'NONE',  ( 4.999999999999992006, -8.660254037844389075, -187.1250000040967905 ) ) ;
#33526=CARTESIAN_POINT ( 'NONE',  ( -2.293366432827344421E-15, -12.48450537969573659, -18.40625000204837036 ) ) ;
#33530=LINE ( 'NONE', #9985, #40806 ) ;
#33531=CARTESIAN_POINT ( 'NONE',  ( -9.999999999999998224, 1.224646799147353059E-15, -39.12500000409676915 ) ) ;
#33532=EDGE_CURVE ( 'NONE', #258, #5415, #12273, .T. ) ;
#33533=CARTESIAN_POINT ( 'NONE',  ( 5.000000000000000000, 8.660254037844385522, -155.1250000040967905 ) ) ;
#33535=CARTESIAN_POINT ( 'NONE',  ( -9.999999999999998224, 1.224646799147353059E-15, -100.6250000040967905 ) ) ;
#33536=CARTESIAN_POINT ( 'NONE',  ( -2.293366432827344421E-15, -12.48450537969573659, -150.4062500020483810 ) ) ;
#33537=CARTESIAN_POINT ( 'NONE',  ( 10.81189881249999907, 6.242252689847868297, -134.7187500020484094 ) ) ;
#33538=ORIENTED_EDGE ( 'NONE', *, *, #37259, .T. ) ;
#33539=CARTESIAN_POINT ( 'NONE',  ( 5.000000000000000000, 8.660254037844385522, -189.6250000040967905 ) ) ;
#33540=CARTESIAN_POINT ( 'NONE',  ( 5.405949406249999534, 9.363379034771803333, -65.78125000204838102 ) ) ;
#33541=VERTEX_POINT ( 'NONE', #12830 ) ;
#33543=CARTESIAN_POINT ( 'NONE',  ( 10.81189881249999729, 0.000000000000000000, -119.8437500020483810 ) ) ;
#33545=CARTESIAN_POINT ( 'NONE',  ( 10.81189881249999551, -6.242252689847874514, -19.46875000204837391 ) ) ;
#33546=CARTESIAN_POINT ( 'NONE',  ( -10.81189881249999729, 6.242252689847871849, -186.7187500020483810 ) ) ;
#33547=CARTESIAN_POINT ( 'NONE',  ( 7.644554776091147741E-16, 12.48450537969573659, -48.96875000204835970 ) ) ;
#33548=CARTESIAN_POINT ( 'NONE',  ( 9.999999999999998224, 0.000000000000000000, -62.37500000409676204 ) ) ;
#33549=CARTESIAN_POINT ( 'NONE',  ( 9.999999999999998224, 0.000000000000000000, -105.8750000040967763 ) ) ;
#33550=CARTESIAN_POINT ( 'NONE',  ( 10.81189881249999729, 0.000000000000000000, -182.8437500020483810 ) ) ;
#33551=CARTESIAN_POINT ( 'NONE',  ( 7.644554776091147741E-16, 12.48450537969573659, -162.9687500020483810 ) ) ;
#33554=CARTESIAN_POINT ( 'NONE',  ( 9.999999999999998224, 0.000000000000000000, -104.3750000040967763 ) ) ;
#33555=CARTESIAN_POINT ( 'NONE',  ( 7.071067811865472841, -7.071067811865472841, -200.0000000000000000 ) ) ;
#33557=CARTESIAN_POINT ( 'NONE',  ( -10.81189881249999729, 6.242252689847871849, -89.21875000204836681 ) ) ;
#33558=DIRECTION ( 'NONE',  ( 1.000000000000000000, 0.000000000000000000, 0.000000000000000000 ) ) ;
#33559=CARTESIAN_POINT ( 'NONE',  ( 10.81189881249999729, 0.000000000000000000, -67.53125000204838102 ) ) ;
#33560=CARTESIAN_POINT ( 'NONE',  ( 9.999999999999998224, 0.000000000000000000, -96.87500000409677625 ) ) ;
#33562=CARTESIAN_POINT ( 'NONE',  ( 7.644554776091147741E-16, 12.48450537969573659, -124.1562500020483952 ) ) ;
#33563=CARTESIAN_POINT ( 'NONE',  ( 10.81189881249999729, 6.242252689847867408, -166.4062500020483810 ) ) ;
#33565=CARTESIAN_POINT ( 'NONE',  ( 9.999999999999996447, -5.773502691896262640, -139.0000000040967905 ) ) ;
#33571=EDGE_CURVE ( 'NONE', #40862, #21406, #32959, .T. ) ;
#33572=CARTESIAN_POINT ( 'NONE',  ( -2.293366432827344421E-15, -12.48450537969573659, -190.9062500020483810 ) ) ;
#33574=ORIENTED_EDGE ( 'NONE', *, *, #9584, .T. ) ;
#33575=CARTESIAN_POINT ( 'NONE',  ( -9.999999999999998224, 5.773502691896259087, -52.37499999999997868 ) ) ;
#33577=CARTESIAN_POINT ( 'NONE',  ( 7.070501591499377789E-16, 11.54700538379251284, -66.50000000409676204 ) ) ;
#33578=EDGE_CURVE ( 'NONE', #19929, #32999, #19457, .T. ) ;
#33580=LINE ( 'NONE', #23438, #9808 ) ;
#33583=CARTESIAN_POINT ( 'NONE',  ( 10.81189881249999729, 0.000000000000000000, -58.53125000204836681 ) ) ;
#33586=CARTESIAN_POINT ( 'NONE',  ( -2.121150477449813534E-15, -11.54700538379251284, -35.37499999999996447 ) ) ;
#33587=CARTESIAN_POINT ( 'NONE',  ( 7.644554776091147741E-16, 12.48450537969573659, -185.6562500020484094 ) ) ;
#33589=CARTESIAN_POINT ( 'NONE',  ( -5.000000000000003553, -8.660254037844383745, -73.37500000409677625 ) ) ;
#33592=( BOUNDED_CURVE ( )  B_SPLINE_CURVE ( 2, ( #40458, #11330, #11538, #7683, #30999, #21049, #20618 ),
 .UNSPECIFIED., .F., .F. ) 
 B_SPLINE_CURVE_WITH_KNOTS ( ( 3, 2, 2, 3 ),
 ( 0.5298507462686568026, 0.5310945273631841879, 0.5323383084577115731, 0.5335820895522389584 ),
 .UNSPECIFIED. ) 
 CURVE ( )  GEOMETRIC_REPRESENTATION_ITEM ( )  RATIONAL_B_SPLINE_CURVE ( ( 0.9999999999999880096, 0.8660254037844506980, 1.000000000000000000, 0.8660254037844387076, 1.000000000000000000, 0.8660254037844267172, 1.000000000000011990 ) ) 
 REPRESENTATION_ITEM ( '' )  );
#33593=CARTESIAN_POINT ( 'NONE',  ( 4.999999999999992006, -8.660254037844389075, -137.6250000040967620 ) ) ;
#33594=CARTESIAN_POINT ( 'NONE',  ( 7.644554776091147741E-16, 12.48450537969573659, -88.15625000204838102 ) ) ;
#33595=ORIENTED_EDGE ( 'NONE', *, *, #15405, .F. ) ;
#33596=CARTESIAN_POINT ( 'NONE',  ( -9.999999999999612754, -5.773502691896474914, -181.5000000040967620 ) ) ;
#33597=EDGE_CURVE ( 'NONE', #468, #39036, #696, .T. ) ;
#33600=EDGE_LOOP ( 'NONE', ( #25432, #37818, #11057, #38302 ) ) ;
#33601=CARTESIAN_POINT ( 'NONE',  ( 10.81189881249999551, -6.242252689847874514, -28.46875000204837036 ) ) ;
#33602=CARTESIAN_POINT ( 'NONE',  ( 5.405949406249992428, -9.363379034771808662, -19.78125000204836326 ) ) ;
#33604=CARTESIAN_POINT ( 'NONE',  ( -10.81189881249999729, 1.324075727343319199E-15, -68.09375000204836681 ) ) ;
#33605=CARTESIAN_POINT ( 'NONE',  ( 4.999999999999992006, -8.660254037844389075, -83.62500000409677625 ) ) ;
#33608=CARTESIAN_POINT ( 'NONE',  ( -5.405949406250003975, -9.363379034771801557, -186.3437500020483810 ) ) ;
#33609=CARTESIAN_POINT ( 'NONE',  ( 10.81189881249999729, 0.000000000000000000, -148.3437500020483810 ) ) ;
#33610=CARTESIAN_POINT ( 'NONE',  ( -9.999999999999998224, 1.224646799147353059E-15, -92.74999999999998579 ) ) ;
#33611=CARTESIAN_POINT ( 'NONE',  ( 7.070501591499376803E-16, 11.54700538379251284, -132.5000000040967905 ) ) ;
#33612=CARTESIAN_POINT ( 'NONE',  ( 4.999999999999992006, -8.660254037844389075, -143.6250000040967905 ) ) ;
#33613=CARTESIAN_POINT ( 'NONE',  ( 4.999999999999992006, -8.660254037844389075, -1.125000004096765593 ) ) ;
#33614=DIRECTION ( 'NONE',  ( -0.000000000000000000, -0.000000000000000000, 1.000000000000000000 ) ) ;
#33615=CARTESIAN_POINT ( 'NONE',  ( 10.81189881249999729, 0.000000000000000000, -118.3437500020483810 ) ) ;
#33616=CARTESIAN_POINT ( 'NONE',  ( 10.81189881249999729, 0.000000000000000000, -90.03125000204838102 ) ) ;
#33617=CARTESIAN_POINT ( 'NONE',  ( 10.81189881249999551, -6.242252689847874514, -101.9687500020483810 ) ) ;
#33620=CARTESIAN_POINT ( 'NONE',  ( -9.999999999999998224, 1.224646799147353059E-15, -162.1250000040967905 ) ) ;
#33627=CARTESIAN_POINT ( 'NONE',  ( 10.00000000000000000, 5.773502691896255534, -70.87499999999998579 ) ) ;
#33629=CARTESIAN_POINT ( 'NONE',  ( -4.999999999999996447, 8.660254037844387298, -91.87500000409677625 ) ) ;
#33632=CARTESIAN_POINT ( 'NONE',  ( 5.405949406249992428, -9.363379034771808662, -84.28125000204838102 ) ) ;
#33635=CARTESIAN_POINT ( 'NONE',  ( 5.000000000000000000, 8.660254037844385522, -168.2500000000000000 ) ) ;
#33637=VERTEX_POINT ( 'NONE', #9607 ) ;
#33638=CARTESIAN_POINT ( 'NONE',  ( 10.00000000000000000, 5.773502691896255534, -7.874999999999974243 ) ) ;
#33639=EDGE_CURVE ( 'NONE', #13865, #15207, #22780, .T. ) ;
#33641=CARTESIAN_POINT ( 'NONE',  ( -5.000000000000003553, -8.660254037844383745, -143.5000000000000000 ) ) ;
#33642=CYLINDRICAL_SURFACE ( 'NONE', #13069, 9.999999999999998224 ) ;
#33644=CARTESIAN_POINT ( 'NONE',  ( 5.405949406249999534, 9.363379034771803333, -137.7812500020483810 ) ) ;
#33645=CARTESIAN_POINT ( 'NONE',  ( 10.00000000000000000, 5.773502691896255534, -190.8750000000000000 ) ) ;
#33646=CARTESIAN_POINT ( 'NONE',  ( -5.000000000000003553, -8.660254037844383745, -184.3750000040967905 ) ) ;
#33647=CARTESIAN_POINT ( 'NONE',  ( -5.405949406250003975, -9.363379034771801557, -114.5312500020483952 ) ) ;
#33648=ORIENTED_EDGE ( 'NONE', *, *, #13142, .T. ) ;
#33649=CARTESIAN_POINT ( 'NONE',  ( -9.999999999999998224, 1.224646799147353059E-15, -166.2500000000000000 ) ) ;
#33650=AXIS2_PLACEMENT_3D ( 'NONE', #39529, #16419, #28987 ) ;
#33651=ORIENTED_EDGE ( 'NONE', *, *, #4339, .F. ) ;
#33652=ORIENTED_EDGE ( 'NONE', *, *, #38642, .F. ) ;
#33654=CARTESIAN_POINT ( 'NONE',  ( 5.405949406249992428, -9.363379034771808662, -48.28125000204838813 ) ) ;
#33656=CARTESIAN_POINT ( 'NONE',  ( 10.81189881249999907, 6.242252689847868297, -98.71875000204838102 ) ) ;
#33657=CARTESIAN_POINT ( 'NONE',  ( -10.81189881249999729, 1.324075727343319199E-15, -123.7812500020483952 ) ) ;
#33658=ORIENTED_EDGE ( 'NONE', *, *, #41105, .F. ) ;
#33659=CARTESIAN_POINT ( 'NONE',  ( -5.000000000000003553, -8.660254037844383745, -133.0000000000000000 ) ) ;
#33660=CARTESIAN_POINT ( 'NONE',  ( 5.405949406249999534, 9.363379034771803333, -193.0937500020484094 ) ) ;
#33662=CARTESIAN_POINT ( 'NONE',  ( -10.00000000000102496, 5.773502691895664007, -54.25000000409675494 ) ) ;
#33663=CARTESIAN_POINT ( 'NONE',  ( -2.293366432827344421E-15, -12.48450537969573659, -120.2187500020483952 ) ) ;
#33667=CARTESIAN_POINT ( 'NONE',  ( -9.999999999999998224, 1.224646799147353059E-15, -189.1250000040967905 ) ) ;
#33669=CARTESIAN_POINT ( 'NONE',  ( 10.81189881249999551, -6.242252689847874514, -178.6562500020484094 ) ) ;
#33670=CARTESIAN_POINT ( 'NONE',  ( 9.999999999999998224, 0.000000000000000000, -0.8750000040967653714 ) ) ;
#33672=CARTESIAN_POINT ( 'NONE',  ( -5.405949406250003975, -9.363379034771801557, -57.34375000204835970 ) ) ;
#33673=CARTESIAN_POINT ( 'NONE',  ( 5.405949406249992428, -9.363379034771808662, -39.09375000204837391 ) ) ;
#33675=CARTESIAN_POINT ( 'NONE',  ( 10.81189881249999551, -6.242252689847874514, -7.656250002048367698 ) ) ;
#33678=CARTESIAN_POINT ( 'NONE',  ( -10.00000000000000000, -5.773502691896251982, -107.6249999999999858 ) ) ;
#33685=CARTESIAN_POINT ( 'NONE',  ( 10.81189881249999729, 0.000000000000000000, -106.5312500020483810 ) ) ;
#33686=ORIENTED_EDGE ( 'NONE', *, *, #4762, .F. ) ;
#33687=CARTESIAN_POINT ( 'NONE',  ( -9.999999999999998224, 1.224646799147353059E-15, -12.12500000409674783 ) ) ;
#33689=CARTESIAN_POINT ( 'NONE',  ( 9.999999999999998224, 0.000000000000000000, -135.8750000040967905 ) ) ;
#33691=EDGE_LOOP ( 'NONE', ( #25845, #36484, #34214, #25325 ) ) ;
#33692=CARTESIAN_POINT ( 'NONE',  ( 4.999999999999992006, -8.660254037844389075, -36.74999999999997868 ) ) ;
#33693=CARTESIAN_POINT ( 'NONE',  ( -2.293366432827344421E-15, -12.48450537969573659, -39.40625000204835260 ) ) ;
#33695=CARTESIAN_POINT ( 'NONE',  ( -9.999999999999998224, 1.224646799147353059E-15, -57.12500000409676204 ) ) ;
#33696=EDGE_CURVE ( 'NONE', #4287, #40862, #1834, .T. ) ;
#33697=CARTESIAN_POINT ( 'NONE',  ( -2.293366432827344421E-15, -12.48450537969573659, -142.9062500020483810 ) ) ;
#33698=LINE ( 'NONE', #7147, #41715 ) ;
#33700=ORIENTED_EDGE ( 'NONE', *, *, #31560, .T. ) ;
#33701=AXIS2_PLACEMENT_3D ( 'NONE', #31136, #28112, #25090 ) ;
#33702=CARTESIAN_POINT ( 'NONE',  ( -2.121150477449813534E-15, -11.54700538379251284, -106.2500000040967905 ) ) ;
#33704=CARTESIAN_POINT ( 'NONE',  ( -5.000000000000003553, -8.660254037844383745, -55.37500000409675494 ) ) ;
#33705=CARTESIAN_POINT ( 'NONE',  ( 10.81189881249999907, 6.242252689847868297, -164.7187500020483810 ) ) ;
#33707=CARTESIAN_POINT ( 'NONE',  ( 10.81189881249999907, 6.242252689847868297, -17.71875000204836681 ) ) ;
#33708=FACE_OUTER_BOUND ( 'NONE', #27629, .T. ) ;
#33709=CARTESIAN_POINT ( 'NONE',  ( 5.405949406249999534, 9.363379034771803333, -145.0937500020483810 ) ) ;
#33710=CARTESIAN_POINT ( 'NONE',  ( 7.644554776091147741E-16, 12.48450537969573659, -135.9687500020483810 ) ) ;
#33711=CARTESIAN_POINT ( 'NONE',  ( -10.81189881249999907, -6.242252689847864744, -107.1562500020483952 ) ) ;
#33715=CARTESIAN_POINT ( 'NONE',  ( 10.81189881249999551, -6.242252689847874514, -8.968750002048359704 ) ) ;
#33718=( BOUNDED_CURVE ( )  B_SPLINE_CURVE ( 2, ( #41659, #15111, #12095, #41445, #25077, #38222, #25288 ),
 .UNSPECIFIED., .F., .F. ) 
 B_SPLINE_CURVE_WITH_KNOTS ( ( 3, 2, 2, 3 ),
 ( 0.05970149253731348721, 0.06094527363184085167, 0.06218905472636821613, 0.06343283582089558059 ),
 .UNSPECIFIED. ) 
 CURVE ( )  GEOMETRIC_REPRESENTATION_ITEM ( )  RATIONAL_B_SPLINE_CURVE ( ( 0.9999999999999940048, 0.8660254037844447028, 1.000000000000000000, 0.8660254037844387076, 1.000000000000000000, 0.8660254037844327124, 1.000000000000005995 ) ) 
 REPRESENTATION_ITEM ( '' )  );
#33720=CARTESIAN_POINT ( 'NONE',  ( -9.999999999999998224, 1.224646799147353059E-15, -124.6250000040967763 ) ) ;
#33723=CARTESIAN_POINT ( 'NONE',  ( 5.405949406249992428, -9.363379034771808662, -81.09375000204838102 ) ) ;
#33724=CARTESIAN_POINT ( 'NONE',  ( -10.81189881249999729, 1.324075727343319199E-15, -63.59375000204836681 ) ) ;
#33725=CARTESIAN_POINT ( 'NONE',  ( -9.999999999999742428, -5.773502691896402084, -117.0000000040967763 ) ) ;
#33726=CARTESIAN_POINT ( 'NONE',  ( 7.644554776091147741E-16, 12.48450537969573659, -40.15625000204836681 ) ) ;
#33728=CYLINDRICAL_SURFACE ( 'NONE', #10950, 9.999999999999998224 ) ;
#33730=CARTESIAN_POINT ( 'NONE',  ( -10.00000000000000000, -5.773502691896251982, -133.1250000000000000 ) ) ;
#33731=CARTESIAN_POINT ( 'NONE',  ( -5.405949406249996869, 9.363379034771805109, -128.5312500020484094 ) ) ;
#33734=CARTESIAN_POINT ( 'NONE',  ( 7.644554776091147741E-16, 12.48450537969573659, -20.65625000204838457 ) ) ;
#33735=ORIENTED_EDGE ( 'NONE', *, *, #37813, .T. ) ;
#33736=( BOUNDED_CURVE ( )  B_SPLINE_CURVE ( 2, ( #37190, #27707, #17330, #17538, #1600, #20790, #27493 ),
 .UNSPECIFIED., .F., .F. ) 
 B_SPLINE_CURVE_WITH_KNOTS ( ( 3, 2, 2, 3 ),
 ( 0.6604477611940301474, 0.6616915422885575326, 0.6629353233830848069, 0.6641791044776121922 ),
 .UNSPECIFIED. ) 
 CURVE ( )  GEOMETRIC_REPRESENTATION_ITEM ( )  RATIONAL_B_SPLINE_CURVE ( ( 0.9999999999999641398, 0.8660254037844745678, 1.000000000000000000, 0.8660254037844387076, 1.000000000000000000, 0.8660254037844148378, 1.000000000000023981 ) ) 
 REPRESENTATION_ITEM ( '' )  );
#33739=CARTESIAN_POINT ( 'NONE',  ( -9.999999999999998224, 1.224646799147353059E-15, -185.7500000000000000 ) ) ;
#33740=CARTESIAN_POINT ( 'NONE',  ( -4.999999999999996447, 8.660254037844387298, -30.37500000409676204 ) ) ;
#33741=CARTESIAN_POINT ( 'NONE',  ( -9.999999999999998224, 1.224646799147353059E-15, -9.125000004096744277 ) ) ;
#33743=EDGE_CURVE ( 'NONE', #32436, #10245, #31331, .T. ) ;
#33745=CARTESIAN_POINT ( 'NONE',  ( 10.81189881249999729, 0.000000000000000000, -156.0312500020484094 ) ) ;
#33746=CARTESIAN_POINT ( 'NONE',  ( -2.293366432827344421E-15, -12.48450537969573659, -132.2187500020483810 ) ) ;
#33751=AXIS2_PLACEMENT_3D ( 'NONE', #29487, #12633, #25620 ) ;
#33752=ORIENTED_EDGE ( 'NONE', *, *, #35208, .F. ) ;
#33754=CARTESIAN_POINT ( 'NONE',  ( -10.81189881249999729, 6.242252689847871849, -114.7187500020483810 ) ) ;
#33756=ADVANCED_FACE ( 'NONE', ( #33356 ), #24280, .T. ) ;
#33757=CARTESIAN_POINT ( 'NONE',  ( 9.999999999999998224, 0.000000000000000000, -129.8750000040967905 ) ) ;
#33758=CARTESIAN_POINT ( 'NONE',  ( 7.644554776091147741E-16, 12.48450537969573659, -188.4687500020484094 ) ) ;
#33759=CARTESIAN_POINT ( 'NONE',  ( 5.405949406249992428, -9.363379034771808662, -39.09375000204837391 ) ) ;
#33760=CARTESIAN_POINT ( 'NONE',  ( 7.070501591499376803E-16, 11.54700538379251284, -62.00000000409677625 ) ) ;
#33761=CARTESIAN_POINT ( 'NONE',  ( -10.81189881249999729, 6.242252689847871849, -177.7187500020484379 ) ) ;
#33762=CARTESIAN_POINT ( 'NONE',  ( 5.405949406249999534, 9.363379034771803333, -161.5937500020484094 ) ) ;
#33765=CARTESIAN_POINT ( 'NONE',  ( -4.999999999999996447, 8.660254037844387298, -133.8750000040967905 ) ) ;
#33766=CARTESIAN_POINT ( 'NONE',  ( -9.999999999999998224, 1.224646799147353059E-15, -35.74999999999997868 ) ) ;
#33768=AXIS2_PLACEMENT_3D ( 'NONE', #30357, #16944, #30142 ) ;
#33769=CARTESIAN_POINT ( 'NONE',  ( 5.405949406249999534, 9.363379034771803333, -89.59375000204838102 ) ) ;
#33771=CARTESIAN_POINT ( 'NONE',  ( 10.81189881249999551, -6.242252689847874514, -66.15625000204839523 ) ) ;
#33774=CARTESIAN_POINT ( 'NONE',  ( 5.405949406249992428, -9.363379034771808662, -124.7812500020483952 ) ) ;
#33775=CARTESIAN_POINT ( 'NONE',  ( 5.405949406249999534, 9.363379034771803333, -151.2812500020484094 ) ) ;
#33777=CARTESIAN_POINT ( 'NONE',  ( 9.999999999999998224, 0.000000000000000000, -128.3750000040967905 ) ) ;
#33779=ORIENTED_EDGE ( 'NONE', *, *, #19100, .T. ) ;
#33783=CARTESIAN_POINT ( 'NONE',  ( -10.81189881249999907, -6.242252689847864744, -185.1562500020484094 ) ) ;
#33785=ORIENTED_EDGE ( 'NONE', *, *, #24077, .F. ) ;
#33786=CARTESIAN_POINT ( 'NONE',  ( -5.000000000000003553, -8.660254037844383745, -51.99999999999996447 ) ) ;
#33788=CARTESIAN_POINT ( 'NONE',  ( -2.121150477449813534E-15, -11.54700538379251284, -67.25000000409676204 ) ) ;
#33789=LINE ( 'NONE', #13900, #3784 ) ;
#33792=CARTESIAN_POINT ( 'NONE',  ( 5.405949406249999534, 9.363379034771803333, -61.28125000204837391 ) ) ;
#33795=CYLINDRICAL_SURFACE ( 'NONE', #6935, 9.999999999999998224 ) ;
#33796=CARTESIAN_POINT ( 'NONE',  ( 5.405949406249999534, 9.363379034771803333, -173.7812500020484094 ) ) ;
#33800=( BOUNDED_CURVE ( )  B_SPLINE_CURVE ( 2, ( #25618, #3159, #6188, #32938, #35960, #39398, #35548 ),
 .UNSPECIFIED., .F., .F. ) 
 B_SPLINE_CURVE_WITH_KNOTS ( ( 3, 2, 2, 3 ),
 ( 0.6641791044776121922, 0.6654228855721395774, 0.6666666666666668517, 0.6679104477611942370 ),
 .UNSPECIFIED. ) 
 CURVE ( )  GEOMETRIC_REPRESENTATION_ITEM ( )  RATIONAL_B_SPLINE_CURVE ( ( 0.9999999999999761302, 0.8660254037844625774, 1.000000000000000000, 0.8660254037844387076, 1.000000000000000000, 0.8660254037844148378, 1.000000000000023981 ) ) 
 REPRESENTATION_ITEM ( '' )  );
#33802=DIRECTION ( 'NONE',  ( 1.000000000000000000, 0.000000000000000000, 0.000000000000000000 ) ) ;
#33803=CARTESIAN_POINT ( 'NONE',  ( 10.00000000000012257, -5.773502691896187144, -169.0000000040967620 ) ) ;
#33805=CARTESIAN_POINT ( 'NONE',  ( -10.81189881249999729, 6.242252689847871849, -83.40625000204836681 ) ) ;
#33807=CARTESIAN_POINT ( 'NONE',  ( -9.999999999999998224, 1.224646799147353059E-15, -24.12500000409675849 ) ) ;
#33809=VERTEX_POINT ( 'NONE', #13668 ) ;
#33811=CARTESIAN_POINT ( 'NONE',  ( -10.81189881249999907, -6.242252689847864744, -22.96875000204837747 ) ) ;
#33812=CARTESIAN_POINT ( 'NONE',  ( -10.81189881249999729, 6.242252689847871849, -11.40625000204835438 ) ) ;
#33813=CARTESIAN_POINT ( 'NONE',  ( 10.81189881249999551, -6.242252689847874514, -67.46875000204838102 ) ) ;
#33814=CARTESIAN_POINT ( 'NONE',  ( 0.000000000000000000, 0.000000000000000000, -200.0000000000000000 ) ) ;
#33817=CARTESIAN_POINT ( 'NONE',  ( -10.81189881249999907, -6.242252689847864744, -187.9687500020484094 ) ) ;
#33818=EDGE_CURVE ( 'NONE', #20035, #39731, #13881, .T. ) ;
#33820=CARTESIAN_POINT ( 'NONE',  ( 9.999999999999998224, 0.000000000000000000, -200.0000000000000000 ) ) ;
#33821=CARTESIAN_POINT ( 'NONE',  ( -10.00000000000001421, 5.773502691896249317, -199.3750000000000000 ) ) ;
#33822=CARTESIAN_POINT ( 'NONE',  ( 9.999999999999479527, 5.773502691896553074, -71.25000000409674783 ) ) ;
#33823=CARTESIAN_POINT ( 'NONE',  ( -2.121150477449813534E-15, -11.54700538379251284, -104.3749999999999858 ) ) ;
#33824=CARTESIAN_POINT ( 'NONE',  ( -9.999999999999998224, 1.224646799147353059E-15, -90.12500000409677625 ) ) ;
#33825=CARTESIAN_POINT ( 'NONE',  ( 10.81189881249999729, 0.000000000000000000, -112.3437500020483810 ) ) ;
#33826=CARTESIAN_POINT ( 'NONE',  ( 9.999999999999998224, 0.000000000000000000, -109.9999999999999858 ) ) ;
#33827=CARTESIAN_POINT ( 'NONE',  ( -5.405949406250003975, -9.363379034771801557, -93.53125000204838102 ) ) ;
#33828=CARTESIAN_POINT ( 'NONE',  ( 7.644554776091147741E-16, 12.48450537969573659, -98.46875000204838102 ) ) ;
#33831=CARTESIAN_POINT ( 'NONE',  ( -10.00000000000000000, -5.773502691896251982, -151.5000000040967905 ) ) ;
#33836=FACE_OUTER_BOUND ( 'NONE', #28930, .T. ) ;
#33838=CARTESIAN_POINT ( 'NONE',  ( -9.999999999999998224, 5.773502691896259087, -70.37499999999998579 ) ) ;
#33840=CARTESIAN_POINT ( 'NONE',  ( -4.999999999999996447, 8.660254037844387298, -93.37500000409677625 ) ) ;
#33841=AXIS2_PLACEMENT_3D ( 'NONE', #40038, #362, #573 ) ;
#33842=PLANE ( 'NONE',  #12064 ) ;
#33844=CARTESIAN_POINT ( 'NONE',  ( 10.81189881249999729, 0.000000000000000000, -85.53125000204838102 ) ) ;
#33847=DIRECTION ( 'NONE',  ( -0.000000000000000000, -0.000000000000000000, 1.000000000000000000 ) ) ;
#33849=VERTEX_POINT ( 'NONE', #37425 ) ;
#33850=CARTESIAN_POINT ( 'NONE',  ( -9.999999999999998224, 1.224646799147353059E-15, -2.749999999999974687 ) ) ;
#33852=CARTESIAN_POINT ( 'NONE',  ( 5.405949406249992428, -9.363379034771808662, -13.59375000204834905 ) ) ;
#33855=CARTESIAN_POINT ( 'NONE',  ( -10.81189881249999907, -6.242252689847864744, -134.1562500020483810 ) ) ;
#33856=CARTESIAN_POINT ( 'NONE',  ( 4.999999999999992006, -8.660254037844389075, -179.2500000000000284 ) ) ;
#33857=DIRECTION ( 'NONE',  ( 3.186890520727785033E-16, -0.7071067811865493491, 0.7071067811865456854 ) ) ;
#33858=CARTESIAN_POINT ( 'NONE',  ( -5.405949406249996869, 9.363379034771805109, -113.5312500020483952 ) ) ;
#33859=VERTEX_POINT ( 'NONE', #14302 ) ;
#33863=CARTESIAN_POINT ( 'NONE',  ( 7.644554776091147741E-16, 12.48450537969573659, -40.15625000204836681 ) ) ;
#33866=CARTESIAN_POINT ( 'NONE',  ( -5.405949406249996869, 9.363379034771805109, -96.84375000204838102 ) ) ;
#33867=CARTESIAN_POINT ( 'NONE',  ( 9.999999999999998224, 0.000000000000000000, -200.0000000000000000 ) ) ;
#33870=CARTESIAN_POINT ( 'NONE',  ( 7.644554776091147741E-16, 12.48450537969573659, -198.9687500020484094 ) ) ;
#33871=EDGE_CURVE ( 'NONE', #25200, #22602, #37360, .T. ) ;
#33873=CARTESIAN_POINT ( 'NONE',  ( -9.999999999999998224, 1.224646799147353059E-15, -137.7499999999999716 ) ) ;
#33875=CARTESIAN_POINT ( 'NONE',  ( -5.405949406250003975, -9.363379034771801557, -127.8437500020483952 ) ) ;
#33876=PRODUCT_DEFINITION_SHAPE ( 'NONE', 'NONE',  #20655 ) ;
#33881=CARTESIAN_POINT ( 'NONE',  ( -9.999999999999998224, 5.773502691896259087, -184.7500000040968189 ) ) ;
#33883=CARTESIAN_POINT ( 'NONE',  ( 5.405949406249999534, 9.363379034771803333, -176.7812500020484094 ) ) ;
#33884=CARTESIAN_POINT ( 'NONE',  ( -9.999999999999998224, 1.224646799147353059E-15, -179.7500000000000284 ) ) ;
#33887=CARTESIAN_POINT ( 'NONE',  ( -2.293366432827344421E-15, -12.48450537969573659, -49.71875000204835970 ) ) ;
#33888=CARTESIAN_POINT ( 'NONE',  ( 7.644554776091147741E-16, 12.48450537969573659, -44.46875000204836681 ) ) ;
#33890=CARTESIAN_POINT ( 'NONE',  ( 5.405949406249992428, -9.363379034771808662, -13.78125000204835615 ) ) ;
#33892=CARTESIAN_POINT ( 'NONE',  ( -2.121150477449813534E-15, -11.54700538379251284, -92.75000000409677625 ) ) ;
#33894=CARTESIAN_POINT ( 'NONE',  ( 5.000000000000000000, 8.660254037844385522, -96.24999999999998579 ) ) ;
#33896=CARTESIAN_POINT ( 'NONE',  ( -10.00000000000000000, -5.773502691896251982, -112.5000000040967905 ) ) ;
#33897=CARTESIAN_POINT ( 'NONE',  ( 9.999999999999994671, -5.773502691896262640, -168.6250000000000000 ) ) ;
#33900=CARTESIAN_POINT ( 'NONE',  ( 5.405949406249999534, 9.363379034771803333, -109.2812500020483810 ) ) ;
#33901=EDGE_LOOP ( 'NONE', ( #41984, #4174, #217, #1974 ) ) ;
#33903=CARTESIAN_POINT ( 'NONE',  ( -9.999999999999998224, 1.224646799147353059E-15, -139.2499999999999716 ) ) ;
#33909=CARTESIAN_POINT ( 'NONE',  ( 5.000000000000000000, 8.660254037844385522, -34.74999999999997868 ) ) ;
#33911=CARTESIAN_POINT ( 'NONE',  ( 5.405949406249999534, 9.363379034771803333, -32.78125000204837391 ) ) ;
#33912=CARTESIAN_POINT ( 'NONE',  ( 9.999999999999996447, -5.773502691896262640, -161.1250000000000284 ) ) ;
#33913=CARTESIAN_POINT ( 'NONE',  ( 9.999999999999998224, 0.000000000000000000, -200.0000000000000000 ) ) ;
#33915=CARTESIAN_POINT ( 'NONE',  ( -5.405949406250003975, -9.363379034771801557, -135.5312500020484094 ) ) ;
#33916=VERTEX_POINT ( 'NONE', #31828 ) ;
#33917=VERTEX_POINT ( 'NONE', #28583 ) ;
#33918=ORIENTED_EDGE ( 'NONE', *, *, #9091, .T. ) ;
#33921=DIRECTION ( 'NONE',  ( -0.000000000000000000, -0.000000000000000000, 1.000000000000000000 ) ) ;
#33922=CARTESIAN_POINT ( 'NONE',  ( 7.644554776091147741E-16, 12.48450537969573659, -164.4687500020483810 ) ) ;
#33924=CARTESIAN_POINT ( 'NONE',  ( -10.81189881249999729, 1.324075727343319199E-15, -15.59375000204835082 ) ) ;
#33925=CYLINDRICAL_SURFACE ( 'NONE', #27423, 9.999999999999998224 ) ;
#33926=CARTESIAN_POINT ( 'NONE',  ( 7.644554776091147741E-16, 12.48450537969573659, -149.4687500020484663 ) ) ;
#33927=CARTESIAN_POINT ( 'NONE',  ( -10.81189881249999729, 1.324075727343319199E-15, -134.0937500020483810 ) ) ;
#33928=( BOUNDED_CURVE ( )  B_SPLINE_CURVE ( 2, ( #36510, #1113, #17699, #30479, #37137, #17274, #23571 ),
 .UNSPECIFIED., .F., .F. ) 
 B_SPLINE_CURVE_WITH_KNOTS ( ( 3, 2, 2, 3 ),
 ( 0.2052238805970149627, 0.2064676616915423202, 0.2077114427860697055, 0.2089552238805970630 ),
 .UNSPECIFIED. ) 
 CURVE ( )  GEOMETRIC_REPRESENTATION_ITEM ( )  RATIONAL_B_SPLINE_CURVE ( ( 0.9999999999999970024, 0.8660254037844417052, 1.000000000000000000, 0.8660254037844387076, 1.000000000000000000, 0.8660254037844327124, 1.000000000000005995 ) ) 
 REPRESENTATION_ITEM ( '' )  );
#33929=CARTESIAN_POINT ( 'NONE',  ( 5.405949406249992428, -9.363379034771808662, -106.7812500020483810 ) ) ;
#33933=CARTESIAN_POINT ( 'NONE',  ( 10.81189881249999907, 6.242252689847868297, -7.218750002048349934 ) ) ;
#33936=CARTESIAN_POINT ( 'NONE',  ( -5.000000000000003553, -8.660254037844383745, -178.3750000040967905 ) ) ;
#33940=ADVANCED_FACE ( 'NONE', ( #18856 ), #5705, .T. ) ;
#33941=CARTESIAN_POINT ( 'NONE',  ( 10.81189881249999729, 0.000000000000000000, -76.34375000204838102 ) ) ;
#33942=CARTESIAN_POINT ( 'NONE',  ( -10.81189881249999907, -6.242252689847864744, -67.96875000204838102 ) ) ;
#33943=CARTESIAN_POINT ( 'NONE',  ( -2.121150477449813534E-15, -11.54700538379251284, -19.25000000409677625 ) ) ;
#33944=CARTESIAN_POINT ( 'NONE',  ( -10.81189881249999729, 6.242252689847871849, -35.40625000204836681 ) ) ;
#33948=CARTESIAN_POINT ( 'NONE',  ( -4.999999999999996447, 8.660254037844387298, -118.5000000000000000 ) ) ;
#33949=CARTESIAN_POINT ( 'NONE',  ( -5.405949406249996869, 9.363379034771805109, -133.0312500020484094 ) ) ;
#33952=CARTESIAN_POINT ( 'NONE',  ( -10.81189881249999729, 1.324075727343319199E-15, -15.78125000204835793 ) ) ;
#33953=ORIENTED_EDGE ( 'NONE', *, *, #22229, .F. ) ;
#33956=CARTESIAN_POINT ( 'NONE',  ( 9.999999999998456346, 5.773502691897149042, -9.374999999999944933 ) ) ;
#33957=CARTESIAN_POINT ( 'NONE',  ( -4.999999999999996447, 8.660254037844387298, -31.87500000409676559 ) ) ;
#33958=CARTESIAN_POINT ( 'NONE',  ( 0.000000000000000000, 0.000000000000000000, -200.0000000000000000 ) ) ;
#33960=AXIS2_PLACEMENT_3D ( 'NONE', #6815, #28861, #29069 ) ;
#33961=CARTESIAN_POINT ( 'NONE',  ( -9.999999999999479527, -5.773502691896549521, -146.6249999999999716 ) ) ;
#33962=CARTESIAN_POINT ( 'NONE',  ( -10.81189881249999729, 1.324075727343319199E-15, -149.2812500020483810 ) ) ;
#33963=CARTESIAN_POINT ( 'NONE',  ( -10.81189881249999729, 6.242252689847871849, -132.7187500020483810 ) ) ;
#33965=ORIENTED_EDGE ( 'NONE', *, *, #12507, .T. ) ;
#33966=CARTESIAN_POINT ( 'NONE',  ( 9.999999999999998224, 0.000000000000000000, -85.99999999999998579 ) ) ;
#33967=ORIENTED_EDGE ( 'NONE', *, *, #39942, .F. ) ;
#33969=CARTESIAN_POINT ( 'NONE',  ( 5.405949406249999534, 9.363379034771803333, -113.5937500020483810 ) ) ;
#33970=VERTEX_POINT ( 'NONE', #2264 ) ;
#33971=CARTESIAN_POINT ( 'NONE',  ( -10.00000000000076916, 5.773502691895813221, -129.2500000040967905 ) ) ;
#33973=CARTESIAN_POINT ( 'NONE',  ( -5.405949406250003975, -9.363379034771801557, -189.3437500020483810 ) ) ;
#33974=CARTESIAN_POINT ( 'NONE',  ( 10.81189881249999551, -6.242252689847874514, -41.96875000204835970 ) ) ;
#33975=CARTESIAN_POINT ( 'NONE',  ( -6.904799017827355279, -7.420746795541425911, 9.002545116942468623E-15 ) ) ;
#33976=CARTESIAN_POINT ( 'NONE',  ( -10.81189881249999729, 6.242252689847871849, -170.2187500020483810 ) ) ;
#33977=CARTESIAN_POINT ( 'NONE',  ( 5.405949406249992428, -9.363379034771808662, -163.5937500020484094 ) ) ;
#33980=CARTESIAN_POINT ( 'NONE',  ( -9.999999999999998224, 1.224646799147353059E-15, -43.24999999999998579 ) ) ;
#33981=( BOUNDED_CURVE ( )  B_SPLINE_CURVE ( 2, ( #24785, #17842, #1470, #40289, #4057, #17199, #30400 ),
 .UNSPECIFIED., .F., .F. ) 
 B_SPLINE_CURVE_WITH_KNOTS ( ( 3, 2, 2, 3 ),
 ( 0.8880597014925376564, 0.8893034825870650417, 0.8905472636815924270, 0.8917910447761197013 ),
 .UNSPECIFIED. ) 
 CURVE ( )  GEOMETRIC_REPRESENTATION_ITEM ( )  RATIONAL_B_SPLINE_CURVE ( ( 0.9999999999999641398, 0.8660254037844745678, 1.000000000000000000, 0.8660254037844387076, 1.000000000000000000, 0.8660254037844028474, 1.000000000000035971 ) ) 
 REPRESENTATION_ITEM ( '' )  );
#33984=CARTESIAN_POINT ( 'NONE',  ( 10.81189881249999907, 6.242252689847868297, -86.71875000204836681 ) ) ;
#33985=CARTESIAN_POINT ( 'NONE',  ( -9.999999999999479527, -5.773502691896549521, -113.6249999999999716 ) ) ;
#33986=CARTESIAN_POINT ( 'NONE',  ( 10.81189881249999729, 0.000000000000000000, -55.53125000204836681 ) ) ;
#33987=CARTESIAN_POINT ( 'NONE',  ( 7.070501591499376803E-16, 11.54700538379251284, -87.50000000409677625 ) ) ;
#33989=CARTESIAN_POINT ( 'NONE',  ( -2.293366432827344421E-15, -12.48450537969573659, -123.4062500020484094 ) ) ;
#33990=CARTESIAN_POINT ( 'NONE',  ( -10.81189881249999729, 6.242252689847871849, -150.9062500020484094 ) ) ;
#33993=CARTESIAN_POINT ( 'NONE',  ( -2.121150477449813534E-15, -11.54700538379251284, -133.2500000040967905 ) ) ;
#33995=ORIENTED_EDGE ( 'NONE', *, *, #34944, .F. ) ;
#33999=CARTESIAN_POINT ( 'NONE',  ( 5.405949406249999534, 9.363379034771803333, -190.2812500020484094 ) ) ;
#34001=CARTESIAN_POINT ( 'NONE',  ( 4.999999999999992006, -8.660254037844389075, -51.74999999999996447 ) ) ;
#34003=CARTESIAN_POINT ( 'NONE',  ( -9.999999999999998224, 1.224646799147353059E-15, -57.12500000409676204 ) ) ;
#34004=CARTESIAN_POINT ( 'NONE',  ( 9.999999999999998224, 0.000000000000000000, -153.5000000000000000 ) ) ;
#34005=CARTESIAN_POINT ( 'NONE',  ( 10.00000000000012257, -5.773502691896187144, -165.6250000000000000 ) ) ;
#34007=CARTESIAN_POINT ( 'NONE',  ( -5.405949406250003975, -9.363379034771801557, -48.53125000204838813 ) ) ;
#34008=ADVANCED_FACE ( 'NONE', ( #1610 ), #2040, .T. ) ;
#34011=CARTESIAN_POINT ( 'NONE',  ( -9.999999999999998224, 1.224646799147353059E-15, -200.0000000000000000 ) ) ;
#34012=CARTESIAN_POINT ( 'NONE',  ( -10.81189881249999907, -6.242252689847864744, -176.1562500020483810 ) ) ;
#34014=DIRECTION ( 'NONE',  ( -0.000000000000000000, -0.000000000000000000, 1.000000000000000000 ) ) ;
#34015=CARTESIAN_POINT ( 'NONE',  ( 9.999999999999998224, 0.000000000000000000, -117.5000000000000000 ) ) ;
#34017=CARTESIAN_POINT ( 'NONE',  ( -9.999999999999872102, -5.773502691896326589, -163.5000000040967620 ) ) ;
#34018=CARTESIAN_POINT ( 'NONE',  ( -5.405949406249996869, 9.363379034771805109, -88.03125000204838102 ) ) ;
#34020=CARTESIAN_POINT ( 'NONE',  ( -10.00000000000051337, 5.773502691895962435, -80.87499999999995737 ) ) ;
#34021=VERTEX_POINT ( 'NONE', #18201 ) ;
#34022=ORIENTED_EDGE ( 'NONE', *, *, #12040, .T. ) ;
#34024=CARTESIAN_POINT ( 'NONE',  ( 10.81189881249999729, 0.000000000000000000, -38.84375000204837391 ) ) ;
#34025=CARTESIAN_POINT ( 'NONE',  ( 5.405949406249999534, 9.363379034771803333, -26.59375000204835970 ) ) ;
#34026=CARTESIAN_POINT ( 'NONE',  ( -10.81189881249999729, 6.242252689847871849, -15.90625000204837391 ) ) ;
#34027=CARTESIAN_POINT ( 'NONE',  ( 10.81189881249999729, 0.000000000000000000, -65.84375000204836681 ) ) ;
#34028=CYLINDRICAL_SURFACE ( 'NONE', #38751, 9.999999999999998224 ) ;
#34031=CARTESIAN_POINT ( 'NONE',  ( -2.293366432827344421E-15, -12.48450537969573659, -181.7187500020484094 ) ) ;
#34035=CARTESIAN_POINT ( 'NONE',  ( 9.999999999999998224, 0.000000000000000000, -141.5000000000000000 ) ) ;
#34037=DIRECTION ( 'NONE',  ( -0.000000000000000000, -0.000000000000000000, 1.000000000000000000 ) ) ;
#34038=CARTESIAN_POINT ( 'NONE',  ( -2.293366432827344421E-15, -12.48450537969573659, -112.7187500020483952 ) ) ;
#34040=CARTESIAN_POINT ( 'NONE',  ( -5.405949406250003975, -9.363379034771801557, -89.03125000204838102 ) ) ;
#34041=CARTESIAN_POINT ( 'NONE',  ( 5.405949406249999534, 9.363379034771803333, -103.0937500020483810 ) ) ;
#34044=CARTESIAN_POINT ( 'NONE',  ( -2.121150477449813534E-15, -11.54700538379251284, -154.2500000040967620 ) ) ;
#34048=CARTESIAN_POINT ( 'NONE',  ( -10.00000000000038547, 5.773502691896036154, -153.2500000040967905 ) ) ;
#34049=CARTESIAN_POINT ( 'NONE',  ( -9.999999999999998224, 1.224646799147353059E-15, -20.74999999999996447 ) ) ;
#34051=CARTESIAN_POINT ( 'NONE',  ( 9.999999999999998224, 0.000000000000000000, -63.49999999999997158 ) ) ;
#34052=CARTESIAN_POINT ( 'NONE',  ( -2.121150477449813534E-15, -11.54700538379251284, -74.37499999999995737 ) ) ;
#34054=CARTESIAN_POINT ( 'NONE',  ( -2.121150477449813534E-15, -11.54700538379251284, -83.75000000409677625 ) ) ;
#34055=( BOUNDED_CURVE ( )  B_SPLINE_CURVE ( 2, ( #24505, #41078, #21033, #11523, #40654, #2058, #21248 ),
 .UNSPECIFIED., .F., .F. ) 
 B_SPLINE_CURVE_WITH_KNOTS ( ( 3, 2, 2, 3 ),
 ( 0.8992537313432839019, 0.9004975124378112872, 0.9017412935323385614, 0.9029850746268659467 ),
 .UNSPECIFIED. ) 
 CURVE ( )  GEOMETRIC_REPRESENTATION_ITEM ( )  RATIONAL_B_SPLINE_CURVE ( ( 0.9999999999999641398, 0.8660254037844745678, 1.000000000000000000, 0.8660254037844387076, 1.000000000000000000, 0.8660254037844148378, 1.000000000000023981 ) ) 
 REPRESENTATION_ITEM ( '' )  );
#34056=CARTESIAN_POINT ( 'NONE',  ( 9.999999999999998224, 0.000000000000000000, -115.9999999999999858 ) ) ;
#34058=CARTESIAN_POINT ( 'NONE',  ( -2.293366432827344421E-15, -12.48450537969573659, -87.40625000204838102 ) ) ;
#34060=CARTESIAN_POINT ( 'NONE',  ( 4.999999999999992006, -8.660254037844389075, -59.24999999999997158 ) ) ;
#34062=ORIENTED_EDGE ( 'NONE', *, *, #26583, .F. ) ;
#34063=CARTESIAN_POINT ( 'NONE',  ( 10.00000000000000000, 5.773502691896255534, -1.874999999999944711 ) ) ;
#34066=CARTESIAN_POINT ( 'NONE',  ( 10.81189881249999729, 6.242252689847867408, -11.71875000204837214 ) ) ;
#34069=CARTESIAN_POINT ( 'NONE',  ( -10.81189881249999907, -6.242252689847864744, -128.1562500020483810 ) ) ;
#34070=CARTESIAN_POINT ( 'NONE',  ( 9.999999999999998224, 0.000000000000000000, -182.0000000000000000 ) ) ;
#34071=CARTESIAN_POINT ( 'NONE',  ( 7.644554776091147741E-16, 12.48450537969573659, -109.1562500020483810 ) ) ;
#34072=ORIENTED_EDGE ( 'NONE', *, *, #21972, .T. ) ;
#34073=CARTESIAN_POINT ( 'NONE',  ( 9.999999999999884537, 5.773502691896319483, -195.3750000000000000 ) ) ;
#34075=ORIENTED_EDGE ( 'NONE', *, *, #1421, .T. ) ;
#34076=CARTESIAN_POINT ( 'NONE',  ( 7.644554776091147741E-16, 12.48450537969573659, -41.65625000204837391 ) ) ;
#34078=CARTESIAN_POINT ( 'NONE',  ( -2.293366432827344421E-15, -12.48450537969573659, -88.71875000204838102 ) ) ;
#34079=DIRECTION ( 'NONE',  ( -0.000000000000000000, -0.000000000000000000, 1.000000000000000000 ) ) ;
#34080=CYLINDRICAL_SURFACE ( 'NONE', #32167, 9.999999999999998224 ) ;
#34083=CARTESIAN_POINT ( 'NONE',  ( -9.999999999999998224, 1.224646799147353059E-15, -139.2499999999999716 ) ) ;
#34084=CARTESIAN_POINT ( 'NONE',  ( 5.405949406249992428, -9.363379034771808662, -127.5937500020483668 ) ) ;
#34086=CARTESIAN_POINT ( 'NONE',  ( -2.293366432827344421E-15, -12.48450537969573659, -1.906250002048373027 ) ) ;
#34088=CARTESIAN_POINT ( 'NONE',  ( 4.999999999999992006, -8.660254037844389075, -179.6250000040968189 ) ) ;
#34090=CARTESIAN_POINT ( 'NONE',  ( 5.405949406249999534, 9.363379034771803333, -178.2812500020484094 ) ) ;
#34095=CARTESIAN_POINT ( 'NONE',  ( 7.644554776091147741E-16, 12.48450537969573659, -48.96875000204835260 ) ) ;
#34096=CARTESIAN_POINT ( 'NONE',  ( 5.405949406249999534, 9.363379034771803333, -43.09375000204837391 ) ) ;
#34098=CARTESIAN_POINT ( 'NONE',  ( -10.81189881249999907, -6.242252689847864744, -6.656250002048364145 ) ) ;
#34101=CARTESIAN_POINT ( 'NONE',  ( -9.999999999999998224, 1.224646799147353059E-15, -97.24999999999998579 ) ) ;
#34103=CARTESIAN_POINT ( 'NONE',  ( -9.999999999999998224, 5.773502691896259087, -112.7500000040967763 ) ) ;
#34104=ADVANCED_BREP_SHAPE_REPRESENTATION ( '', ( #30024, #39998 ), #15874 ) ;
#34105=DIRECTION ( 'NONE',  ( -0.000000000000000000, -0.000000000000000000, 1.000000000000000000 ) ) ;
#34108=CARTESIAN_POINT ( 'NONE',  ( 10.81189881249999729, 6.242252689847867408, -107.9062500020483952 ) ) ;
#34109=ORIENTED_EDGE ( 'NONE', *, *, #16142, .F. ) ;
#34110=CARTESIAN_POINT ( 'NONE',  ( -10.00000000000154188, 5.773502691895366468, -7.750000004096709638 ) ) ;
#34113=CARTESIAN_POINT ( 'NONE',  ( 10.81189881249999907, 6.242252689847868297, -163.4062500020484094 ) ) ;
#34115=ORIENTED_EDGE ( 'NONE', *, *, #39913, .T. ) ;
#34116=CARTESIAN_POINT ( 'NONE',  ( -10.00000000000000000, -5.773502691896251982, -25.12499999999997513 ) ) ;
#34117=EDGE_CURVE ( 'NONE', #7028, #3605, #19708, .T. ) ;
#34118=CARTESIAN_POINT ( 'NONE',  ( 7.644554776091147741E-16, 12.48450537969573659, -38.65625000204835260 ) ) ;
#34119=CARTESIAN_POINT ( 'NONE',  ( -10.00000000000000000, -5.773502691896251982, -163.1250000000000284 ) ) ;
#34121=DIRECTION ( 'NONE',  ( -0.000000000000000000, -0.000000000000000000, 1.000000000000000000 ) ) ;
#34124=EDGE_CURVE ( 'NONE', #26629, #32856, #39330, .T. ) ;
#34125=CYLINDRICAL_SURFACE ( 'NONE', #15311, 9.999999999999998224 ) ;
#34126=CARTESIAN_POINT ( 'NONE',  ( 7.644554776091147741E-16, 12.48450537969573659, -137.6562500020483810 ) ) ;
#34127=CARTESIAN_POINT ( 'NONE',  ( 9.169761814809081812, 5.423027170935617036, 5.369687683974985216E-15 ) ) ;
#34128=CARTESIAN_POINT ( 'NONE',  ( -9.999999999999998224, 1.224646799147353059E-15, -174.1250000040968189 ) ) ;
#34129=EDGE_LOOP ( 'NONE', ( #38259, #39476, #6145, #24040 ) ) ;
#34131=ORIENTED_EDGE ( 'NONE', *, *, #20105, .F. ) ;
#34132=EDGE_CURVE ( 'NONE', #28672, #2082, #204, .T. ) ;
#34134=DIRECTION ( 'NONE',  ( 1.000000000000000000, 0.000000000000000000, 0.000000000000000000 ) ) ;
#34135=CARTESIAN_POINT ( 'NONE',  ( -10.81189881249999907, -6.242252689847864744, -162.4687500020483526 ) ) ;
#34136=VECTOR ( 'NONE', #19594, 1000.000000000000000 ) ;
#34139=CARTESIAN_POINT ( 'NONE',  ( 7.644554776091147741E-16, 12.48450537969573659, -15.96875000204835615 ) ) ;
#34140=CYLINDRICAL_SURFACE ( 'NONE', #24688, 9.999999999999998224 ) ;
#34142=CARTESIAN_POINT ( 'NONE',  ( -2.293366432827344421E-15, -12.48450537969573659, -145.7187500020484094 ) ) ;
#34143=CARTESIAN_POINT ( 'NONE',  ( 10.81189881249999907, 6.242252689847868297, -136.2187500020483810 ) ) ;
#34144=CARTESIAN_POINT ( 'NONE',  ( -10.81189881249999729, 6.242252689847871849, -102.9062500020483810 ) ) ;
#34148=CARTESIAN_POINT ( 'NONE',  ( 5.405949406249999534, 9.363379034771803333, -5.593750002048370362 ) ) ;
#34151=CARTESIAN_POINT ( 'NONE',  ( 9.999999999999998224, 0.000000000000000000, -5.375000004096769146 ) ) ;
#34154=CARTESIAN_POINT ( 'NONE',  ( 7.644554776091147741E-16, 12.48450537969573659, -77.46875000204838102 ) ) ;
#34155=CARTESIAN_POINT ( 'NONE',  ( 10.81189881249999907, 6.242252689847868297, -68.71875000204838102 ) ) ;
#34157=CARTESIAN_POINT ( 'NONE',  ( 7.644554776091147741E-16, 12.48450537969573659, -32.65625000204835970 ) ) ;
#34160=CARTESIAN_POINT ( 'NONE',  ( 7.070501591499377789E-16, 11.54700538379251284, -121.6249999999999858 ) ) ;
#34161=CARTESIAN_POINT ( 'NONE',  ( -2.293366432827344421E-15, -12.48450537969573659, -127.9062500020483952 ) ) ;
#34163=DIRECTION ( 'NONE',  ( 1.000000000000000000, 0.000000000000000000, 0.000000000000000000 ) ) ;
#34166=CARTESIAN_POINT ( 'NONE',  ( -10.81189881249999729, 6.242252689847871849, -14.40625000204836681 ) ) ;
#34167=ORIENTED_EDGE ( 'NONE', *, *, #7149, .F. ) ;
#34170=CARTESIAN_POINT ( 'NONE',  ( -9.999999999999998224, 1.224646799147353059E-15, -52.62500000409675494 ) ) ;
#34171=CARTESIAN_POINT ( 'NONE',  ( -9.999999999999998224, 1.224646799147353059E-15, -31.62500000409676559 ) ) ;
#34172=AXIS2_PLACEMENT_3D ( 'NONE', #42372, #40200, #40831 ) ;
#34173=DIRECTION ( 'NONE',  ( -0.000000000000000000, -0.000000000000000000, 1.000000000000000000 ) ) ;
#34175=EDGE_CURVE ( 'NONE', #18020, #17561, #12023, .T. ) ;
#34176=CARTESIAN_POINT ( 'NONE',  ( 9.999999999999998224, 0.000000000000000000, -39.87500000409676915 ) ) ;
#34177=CARTESIAN_POINT ( 'NONE',  ( -10.81189881249999729, 1.324075727343319199E-15, -155.2812500020484094 ) ) ;
#34178=CARTESIAN_POINT ( 'NONE',  ( -10.81189881249999729, 1.324075727343319199E-15, -126.5937500020483668 ) ) ;
#34179=CARTESIAN_POINT ( 'NONE',  ( 9.999999999999998224, 0.000000000000000000, -131.3750000040967905 ) ) ;
#34180=EDGE_LOOP ( 'NONE', ( #16525, #28981, #8224, #19458 ) ) ;
#34181=CARTESIAN_POINT ( 'NONE',  ( -10.00000000000102496, 5.773502691895664007, -31.37499999999992539 ) ) ;
#34182=ORIENTED_EDGE ( 'NONE', *, *, #36445, .F. ) ;
#34183=ORIENTED_EDGE ( 'NONE', *, *, #17359, .F. ) ;
#34184=CARTESIAN_POINT ( 'NONE',  ( -5.405949406250003975, -9.363379034771801557, -111.3437500020483810 ) ) ;
#34185=VERTEX_POINT ( 'NONE', #19691 ) ;
#34186=( BOUNDED_CURVE ( )  B_SPLINE_CURVE ( 2, ( #22595, #42218, #41590, #18715, #12022, #31908, #5778 ),
 .UNSPECIFIED., .F., .F. ) 
 B_SPLINE_CURVE_WITH_KNOTS ( ( 3, 2, 2, 3 ),
 ( 0.1305970149253731227, 0.1318407960199005080, 0.1330845771144278378, 0.1343283582089551953 ),
 .UNSPECIFIED. ) 
 CURVE ( )  GEOMETRIC_REPRESENTATION_ITEM ( )  RATIONAL_B_SPLINE_CURVE ( ( 1.000000000000000000, 0.8660254037844387076, 1.000000000000000000, 0.8660254037844387076, 1.000000000000000000, 0.8660254037844417052, 0.9999999999999970024 ) ) 
 REPRESENTATION_ITEM ( '' )  );
#34187=VECTOR ( 'NONE', #12141, 1000.000000000000000 ) ;
#34188=EDGE_CURVE ( 'NONE', #12174, #33849, #16222, .T. ) ;
#34189=CARTESIAN_POINT ( 'NONE',  ( -5.000000000000003553, -8.660254037844383745, -145.3750000040967905 ) ) ;
#34190=CARTESIAN_POINT ( 'NONE',  ( 5.405949406249992428, -9.363379034771808662, -186.0937500020483810 ) ) ;
#34191=CARTESIAN_POINT ( 'NONE',  ( 10.81189881249999551, -6.242252689847874514, -38.96875000204835970 ) ) ;
#34192=CARTESIAN_POINT ( 'NONE',  ( 5.325955911939489695, -9.231538742169870915, -4.316514933816155950E-15 ) ) ;
#34193=DIRECTION ( 'NONE',  ( -0.000000000000000000, -0.000000000000000000, 1.000000000000000000 ) ) ;
#34194=CARTESIAN_POINT ( 'NONE',  ( -10.81189881249999729, 1.324075727343319199E-15, -174.5937500020484094 ) ) ;
#34195=CARTESIAN_POINT ( 'NONE',  ( -5.405949406249996869, 9.363379034771805109, -164.3437500020484094 ) ) ;
#34196=CARTESIAN_POINT ( 'NONE',  ( 10.00000000000154010, -5.773502691895370020, -25.00000000409672651 ) ) ;
#34200=FACE_OUTER_BOUND ( 'NONE', #5355, .T. ) ;
#34201=CARTESIAN_POINT ( 'NONE',  ( -9.999999999999998224, 1.224646799147353059E-15, -88.24999999999998579 ) ) ;
#34203=CARTESIAN_POINT ( 'NONE',  ( 10.81189881249999551, -6.242252689847874514, -88.46875000204836681 ) ) ;
#34205=CARTESIAN_POINT ( 'NONE',  ( -10.81189881249999729, 6.242252689847871849, -62.40625000204838813 ) ) ;
#34208=CARTESIAN_POINT ( 'NONE',  ( -10.81189881249999907, -6.242252689847864744, -114.6562500020483952 ) ) ;
#34209=CARTESIAN_POINT ( 'NONE',  ( -2.293366432827344421E-15, -12.48450537969573659, -151.9062500020483810 ) ) ;
#34212=CARTESIAN_POINT ( 'NONE',  ( 10.00000000000000000, 5.773502691896255534, -126.7500000040967905 ) ) ;
#34214=ORIENTED_EDGE ( 'NONE', *, *, #20946, .T. ) ;
#34217=CARTESIAN_POINT ( 'NONE',  ( -9.183694056713489507E-15, -20.00000000000000355, 12.49999999999999112 ) ) ;
#34218=CARTESIAN_POINT ( 'NONE',  ( 7.644554776091147741E-16, 12.48450537969573659, -178.1562500020484094 ) ) ;
#34219=ORIENTED_EDGE ( 'NONE', *, *, #23075, .F. ) ;
#34220=CARTESIAN_POINT ( 'NONE',  ( 9.999999999999996447, -5.773502691896262640, -53.12499999999997868 ) ) ;
#34222=CARTESIAN_POINT ( 'NONE',  ( 9.999999999999998224, 0.000000000000000000, -57.87500000409676204 ) ) ;
#34223=DIRECTION ( 'NONE',  ( -0.000000000000000000, -0.000000000000000000, 1.000000000000000000 ) ) ;
#34224=CARTESIAN_POINT ( 'NONE',  ( -9.999999999999998224, 1.224646799147353059E-15, -200.0000000000000000 ) ) ;
#34226=CARTESIAN_POINT ( 'NONE',  ( 7.644554776091147741E-16, 12.48450537969573659, -53.65625000204838102 ) ) ;
#34229=CARTESIAN_POINT ( 'NONE',  ( -9.999999999999998224, 1.224646799147353059E-15, -2.749999999999974687 ) ) ;
#34230=CARTESIAN_POINT ( 'NONE',  ( -10.81189881249999907, -6.242252689847864744, -179.1562500020484094 ) ) ;
#34232=CARTESIAN_POINT ( 'NONE',  ( 9.999999999999998224, 0.000000000000000000, -199.4375000020484094 ) ) ;
#34235=( BOUNDED_CURVE ( )  B_SPLINE_CURVE ( 2, ( #13851, #14056, #3955, #36750, #19916, #27046, #4163 ),
 .UNSPECIFIED., .F., .F. ) 
 B_SPLINE_CURVE_WITH_KNOTS ( ( 3, 2, 2, 3 ),
 ( 0.6977611940298510396, 0.6990049751243784248, 0.7002487562189056991, 0.7014925373134330844 ),
 .UNSPECIFIED. ) 
 CURVE ( )  GEOMETRIC_REPRESENTATION_ITEM ( )  RATIONAL_B_SPLINE_CURVE ( ( 0.9999999999999641398, 0.8660254037844745678, 1.000000000000000000, 0.8660254037844387076, 1.000000000000000000, 0.8660254037844148378, 1.000000000000023981 ) ) 
 REPRESENTATION_ITEM ( '' )  );
#34236=CARTESIAN_POINT ( 'NONE',  ( -9.999999999999998224, 1.224646799147353059E-15, -39.12500000409676915 ) ) ;
#34238=CARTESIAN_POINT ( 'NONE',  ( -5.405949406249996869, 9.363379034771805109, -82.03125000204839523 ) ) ;
#34239=EDGE_LOOP ( 'NONE', ( #10636, #18764, #14774, #4601 ) ) ;
#34240=CARTESIAN_POINT ( 'NONE',  ( 0.000000000000000000, 5.321294541346989426, -220.0000000000000000 ) ) ;
#34243=CARTESIAN_POINT ( 'NONE',  ( -2.293366432827344421E-15, -12.48450537969573659, -36.21875000204835970 ) ) ;
#34244=CARTESIAN_POINT ( 'NONE',  ( 10.81189881249999907, 6.242252689847868297, -25.21875000204837036 ) ) ;
#34245=CARTESIAN_POINT ( 'NONE',  ( -10.81189881249999729, 1.324075727343319199E-15, -11.28125000204835438 ) ) ;
#34246=( BOUNDED_CURVE ( )  B_SPLINE_CURVE ( 2, ( #17485, #40572, #11015, #20951, #4345, #40789, #11230 ),
 .UNSPECIFIED., .F., .F. ) 
 B_SPLINE_CURVE_WITH_KNOTS ( ( 3, 2, 2, 3 ),
 ( 0.3246268656716419510, 0.3258706467661692807, 0.3271144278606965550, 0.3283582089552238847 ),
 .UNSPECIFIED. ) 
 CURVE ( )  GEOMETRIC_REPRESENTATION_ITEM ( )  RATIONAL_B_SPLINE_CURVE ( ( 0.9999999999999820144, 0.8660254037844566932, 1.000000000000000000, 0.8660254037844387076, 1.000000000000000000, 0.8660254037844387076, 1.000000000000000000 ) ) 
 REPRESENTATION_ITEM ( '' )  );
#34247=CARTESIAN_POINT ( 'NONE',  ( -2.293366432827344421E-15, -12.48450537969573659, -66.21875000204836681 ) ) ;
#34248=CARTESIAN_POINT ( 'NONE',  ( 9.999999999999998224, 0.000000000000000000, -93.49999999999998579 ) ) ;
#34250=CARTESIAN_POINT ( 'NONE',  ( 5.405949406249999534, 9.363379034771803333, -188.5937500020483810 ) ) ;
#34252=EDGE_CURVE ( 'NONE', #2342, #14232, #42350, .T. ) ;
#34254=CARTESIAN_POINT ( 'NONE',  ( -9.999999999999998224, 1.224646799147353059E-15, -200.0000000000000000 ) ) ;
#34255=CARTESIAN_POINT ( 'NONE',  ( 9.999999999999998224, 0.000000000000000000, -113.3750000040967763 ) ) ;
#34256=CARTESIAN_POINT ( 'NONE',  ( -9.999999999999479527, -5.773502691896549521, -90.00000000409674783 ) ) ;
#34257=CARTESIAN_POINT ( 'NONE',  ( 5.405949406249999534, 9.363379034771803333, -115.0937500020483810 ) ) ;
#34258=CYLINDRICAL_SURFACE ( 'NONE', #22498, 9.999999999999998224 ) ;
#34259=CARTESIAN_POINT ( 'NONE',  ( -10.81189881249999907, -6.242252689847864744, -78.65625000204839523 ) ) ;
#34260=CARTESIAN_POINT ( 'NONE',  ( 5.405949406249999534, 9.363379034771803333, -101.5937500020483810 ) ) ;
#34263=CARTESIAN_POINT ( 'NONE',  ( -9.999999999999998224, 1.224646799147353059E-15, -150.1250000040967905 ) ) ;
#34268=CARTESIAN_POINT ( 'NONE',  ( 9.999999999999998224, 0.000000000000000000, -173.0000000000000284 ) ) ;
#34270=CARTESIAN_POINT ( 'NONE',  ( -9.999999999999998224, 1.224646799147353059E-15, -25.24999999999996803 ) ) ;
#34271=CARTESIAN_POINT ( 'NONE',  ( 9.999999999999996447, -5.773502691896262640, -69.62499999999998579 ) ) ;
#34273=CARTESIAN_POINT ( 'NONE',  ( -2.121150477449813534E-15, -11.54700538379251284, -82.25000000409676204 ) ) ;
#34274=FACE_OUTER_BOUND ( 'NONE', #10113, .T. ) ;
#34276=CARTESIAN_POINT ( 'NONE',  ( -10.81189881249999729, -6.242252689847864744, -72.65625000204836681 ) ) ;
#34280=ORIENTED_EDGE ( 'NONE', *, *, #32791, .F. ) ;
#34281=CARTESIAN_POINT ( 'NONE',  ( 10.81189881249999907, 6.242252689847868297, -197.9062500020484379 ) ) ;
#34283=CARTESIAN_POINT ( 'NONE',  ( 7.644554776091147741E-16, 12.48450537969573659, -14.46875000204836859 ) ) ;
#34285=CARTESIAN_POINT ( 'NONE',  ( -10.81189881249999907, -6.242252689847864744, -126.6562500020483810 ) ) ;
#34286=EDGE_CURVE ( 'NONE', #41485, #22272, #3514, .T. ) ;
#34287=CARTESIAN_POINT ( 'NONE',  ( 5.000000000000000000, 8.660254037844385522, -178.7500000000000284 ) ) ;
#34288=CYLINDRICAL_SURFACE ( 'NONE', #12372, 9.999999999999998224 ) ;
#34289=CARTESIAN_POINT ( 'NONE',  ( 5.405949406249992428, -9.363379034771808662, -106.7812500020483810 ) ) ;
#34290=ORIENTED_EDGE ( 'NONE', *, *, #42385, .T. ) ;
#34292=VERTEX_POINT ( 'NONE', #22311 ) ;
#34293=ORIENTED_EDGE ( 'NONE', *, *, #40949, .F. ) ;
#34294=CARTESIAN_POINT ( 'NONE',  ( 10.81189881249999907, 6.242252689847868297, -37.40625000204836681 ) ) ;
#34296=CARTESIAN_POINT ( 'NONE',  ( -10.81189881249999907, -6.242252689847864744, -84.46875000204836681 ) ) ;
#34297=CARTESIAN_POINT ( 'NONE',  ( 9.999999999999998224, 0.000000000000000000, -69.87500000409677625 ) ) ;
#34299=CARTESIAN_POINT ( 'NONE',  ( 10.00000000000102318, -5.773502691895667560, -32.50000000409672651 ) ) ;
#34301=CARTESIAN_POINT ( 'NONE',  ( -9.999999999998969713, -5.773502691896847949, -68.62499999999995737 ) ) ;
#34303=CARTESIAN_POINT ( 'NONE',  ( -5.405949406249996869, 9.363379034771805109, -123.8437500020483952 ) ) ;
#34304=( BOUNDED_CURVE ( )  B_SPLINE_CURVE ( 2, ( #31784, #35438, #25305, #18161, #35017, #2215, #5446 ),
 .UNSPECIFIED., .F., .F. ) 
 B_SPLINE_CURVE_WITH_KNOTS ( ( 3, 2, 2, 3 ),
 ( 0.1455223880597014963, 0.1467661691542288538, 0.1480099502487562391, 0.1492537313432835966 ),
 .UNSPECIFIED. ) 
 CURVE ( )  GEOMETRIC_REPRESENTATION_ITEM ( )  RATIONAL_B_SPLINE_CURVE ( ( 1.000000000000000000, 0.8660254037844387076, 1.000000000000000000, 0.8660254037844387076, 1.000000000000000000, 0.8660254037844357100, 1.000000000000003109 ) ) 
 REPRESENTATION_ITEM ( '' )  );
#34306=CARTESIAN_POINT ( 'NONE',  ( 10.70731569305672615, 1.500182182589836044, 0.000000000000000000 ) ) ;
#34309=CARTESIAN_POINT ( 'NONE',  ( 5.000000000000000000, 8.660254037844385522, -177.6250000040968189 ) ) ;
#34311=CARTESIAN_POINT ( 'NONE',  ( -10.81189881249999729, 1.324075727343319199E-15, -174.7812500020484094 ) ) ;
#34312=CARTESIAN_POINT ( 'NONE',  ( 4.999999999999992006, -8.660254037844389075, -28.12500000409676204 ) ) ;
#34313=CARTESIAN_POINT ( 'NONE',  ( -4.999999999999996447, 8.660254037844387298, -181.5000000000000000 ) ) ;
#34315=CARTESIAN_POINT ( 'NONE',  ( -10.81189881249999729, 1.324075727343319199E-15, -54.59375000204835970 ) ) ;
#34317=CARTESIAN_POINT ( 'NONE',  ( 5.405949406249999534, 9.363379034771803333, -10.28125000204835260 ) ) ;
#34321=CARTESIAN_POINT ( 'NONE',  ( 9.999999999999996447, -5.773502691896262640, -98.12499999999998579 ) ) ;
#34323=CARTESIAN_POINT ( 'NONE',  ( 5.000000000000000000, 8.660254037844385522, -104.1250000040967763 ) ) ;
#34326=CARTESIAN_POINT ( 'NONE',  ( -5.405949406249996869, 9.363379034771805109, -97.03125000204839523 ) ) ;
#34329=CARTESIAN_POINT ( 'NONE',  ( -4.999999999999996447, 8.660254037844387298, -141.3750000040967905 ) ) ;
#34330=CARTESIAN_POINT ( 'NONE',  ( -10.81189881249999729, 1.324075727343319199E-15, -167.2812500020484094 ) ) ;
#34332=ORIENTED_EDGE ( 'NONE', *, *, #17831, .T. ) ;
#34333=CARTESIAN_POINT ( 'NONE',  ( 10.00000000000000000, 5.773502691896255534, -22.87499999999997868 ) ) ;
#34334=CARTESIAN_POINT ( 'NONE',  ( 10.81189881249999729, 0.000000000000000000, -39.03125000204838102 ) ) ;
#34335=CARTESIAN_POINT ( 'NONE',  ( 4.999999999999992006, -8.660254037844389075, -161.2500000000000000 ) ) ;
#34336=AXIS2_PLACEMENT_3D ( 'NONE', #31493, #7752, #27817 ) ;
#34337=LINE ( 'NONE', #14225, #22152 ) ;
#34339=CARTESIAN_POINT ( 'NONE',  ( -9.999999999999998224, 1.224646799147353059E-15, -23.74999999999996447 ) ) ;
#34340=CARTESIAN_POINT ( 'NONE',  ( 5.405949406249999534, 9.363379034771803333, -130.2812500020483810 ) ) ;
#34341=CARTESIAN_POINT ( 'NONE',  ( 5.000000000000000000, 8.660254037844385522, -111.2499999999999858 ) ) ;
#34343=ORIENTED_EDGE ( 'NONE', *, *, #9091, .F. ) ;
#34344=CARTESIAN_POINT ( 'NONE',  ( -10.81189881249999729, 1.324075727343319199E-15, -59.28125000204836681 ) ) ;
#34347=CYLINDRICAL_SURFACE ( 'NONE', #34597, 9.999999999999998224 ) ;
#34349=CARTESIAN_POINT ( 'NONE',  ( -5.405949406250003975, -9.363379034771801557, -162.3437500020484094 ) ) ;
#34351=CARTESIAN_POINT ( 'NONE',  ( -5.405949406250003975, -9.363379034771801557, -12.34375000204834905 ) ) ;
#34352=CARTESIAN_POINT ( 'NONE',  ( -10.00000000000051337, 5.773502691895962435, -49.37499999999996447 ) ) ;
#34353=EDGE_CURVE ( 'NONE', #26059, #37408, #33309, .T. ) ;
#34354=CARTESIAN_POINT ( 'NONE',  ( -10.81189881249999729, 1.324075727343319199E-15, -147.5937500020483810 ) ) ;
#34356=CARTESIAN_POINT ( 'NONE',  ( -5.405949406250003975, -9.363379034771801557, -129.3437500020484094 ) ) ;
#34357=EDGE_CURVE ( 'NONE', #25200, #35567, #3943, .T. ) ;
#34358=CARTESIAN_POINT ( 'NONE',  ( 10.81189881249999729, 0.000000000000000000, -108.0312500020483810 ) ) ;
#34362=CARTESIAN_POINT ( 'NONE',  ( -5.405949406249996869, 9.363379034771805109, -0.8437500020483656993 ) ) ;
#34368=CARTESIAN_POINT ( 'NONE',  ( -5.405949406249996869, 9.363379034771805109, -77.34375000204838102 ) ) ;
#34369=CARTESIAN_POINT ( 'NONE',  ( 7.644554776091147741E-16, 12.48450537969573659, -63.96875000204837391 ) ) ;
#34371=CARTESIAN_POINT ( 'NONE',  ( -10.81189881249999729, 1.324075727343319199E-15, -32.28125000204837391 ) ) ;
#34373=CARTESIAN_POINT ( 'NONE',  ( -9.999999999999998224, 1.224646799147353059E-15, -31.62500000409676559 ) ) ;
#34375=CARTESIAN_POINT ( 'NONE',  ( 4.999999999999992006, -8.660254037844389075, -122.2500000000000000 ) ) ;
#34376=CARTESIAN_POINT ( 'NONE',  ( 10.81189881249999729, 0.000000000000000000, -130.5312500020484094 ) ) ;
#34379=CARTESIAN_POINT ( 'NONE',  ( 7.644554776091147741E-16, 12.48450537969573659, -16.15625000204837747 ) ) ;
#34383=CARTESIAN_POINT ( 'NONE',  ( 10.00000000000038014, -5.773502691896040595, -179.5000000040967620 ) ) ;
#34384=CARTESIAN_POINT ( 'NONE',  ( 9.999999999999996447, -5.773502691896262640, -35.50000000409675494 ) ) ;
#34385=CARTESIAN_POINT ( 'NONE',  ( -4.999999999999996447, 8.660254037844387298, -74.99999999999998579 ) ) ;
#34387=CARTESIAN_POINT ( 'NONE',  ( 10.00000000000021672, -5.773502691896130301, -191.1249999999999716 ) ) ;
#34388=CARTESIAN_POINT ( 'NONE',  ( 5.405949406249992428, -9.363379034771808662, -156.2812500020484094 ) ) ;
#34389=CARTESIAN_POINT ( 'NONE',  ( -5.405949406250003975, -9.363379034771801557, -127.8437500020483952 ) ) ;
#34390=CARTESIAN_POINT ( 'NONE',  ( -9.999999999999998224, 1.224646799147353059E-15, -8.749999999999952038 ) ) ;
#34391=ADVANCED_FACE ( 'NONE', ( #14257 ), #719, .T. ) ;
#34393=CARTESIAN_POINT ( 'NONE',  ( 10.40594940624999865, 0.000000000000000000, -199.1093750030726142 ) ) ;
#34394=ORIENTED_EDGE ( 'NONE', *, *, #6160, .F. ) ;
#34395=ORIENTED_EDGE ( 'NONE', *, *, #40441, .F. ) ;
#34396=ORIENTED_EDGE ( 'NONE', *, *, #14409, .F. ) ;
#34397=CARTESIAN_POINT ( 'NONE',  ( -10.00000000000022027, 5.773502691896128525, -188.8750000000000284 ) ) ;
#34398=CARTESIAN_POINT ( 'NONE',  ( -5.405949406250003975, -9.363379034771801557, -193.8437500020484094 ) ) ;
#34399=CARTESIAN_POINT ( 'NONE',  ( -10.81189881249999729, 1.324075727343319199E-15, -39.59375000204837391 ) ) ;
#34400=CARTESIAN_POINT ( 'NONE',  ( 1.250775920587201551, -10.41851302423964221, 8.157905031340290035E-16 ) ) ;
#34401=CARTESIAN_POINT ( 'NONE',  ( 9.999999999999998224, 0.000000000000000000, -14.37500000409674961 ) ) ;
#34402=EDGE_CURVE ( 'NONE', #6396, #21320, #16667, .T. ) ;
#34403=CARTESIAN_POINT ( 'NONE',  ( 5.405949406249992428, -9.363379034771808662, -175.5937500020484094 ) ) ;
#34404=CARTESIAN_POINT ( 'NONE',  ( -10.81189881249999729, 6.242252689847871849, -158.2187500020483810 ) ) ;
#34410=DIRECTION ( 'NONE',  ( -0.000000000000000000, -0.000000000000000000, 1.000000000000000000 ) ) ;
#34414=CARTESIAN_POINT ( 'NONE',  ( 5.405949406249999534, 9.363379034771803333, -86.59375000204836681 ) ) ;
#34415=CARTESIAN_POINT ( 'NONE',  ( -4.999999999999996447, 8.660254037844387298, -198.3750000040967905 ) ) ;
#34416=CARTESIAN_POINT ( 'NONE',  ( -10.81189881249999729, 6.242252689847871849, -60.90625000204837391 ) ) ;
#34417=CARTESIAN_POINT ( 'NONE',  ( -9.999999999998456346, -5.773502691897145489, -16.50000000409671941 ) ) ;
#34419=CARTESIAN_POINT ( 'NONE',  ( -10.81189881249999729, 1.324075727343319199E-15, -113.2812500020483952 ) ) ;
#34420=CARTESIAN_POINT ( 'NONE',  ( 10.81189881249999551, -6.242252689847874514, -153.1562500020484094 ) ) ;
#34423=CARTESIAN_POINT ( 'NONE',  ( -9.999999999999998224, 1.224646799147353059E-15, -133.6250000040967620 ) ) ;
#34425=EDGE_LOOP ( 'NONE', ( #21491, #22290, #38291, #12902 ) ) ;
#34428=LINE ( 'NONE', #34217, #7715 ) ;
#34429=VECTOR ( 'NONE', #4243, 1000.000000000000000 ) ;
#34430=CARTESIAN_POINT ( 'NONE',  ( 10.81189881249999551, -6.242252689847874514, -183.1562500020484094 ) ) ;
#34431=VERTEX_POINT ( 'NONE', #27032 ) ;
#34433=CARTESIAN_POINT ( 'NONE',  ( 4.999999999999992006, -8.660254037844389075, -55.12500000409675494 ) ) ;
#34435=CARTESIAN_POINT ( 'NONE',  ( -10.00000000000076916, 5.773502691895813221, -130.3750000000000000 ) ) ;
#34437=CARTESIAN_POINT ( 'NONE',  ( 10.81189881249999551, -6.242252689847874514, -49.65625000204837391 ) ) ;
#34438=EDGE_CURVE ( 'NONE', #7438, #6420, #10608, .T. ) ;
#34442=CARTESIAN_POINT ( 'NONE',  ( -9.999999999999998224, 1.224646799147353059E-15, -200.0000000000000000 ) ) ;
#34443=CARTESIAN_POINT ( 'NONE',  ( -5.405949406249996869, 9.363379034771805109, -176.5312500020483810 ) ) ;
#34444=DIRECTION ( 'NONE',  ( -0.000000000000000000, -0.000000000000000000, 1.000000000000000000 ) ) ;
#34445=PLANE ( 'NONE',  #31695 ) ;
#34446=ORIENTED_EDGE ( 'NONE', *, *, #15885, .F. ) ;
#34447=CARTESIAN_POINT ( 'NONE',  ( 4.999999999999992006, -8.660254037844389075, -0.7499999999999729106 ) ) ;
#34450=CARTESIAN_POINT ( 'NONE',  ( 10.81189881249999551, -6.242252689847874514, -87.15625000204838102 ) ) ;
#34452=LINE ( 'NONE', #21482, #32396 ) ;
#34453=EDGE_LOOP ( 'NONE', ( #6084, #4704, #10427, #7091 ) ) ;
#34455=CARTESIAN_POINT ( 'NONE',  ( 7.644554776091147741E-16, 12.48450537969573659, -35.46875000204835260 ) ) ;
#34456=CARTESIAN_POINT ( 'NONE',  ( 10.81189881249999729, 0.000000000000000000, -29.84375000204836326 ) ) ;
#34457=CARTESIAN_POINT ( 'NONE',  ( -10.81189881249999729, 6.242252689847871849, -17.40625000204838457 ) ) ;
#34459=CARTESIAN_POINT ( 'NONE',  ( 10.81189881249999729, 0.000000000000000000, -62.84375000204836681 ) ) ;
#34462=CARTESIAN_POINT ( 'NONE',  ( 5.405949406249999534, 9.363379034771803333, -184.0937500020483810 ) ) ;
#34465=CARTESIAN_POINT ( 'NONE',  ( 9.999999999998969713, 5.773502691896851502, -59.25000000409674783 ) ) ;
#34466=CARTESIAN_POINT ( 'NONE',  ( 9.999999999999998224, 0.000000000000000000, -71.37500000409677625 ) ) ;
#34467=CARTESIAN_POINT ( 'NONE',  ( -9.999999999999998224, 1.224646799147353059E-15, -104.7499999999999858 ) ) ;
#34468=CARTESIAN_POINT ( 'NONE',  ( 9.999999999998969713, 5.773502691896851502, -60.75000000409676204 ) ) ;
#34469=CARTESIAN_POINT ( 'NONE',  ( 5.405949406249992428, -9.363379034771808662, -114.0937500020483810 ) ) ;
#34471=CARTESIAN_POINT ( 'NONE',  ( -10.81189881249999729, 1.324075727343319199E-15, -84.78125000204838102 ) ) ;
#34472=CARTESIAN_POINT ( 'NONE',  ( 10.81189881249999551, -6.242252689847874514, -91.46875000204838102 ) ) ;
#34475=CARTESIAN_POINT ( 'NONE',  ( -10.00000000000000000, -5.773502691896251982, -157.5000000040968189 ) ) ;
#34477=( BOUNDED_CURVE ( )  B_SPLINE_CURVE ( 2, ( #17907, #38204, #34341, #28077, #14450, #8649, #1103 ),
 .UNSPECIFIED., .F., .F. ) 
 B_SPLINE_CURVE_WITH_KNOTS ( ( 3, 2, 2, 3 ),
 ( 0.4402985074626867279, 0.4415422885572141132, 0.4427860696517414429, 0.4440298507462688282 ),
 .UNSPECIFIED. ) 
 CURVE ( )  GEOMETRIC_REPRESENTATION_ITEM ( )  RATIONAL_B_SPLINE_CURVE ( ( 0.9999999999999820144, 0.8660254037844566932, 1.000000000000000000, 0.8660254037844387076, 1.000000000000000000, 0.8660254037844207220, 1.000000000000017986 ) ) 
 REPRESENTATION_ITEM ( '' )  );
#34480=ADVANCED_FACE ( 'NONE', ( #40176 ), #33728, .T. ) ;
#34481=DIRECTION ( 'NONE',  ( 1.000000000000000000, 0.000000000000000000, 0.000000000000000000 ) ) ;
#34484=CARTESIAN_POINT ( 'NONE',  ( -4.999999999999996447, 8.660254037844387298, -10.49999999999995381 ) ) ;
#34485=CARTESIAN_POINT ( 'NONE',  ( 9.999999999999998224, 0.000000000000000000, -73.99999999999998579 ) ) ;
#34487=CARTESIAN_POINT ( 'NONE',  ( 9.999999999999996447, -5.773502691896262640, -79.00000000409677625 ) ) ;
#34490=CARTESIAN_POINT ( 'NONE',  ( -5.405949406249996869, 9.363379034771805109, -79.03125000204838102 ) ) ;
#34491=( BOUNDED_CURVE ( )  B_SPLINE_CURVE ( 2, ( #17566, #39819, #775, #567, #24078, #7033, #40236 ),
 .UNSPECIFIED., .F., .F. ) 
 B_SPLINE_CURVE_WITH_KNOTS ( ( 3, 2, 2, 3 ),
 ( 0.09701492537313441411, 0.09825870646766173000, 0.09950248756218905977, 0.1007462686567163757 ),
 .UNSPECIFIED. ) 
 CURVE ( )  GEOMETRIC_REPRESENTATION_ITEM ( )  RATIONAL_B_SPLINE_CURVE ( ( 0.9999999999999910072, 0.8660254037844477004, 1.000000000000000000, 0.8660254037844387076, 1.000000000000000000, 0.8660254037844431485, 0.9999999999999955591 ) ) 
 REPRESENTATION_ITEM ( '' )  );
#34494=ORIENTED_EDGE ( 'NONE', *, *, #35036, .F. ) ;
#34495=CARTESIAN_POINT ( 'NONE',  ( 9.999999999999996447, -5.773502691896262640, -3.624999999999953371 ) ) ;
#34496=VECTOR ( 'NONE', #35770, 1000.000000000000000 ) ;
#34498=CARTESIAN_POINT ( 'NONE',  ( 5.405949406249999534, 9.363379034771803333, -14.59375000204835082 ) ) ;
#34499=CARTESIAN_POINT ( 'NONE',  ( -2.121150477449813534E-15, -11.54700538379251284, -64.25000000409677625 ) ) ;
#34502=CARTESIAN_POINT ( 'NONE',  ( -10.81189881249999729, 6.242252689847871849, -129.9062500020483810 ) ) ;
#34503=( BOUNDED_CURVE ( )  B_SPLINE_CURVE ( 2, ( #29530, #13314, #42672, #26297, #39446, #36211, #26503 ),
 .UNSPECIFIED., .F., .F. ) 
 B_SPLINE_CURVE_WITH_KNOTS ( ( 3, 2, 2, 3 ),
 ( 0.2126865671641791633, 0.2139303482587065208, 0.2151741293532339061, 0.2164179104477612636 ),
 .UNSPECIFIED. ) 
 CURVE ( )  GEOMETRIC_REPRESENTATION_ITEM ( )  RATIONAL_B_SPLINE_CURVE ( ( 0.9999999999999940048, 0.8660254037844447028, 1.000000000000000000, 0.8660254037844387076, 1.000000000000000000, 0.8660254037844297148, 1.000000000000008882 ) ) 
 REPRESENTATION_ITEM ( '' )  );
#34504=CARTESIAN_POINT ( 'NONE',  ( -4.999999999999996447, 8.660254037844387298, -186.0000000000000000 ) ) ;
#34505=CARTESIAN_POINT ( 'NONE',  ( 9.999999999999998224, 0.000000000000000000, -125.0000000000000000 ) ) ;
#34506=CARTESIAN_POINT ( 'NONE',  ( 5.405949406249999534, 9.363379034771803333, -106.2812500020483810 ) ) ;
#34507=VERTEX_POINT ( 'NONE', #10822 ) ;
#34509=ORIENTED_EDGE ( 'NONE', *, *, #31909, .T. ) ;
#34510=ORIENTED_EDGE ( 'NONE', *, *, #25926, .T. ) ;
#34511=CARTESIAN_POINT ( 'NONE',  ( 5.405949406249999534, 9.363379034771803333, -41.78125000204838102 ) ) ;
#34513=CARTESIAN_POINT ( 'NONE',  ( 10.81189881249999551, -6.242252689847874514, -88.46875000204836681 ) ) ;
#34514=CARTESIAN_POINT ( 'NONE',  ( 9.999999999999998224, 0.000000000000000000, -128.3750000040967905 ) ) ;
#34518=CARTESIAN_POINT ( 'NONE',  ( 7.070501591499376803E-16, 11.54700538379251284, -54.50000000409677625 ) ) ;
#34519=AXIS2_PLACEMENT_3D ( 'NONE', #39345, #36332, #6763 ) ;
#34520=CARTESIAN_POINT ( 'NONE',  ( 10.81189881249999729, 0.000000000000000000, -121.3437500020483952 ) ) ;
#34522=CARTESIAN_POINT ( 'NONE',  ( -10.81189881249999729, 6.242252689847871849, -5.406250002048357928 ) ) ;
#34525=CARTESIAN_POINT ( 'NONE',  ( 7.070501591499377789E-16, 11.54700538379251284, -177.5000000040967905 ) ) ;
#34526=CARTESIAN_POINT ( 'NONE',  ( 10.81189881249999729, 0.000000000000000000, -169.5312500020484094 ) ) ;
#34529=CARTESIAN_POINT ( 'NONE',  ( 5.405949406249992428, -9.363379034771808662, -55.59375000204835970 ) ) ;
#34531=CARTESIAN_POINT ( 'NONE',  ( -5.405949406249996869, 9.363379034771805109, -11.53125000204835438 ) ) ;
#34533=FACE_OUTER_BOUND ( 'NONE', #3387, .T. ) ;
#34535=CARTESIAN_POINT ( 'NONE',  ( -9.999999999999998224, 5.773502691896259087, -97.37500000000000000 ) ) ;
#34537=CARTESIAN_POINT ( 'NONE',  ( 7.070501591499377789E-16, 11.54700538379251284, -104.0000000040967763 ) ) ;
#34540=CARTESIAN_POINT ( 'NONE',  ( 10.81189881249999729, 6.242252689847867408, -103.4062500020483952 ) ) ;
#34543=CARTESIAN_POINT ( 'NONE',  ( -9.999999999999998224, 1.224646799147353059E-15, -163.6250000040967905 ) ) ;
#34544=CARTESIAN_POINT ( 'NONE',  ( 5.405949406249999534, 9.363379034771803333, -163.2812500020484094 ) ) ;
#34547=CARTESIAN_POINT ( 'NONE',  ( -10.00000000000000000, -5.773502691896251982, -23.62499999999998224 ) ) ;
#34548=CARTESIAN_POINT ( 'NONE',  ( 10.81189881249999729, 0.000000000000000000, -27.03125000204836681 ) ) ;
#34549=CARTESIAN_POINT ( 'NONE',  ( -4.999999999999996447, 8.660254037844387298, -162.0000000000000000 ) ) ;
#34550=CARTESIAN_POINT ( 'NONE',  ( -9.999999999999998224, 1.224646799147353059E-15, -25.62500000409675849 ) ) ;
#34554=CARTESIAN_POINT ( 'NONE',  ( 5.405949406249992428, -9.363379034771808662, -133.7812500020483810 ) ) ;
#34557=CARTESIAN_POINT ( 'NONE',  ( -10.81189881249999729, 6.242252689847871849, -60.90625000204837391 ) ) ;
#34560=ORIENTED_EDGE ( 'NONE', *, *, #32743, .T. ) ;
#34561=( BOUNDED_CURVE ( )  B_SPLINE_CURVE ( 2, ( #10133, #6066, #32193, #15752, #32614, #2620, #3039 ),
 .UNSPECIFIED., .F., .F. ) 
 B_SPLINE_CURVE_WITH_KNOTS ( ( 3, 2, 2, 3 ),
 ( 0.2462686567164180107, 0.2475124378109453960, 0.2487562189054727535, 0.2500000000000001110 ),
 .UNSPECIFIED. ) 
 CURVE ( )  GEOMETRIC_REPRESENTATION_ITEM ( )  RATIONAL_B_SPLINE_CURVE ( ( 0.9999999999999880096, 0.8660254037844506980, 1.000000000000000000, 0.8660254037844387076, 1.000000000000000000, 0.8660254037844267172, 1.000000000000011990 ) ) 
 REPRESENTATION_ITEM ( '' )  );
#34562=CARTESIAN_POINT ( 'NONE',  ( 9.999999999999676703, 5.773502691896441164, -182.2500000040967620 ) ) ;
#34564=CARTESIAN_POINT ( 'NONE',  ( 10.81189881249999729, 0.000000000000000000, -160.3437500020484094 ) ) ;
#34566=CARTESIAN_POINT ( 'NONE',  ( -5.405949406249996869, 9.363379034771805109, -11.34375000204834727 ) ) ;
#34567=DIRECTION ( 'NONE',  ( 1.000000000000000000, 0.000000000000000000, 0.000000000000000000 ) ) ;
#34568=CARTESIAN_POINT ( 'NONE',  ( 10.81189881249999729, 6.242252689847867408, -149.7187500020483810 ) ) ;
#34569=CARTESIAN_POINT ( 'NONE',  ( -10.81189881249999907, -6.242252689847864744, -105.6562500020483952 ) ) ;
#34571=CARTESIAN_POINT ( 'NONE',  ( -9.999999999999742428, -5.773502691896402084, -161.6250000000000284 ) ) ;
#34573=CARTESIAN_POINT ( 'NONE',  ( 10.81189881249999729, 0.000000000000000000, -5.843750002048370362 ) ) ;
#34576=CARTESIAN_POINT ( 'NONE',  ( -5.405949406249996869, 9.363379034771805109, -191.5312500020484094 ) ) ;
#34577=CARTESIAN_POINT ( 'NONE',  ( 10.00000000000000000, 5.773502691896255534, -165.7500000040967905 ) ) ;
#34581=CARTESIAN_POINT ( 'NONE',  ( 10.81189881249999729, 6.242252689847867408, -74.71875000204838102 ) ) ;
#34582=CARTESIAN_POINT ( 'NONE',  ( 5.405949406249999534, 9.363379034771803333, -56.59375000204835970 ) ) ;
#34583=CARTESIAN_POINT ( 'NONE',  ( 4.999999999999992006, -8.660254037844389075, -116.6250000040967905 ) ) ;
#34584=CARTESIAN_POINT ( 'NONE',  ( 5.405949406249999534, 9.363379034771803333, -34.28125000204837391 ) ) ;
#34586=CARTESIAN_POINT ( 'NONE',  ( 7.070501591499376803E-16, 11.54700538379251284, -53.00000000409676915 ) ) ;
#34588=CARTESIAN_POINT ( 'NONE',  ( 9.999999999999996447, -5.773502691896262640, -125.1249999999999858 ) ) ;
#34589=CARTESIAN_POINT ( 'NONE',  ( 5.000000000000000000, 8.660254037844385522, -42.24999999999997868 ) ) ;
#34591=CARTESIAN_POINT ( 'NONE',  ( 7.644554776091147741E-16, 12.48450537969573659, -7.156250002048365921 ) ) ;
#34597=AXIS2_PLACEMENT_3D ( 'NONE', #27436, #40999, #31111 ) ;
#34598=CARTESIAN_POINT ( 'NONE',  ( -5.000000000000003553, -8.660254037844383745, -31.37500000409676559 ) ) ;
#34601=CARTESIAN_POINT ( 'NONE',  ( -9.999999999999479527, -5.773502691896549521, -100.1249999999999574 ) ) ;
#34602=CARTESIAN_POINT ( 'NONE',  ( -2.293366432827344421E-15, -12.48450537969573659, -147.4062500020483810 ) ) ;
#34603=CARTESIAN_POINT ( 'NONE',  ( -2.293366432827344421E-15, -12.48450537969573659, -129.2187500020483810 ) ) ;
#34604=CARTESIAN_POINT ( 'NONE',  ( -10.00000000000051337, 5.773502691895962435, -151.3750000000000284 ) ) ;
#34605=EDGE_CURVE ( 'NONE', #18513, #27003, #29938, .T. ) ;
#34606=EDGE_CURVE ( 'NONE', #8915, #21961, #16411, .T. ) ;
#34608=ORIENTED_EDGE ( 'NONE', *, *, #3429, .F. ) ;
#34609=AXIS2_PLACEMENT_3D ( 'NONE', #29357, #26119, #12713 ) ;
#34611=EDGE_LOOP ( 'NONE', ( #19987, #11271, #12339, #22740 ) ) ;
#34612=ORIENTED_EDGE ( 'NONE', *, *, #10841, .F. ) ;
#34613=CARTESIAN_POINT ( 'NONE',  ( -4.999999999999996447, 8.660254037844387298, -129.3750000040967905 ) ) ;
#34614=CARTESIAN_POINT ( 'NONE',  ( 7.644554776091147741E-16, 12.48450537969573659, -183.9687500020484094 ) ) ;
#34615=CARTESIAN_POINT ( 'NONE',  ( 10.81189881249999551, -6.242252689847874514, -35.96875000204835260 ) ) ;
#34616=CARTESIAN_POINT ( 'NONE',  ( -10.00000000000025580, 5.773502691896109873, -118.3750000000000142 ) ) ;
#34617=CARTESIAN_POINT ( 'NONE',  ( 7.644554776091147741E-16, 12.48450537969573659, -168.9687500020483810 ) ) ;
#34618=CARTESIAN_POINT ( 'NONE',  ( 5.405949406249992428, -9.363379034771808662, -153.0937500020483810 ) ) ;
#34622=CARTESIAN_POINT ( 'NONE',  ( -9.999999999999998224, 1.224646799147353059E-15, -40.62500000409677625 ) ) ;
#34623=DIRECTION ( 'NONE',  ( 1.000000000000000000, 0.000000000000000000, 0.000000000000000000 ) ) ;
#34625=CARTESIAN_POINT ( 'NONE',  ( 10.81189881249999551, -6.242252689847874514, -79.46875000204838102 ) ) ;
#34627=CARTESIAN_POINT ( 'NONE',  ( -5.405949406250003975, -9.363379034771801557, -59.03125000204836681 ) ) ;
#34630=CARTESIAN_POINT ( 'NONE',  ( -5.405949406250003975, -9.363379034771801557, -113.0312500020483952 ) ) ;
#34631=CARTESIAN_POINT ( 'NONE',  ( 5.405949406249992428, -9.363379034771808662, -154.7812500020484094 ) ) ;
#34634=CARTESIAN_POINT ( 'NONE',  ( -9.999999999999998224, 1.224646799147353059E-15, -126.1250000040967620 ) ) ;
#34636=VECTOR ( 'NONE', #18671, 1000.000000000000114 ) ;
#34637=VERTEX_POINT ( 'NONE', #2211 ) ;
#34641=CARTESIAN_POINT ( 'NONE',  ( 5.405949406249992428, -9.363379034771808662, -183.2812500020484094 ) ) ;
#34642=ORIENTED_EDGE ( 'NONE', *, *, #30488, .T. ) ;
#34644=CARTESIAN_POINT ( 'NONE',  ( 9.999999999999998224, 0.000000000000000000, -59.37500000409676204 ) ) ;
#34645=CARTESIAN_POINT ( 'NONE',  ( -9.999999999999998224, 1.224646799147353059E-15, -187.2500000000000000 ) ) ;
#34646=CARTESIAN_POINT ( 'NONE',  ( 9.999999999999998224, 0.000000000000000000, -117.5000000000000000 ) ) ;
#34650=CARTESIAN_POINT ( 'NONE',  ( 4.999999999999992006, -8.660254037844389075, -148.1250000040967905 ) ) ;
#34651=CARTESIAN_POINT ( 'NONE',  ( -10.81189881249999907, -6.242252689847864744, -174.6562500020483810 ) ) ;
#34653=CARTESIAN_POINT ( 'NONE',  ( 5.000000000000000000, 8.660254037844385522, -2.125000004096766482 ) ) ;
#34655=ORIENTED_EDGE ( 'NONE', *, *, #21492, .T. ) ;
#34657=EDGE_CURVE ( 'NONE', #8341, #17742, #10874, .T. ) ;
#34659=CARTESIAN_POINT ( 'NONE',  ( -9.999999999999998224, 1.224646799147353059E-15, -61.24999999999997158 ) ) ;
#34660=EDGE_CURVE ( 'NONE', #39053, #30365, #5102, .T. ) ;
#34661=DIRECTION ( 'NONE',  ( -1.000000000000000000, 0.000000000000000000, 0.000000000000000000 ) ) ;
#34662=CARTESIAN_POINT ( 'NONE',  ( -2.293366432827344421E-15, -12.48450537969573659, -81.40625000204838102 ) ) ;
#34663=ORIENTED_EDGE ( 'NONE', *, *, #34676, .T. ) ;
#34664=( NAMED_UNIT ( * ) PLANE_ANGLE_UNIT ( ) SI_UNIT ( $, .RADIAN. ) );
#34666=EDGE_LOOP ( 'NONE', ( #40103, #11973, #19958, #20147 ) ) ;
#34669=CARTESIAN_POINT ( 'NONE',  ( -5.405949406249996869, 9.363379034771805109, -36.84375000204836681 ) ) ;
#34670=CARTESIAN_POINT ( 'NONE',  ( 5.000000000000000000, 8.660254037844385522, -77.12500000409677625 ) ) ;
#34671=CARTESIAN_POINT ( 'NONE',  ( -2.293366432827344421E-15, -12.48450537969573659, -10.90625000204838457 ) ) ;
#34672=CARTESIAN_POINT ( 'NONE',  ( 5.405949406249999534, 9.363379034771803333, -59.59375000204835970 ) ) ;
#34676=EDGE_CURVE ( 'NONE', #38192, #28563, #4594, .T. ) ;
#34677=CARTESIAN_POINT ( 'NONE',  ( -5.405949406250003975, -9.363379034771801557, -192.3437500020484094 ) ) ;
#34678=CARTESIAN_POINT ( 'NONE',  ( 7.644554776091147741E-16, 12.48450537969573659, -173.4687500020483810 ) ) ;
#34680=DIRECTION ( 'NONE',  ( -0.000000000000000000, -0.000000000000000000, 1.000000000000000000 ) ) ;
#34681=CARTESIAN_POINT ( 'NONE',  ( -4.999999999999996447, 8.660254037844387298, -58.87500000409676204 ) ) ;
#34683=EDGE_CURVE ( 'NONE', #3609, #33095, #38752, .T. ) ;
#34685=CARTESIAN_POINT ( 'NONE',  ( -10.81189881249999729, 1.324075727343319199E-15, -114.5937500020483810 ) ) ;
#34687=CARTESIAN_POINT ( 'NONE',  ( 10.81189881249999551, -6.242252689847874514, -81.15625000204839523 ) ) ;
#34688=CARTESIAN_POINT ( 'NONE',  ( -10.81189881249999729, 1.324075727343319199E-15, -92.09375000204838102 ) ) ;
#34691=CARTESIAN_POINT ( 'NONE',  ( -5.000000000000003553, -8.660254037844383745, -154.3750000040967905 ) ) ;
#34695=LINE ( 'NONE', #28215, #8234 ) ;
#34696=CARTESIAN_POINT ( 'NONE',  ( 10.00000000000044764, -5.773502691896004180, -182.1250000000000000 ) ) ;
#34698=VERTEX_POINT ( 'NONE', #31566 ) ;
#34699=CARTESIAN_POINT ( 'NONE',  ( -9.999999999999998224, 1.224646799147353059E-15, -62.74999999999997158 ) ) ;
#34701=CARTESIAN_POINT ( 'NONE',  ( -5.000000000000003553, -8.660254037844383745, -83.87500000409677625 ) ) ;
#34703=CARTESIAN_POINT ( 'NONE',  ( 10.00000000000051159, -5.773502691895965988, -142.0000000040967905 ) ) ;
#34705=CARTESIAN_POINT ( 'NONE',  ( 10.81189881249999729, 0.000000000000000000, -72.03125000204838102 ) ) ;
#34707=CARTESIAN_POINT ( 'NONE',  ( 4.999999999999992006, -8.660254037844389075, -77.62500000409677625 ) ) ;
#34710=CARTESIAN_POINT ( 'NONE',  ( -5.405949406250003975, -9.363379034771801557, -198.5312500020484094 ) ) ;
#34712=CARTESIAN_POINT ( 'NONE',  ( 10.81189881249999551, -6.242252689847874514, -10.46875000204836503 ) ) ;
#34713=CARTESIAN_POINT ( 'NONE',  ( 5.405949406249992428, -9.363379034771808662, -145.5937500020483810 ) ) ;
#34715=CARTESIAN_POINT ( 'NONE',  ( 9.999999999998969713, 5.773502691896851502, -57.75000000409676915 ) ) ;
#34716=CARTESIAN_POINT ( 'NONE',  ( 7.644554776091147741E-16, 12.48450537969573659, -128.6562500020483810 ) ) ;
#34717=CARTESIAN_POINT ( 'NONE',  ( 9.999999999999998224, 0.000000000000000000, -186.5000000000000000 ) ) ;
#34718=DIRECTION ( 'NONE',  ( -0.000000000000000000, -0.000000000000000000, 1.000000000000000000 ) ) ;
#34719=CARTESIAN_POINT ( 'NONE',  ( 10.81189881249999551, -6.242252689847874514, -109.6562500020483810 ) ) ;
#34720=ORIENTED_EDGE ( 'NONE', *, *, #7041, .T. ) ;
#34721=LINE ( 'NONE', #11811, #11753 ) ;
#34722=ORIENTED_EDGE ( 'NONE', *, *, #16959, .T. ) ;
#34723=ORIENTED_EDGE ( 'NONE', *, *, #40550, .T. ) ;
#34724=CARTESIAN_POINT ( 'NONE',  ( -10.81189881249999729, 1.324075727343319199E-15, -35.28125000204837391 ) ) ;
#34726=ADVANCED_FACE ( 'NONE', ( #11465 ), #17937, .T. ) ;
#34727=CARTESIAN_POINT ( 'NONE',  ( 7.644554776091147741E-16, 12.48450537969573659, -90.96875000204838102 ) ) ;
#34728=CARTESIAN_POINT ( 'NONE',  ( 0.000000000000000000, 0.000000000000000000, -200.0000000000000000 ) ) ;
#34729=CARTESIAN_POINT ( 'NONE',  ( 5.000000000000000000, 8.660254037844385522, -174.2500000000000284 ) ) ;
#34731=CARTESIAN_POINT ( 'NONE',  ( 9.999999999999998224, 0.000000000000000000, -170.3750000040968189 ) ) ;
#34733=CARTESIAN_POINT ( 'NONE',  ( 4.999999999999992006, -8.660254037844389075, -77.24999999999998579 ) ) ;
#34734=CARTESIAN_POINT ( 'NONE',  ( 10.81189881249999551, -6.242252689847874514, -116.9687500020483810 ) ) ;
#34736=FACE_OUTER_BOUND ( 'NONE', #626, .T. ) ;
#34739=CARTESIAN_POINT ( 'NONE',  ( -4.999999999999996447, 8.660254037844387298, -181.8750000040967905 ) ) ;
#34740=CARTESIAN_POINT ( 'NONE',  ( -5.405949406249996869, 9.363379034771805109, -172.0312500020484094 ) ) ;
#34741=( BOUNDED_CURVE ( )  B_SPLINE_CURVE ( 2, ( #7429, #39585, #13666, #7217, #29894, #3774, #26648 ),
 .UNSPECIFIED., .F., .F. ) 
 B_SPLINE_CURVE_WITH_KNOTS ( ( 3, 2, 2, 3 ),
 ( 0.8208955223880598506, 0.8221393034825871249, 0.8233830845771146212, 0.8246268656716420065 ),
 .UNSPECIFIED. ) 
 CURVE ( )  GEOMETRIC_REPRESENTATION_ITEM ( )  RATIONAL_B_SPLINE_CURVE ( ( 0.9999999999999880096, 0.8660254037844506980, 1.000000000000000000, 0.8660254037844387076, 1.000000000000000000, 0.8660254037844148378, 1.000000000000023981 ) ) 
 REPRESENTATION_ITEM ( '' )  );
#34742=CARTESIAN_POINT ( 'NONE',  ( -2.121150477449813534E-15, -11.54700538379251284, -70.25000000409679046 ) ) ;
#34745=CARTESIAN_POINT ( 'NONE',  ( -10.81189881249999729, -6.242252689847864744, -55.96875000204836681 ) ) ;
#34747=CARTESIAN_POINT ( 'NONE',  ( 7.644554776091147741E-16, 12.48450537969573659, 0.3437499979516377424 ) ) ;
#34749=CYLINDRICAL_SURFACE ( 'NONE', #17128, 9.999999999999998224 ) ;
#34751=CARTESIAN_POINT ( 'NONE',  ( -9.999999999999998224, 1.224646799147353059E-15, -100.2499999999999858 ) ) ;
#34753=CARTESIAN_POINT ( 'NONE',  ( -2.121150477449813534E-15, -11.54700538379251284, -106.2500000040967763 ) ) ;
#34754=CARTESIAN_POINT ( 'NONE',  ( 5.000000000000000000, 8.660254037844385522, -82.74999999999997158 ) ) ;
#34757=CARTESIAN_POINT ( 'NONE',  ( 10.81189881249999551, -6.242252689847874514, -99.15625000204839523 ) ) ;
#34760=CARTESIAN_POINT ( 'NONE',  ( 5.405949406249999534, 9.363379034771803333, -157.2812500020484094 ) ) ;
#34763=CARTESIAN_POINT ( 'NONE',  ( -5.000000000000003553, -8.660254037844383745, -24.99999999999996803 ) ) ;
#34764=APPLICATION_CONTEXT ( 'configuration controlled 3d designs of mechanical parts and assemblies' ) ;
#34765=CARTESIAN_POINT ( 'NONE',  ( 10.81189881249999729, 6.242252689847867408, -26.90625000204837391 ) ) ;
#34766=CARTESIAN_POINT ( 'NONE',  ( 7.070501591499377789E-16, 11.54700538379251284, -160.6250000000000284 ) ) ;
#34767=CARTESIAN_POINT ( 'NONE',  ( -9.999999999999998224, 1.224646799147353059E-15, -190.6250000040967905 ) ) ;
#34769=CYLINDRICAL_SURFACE ( 'NONE', #41489, 10.00000000000000178 ) ;
#34770=CARTESIAN_POINT ( 'NONE',  ( 10.81189881249999729, 0.000000000000000000, -136.5312500020484094 ) ) ;
#34771=CARTESIAN_POINT ( 'NONE',  ( 5.000000000000000000, 8.660254037844385522, -75.62500000409677625 ) ) ;
#34774=CARTESIAN_POINT ( 'NONE',  ( 10.81189881249999729, 0.000000000000000000, -58.53125000204836681 ) ) ;
#34776=ADVANCED_FACE ( 'NONE', ( #27888 ), #41021, .T. ) ;
#34780=CARTESIAN_POINT ( 'NONE',  ( 9.999999999999998224, 0.000000000000000000, -25.99999999999996803 ) ) ;
#34781=CARTESIAN_POINT ( 'NONE',  ( -10.81189881249999729, 6.242252689847871849, -155.2187500020483810 ) ) ;
#34783=CARTESIAN_POINT ( 'NONE',  ( 10.81189881249999907, 6.242252689847868297, -5.718750002048342829 ) ) ;
#34784=CARTESIAN_POINT ( 'NONE',  ( 5.405949406249999534, 9.363379034771803333, -139.0937500020483810 ) ) ;
#34785=CARTESIAN_POINT ( 'NONE',  ( 7.644554776091147741E-16, 12.48450537969573659, -97.15625000204839523 ) ) ;
#34787=FACE_OUTER_BOUND ( 'NONE', #8174, .T. ) ;
#34789=CARTESIAN_POINT ( 'NONE',  ( -5.405949406250003975, -9.363379034771801557, -6.343750002048370362 ) ) ;
#34792=CARTESIAN_POINT ( 'NONE',  ( 10.81189881249999729, 0.000000000000000000, -198.0312500020484094 ) ) ;
#34793=CARTESIAN_POINT ( 'NONE',  ( 5.000000000000000000, 8.660254037844385522, -12.24999999999995559 ) ) ;
#34796=CARTESIAN_POINT ( 'NONE',  ( -5.405949406250003975, -9.363379034771801557, -76.84375000204838102 ) ) ;
#34797=CARTESIAN_POINT ( 'NONE',  ( 5.405949406249992428, -9.363379034771808662, -57.09375000204835970 ) ) ;
#34799=CARTESIAN_POINT ( 'NONE',  ( -10.81189881249999729, 1.324075727343319199E-15, -30.78125000204837036 ) ) ;
#34801=CARTESIAN_POINT ( 'NONE',  ( -4.999999999999996447, 8.660254037844387298, -136.5000000000000000 ) ) ;
#34803=CARTESIAN_POINT ( 'NONE',  ( 10.00000000000000000, 5.773502691896255534, -120.3749999999999858 ) ) ;
#34807=CARTESIAN_POINT ( 'NONE',  ( -5.405949406249996869, 9.363379034771805109, -7.031250002048378356 ) ) ;
#34808=ORIENTED_EDGE ( 'NONE', *, *, #13142, .F. ) ;
#34811=CARTESIAN_POINT ( 'NONE',  ( 9.999999999999998224, 0.000000000000000000, -99.49999999999998579 ) ) ;
#34813=CARTESIAN_POINT ( 'NONE',  ( -5.000000000000003553, -8.660254037844383745, -23.87500000409675849 ) ) ;
#34814=CARTESIAN_POINT ( 'NONE',  ( 7.070501591499376803E-16, 11.54700538379251284, -148.6250000000000000 ) ) ;
#34816=CARTESIAN_POINT ( 'NONE',  ( 4.999999999999992006, -8.660254037844389075, -105.7499999999999858 ) ) ;
#34817=CARTESIAN_POINT ( 'NONE',  ( -2.293366432827344421E-15, -12.48450537969573659, -148.9062500020483810 ) ) ;
#34819=CARTESIAN_POINT ( 'NONE',  ( 5.405949406249999534, 9.363379034771803333, -127.0937500020483668 ) ) ;
#34820=CARTESIAN_POINT ( 'NONE',  ( 9.999999999999998224, 0.000000000000000000, -200.0000000000000000 ) ) ;
#34821=( BOUNDED_CURVE ( )  B_SPLINE_CURVE ( 2, ( #40418, #37636, #10862, #7643, #24053, #20794, #8075 ),
 .UNSPECIFIED., .F., .F. ) 
 B_SPLINE_CURVE_WITH_KNOTS ( ( 3, 2, 2, 3 ),
 ( 0.6567164179104479915, 0.6579601990049753768, 0.6592039800995028731, 0.6604477611940301474 ),
 .UNSPECIFIED. ) 
 CURVE ( )  GEOMETRIC_REPRESENTATION_ITEM ( )  RATIONAL_B_SPLINE_CURVE ( ( 0.9999999999999761302, 0.8660254037844625774, 1.000000000000000000, 0.8660254037844387076, 1.000000000000000000, 0.8660254037844028474, 1.000000000000035971 ) ) 
 REPRESENTATION_ITEM ( '' )  );
#34824=EDGE_CURVE ( 'NONE', #39040, #23886, #4844, .T. ) ;
#34826=ORIENTED_EDGE ( 'NONE', *, *, #22769, .T. ) ;
#34827=CARTESIAN_POINT ( 'NONE',  ( 10.81189881249999907, 6.242252689847868297, -185.7187500020483810 ) ) ;
#34828=CARTESIAN_POINT ( 'NONE',  ( 5.405949406249999534, 9.363379034771803333, -34.09375000204836681 ) ) ;
#34829=CARTESIAN_POINT ( 'NONE',  ( -9.999999999999998224, 1.224646799147353059E-15, -41.74999999999997868 ) ) ;
#34830=CARTESIAN_POINT ( 'NONE',  ( -5.405949406249996869, 9.363379034771805109, -174.8437500020484094 ) ) ;
#34831=CARTESIAN_POINT ( 'NONE',  ( 7.644554776091147741E-16, 12.48450537969573659, -150.9687500020483810 ) ) ;
#34832=LINE ( 'NONE', #11284, #23825 ) ;
#34834=AXIS2_PLACEMENT_3D ( 'NONE', #2262, #15383, #5703 ) ;
#34837=CARTESIAN_POINT ( 'NONE',  ( -10.00000000000076916, 5.773502691895813221, -128.8749999999999716 ) ) ;
#34839=CARTESIAN_POINT ( 'NONE',  ( -2.293366432827344421E-15, -12.48450537969573659, -81.21875000204838102 ) ) ;
#34840=CARTESIAN_POINT ( 'NONE',  ( 10.00000000000102318, -5.773502691895667560, -82.00000000409670520 ) ) ;
#34841=CARTESIAN_POINT ( 'NONE',  ( -10.81189881249999729, 6.242252689847871849, -59.40625000204838813 ) ) ;
#34845=CARTESIAN_POINT ( 'NONE',  ( 10.81189881249999551, -6.242252689847874514, -115.6562500020483810 ) ) ;
#34846=CARTESIAN_POINT ( 'NONE',  ( 5.405949406249992428, -9.363379034771808662, -145.7812500020483810 ) ) ;
#34849=CARTESIAN_POINT ( 'NONE',  ( -2.121150477449813534E-15, -11.54700538379251284, -125.7500000040967763 ) ) ;
#34851=ORIENTED_EDGE ( 'NONE', *, *, #6433, .F. ) ;
#34852=VECTOR ( 'NONE', #22055, 1000.000000000000000 ) ;
#34855=CARTESIAN_POINT ( 'NONE',  ( 0.000000000000000000, 0.000000000000000000, -200.0000000000000000 ) ) ;
#34856=CARTESIAN_POINT ( 'NONE',  ( 10.81189881249999729, 0.000000000000000000, -184.5312500020484094 ) ) ;
#34859=CARTESIAN_POINT ( 'NONE',  ( -2.121150477449813534E-15, -11.54700538379251284, -56.75000000409676915 ) ) ;
#34861=CYLINDRICAL_SURFACE ( 'NONE', #15934, 9.999999999999998224 ) ;
#34863=( BOUNDED_CURVE ( )  B_SPLINE_CURVE ( 2, ( #29946, #36195, #3397, #39847, #20213, #26279, #6632 ),
 .UNSPECIFIED., .F., .F. ) 
 B_SPLINE_CURVE_WITH_KNOTS ( ( 3, 2, 2, 3 ),
 ( 0.5932835820895523415, 0.5945273631840797268, 0.5957711442786072231, 0.5970149253731344974 ),
 .UNSPECIFIED. ) 
 CURVE ( )  GEOMETRIC_REPRESENTATION_ITEM ( )  RATIONAL_B_SPLINE_CURVE ( ( 0.9999999999999880096, 0.8660254037844506980, 1.000000000000000000, 0.8660254037844387076, 1.000000000000000000, 0.8660254037844148378, 1.000000000000023981 ) ) 
 REPRESENTATION_ITEM ( '' )  );
#34866=CARTESIAN_POINT ( 'NONE',  ( 5.405949406249999534, 9.363379034771803333, -166.2812500020484094 ) ) ;
#34867=DIRECTION ( 'NONE',  ( -0.000000000000000000, -0.000000000000000000, 1.000000000000000000 ) ) ;
#34868=CARTESIAN_POINT ( 'NONE',  ( -9.999999999999998224, 1.224646799147353059E-15, -23.74999999999996447 ) ) ;
#34869=ORIENTED_EDGE ( 'NONE', *, *, #31375, .T. ) ;
#34870=CARTESIAN_POINT ( 'NONE',  ( -4.999999999999996447, 8.660254037844387298, -84.37500000409677625 ) ) ;
#34871=AXIS2_PLACEMENT_3D ( 'NONE', #31819, #28573, #22300 ) ;
#34872=CARTESIAN_POINT ( 'NONE',  ( 9.999999999999998224, 0.000000000000000000, -150.8750000040967905 ) ) ;
#34873=CARTESIAN_POINT ( 'NONE',  ( 5.405949406249992428, -9.363379034771808662, -81.28125000204839523 ) ) ;
#34874=VERTEX_POINT ( 'NONE', #5862 ) ;
#34876=CARTESIAN_POINT ( 'NONE',  ( 5.000000000000000000, 8.660254037844385522, -30.24999999999997158 ) ) ;
#34880=CARTESIAN_POINT ( 'NONE',  ( -2.293366432827344421E-15, -12.48450537969573659, -37.71875000204836681 ) ) ;
#34881=CARTESIAN_POINT ( 'NONE',  ( -9.999999999999998224, 1.224646799147353059E-15, -187.2500000000000000 ) ) ;
#34882=CARTESIAN_POINT ( 'NONE',  ( 5.405949406249992428, -9.363379034771808662, -7.781250002048350822 ) ) ;
#34883=CARTESIAN_POINT ( 'NONE',  ( 10.81189881249999551, -6.242252689847874514, -64.46875000204838102 ) ) ;
#34884=ORIENTED_EDGE ( 'NONE', *, *, #33532, .T. ) ;
#34885=CARTESIAN_POINT ( 'NONE',  ( -9.999999999998969713, -5.773502691896847949, -4.124999999999929834 ) ) ;
#34887=CYLINDRICAL_SURFACE ( 'NONE', #112, 9.999999999999998224 ) ;
#34888=CARTESIAN_POINT ( 'NONE',  ( 10.81189881249999907, 6.242252689847868297, -178.2187500020483810 ) ) ;
#34890=CARTESIAN_POINT ( 'NONE',  ( 9.999999999999479527, 5.773502691896553074, -43.87499999999995737 ) ) ;
#34891=CARTESIAN_POINT ( 'NONE',  ( -9.999999999999998224, 1.224646799147353059E-15, -127.6250000040967620 ) ) ;
#34892=CARTESIAN_POINT ( 'NONE',  ( -5.000000000000003553, -8.660254037844383745, -101.8750000040967905 ) ) ;
#34894=CARTESIAN_POINT ( 'NONE',  ( -10.81189881249999729, 6.242252689847871849, -105.7187500020483668 ) ) ;
#34895=CARTESIAN_POINT ( 'NONE',  ( 0.000000000000000000, 0.000000000000000000, -200.0000000000000000 ) ) ;
#34896=CARTESIAN_POINT ( 'NONE',  ( -10.81189881249999729, 6.242252689847871849, -81.90625000204838102 ) ) ;
#34898=CARTESIAN_POINT ( 'NONE',  ( 10.81189881249999729, 0.000000000000000000, -89.84375000204838102 ) ) ;
#34899=EDGE_CURVE ( 'NONE', #7087, #6715, #35434, .T. ) ;
#34901=CARTESIAN_POINT ( 'NONE',  ( 10.00000000000000000, 5.773502691896255534, -146.2500000040967905 ) ) ;
#34905=DIRECTION ( 'NONE',  ( -4.506943796211477094E-16, 1.000000000000000000, 0.000000000000000000 ) ) ;
#34906=CARTESIAN_POINT ( 'NONE',  ( 9.999999999999998224, 0.000000000000000000, -197.0000000000000000 ) ) ;
#34908=ORIENTED_EDGE ( 'NONE', *, *, #31002, .T. ) ;
#34909=CARTESIAN_POINT ( 'NONE',  ( -9.999999999999998224, 5.773502691896259087, -68.87499999999998579 ) ) ;
#34911=CARTESIAN_POINT ( 'NONE',  ( 9.999999999999998224, 0.000000000000000000, -80.37500000409677625 ) ) ;
#34912=CARTESIAN_POINT ( 'NONE',  ( 9.999999999999998224, 0.000000000000000000, -46.99999999999998579 ) ) ;
#34913=CARTESIAN_POINT ( 'NONE',  ( 7.070501591499376803E-16, 11.54700538379251284, -8.000000004096749606 ) ) ;
#34915=CARTESIAN_POINT ( 'NONE',  ( -5.405949406249996869, 9.363379034771805109, -73.03125000204838102 ) ) ;
#34917=DIRECTION ( 'NONE',  ( 0.4999999999999998335, 0.8660254037844387076, 0.000000000000000000 ) ) ;
#34920=CARTESIAN_POINT ( 'NONE',  ( 10.81189881249999551, -6.242252689847874514, -193.6562500020484379 ) ) ;
#34922=CARTESIAN_POINT ( 'NONE',  ( 5.405949406249992428, -9.363379034771808662, -9.093750002048345493 ) ) ;
#34923=CARTESIAN_POINT ( 'NONE',  ( -9.999999999999998224, 1.224646799147353059E-15, -15.12500000409674961 ) ) ;
#34925=CARTESIAN_POINT ( 'NONE',  ( -2.293366432827344421E-15, -12.48450537969573659, -147.2187500020484094 ) ) ;
#34926=CARTESIAN_POINT ( 'NONE',  ( 10.00000000000102318, -5.773502691895667560, -37.00000000409672651 ) ) ;
#34927=FACE_OUTER_BOUND ( 'NONE', #34453, .T. ) ;
#34928=CARTESIAN_POINT ( 'NONE',  ( -5.000000000000003553, -8.660254037844383745, -172.0000000000000000 ) ) ;
#34929=CARTESIAN_POINT ( 'NONE',  ( -9.999999999999998224, 1.224646799147353059E-15, -36.12500000409676915 ) ) ;
#34930=CARTESIAN_POINT ( 'NONE',  ( -5.405949406250003975, -9.363379034771801557, -104.0312500020483810 ) ) ;
#34931=ORIENTED_EDGE ( 'NONE', *, *, #17469, .T. ) ;
#34932=CARTESIAN_POINT ( 'NONE',  ( 0.000000000000000000, 0.000000000000000000, -200.0000000000000000 ) ) ;
#34934=ORIENTED_EDGE ( 'NONE', *, *, #15931, .F. ) ;
#34936=CARTESIAN_POINT ( 'NONE',  ( 7.644554776091147741E-16, 12.48450537969573659, -28.15625000204838457 ) ) ;
#34938=CARTESIAN_POINT ( 'NONE',  ( 10.81189881249999729, 0.000000000000000000, -89.84375000204838102 ) ) ;
#34939=DIRECTION ( 'NONE',  ( 1.000000000000000000, 0.000000000000000000, 0.000000000000000000 ) ) ;
#34941=CARTESIAN_POINT ( 'NONE',  ( 9.999999999999479527, 5.773502691896553074, -123.3749999999999858 ) ) ;
#34943=CARTESIAN_POINT ( 'NONE',  ( 7.070501591499377789E-16, 11.54700538379251284, -9.500000004096756712 ) ) ;
#34944=EDGE_CURVE ( 'NONE', #36032, #16199, #13638, .T. ) ;
#34945=CARTESIAN_POINT ( 'NONE',  ( -2.293366432827344421E-15, -12.48450537969573659, -118.7187500020483668 ) ) ;
#34948=CARTESIAN_POINT ( 'NONE',  ( 7.644554776091147741E-16, 12.48450537969573659, -2.656250002048344161 ) ) ;
#34951=CARTESIAN_POINT ( 'NONE',  ( 7.070501591499377789E-16, 11.54700538379251284, -180.5000000040967905 ) ) ;
#34952=CARTESIAN_POINT ( 'NONE',  ( 5.405949406249999534, 9.363379034771803333, -172.2812500020484094 ) ) ;
#34957=CARTESIAN_POINT ( 'NONE',  ( -2.293366432827344421E-15, -12.48450537969573659, -42.21875000204835260 ) ) ;
#34958=EDGE_CURVE ( 'NONE', #19609, #41727, #18073, .T. ) ;
#34960=CARTESIAN_POINT ( 'NONE',  ( 10.81189881249999551, -6.242252689847874514, -1.656250002048371694 ) ) ;
#34962=CARTESIAN_POINT ( 'NONE',  ( -2.121150477449813534E-15, -11.54700538379251284, -193.2500000040968473 ) ) ;
#34964=CARTESIAN_POINT ( 'NONE',  ( 10.00000000000000000, 5.773502691896255534, -88.87499999999998579 ) ) ;
#34966=CARTESIAN_POINT ( 'NONE',  ( -4.999999999999996447, 8.660254037844387298, -108.3750000040967763 ) ) ;
#34967=DIRECTION ( 'NONE',  ( -0.000000000000000000, -0.000000000000000000, 1.000000000000000000 ) ) ;
#34970=CARTESIAN_POINT ( 'NONE',  ( 5.405949406249999534, 9.363379034771803333, -101.7812500020483952 ) ) ;
#34971=EDGE_LOOP ( 'NONE', ( #38197, #28964, #26414, #15469 ) ) ;
#34973=CARTESIAN_POINT ( 'NONE',  ( -9.999999999999998224, 1.224646799147353059E-15, -28.62500000409676204 ) ) ;
#34974=CARTESIAN_POINT ( 'NONE',  ( -2.293366432827344421E-15, -12.48450537969573659, -154.9062500020483810 ) ) ;
#34976=ORIENTED_EDGE ( 'NONE', *, *, #3590, .T. ) ;
#34977=CARTESIAN_POINT ( 'NONE',  ( -2.121150477449813534E-15, -11.54700538379251284, -14.37499999999997158 ) ) ;
#34978=CARTESIAN_POINT ( 'NONE',  ( -10.81189881249999729, 1.324075727343319199E-15, -29.28125000204837036 ) ) ;
#34979=CARTESIAN_POINT ( 'NONE',  ( -9.999999999999998224, 1.224646799147353059E-15, -151.2500000000000000 ) ) ;
#34983=CARTESIAN_POINT ( 'NONE',  ( -5.405949406250003975, -9.363379034771801557, -122.0312500020483952 ) ) ;
#34984=CARTESIAN_POINT ( 'NONE',  ( 5.134740825434541023, 9.087941876063259983, -1.486633740873807081E-14 ) ) ;
#34985=CARTESIAN_POINT ( 'NONE',  ( 4.999999999999992006, -8.660254037844389075, -44.62500000409677625 ) ) ;
#34987=( BOUNDED_CURVE ( )  B_SPLINE_CURVE ( 2, ( #31851, #32264, #5505, #25153, #18876, #2285, #16035 ),
 .UNSPECIFIED., .F., .F. ) 
 B_SPLINE_CURVE_WITH_KNOTS ( ( 3, 2, 2, 3 ),
 ( 0.7126865671641793298, 0.7139303482587067151, 0.7151741293532342114, 0.7164179104477614857 ),
 .UNSPECIFIED. ) 
 CURVE ( )  GEOMETRIC_REPRESENTATION_ITEM ( )  RATIONAL_B_SPLINE_CURVE ( ( 0.9999999999999761302, 0.8660254037844625774, 1.000000000000000000, 0.8660254037844387076, 1.000000000000000000, 0.8660254037844028474, 1.000000000000035971 ) ) 
 REPRESENTATION_ITEM ( '' )  );
#34988=CARTESIAN_POINT ( 'NONE',  ( 10.81189881249999551, -6.242252689847874514, -60.15625000204839523 ) ) ;
#34990=CARTESIAN_POINT ( 'NONE',  ( 7.644554776091147741E-16, 12.48450537969573659, -110.4687500020483668 ) ) ;
#34991=VERTEX_POINT ( 'NONE', #20704 ) ;
#34993=DIRECTION ( 'NONE',  ( 1.000000000000000000, 0.000000000000000000, 0.000000000000000000 ) ) ;
#34994=DIRECTION ( 'NONE',  ( -0.000000000000000000, -0.000000000000000000, 1.000000000000000000 ) ) ;
#34995=CARTESIAN_POINT ( 'NONE',  ( 10.81189881249999907, 6.242252689847868297, -154.2187500020483810 ) ) ;
#34997=CARTESIAN_POINT ( 'NONE',  ( 5.405949406249992428, -9.363379034771808662, -7.593750002048343717 ) ) ;
#34998=CARTESIAN_POINT ( 'NONE',  ( -2.293366432827344421E-15, -12.48450537969573659, -139.7187500020483810 ) ) ;
#35002=CARTESIAN_POINT ( 'NONE',  ( 5.405949406249999534, 9.363379034771803333, 0.4062499979516354109 ) ) ;
#35004=CARTESIAN_POINT ( 'NONE',  ( 5.405949406249992428, -9.363379034771808662, -193.7812500020484094 ) ) ;
#35008=CARTESIAN_POINT ( 'NONE',  ( -10.81189881249999729, 6.242252689847871849, -71.21875000204839523 ) ) ;
#35009=CARTESIAN_POINT ( 'NONE',  ( 7.644554776091147741E-16, 12.48450537969573659, -54.96875000204836681 ) ) ;
#35011=CARTESIAN_POINT ( 'NONE',  ( -5.405949406249996869, 9.363379034771805109, -29.53125000204837036 ) ) ;
#35012=VECTOR ( 'NONE', #389, 1000.000000000000000 ) ;
#35014=CARTESIAN_POINT ( 'NONE',  ( -10.00000000000076916, 5.773502691895813221, -136.3749999999999716 ) ) ;
#35016=CARTESIAN_POINT ( 'NONE',  ( 4.999999999999992006, -8.660254037844389075, -111.7499999999999858 ) ) ;
#35017=CARTESIAN_POINT ( 'NONE',  ( 4.999999999999992006, -8.660254037844389075, -170.2500000000000000 ) ) ;
#35020=CARTESIAN_POINT ( 'NONE',  ( 10.81189881249999729, 6.242252689847867408, -11.90625000204835615 ) ) ;
#35021=VERTEX_POINT ( 'NONE', #30649 ) ;
#35025=CARTESIAN_POINT ( 'NONE',  ( -9.999999999999998224, 1.224646799147353059E-15, -47.74999999999998579 ) ) ;
#35027=CARTESIAN_POINT ( 'NONE',  ( -10.00000000000000000, -5.773502691896251982, -27.00000000409677625 ) ) ;
#35028=CARTESIAN_POINT ( 'NONE',  ( -9.999999999998969713, -5.773502691896847949, -3.000000004096732731 ) ) ;
#35030=CARTESIAN_POINT ( 'NONE',  ( -5.000000000000003553, -8.660254037844383745, -99.99999999999998579 ) ) ;
#35031=CARTESIAN_POINT ( 'NONE',  ( -10.81189881249999907, -6.242252689847864744, -141.6562500020483810 ) ) ;
#35032=CARTESIAN_POINT ( 'NONE',  ( -10.81189881249999729, 6.242252689847871849, -131.2187500020483810 ) ) ;
#35034=CARTESIAN_POINT ( 'NONE',  ( -2.121150477449813534E-15, -11.54700538379251284, -127.2500000040967763 ) ) ;
#35036=EDGE_CURVE ( 'NONE', #2553, #18128, #37099, .T. ) ;
#35037=ORIENTED_EDGE ( 'NONE', *, *, #36779, .T. ) ;
#35041=CARTESIAN_POINT ( 'NONE',  ( 0.000000000000000000, 0.000000000000000000, -200.0000000000000000 ) ) ;
#35042=CARTESIAN_POINT ( 'NONE',  ( 7.644554776091147741E-16, 12.48450537969573659, -179.4687500020483810 ) ) ;
#35043=CARTESIAN_POINT ( 'NONE',  ( -10.81189881249999729, 1.324075727343319199E-15, -33.59375000204836681 ) ) ;
#35044=CARTESIAN_POINT ( 'NONE',  ( 5.405949406249992428, -9.363379034771808662, -168.0937500020484094 ) ) ;
#35045=CARTESIAN_POINT ( 'NONE',  ( -10.81189881249999729, 6.242252689847871849, -153.7187500020483526 ) ) ;
#35046=CYLINDRICAL_SURFACE ( 'NONE', #19678, 9.999999999999998224 ) ;
#35050=CARTESIAN_POINT ( 'NONE',  ( 9.999999999999998224, 0.000000000000000000, -129.5000000000000000 ) ) ;
#35051=CARTESIAN_POINT ( 'NONE',  ( 9.999999999999998224, 0.000000000000000000, -11.37500000409674783 ) ) ;
#35053=CARTESIAN_POINT ( 'NONE',  ( 5.405949406249992428, -9.363379034771808662, -79.59375000204838102 ) ) ;
#35054=LINE ( 'NONE', #19061, #10685 ) ;
#35055=CARTESIAN_POINT ( 'NONE',  ( 10.81189881249999551, -6.242252689847874514, -46.65625000204835970 ) ) ;
#35058=CARTESIAN_POINT ( 'NONE',  ( -10.81189881249999729, 6.242252689847871849, -111.9062500020483810 ) ) ;
#35059=CARTESIAN_POINT ( 'NONE',  ( -10.81189881249999729, 1.324075727343319199E-15, -146.2812500020483810 ) ) ;
#35060=CARTESIAN_POINT ( 'NONE',  ( 9.999999999999998224, 0.000000000000000000, -143.3750000040967905 ) ) ;
#35062=CARTESIAN_POINT ( 'NONE',  ( 10.00000000000000000, 5.773502691896255534, -123.7500000040967905 ) ) ;
#35064=EDGE_CURVE ( 'NONE', #35302, #13289, #22495, .T. ) ;
#35065=VERTEX_POINT ( 'NONE', #13366 ) ;
#35068=CARTESIAN_POINT ( 'NONE',  ( 9.999999999999678479, 5.773502691896442940, -184.8750000000000284 ) ) ;
#35069=CARTESIAN_POINT ( 'NONE',  ( 5.405949406249999534, 9.363379034771803333, -182.7812500020484094 ) ) ;
#35070=ORIENTED_EDGE ( 'NONE', *, *, #13176, .F. ) ;
#35071=CARTESIAN_POINT ( 'NONE',  ( -10.00000000000000000, -5.773502691896251982, -51.00000000409676204 ) ) ;
#35076=DIRECTION ( 'NONE',  ( -0.000000000000000000, -0.000000000000000000, 1.000000000000000000 ) ) ;
#35077=CARTESIAN_POINT ( 'NONE',  ( 10.81189881249999907, 6.242252689847868297, -166.4062500020483810 ) ) ;
#35079=CARTESIAN_POINT ( 'NONE',  ( 10.00000000000051159, -5.773502691895965988, -34.00000000409673362 ) ) ;
#35082=CARTESIAN_POINT ( 'NONE',  ( 7.070501591499376803E-16, 11.54700538379251284, -17.00000000409675849 ) ) ;
#35083=CARTESIAN_POINT ( 'NONE',  ( -2.121150477449813534E-15, -11.54700538379251284, -194.3750000000000284 ) ) ;
#35084=CARTESIAN_POINT ( 'NONE',  ( -9.999999999999998224, 1.224646799147353059E-15, -136.6250000040967620 ) ) ;
#35085=CARTESIAN_POINT ( 'NONE',  ( -10.81189881249999729, 6.242252689847871849, -80.40625000204839523 ) ) ;
#35089=ORIENTED_EDGE ( 'NONE', *, *, #12748, .F. ) ;
#35090=CARTESIAN_POINT ( 'NONE',  ( 7.644554776091147741E-16, 12.48450537969573659, -30.96875000204835260 ) ) ;
#35092=CARTESIAN_POINT ( 'NONE',  ( -2.293366432827344421E-15, -12.48450537969573659, -3.406250002048348158 ) ) ;
#35093=CARTESIAN_POINT ( 'NONE',  ( 10.81189881249999729, 0.000000000000000000, -58.34375000204835970 ) ) ;
#35094=VERTEX_POINT ( 'NONE', #16814 ) ;
#35095=DIRECTION ( 'NONE',  ( 1.000000000000000000, 0.000000000000000000, 0.000000000000000000 ) ) ;
#35098=CARTESIAN_POINT ( 'NONE',  ( 10.81189881249999551, -6.242252689847874514, -184.4687500020483810 ) ) ;
#35099=CARTESIAN_POINT ( 'NONE',  ( 7.644554776091147741E-16, 12.48450537969573659, -176.4687500020483810 ) ) ;
#35103=CARTESIAN_POINT ( 'NONE',  ( 9.999999999999998224, 0.000000000000000000, -191.3750000040967905 ) ) ;
#35106=CARTESIAN_POINT ( 'NONE',  ( 10.81189881249999729, 0.000000000000000000, -101.8437500020483810 ) ) ;
#35107=CARTESIAN_POINT ( 'NONE',  ( -9.999999999999998224, 1.224646799147353059E-15, -115.6250000040967905 ) ) ;
#35108=CARTESIAN_POINT ( 'NONE',  ( -10.81189881249999729, 6.242252689847871849, -83.40625000204836681 ) ) ;
#35109=CARTESIAN_POINT ( 'NONE',  ( -10.81189881249999729, -6.242252689847864744, -90.46875000204838102 ) ) ;
#35111=CARTESIAN_POINT ( 'NONE',  ( -9.999999999999998224, 1.224646799147353059E-15, -142.6250000040967905 ) ) ;
#35117=CARTESIAN_POINT ( 'NONE',  ( -9.999999999999998224, 1.224646799147353059E-15, -97.62500000409677625 ) ) ;
#35118=CARTESIAN_POINT ( 'NONE',  ( -2.121150477449813534E-15, -11.54700538379251284, -51.87499999999997868 ) ) ;
#35120=ORIENTED_EDGE ( 'NONE', *, *, #27036, .T. ) ;
#35121=CARTESIAN_POINT ( 'NONE',  ( -4.999999999999996447, 8.660254037844387298, -62.99999999999997158 ) ) ;
#35123=CARTESIAN_POINT ( 'NONE',  ( 5.000000000000000000, 8.660254037844385522, -75.62500000409677625 ) ) ;
#35127=CARTESIAN_POINT ( 'NONE',  ( -5.405949406250003975, -9.363379034771801557, -74.03125000204838102 ) ) ;
#35128=( BOUNDED_CURVE ( )  B_SPLINE_CURVE ( 2, ( #35725, #30256, #12600, #16841, #23989, #6155, #33496 ),
 .UNSPECIFIED., .F., .F. ) 
 B_SPLINE_CURVE_WITH_KNOTS ( ( 3, 2, 2, 3 ),
 ( 0.4552238805970150737, 0.4564676616915424590, 0.4577114427860698442, 0.4589552238805971740 ),
 .UNSPECIFIED. ) 
 CURVE ( )  GEOMETRIC_REPRESENTATION_ITEM ( )  RATIONAL_B_SPLINE_CURVE ( ( 0.9999999999999820144, 0.8660254037844566932, 1.000000000000000000, 0.8660254037844387076, 1.000000000000000000, 0.8660254037844207220, 1.000000000000017986 ) ) 
 REPRESENTATION_ITEM ( '' )  );
#35132=VERTEX_POINT ( 'NONE', #30013 ) ;
#35133=CARTESIAN_POINT ( 'NONE',  ( 5.405949406249992428, -9.363379034771808662, -192.2812500020484094 ) ) ;
#35135=CARTESIAN_POINT ( 'NONE',  ( 7.644554776091147741E-16, 12.48450537969573659, -2.468750002048359704 ) ) ;
#35138=CARTESIAN_POINT ( 'NONE',  ( -9.999999999999998224, 5.773502691896259087, -175.3750000000000000 ) ) ;
#35139=CARTESIAN_POINT ( 'NONE',  ( 0.000000000000000000, 0.000000000000000000, -200.0000000000000000 ) ) ;
#35140=CARTESIAN_POINT ( 'NONE',  ( -10.81189881249999729, 1.324075727343319199E-15, -104.2812500020483810 ) ) ;
#35141=EDGE_LOOP ( 'NONE', ( #40437, #27511, #11872, #13011 ) ) ;
#35144=ORIENTED_EDGE ( 'NONE', *, *, #24156, .F. ) ;
#35145=ADVANCED_FACE ( 'NONE', ( #10349 ), #23537, .T. ) ;
#35146=ORIENTED_EDGE ( 'NONE', *, *, #21446, .F. ) ;
#35147=CARTESIAN_POINT ( 'NONE',  ( 7.644554776091147741E-16, 12.48450537969573659, -31.15625000204835260 ) ) ;
#35149=CARTESIAN_POINT ( 'NONE',  ( 10.81189881249999551, -6.242252689847874514, -80.96875000204838102 ) ) ;
#35150=CARTESIAN_POINT ( 'NONE',  ( 4.999999999999992006, -8.660254037844389075, -4.125000004096768258 ) ) ;
#35151=CARTESIAN_POINT ( 'NONE',  ( 10.81189881249999907, 6.242252689847868297, -199.2187500020484094 ) ) ;
#35152=CARTESIAN_POINT ( 'NONE',  ( 9.999999999999998224, 0.000000000000000000, -69.87500000409677625 ) ) ;
#35154=CARTESIAN_POINT ( 'NONE',  ( 10.00000000000000000, 5.773502691896255534, -14.25000000409676382 ) ) ;
#35156=CARTESIAN_POINT ( 'NONE',  ( 10.81189881249999551, -6.242252689847874514, -125.9687500020483810 ) ) ;
#35157=CARTESIAN_POINT ( 'NONE',  ( -10.81189881249999729, -6.242252689847864744, -118.9687500020483810 ) ) ;
#35161=CARTESIAN_POINT ( 'NONE',  ( 9.999999999999996447, -5.773502691896262640, -173.5000000040968189 ) ) ;
#35162=CARTESIAN_POINT ( 'NONE',  ( 10.81189881249999729, 0.000000000000000000, -168.0312500020484094 ) ) ;
#35163=CARTESIAN_POINT ( 'NONE',  ( -4.999999999999996447, 8.660254037844387298, -102.3750000040967905 ) ) ;
#35166=CARTESIAN_POINT ( 'NONE',  ( 7.644554776091147741E-16, 12.48450537969573659, -41.46875000204835260 ) ) ;
#35167=AXIS2_PLACEMENT_3D ( 'NONE', #14768, #41093, #21691 ) ;
#35169=CARTESIAN_POINT ( 'NONE',  ( -5.405949406249996869, 9.363379034771805109, -4.031250002048375691 ) ) ;
#35171=CARTESIAN_POINT ( 'NONE',  ( -9.999999999999998224, 1.224646799147353059E-15, -64.24999999999997158 ) ) ;
#35173=CARTESIAN_POINT ( 'NONE',  ( 9.999999999999998224, 0.000000000000000000, -87.49999999999998579 ) ) ;
#35175=CARTESIAN_POINT ( 'NONE',  ( -5.000000000000003553, -8.660254037844383745, -94.37500000409677625 ) ) ;
#35176=DIRECTION ( 'NONE',  ( -0.000000000000000000, -0.000000000000000000, 1.000000000000000000 ) ) ;
#35178=CARTESIAN_POINT ( 'NONE',  ( 5.405949406249999534, 9.363379034771803333, -97.28125000204839523 ) ) ;
#35181=CARTESIAN_POINT ( 'NONE',  ( -2.293366432827344421E-15, -12.48450537969573659, -156.4062500020483810 ) ) ;
#35183=EDGE_LOOP ( 'NONE', ( #3269, #17088, #32647, #7900 ) ) ;
#35184=CARTESIAN_POINT ( 'NONE',  ( 9.999999999999996447, -5.773502691896262640, -14.12499999999997158 ) ) ;
#35185=CARTESIAN_POINT ( 'NONE',  ( -10.81189881249999729, 1.324075727343319199E-15, -30.78125000204837036 ) ) ;
#35186=CARTESIAN_POINT ( 'NONE',  ( 4.999999999999992006, -8.660254037844389075, -150.7500000000000000 ) ) ;
#35188=CARTESIAN_POINT ( 'NONE',  ( -9.999999999999998224, 1.224646799147353059E-15, -136.6250000040967620 ) ) ;
#35189=CARTESIAN_POINT ( 'NONE',  ( 10.81189881249999907, 6.242252689847868297, -127.4062500020483810 ) ) ;
#35191=CARTESIAN_POINT ( 'NONE',  ( 9.999999999999479527, 5.773502691896553074, -90.37499999999997158 ) ) ;
#35193=CARTESIAN_POINT ( 'NONE',  ( 9.999999999999998224, 0.000000000000000000, -44.37500000409677625 ) ) ;
#35196=CARTESIAN_POINT ( 'NONE',  ( 7.644554776091147741E-16, 12.48450537969573659, -53.65625000204838102 ) ) ;
#35198=CARTESIAN_POINT ( 'NONE',  ( 10.81189881249999907, 6.242252689847868297, -103.2187500020483810 ) ) ;
#35199=ORIENTED_EDGE ( 'NONE', *, *, #31765, .F. ) ;
#35200=VERTEX_POINT ( 'NONE', #31512 ) ;
#35203=CARTESIAN_POINT ( 'NONE',  ( 9.999999999999479527, 5.773502691896553074, -144.7500000040967620 ) ) ;
#35204=CARTESIAN_POINT ( 'NONE',  ( -10.81189881249999729, 6.242252689847871849, -161.2187500020483526 ) ) ;
#35206=CARTESIAN_POINT ( 'NONE',  ( -10.81189881249999907, -6.242252689847864744, -4.968750002048339276 ) ) ;
#35207=CARTESIAN_POINT ( 'NONE',  ( 5.000000000000000000, 8.660254037844385522, -14.12500000409674961 ) ) ;
#35208=EDGE_CURVE ( 'NONE', #17371, #4845, #20840, .T. ) ;
#35209=CARTESIAN_POINT ( 'NONE',  ( 5.405949406249992428, -9.363379034771808662, -141.0937500020483810 ) ) ;
#35213=CARTESIAN_POINT ( 'NONE',  ( -4.999999999999996447, 8.660254037844387298, -190.8750000040967905 ) ) ;
#35215=CARTESIAN_POINT ( 'NONE',  ( 10.81189881249999729, 6.242252689847867408, -196.4062500020484094 ) ) ;
#35216=CARTESIAN_POINT ( 'NONE',  ( 4.999999999999992006, -8.660254037844389075, -5.625000004096769146 ) ) ;
#35219=ADVANCED_FACE ( 'NONE', ( #34533 ), #30859, .T. ) ;
#35220=CARTESIAN_POINT ( 'NONE',  ( -10.81189881249999729, 6.242252689847871849, -68.21875000204838102 ) ) ;
#35221=CARTESIAN_POINT ( 'NONE',  ( -10.81189881249999729, 6.242252689847871849, -57.71875000204836681 ) ) ;
#35223=CARTESIAN_POINT ( 'NONE',  ( -10.81189881249999729, 1.324075727343319199E-15, -24.78125000204836681 ) ) ;
#35227=CARTESIAN_POINT ( 'NONE',  ( -2.121150477449813534E-15, -11.54700538379251284, -114.8749999999999716 ) ) ;
#35231=CARTESIAN_POINT ( 'NONE',  ( 5.405949406249999534, 9.363379034771803333, -13.28125000204835615 ) ) ;
#35233=CARTESIAN_POINT ( 'NONE',  ( 9.999999999999966249, 5.773502691896273298, -197.2500000040968473 ) ) ;
#35235=FACE_OUTER_BOUND ( 'NONE', #39525, .T. ) ;
#35237=CARTESIAN_POINT ( 'NONE',  ( 10.00000000000000000, 5.773502691896255534, -43.87499999999996447 ) ) ;
#35239=CARTESIAN_POINT ( 'NONE',  ( -10.00000000000000000, -5.773502691896251982, -22.50000000409676915 ) ) ;
#35240=CARTESIAN_POINT ( 'NONE',  ( -10.81189881249999729, 1.324075727343319199E-15, -50.28125000204835970 ) ) ;
#35243=( BOUNDED_CURVE ( )  B_SPLINE_CURVE ( 2, ( #27960, #30993, #37882, #14115, #24949, #18227, #27317 ),
 .UNSPECIFIED., .F., .F. ) 
 B_SPLINE_CURVE_WITH_KNOTS ( ( 3, 2, 2, 3 ),
 ( 0.007462686567164185901, 0.008706467661691551230, 0.009950248756218915691, 0.01119402985074628015 ),
 .UNSPECIFIED. ) 
 CURVE ( )  GEOMETRIC_REPRESENTATION_ITEM ( )  RATIONAL_B_SPLINE_CURVE ( ( 0.9999999999999993339, 0.8660254037844394848, 1.000000000000000000, 0.8660254037844387076, 1.000000000000000000, 0.8660254037844373753, 1.000000000000001332 ) ) 
 REPRESENTATION_ITEM ( '' )  );
#35244=CARTESIAN_POINT ( 'NONE',  ( -9.999999999999998224, 1.224646799147353059E-15, -100.2499999999999858 ) ) ;
#35245=CARTESIAN_POINT ( 'NONE',  ( 10.81189881249999729, 0.000000000000000000, -145.5312500020483810 ) ) ;
#35246=CARTESIAN_POINT ( 'NONE',  ( -5.405949406250003975, -9.363379034771801557, -153.5312500020484094 ) ) ;
#35247=CARTESIAN_POINT ( 'NONE',  ( -4.999999999999996447, 8.660254037844387298, -78.37500000409677625 ) ) ;
#35249=ORIENTED_EDGE ( 'NONE', *, *, #3677, .F. ) ;
#35251=ORIENTED_EDGE ( 'NONE', *, *, #1114, .F. ) ;
#35252=CARTESIAN_POINT ( 'NONE',  ( -9.999999999999742428, -5.773502691896402084, -100.5000000040967905 ) ) ;
#35253=CARTESIAN_POINT ( 'NONE',  ( 10.81189881249999729, 0.000000000000000000, -185.8437500020483810 ) ) ;
#35255=CARTESIAN_POINT ( 'NONE',  ( 10.81189881249999907, 6.242252689847868297, -34.21875000204835260 ) ) ;
#35256=EDGE_CURVE ( 'NONE', #15045, #37944, #15301, .T. ) ;
#35257=FACE_OUTER_BOUND ( 'NONE', #35444, .T. ) ;
#35258=CARTESIAN_POINT ( 'NONE',  ( 5.405949406249999534, 9.363379034771803333, -163.0937500020484094 ) ) ;
#35259=CARTESIAN_POINT ( 'NONE',  ( -5.405949406249996869, 9.363379034771805109, -155.3437500020483810 ) ) ;
#35260=DIRECTION ( 'NONE',  ( -0.000000000000000000, -0.000000000000000000, 1.000000000000000000 ) ) ;
#35266=CARTESIAN_POINT ( 'NONE',  ( 9.999999999999742428, 5.773502691896404748, -157.8750000000000000 ) ) ;
#35269=CARTESIAN_POINT ( 'NONE',  ( -10.81189881249999729, 6.242252689847871849, -77.21875000204838102 ) ) ;
#35270=LINE ( 'NONE', #25129, #9319 ) ;
#35271=CARTESIAN_POINT ( 'NONE',  ( 5.405949406249992428, -9.363379034771808662, -48.28125000204838813 ) ) ;
#35274=CARTESIAN_POINT ( 'NONE',  ( 4.999999999999992006, -8.660254037844389075, -135.7499999999999716 ) ) ;
#35275=CARTESIAN_POINT ( 'NONE',  ( -10.81189881249999729, 1.324075727343319199E-15, -144.7812500020483810 ) ) ;
#35276=CARTESIAN_POINT ( 'NONE',  ( 7.070501591499376803E-16, 11.54700538379251284, -143.0000000040967905 ) ) ;
#35278=CARTESIAN_POINT ( 'NONE',  ( -10.00000000000000000, -5.773502691896251982, -124.5000000040967620 ) ) ;
#35280=EDGE_LOOP ( 'NONE', ( #36765, #3019, #34509, #31051 ) ) ;
#35283=CARTESIAN_POINT ( 'NONE',  ( 9.999999999999998224, 0.000000000000000000, -48.49999999999998579 ) ) ;
#35284=CARTESIAN_POINT ( 'NONE',  ( 5.405949406249999534, 9.363379034771803333, -173.7812500020484094 ) ) ;
#35285=CARTESIAN_POINT ( 'NONE',  ( -9.999999999999998224, 1.224646799147353059E-15, -51.12500000409675494 ) ) ;
#35286=CARTESIAN_POINT ( 'NONE',  ( -10.00000000000051337, 5.773502691895962435, -48.25000000409676204 ) ) ;
#35288=VECTOR ( 'NONE', #4754, 1000.000000000000000 ) ;
#35289=DIRECTION ( 'NONE',  ( 1.000000000000000000, 0.000000000000000000, 0.000000000000000000 ) ) ;
#35290=CARTESIAN_POINT ( 'NONE',  ( -10.81189881249999729, 6.242252689847871849, -167.4062500020483810 ) ) ;
#35293=DIRECTION ( 'NONE',  ( 1.000000000000000000, 0.000000000000000000, 0.000000000000000000 ) ) ;
#35294=ORIENTED_EDGE ( 'NONE', *, *, #523, .T. ) ;
#35296=CYLINDRICAL_SURFACE ( 'NONE', #23834, 9.999999999999998224 ) ;
#35297=CARTESIAN_POINT ( 'NONE',  ( 7.070501591499376803E-16, 11.54700538379251284, -27.12499999999998224 ) ) ;
#35298=VECTOR ( 'NONE', #28394, 1000.000000000000000 ) ;
#35299=CARTESIAN_POINT ( 'NONE',  ( 7.644554776091147741E-16, 12.48450537969573659, -77.65625000204838102 ) ) ;
#35302=VERTEX_POINT ( 'NONE', #31080 ) ;
#35304=CARTESIAN_POINT ( 'NONE',  ( 10.81189881249999729, 0.000000000000000000, -32.84375000204836681 ) ) ;
#35305=CARTESIAN_POINT ( 'NONE',  ( -5.000000000000003553, -8.660254037844383745, -187.0000000000000000 ) ) ;
#35306=CARTESIAN_POINT ( 'NONE',  ( -5.405949406249996869, 9.363379034771805109, -4.031250002048375691 ) ) ;
#35307=CARTESIAN_POINT ( 'NONE',  ( -10.81189881249999729, 6.242252689847871849, -53.21875000204837391 ) ) ;
#35311=CARTESIAN_POINT ( 'NONE',  ( -10.81189881249999729, 6.242252689847871849, -191.2187500020484663 ) ) ;
#35312=CARTESIAN_POINT ( 'NONE',  ( 5.405949406249992428, -9.363379034771808662, -180.0937500020484094 ) ) ;
#35314=VECTOR ( 'NONE', #4713, 1000.000000000000000 ) ;
#35316=DIRECTION ( 'NONE',  ( -0.000000000000000000, -0.000000000000000000, 1.000000000000000000 ) ) ;
#35319=CARTESIAN_POINT ( 'NONE',  ( 10.81189881249999907, 6.242252689847868297, -107.7187500020483810 ) ) ;
#35320=FACE_OUTER_BOUND ( 'NONE', #33691, .T. ) ;
#35321=CARTESIAN_POINT ( 'NONE',  ( 10.81189881249999907, 6.242252689847868297, -74.90625000204839523 ) ) ;
#35322=CARTESIAN_POINT ( 'NONE',  ( -5.405949406249996869, 9.363379034771805109, -92.34375000204838102 ) ) ;
#35325=CARTESIAN_POINT ( 'NONE',  ( 9.999999999999996447, -5.773502691896262640, -146.5000000040967905 ) ) ;
#35327=EDGE_CURVE ( 'NONE', #18023, #36134, #17665, .T. ) ;
#35328=ORIENTED_EDGE ( 'NONE', *, *, #37982, .F. ) ;
#35331=CARTESIAN_POINT ( 'NONE',  ( -9.999999999999998224, 1.224646799147353059E-15, -7.249999999999978684 ) ) ;
#35334=ORIENTED_EDGE ( 'NONE', *, *, #29207, .T. ) ;
#35335=CARTESIAN_POINT ( 'NONE',  ( 7.070501591499377789E-16, 11.54700538379251284, -61.62499999999998579 ) ) ;
#35337=CARTESIAN_POINT ( 'NONE',  ( 4.999999999999992006, -8.660254037844389075, -71.62500000409677625 ) ) ;
#35340=CARTESIAN_POINT ( 'NONE',  ( -5.405949406249996869, 9.363379034771805109, -67.03125000204838102 ) ) ;
#35342=DIRECTION ( 'NONE',  ( 1.000000000000000000, 0.000000000000000000, 0.000000000000000000 ) ) ;
#35345=CARTESIAN_POINT ( 'NONE',  ( 10.81189881249999551, -6.242252689847874514, -195.1562500020484379 ) ) ;
#35347=CARTESIAN_POINT ( 'NONE',  ( -10.81189881249999729, 6.242252689847871849, -8.218750002048354375 ) ) ;
#35348=CARTESIAN_POINT ( 'NONE',  ( -9.999999999999998224, 1.224646799147353059E-15, -111.1250000040967763 ) ) ;
#35349=CARTESIAN_POINT ( 'NONE',  ( -5.000000000000003553, -8.660254037844383745, -62.87500000409676204 ) ) ;
#35350=CARTESIAN_POINT ( 'NONE',  ( 5.000000000000000000, 8.660254037844385522, -175.7500000000000284 ) ) ;
#35352=CARTESIAN_POINT ( 'NONE',  ( -10.81189881249999729, 1.324075727343319199E-15, -99.78125000204839523 ) ) ;
#35353=ORIENTED_EDGE ( 'NONE', *, *, #31488, .F. ) ;
#35354=EDGE_CURVE ( 'NONE', #15394, #35065, #6246, .T. ) ;
#35357=VERTEX_POINT ( 'NONE', #1731 ) ;
#35358=CARTESIAN_POINT ( 'NONE',  ( 10.81189881249999729, 0.000000000000000000, -33.03125000204837391 ) ) ;
#35361=CARTESIAN_POINT ( 'NONE',  ( 5.405949406249992428, -9.363379034771808662, -82.59375000204836681 ) ) ;
#35362=CARTESIAN_POINT ( 'NONE',  ( 0.000000000000000000, 0.000000000000000000, -200.0000000000000000 ) ) ;
#35363=CARTESIAN_POINT ( 'NONE',  ( 5.405949406249999534, 9.363379034771803333, -197.5937500020484094 ) ) ;
#35364=( BOUNDED_CURVE ( )  B_SPLINE_CURVE ( 2, ( #2898, #25990, #36118, #6551, #32888, #23605, #10202 ),
 .UNSPECIFIED., .F., .F. ) 
 B_SPLINE_CURVE_WITH_KNOTS ( ( 3, 2, 2, 3 ),
 ( 0.5335820895522389584, 0.5348258706467662327, 0.5360696517412936180, 0.5373134328358210032 ),
 .UNSPECIFIED. ) 
 CURVE ( )  GEOMETRIC_REPRESENTATION_ITEM ( )  RATIONAL_B_SPLINE_CURVE ( ( 0.9999999999999880096, 0.8660254037844506980, 1.000000000000000000, 0.8660254037844387076, 1.000000000000000000, 0.8660254037844267172, 1.000000000000011990 ) ) 
 REPRESENTATION_ITEM ( '' )  );
#35365=DIRECTION ( 'NONE',  ( -0.000000000000000000, -0.000000000000000000, 1.000000000000000000 ) ) ;
#35366=CARTESIAN_POINT ( 'NONE',  ( 7.070501591499376803E-16, 11.54700538379251284, -30.50000000409674428 ) ) ;
#35368=CARTESIAN_POINT ( 'NONE',  ( -9.999999999999998224, 5.773502691896259087, -12.25000000409677092 ) ) ;
#35369=CARTESIAN_POINT ( 'NONE',  ( 9.999999999999998224, 0.000000000000000000, -76.99999999999998579 ) ) ;
#35370=CARTESIAN_POINT ( 'NONE',  ( -5.405949406250003975, -9.363379034771801557, -127.8437500020483952 ) ) ;
#35371=CARTESIAN_POINT ( 'NONE',  ( -10.81189881249999729, 1.324075727343319199E-15, -117.5937500020483810 ) ) ;
#35374=CARTESIAN_POINT ( 'NONE',  ( 10.00000000000000000, 5.773502691896255534, -170.2500000040967905 ) ) ;
#35375=CARTESIAN_POINT ( 'NONE',  ( 10.81189881249999729, 0.000000000000000000, -171.0312500020484094 ) ) ;
#35377=CARTESIAN_POINT ( 'NONE',  ( 0.000000000000000000, 0.000000000000000000, -200.0000000000000000 ) ) ;
#35380=CARTESIAN_POINT ( 'NONE',  ( -5.405949406249996869, 9.363379034771805109, -44.34375000204837391 ) ) ;
#35382=CARTESIAN_POINT ( 'NONE',  ( -10.81189881249999729, 6.242252689847871849, -3.906250002048350822 ) ) ;
#35384=DIRECTION ( 'NONE',  ( -0.000000000000000000, -0.000000000000000000, 1.000000000000000000 ) ) ;
#35386=EDGE_CURVE ( 'NONE', #24195, #39779, #28299, .T. ) ;
#35387=CARTESIAN_POINT ( 'NONE',  ( -2.121150477449813534E-15, -11.54700538379251284, -92.37500000000000000 ) ) ;
#35389=CARTESIAN_POINT ( 'NONE',  ( 4.999999999999992006, -8.660254037844389075, -101.6250000040967905 ) ) ;
#35390=LINE ( 'NONE', #22000, #5202 ) ;
#35392=CARTESIAN_POINT ( 'NONE',  ( -10.81189881249999729, 6.242252689847871849, -90.90625000204838102 ) ) ;
#35393=ORIENTED_EDGE ( 'NONE', *, *, #27477, .F. ) ;
#35395=CARTESIAN_POINT ( 'NONE',  ( 7.070501591499376803E-16, 11.54700538379251284, -72.12499999999995737 ) ) ;
#35396=CARTESIAN_POINT ( 'NONE',  ( -2.293366432827344421E-15, -12.48450537969573659, -159.4062500020483810 ) ) ;
#35399=CARTESIAN_POINT ( 'NONE',  ( -5.000000000000003553, -8.660254037844383745, -17.49999999999996092 ) ) ;
#35400=CARTESIAN_POINT ( 'NONE',  ( 10.81189881249999729, 6.242252689847867408, -23.90625000204838102 ) ) ;
#35401=CARTESIAN_POINT ( 'NONE',  ( -10.00000000000000000, -5.773502691896251982, -155.6249999999999716 ) ) ;
#35403=CARTESIAN_POINT ( 'NONE',  ( -4.999999999999996447, 8.660254037844387298, -198.0000000000000000 ) ) ;
#35404=CARTESIAN_POINT ( 'NONE',  ( 10.81189881249999729, 0.000000000000000000, -129.0312500020484094 ) ) ;
#35408=CARTESIAN_POINT ( 'NONE',  ( 5.405949406249992428, -9.363379034771808662, -55.78125000204836681 ) ) ;
#35410=CARTESIAN_POINT ( 'NONE',  ( 10.81189881249999551, -6.242252689847874514, -103.4687500020483810 ) ) ;
#35411=ORIENTED_EDGE ( 'NONE', *, *, #29931, .T. ) ;
#35412=ORIENTED_EDGE ( 'NONE', *, *, #24647, .F. ) ;
#35413=DIRECTION ( 'NONE',  ( -0.000000000000000000, -0.000000000000000000, 1.000000000000000000 ) ) ;
#35414=LINE ( 'NONE', #18574, #11109 ) ;
#35415=CARTESIAN_POINT ( 'NONE',  ( -5.405949406250003975, -9.363379034771801557, -156.3437500020483810 ) ) ;
#35417=CARTESIAN_POINT ( 'NONE',  ( 5.405949406249992428, -9.363379034771808662, -10.59375000204834727 ) ) ;
#35418=CYLINDRICAL_SURFACE ( 'NONE', #19032, 9.999999999999998224 ) ;
#35419=CARTESIAN_POINT ( 'NONE',  ( -10.81189881249999729, -6.242252689847864744, -139.9687500020483810 ) ) ;
#35421=CARTESIAN_POINT ( 'NONE',  ( 0.000000000000000000, 0.000000000000000000, -200.0000000000000000 ) ) ;
#35423=CARTESIAN_POINT ( 'NONE',  ( -9.999999999999998224, 5.773502691896259087, -196.7500000040968189 ) ) ;
#35425=CARTESIAN_POINT ( 'NONE',  ( 5.405949406249992428, -9.363379034771808662, -192.2812500020484094 ) ) ;
#35429=CARTESIAN_POINT ( 'NONE',  ( -10.81189881249999729, -6.242252689847864744, -69.46875000204838102 ) ) ;
#35430=CARTESIAN_POINT ( 'NONE',  ( -5.405949406250003975, -9.363379034771801557, -58.84375000204835970 ) ) ;
#35432=CARTESIAN_POINT ( 'NONE',  ( -10.81189881249999907, -6.242252689847864744, -26.15625000204837391 ) ) ;
#35434=LINE ( 'NONE', #12938, #8874 ) ;
#35437=CARTESIAN_POINT ( 'NONE',  ( -9.999999999999998224, 1.224646799147353059E-15, -110.7499999999999858 ) ) ;
#35438=CARTESIAN_POINT ( 'NONE',  ( -10.00000000000000000, -5.773502691896252870, -170.6249999999999716 ) ) ;
#35439=EDGE_CURVE ( 'NONE', #29342, #23818, #3216, .T. ) ;
#35442=CARTESIAN_POINT ( 'NONE',  ( 7.644554776091147741E-16, 12.48450537969573659, -13.15625000204836326 ) ) ;
#35443=ADVANCED_FACE ( 'NONE', ( #21568 ), #34749, .T. ) ;
#35444=EDGE_LOOP ( 'NONE', ( #35879, #23161, #9856, #27210 ) ) ;
#35445=CARTESIAN_POINT ( 'NONE',  ( 5.000000000000000000, 8.660254037844385522, -197.1250000040967905 ) ) ;
#35447=FACE_OUTER_BOUND ( 'NONE', #9982, .T. ) ;
#35449=CARTESIAN_POINT ( 'NONE',  ( 7.070501591499377789E-16, 11.54700538379251284, -40.62499999999997158 ) ) ;
#35450=CARTESIAN_POINT ( 'NONE',  ( -9.999999999999998224, 1.224646799147353059E-15, -28.62500000409676204 ) ) ;
#35451=CARTESIAN_POINT ( 'NONE',  ( 7.644554776091147741E-16, 12.48450537969573659, -55.15625000204837391 ) ) ;
#35452=( BOUNDED_CURVE ( )  B_SPLINE_CURVE ( 2, ( #34004, #7032, #37218, #19969, #23653, #7665, #30765 ),
 .UNSPECIFIED., .F., .F. ) 
 B_SPLINE_CURVE_WITH_KNOTS ( ( 3, 2, 2, 3 ),
 ( 0.2313432835820896372, 0.2325870646766169947, 0.2338308457711443245, 0.2350746268656717097 ),
 .UNSPECIFIED. ) 
 CURVE ( )  GEOMETRIC_REPRESENTATION_ITEM ( )  RATIONAL_B_SPLINE_CURVE ( ( 0.9999999999999910072, 0.8660254037844477004, 1.000000000000000000, 0.8660254037844387076, 1.000000000000000000, 0.8660254037844327124, 1.000000000000005995 ) ) 
 REPRESENTATION_ITEM ( '' )  );
#35456=CARTESIAN_POINT ( 'NONE',  ( -4.999999999999996447, 8.660254037844387298, -23.99999999999996447 ) ) ;
#35457=CARTESIAN_POINT ( 'NONE',  ( 10.81189881249999907, 6.242252689847868297, -145.4062500020484094 ) ) ;
#35458=CARTESIAN_POINT ( 'NONE',  ( 7.644554776091147741E-16, 12.48450537969573659, -149.6562500020484094 ) ) ;
#35460=ADVANCED_FACE ( 'NONE', ( #15708 ), #39448, .T. ) ;
#35463=VERTEX_POINT ( 'NONE', #32571 ) ;
#35465=EDGE_CURVE ( 'NONE', #29936, #5836, #9010, .T. ) ;
#35466=DIRECTION ( 'NONE',  ( 0.000000000000000000, 1.000000000000000000, 0.000000000000000000 ) ) ;
#35467=CARTESIAN_POINT ( 'NONE',  ( 5.405949406249992428, -9.363379034771808662, -183.0937500020483810 ) ) ;
#35468=CARTESIAN_POINT ( 'NONE',  ( 5.405949406249992428, -9.363379034771808662, -33.09375000204836681 ) ) ;
#35469=DIRECTION ( 'NONE',  ( -0.000000000000000000, -0.000000000000000000, 1.000000000000000000 ) ) ;
#35470=CARTESIAN_POINT ( 'NONE',  ( 10.81189881249999729, 6.242252689847867408, -163.2187500020483810 ) ) ;
#35471=CARTESIAN_POINT ( 'NONE',  ( -5.405949406250003975, -9.363379034771801557, -154.8437500020483810 ) ) ;
#35475=CARTESIAN_POINT ( 'NONE',  ( 5.405949406249992428, -9.363379034771808662, -18.09375000204835260 ) ) ;
#35477=CARTESIAN_POINT ( 'NONE',  ( 4.999999999999992006, -8.660254037844389075, -152.2500000000000000 ) ) ;
#35478=CARTESIAN_POINT ( 'NONE',  ( -9.999999999999804601, 5.773502691896371886, -177.2500000040967905 ) ) ;
#35480=CARTESIAN_POINT ( 'NONE',  ( 10.81189881249999907, 6.242252689847868297, -82.21875000204836681 ) ) ;
#35482=CARTESIAN_POINT ( 'NONE',  ( -2.293366432827344421E-15, -12.48450537969573659, -46.90625000204836681 ) ) ;
#35484=CARTESIAN_POINT ( 'NONE',  ( 4.999999999999992006, -8.660254037844389075, -16.12500000409675138 ) ) ;
#35486=CARTESIAN_POINT ( 'NONE',  ( -9.999999999999998224, 5.773502691896259087, -134.8750000000000000 ) ) ;
#35487=CARTESIAN_POINT ( 'NONE',  ( -5.405949406249996869, 9.363379034771805109, -148.0312500020483810 ) ) ;
#35490=CARTESIAN_POINT ( 'NONE',  ( -9.999999999999998224, 5.773502691896259087, -120.2500000040967763 ) ) ;
#35492=( BOUNDED_CURVE ( )  B_SPLINE_CURVE ( 2, ( #17161, #29721, #26475, #39838, #20202, #39622, #6830 ),
 .UNSPECIFIED., .F., .F. ) 
 B_SPLINE_CURVE_WITH_KNOTS ( ( 3, 2, 2, 3 ),
 ( 0.1865671641791045166, 0.1878109452736318741, 0.1890547263681592594, 0.1902985074626866169 ),
 .UNSPECIFIED. ) 
 CURVE ( )  GEOMETRIC_REPRESENTATION_ITEM ( )  RATIONAL_B_SPLINE_CURVE ( ( 0.9999999999999970024, 0.8660254037844417052, 1.000000000000000000, 0.8660254037844387076, 1.000000000000000000, 0.8660254037844327124, 1.000000000000005995 ) ) 
 REPRESENTATION_ITEM ( '' )  );
#35498=CARTESIAN_POINT ( 'NONE',  ( 5.405949406249992428, -9.363379034771808662, -172.7812500020484094 ) ) ;
#35499=CARTESIAN_POINT ( 'NONE',  ( 4.999999999999992006, -8.660254037844389075, -52.12500000409675494 ) ) ;
#35500=DIRECTION ( 'NONE',  ( -0.000000000000000000, -0.000000000000000000, 1.000000000000000000 ) ) ;
#35504=CARTESIAN_POINT ( 'NONE',  ( 5.405949406249992428, -9.363379034771808662, -169.7812500020484094 ) ) ;
#35506=CARTESIAN_POINT ( 'NONE',  ( -9.999999999999998224, 1.224646799147353059E-15, -64.24999999999997158 ) ) ;
#35508=CARTESIAN_POINT ( 'NONE',  ( -2.121150477449813534E-15, -11.54700538379251284, -52.25000000409676915 ) ) ;
#35509=EDGE_CURVE ( 'NONE', #12293, #29936, #41517, .T. ) ;
#35510=CYLINDRICAL_SURFACE ( 'NONE', #28264, 9.999999999999998224 ) ;
#35511=CARTESIAN_POINT ( 'NONE',  ( 10.81189881249999729, 0.000000000000000000, -79.53125000204838102 ) ) ;
#35514=CARTESIAN_POINT ( 'NONE',  ( -9.999999999999998224, 1.224646799147353059E-15, -119.7500000000000000 ) ) ;
#35516=ORIENTED_EDGE ( 'NONE', *, *, #34124, .F. ) ;
#35517=CARTESIAN_POINT ( 'NONE',  ( -2.293366432827344421E-15, -12.48450537969573659, -27.21875000204838102 ) ) ;
#35519=CARTESIAN_POINT ( 'NONE',  ( -5.405949406249996869, 9.363379034771805109, -7.031250002048378356 ) ) ;
#35520=CARTESIAN_POINT ( 'NONE',  ( 7.644554776091147741E-16, 12.48450537969573659, -54.96875000204836681 ) ) ;
#35521=VERTEX_POINT ( 'NONE', #2579 ) ;
#35522=CARTESIAN_POINT ( 'NONE',  ( -4.999999999999996447, 8.660254037844387298, -28.49999999999997158 ) ) ;
#35524=CARTESIAN_POINT ( 'NONE',  ( 10.81189881249999729, 6.242252689847867408, -185.7187500020484094 ) ) ;
#35525=CARTESIAN_POINT ( 'NONE',  ( -10.81189881249999907, -6.242252689847864744, -177.4687500020484094 ) ) ;
#35528=CARTESIAN_POINT ( 'NONE',  ( -4.999999999999996447, 8.660254037844387298, -40.87500000409677625 ) ) ;
#35531=CARTESIAN_POINT ( 'NONE',  ( -10.81189881249999907, -6.242252689847864744, -108.4687500020483810 ) ) ;
#35533=CARTESIAN_POINT ( 'NONE',  ( 10.81189881249999729, 0.000000000000000000, -72.03125000204838102 ) ) ;
#35534=CARTESIAN_POINT ( 'NONE',  ( 10.81189881249999729, 6.242252689847867408, -86.71875000204836681 ) ) ;
#35536=CARTESIAN_POINT ( 'NONE',  ( 10.00000000000000000, 5.773502691896255534, -147.7500000040967905 ) ) ;
#35538=VERTEX_POINT ( 'NONE', #35171 ) ;
#35541=FACE_OUTER_BOUND ( 'NONE', #24206, .T. ) ;
#35542=CARTESIAN_POINT ( 'NONE',  ( -9.999999999999998224, 1.224646799147353059E-15, -52.24999999999996447 ) ) ;
#35544=ORIENTED_EDGE ( 'NONE', *, *, #25190, .T. ) ;
#35545=CARTESIAN_POINT ( 'NONE',  ( -2.121150477449813534E-15, -11.54700538379251284, -65.37499999999998579 ) ) ;
#35547=CARTESIAN_POINT ( 'NONE',  ( -5.000000000000003553, -8.660254037844383745, -70.37500000409677625 ) ) ;
#35548=CARTESIAN_POINT ( 'NONE',  ( -9.999999999999998224, 1.224646799147353059E-15, -65.74999999999997158 ) ) ;
#35551=AXIS2_PLACEMENT_3D ( 'NONE', #19756, #33156, #39399 ) ;
#35552=CARTESIAN_POINT ( 'NONE',  ( -10.81189881249999729, -6.242252689847864744, -68.15625000204840944 ) ) ;
#35554=CARTESIAN_POINT ( 'NONE',  ( -9.999999999999998224, 1.224646799147353059E-15, -93.12500000409677625 ) ) ;
#35557=CARTESIAN_POINT ( 'NONE',  ( -10.81189881249999907, -6.242252689847864744, -191.1562500020484094 ) ) ;
#35558=EDGE_CURVE ( 'NONE', #30518, #2913, #18333, .T. ) ;
#35560=CARTESIAN_POINT ( 'NONE',  ( -5.405949406249996869, 9.363379034771805109, -3.843750002048368586 ) ) ;
#35561=CARTESIAN_POINT ( 'NONE',  ( -4.999999999999996447, 8.660254037844387298, -186.3750000040967905 ) ) ;
#35563=CARTESIAN_POINT ( 'NONE',  ( -9.999999999999998224, 1.224646799147353059E-15, -44.74999999999998579 ) ) ;
#35564=CARTESIAN_POINT ( 'NONE',  ( -9.999999999999998224, 1.224646799147353059E-15, -178.2500000000000284 ) ) ;
#35565=DIRECTION ( 'NONE',  ( -0.000000000000000000, -0.000000000000000000, 1.000000000000000000 ) ) ;
#35566=CARTESIAN_POINT ( 'NONE',  ( -2.293366432827344421E-15, -12.48450537969573659, -100.9062500020483952 ) ) ;
#35567=VERTEX_POINT ( 'NONE', #6023 ) ;
#35569=ORIENTED_EDGE ( 'NONE', *, *, #27910, .T. ) ;
#35570=ORIENTED_EDGE ( 'NONE', *, *, #6673, .T. ) ;
#35571=EDGE_CURVE ( 'NONE', #17005, #15077, #29676, .T. ) ;
#35572=CARTESIAN_POINT ( 'NONE',  ( -5.405949406250003975, -9.363379034771801557, -32.03125000204837391 ) ) ;
#35573=CARTESIAN_POINT ( 'NONE',  ( -10.81189881249999729, 1.324075727343319199E-15, -83.09375000204836681 ) ) ;
#35574=DIRECTION ( 'NONE',  ( -0.000000000000000000, -0.000000000000000000, 1.000000000000000000 ) ) ;
#35575=( BOUNDED_CURVE ( )  B_SPLINE_CURVE ( 2, ( #37879, #27957, #10892, #24511, #14110, #27099, #40241 ),
 .UNSPECIFIED., .F., .F. ) 
 B_SPLINE_CURVE_WITH_KNOTS ( ( 3, 2, 2, 3 ),
 ( 0.5522388059701495155, 0.5534825870646767898, 0.5547263681592041751, 0.5559701492537315604 ),
 .UNSPECIFIED. ) 
 CURVE ( )  GEOMETRIC_REPRESENTATION_ITEM ( )  RATIONAL_B_SPLINE_CURVE ( ( 0.9999999999999761302, 0.8660254037844625774, 1.000000000000000000, 0.8660254037844387076, 1.000000000000000000, 0.8660254037844148378, 1.000000000000023981 ) ) 
 REPRESENTATION_ITEM ( '' )  );
#35577=CARTESIAN_POINT ( 'NONE',  ( 9.999999999998969713, 5.773502691896851502, -30.75000000409672651 ) ) ;
#35579=CARTESIAN_POINT ( 'NONE',  ( 7.070501591499377789E-16, 11.54700538379251284, -14.00000000409676382 ) ) ;
#35580=CARTESIAN_POINT ( 'NONE',  ( 0.000000000000000000, 0.000000000000000000, -200.0000000000000000 ) ) ;
#35581=CARTESIAN_POINT ( 'NONE',  ( -2.293366432827344421E-15, -12.48450537969573659, -129.2187500020483810 ) ) ;
#35582=CARTESIAN_POINT ( 'NONE',  ( 7.644554776091147741E-16, 12.48450537969573659, -101.6562500020483952 ) ) ;
#35583=CARTESIAN_POINT ( 'NONE',  ( 10.81189881249999551, -6.242252689847874514, -119.9687500020483952 ) ) ;
#35584=AXIS2_PLACEMENT_3D ( 'NONE', #16688, #34193, #37187 ) ;
#35587=CARTESIAN_POINT ( 'NONE',  ( 5.000000000000000000, 8.660254037844385522, -170.1250000040968189 ) ) ;
#35588=FACE_OUTER_BOUND ( 'NONE', #22239, .T. ) ;
#35591=CARTESIAN_POINT ( 'NONE',  ( 10.81189881249999729, 0.000000000000000000, -44.84375000204837391 ) ) ;
#35593=CARTESIAN_POINT ( 'NONE',  ( 10.81189881249999907, 6.242252689847868297, -2.906250002048345937 ) ) ;
#35595=LINE ( 'NONE', #19173, #24061 ) ;
#35597=CARTESIAN_POINT ( 'NONE',  ( -2.121150477449813534E-15, -11.54700538379251284, -90.87499999999997158 ) ) ;
#35599=CARTESIAN_POINT ( 'NONE',  ( -10.00000000000000000, -5.773502691896251982, -96.00000000409679046 ) ) ;
#35600=DIRECTION ( 'NONE',  ( -0.000000000000000000, -0.000000000000000000, 1.000000000000000000 ) ) ;
#35602=CARTESIAN_POINT ( 'NONE',  ( 10.81189881249999729, 0.000000000000000000, -88.53125000204838102 ) ) ;
#35604=EDGE_CURVE ( 'NONE', #34874, #35982, #35595, .T. ) ;
#35609=CARTESIAN_POINT ( 'NONE',  ( -5.000000000000003553, -8.660254037844383745, -14.49999999999995737 ) ) ;
#35610=CARTESIAN_POINT ( 'NONE',  ( 5.405949406249992428, -9.363379034771808662, -22.78125000204836326 ) ) ;
#35611=CARTESIAN_POINT ( 'NONE',  ( 5.000000000000000000, 8.660254037844385522, -153.2500000000000000 ) ) ;
#35613=CARTESIAN_POINT ( 'NONE',  ( 5.000000000000000000, 8.660254037844385522, -195.2500000000000000 ) ) ;
#35614=CARTESIAN_POINT ( 'NONE',  ( 10.81189881249999551, -6.242252689847874514, -123.1562500020483952 ) ) ;
#35616=ORIENTED_EDGE ( 'NONE', *, *, #24908, .F. ) ;
#35617=( BOUNDED_CURVE ( )  B_SPLINE_CURVE ( 2, ( #262, #37124, #23981, #26575, #36494, #20722, #13593 ),
 .UNSPECIFIED., .F., .F. ) 
 B_SPLINE_CURVE_WITH_KNOTS ( ( 3, 2, 2, 3 ),
 ( 0.8134328358208956500, 0.8146766169154230353, 0.8159203980099504205, 0.8171641791044778058 ),
 .UNSPECIFIED. ) 
 CURVE ( )  GEOMETRIC_REPRESENTATION_ITEM ( )  RATIONAL_B_SPLINE_CURVE ( ( 0.9999999999999880096, 0.8660254037844506980, 1.000000000000000000, 0.8660254037844387076, 1.000000000000000000, 0.8660254037844148378, 1.000000000000023981 ) ) 
 REPRESENTATION_ITEM ( '' )  );
#35618=CARTESIAN_POINT ( 'NONE',  ( 10.81189881249999551, -6.242252689847874514, -51.15625000204838813 ) ) ;
#35620=CARTESIAN_POINT ( 'NONE',  ( 5.405949406249992428, -9.363379034771808662, -105.0937500020483810 ) ) ;
#35621=EDGE_CURVE ( 'NONE', #30674, #34637, #32362, .T. ) ;
#35623=ORIENTED_EDGE ( 'NONE', *, *, #20247, .T. ) ;
#35625=CARTESIAN_POINT ( 'NONE',  ( 5.000000000000000000, 8.660254037844385522, -144.6250000040967905 ) ) ;
#35626=CARTESIAN_POINT ( 'NONE',  ( 10.81189881249999907, 6.242252689847868297, -152.7187500020483810 ) ) ;
#35627=( BOUNDED_CURVE ( )  B_SPLINE_CURVE ( 2, ( #12295, #38640, #21600, #22448, #28731, #5422, #5633 ),
 .UNSPECIFIED., .F., .F. ) 
 B_SPLINE_CURVE_WITH_KNOTS ( ( 3, 2, 2, 3 ),
 ( 0.003731343283582092950, 0.004975124378109457846, 0.006218905472636822307, 0.007462686567164185901 ),
 .UNSPECIFIED. ) 
 CURVE ( )  GEOMETRIC_REPRESENTATION_ITEM ( )  RATIONAL_B_SPLINE_CURVE ( ( 0.9999999999999996669, 0.8660254037844390407, 1.000000000000000000, 0.8660254037844387076, 1.000000000000000000, 0.8660254037844379305, 1.000000000000000666 ) ) 
 REPRESENTATION_ITEM ( '' )  );
#35629=CARTESIAN_POINT ( 'NONE',  ( -10.81189881249999729, 6.242252689847871849, -11.21875000204836859 ) ) ;
#35631=CARTESIAN_POINT ( 'NONE',  ( 5.405949406249999534, 9.363379034771803333, -137.5937500020483810 ) ) ;
#35633=CARTESIAN_POINT ( 'NONE',  ( -9.999999999999998224, 1.224646799147353059E-15, -115.6250000040967905 ) ) ;
#35635=CARTESIAN_POINT ( 'NONE',  ( 7.070501591499377789E-16, 11.54700538379251284, -195.5000000040968189 ) ) ;
#35637=CARTESIAN_POINT ( 'NONE',  ( 5.405949406249992428, -9.363379034771808662, -189.2812500020484094 ) ) ;
#35641=CARTESIAN_POINT ( 'NONE',  ( 5.405949406249992428, -9.363379034771808662, -69.09375000204836681 ) ) ;
#35642=CARTESIAN_POINT ( 'NONE',  ( -5.405949406249996869, 9.363379034771805109, -50.34375000204835260 ) ) ;
#35644=CARTESIAN_POINT ( 'NONE',  ( -10.81189881249999907, -6.242252689847864744, -23.15625000204837747 ) ) ;
#35648=CARTESIAN_POINT ( 'NONE',  ( 9.999999999999998224, 0.000000000000000000, -114.4999999999999858 ) ) ;
#35649=CARTESIAN_POINT ( 'NONE',  ( 9.999999999999998224, 0.000000000000000000, -114.4999999999999858 ) ) ;
#35652=CARTESIAN_POINT ( 'NONE',  ( 10.81189881249999729, 0.000000000000000000, -112.5312500020483952 ) ) ;
#35654=CARTESIAN_POINT ( 'NONE',  ( -4.999999999999996447, 8.660254037844387298, -196.8750000040967905 ) ) ;
#35658=CARTESIAN_POINT ( 'NONE',  ( -9.999999999999998224, 5.773502691896259087, -43.37499999999997158 ) ) ;
#35659=CARTESIAN_POINT ( 'NONE',  ( 9.999999999999998224, 0.000000000000000000, -26.37500000409676204 ) ) ;
#35660=CARTESIAN_POINT ( 'NONE',  ( -10.81189881249999729, 6.242252689847871849, -42.90625000204838102 ) ) ;
#35661=CARTESIAN_POINT ( 'NONE',  ( 0.000000000000000000, 0.000000000000000000, -200.0000000000000000 ) ) ;
#35664=CARTESIAN_POINT ( 'NONE',  ( -10.00000000000025580, 5.773502691896109873, -156.2500000040968189 ) ) ;
#35665=CARTESIAN_POINT ( 'NONE',  ( -10.81189881249999729, 1.324075727343319199E-15, -138.7812500020483810 ) ) ;
#35666=CARTESIAN_POINT ( 'NONE',  ( -10.81189881249999907, -6.242252689847864744, -152.1562500020484094 ) ) ;
#35667=CARTESIAN_POINT ( 'NONE',  ( -4.999999999999996447, 8.660254037844387298, -59.99999999999997158 ) ) ;
#35668=CARTESIAN_POINT ( 'NONE',  ( -9.999999999999998224, 1.224646799147353059E-15, -124.2500000000000000 ) ) ;
#35670=EDGE_LOOP ( 'NONE', ( #41518, #11705, #13071, #32645 ) ) ;
#35671=EDGE_CURVE ( 'NONE', #33809, #40301, #17402, .T. ) ;
#35672=ORIENTED_EDGE ( 'NONE', *, *, #34605, .F. ) ;
#35674=CARTESIAN_POINT ( 'NONE',  ( -9.999999999999998224, 1.224646799147353059E-15, -117.1250000040967905 ) ) ;
#35675=CARTESIAN_POINT ( 'NONE',  ( -10.81189881249999729, 1.324075727343319199E-15, -170.0937500020484094 ) ) ;
#35676=CARTESIAN_POINT ( 'NONE',  ( -10.81189881249999907, -6.242252689847864744, -31.96875000204835970 ) ) ;
#35679=CARTESIAN_POINT ( 'NONE',  ( -5.405949406249996869, 9.363379034771805109, -167.3437500020484094 ) ) ;
#35680=CARTESIAN_POINT ( 'NONE',  ( -10.81189881249999907, -6.242252689847864744, -148.9687500020484094 ) ) ;
#35684=CARTESIAN_POINT ( 'NONE',  ( -2.293366432827344421E-15, -12.48450537969573659, -16.71875000204836326 ) ) ;
#35686=CARTESIAN_POINT ( 'NONE',  ( 5.000000000000000000, 8.660254037844385522, -135.2499999999999716 ) ) ;
#35689=CARTESIAN_POINT ( 'NONE',  ( -10.81189881249999729, 1.324075727343319199E-15, -69.59375000204836681 ) ) ;
#35690=CARTESIAN_POINT ( 'NONE',  ( 5.405949406249999534, 9.363379034771803333, -52.28125000204835970 ) ) ;
#35694=CARTESIAN_POINT ( 'NONE',  ( 9.999999999999996447, -5.773502691896262640, -134.1250000000000000 ) ) ;
#35695=CARTESIAN_POINT ( 'NONE',  ( -2.293366432827344421E-15, -12.48450537969573659, -148.9062500020484379 ) ) ;
#35696=( BOUNDED_CURVE ( )  B_SPLINE_CURVE ( 2, ( #34056, #40710, #23919, #17620, #411, #7936, #29969 ),
 .UNSPECIFIED., .F., .F. ) 
 B_SPLINE_CURVE_WITH_KNOTS ( ( 3, 2, 2, 3 ),
 ( 0.4179104477611941260, 0.4191542288557215112, 0.4203980099502488965, 0.4216417910447762818 ),
 .UNSPECIFIED. ) 
 CURVE ( )  GEOMETRIC_REPRESENTATION_ITEM ( )  RATIONAL_B_SPLINE_CURVE ( ( 0.9999999999999880096, 0.8660254037844506980, 1.000000000000000000, 0.8660254037844387076, 1.000000000000000000, 0.8660254037844207220, 1.000000000000017986 ) ) 
 REPRESENTATION_ITEM ( '' )  );
#35697=CARTESIAN_POINT ( 'NONE',  ( -4.999999999999996447, 8.660254037844387298, -15.37500000409675138 ) ) ;
#35698=CARTESIAN_POINT ( 'NONE',  ( 5.000000000000000000, 8.660254037844385522, -125.1250000040967620 ) ) ;
#35703=CARTESIAN_POINT ( 'NONE',  ( 9.999999999998969713, 5.773502691896851502, -52.87499999999995737 ) ) ;
#35704=CARTESIAN_POINT ( 'NONE',  ( -10.81189881249999729, 6.242252689847871849, -168.9062500020483810 ) ) ;
#35705=CARTESIAN_POINT ( 'NONE',  ( 7.070501591499377789E-16, 11.54700538379251284, -48.50000000409676915 ) ) ;
#35709=CARTESIAN_POINT ( 'NONE',  ( 10.81189881249999907, 6.242252689847868297, -164.9062500020484094 ) ) ;
#35710=CARTESIAN_POINT ( 'NONE',  ( -2.293366432827344421E-15, -12.48450537969573659, -141.2187500020483810 ) ) ;
#35711=AXIS2_PLACEMENT_3D ( 'NONE', #10755, #37091, #11185 ) ;
#35712=LINE ( 'NONE', #9993, #29102 ) ;
#35713=CARTESIAN_POINT ( 'NONE',  ( 7.070501591499376803E-16, 11.54700538379251284, -80.00000000409677625 ) ) ;
#35715=VERTEX_POINT ( 'NONE', #10298 ) ;
#35716=CARTESIAN_POINT ( 'NONE',  ( 5.405949406249999534, 9.363379034771803333, -68.78125000204838102 ) ) ;
#35719=EDGE_CURVE ( 'NONE', #22184, #8341, #38498, .T. ) ;
#35720=CARTESIAN_POINT ( 'NONE',  ( -10.00000000000154188, 5.773502691895366468, -29.87499999999990763 ) ) ;
#35721=ORIENTED_EDGE ( 'NONE', *, *, #15405, .T. ) ;
#35723=EDGE_CURVE ( 'NONE', #27003, #10661, #30389, .T. ) ;
#35724=CARTESIAN_POINT ( 'NONE',  ( -10.81189881249999729, 1.324075727343319199E-15, -29.09375000204836326 ) ) ;
#35725=CARTESIAN_POINT ( 'NONE',  ( 9.999999999999998224, 0.000000000000000000, -108.4999999999999858 ) ) ;
#35726=CARTESIAN_POINT ( 'NONE',  ( -5.405949406249996869, 9.363379034771805109, -2.531250002048373915 ) ) ;
#35727=CARTESIAN_POINT ( 'NONE',  ( 10.81189881249999729, 0.000000000000000000, -56.84375000204835970 ) ) ;
#35731=CARTESIAN_POINT ( 'NONE',  ( -5.405949406250003975, -9.363379034771801557, -187.8437500020483810 ) ) ;
#35732=CARTESIAN_POINT ( 'NONE',  ( 5.405949406249999534, 9.363379034771803333, -167.5937500020484094 ) ) ;
#35740=CARTESIAN_POINT ( 'NONE',  ( -5.405949406249996869, 9.363379034771805109, -104.3437500020483810 ) ) ;
#35741=DIRECTION ( 'NONE',  ( -0.000000000000000000, -0.000000000000000000, 1.000000000000000000 ) ) ;
#35742=CARTESIAN_POINT ( 'NONE',  ( -10.81189881249999729, 1.324075727343319199E-15, -71.28125000204838102 ) ) ;
#35743=CARTESIAN_POINT ( 'NONE',  ( -9.999999999999998224, 1.224646799147353059E-15, -160.2500000000000000 ) ) ;
#35744=CARTESIAN_POINT ( 'NONE',  ( -10.81189881249999729, 1.324075727343319199E-15, -81.59375000204838102 ) ) ;
#35747=CARTESIAN_POINT ( 'NONE',  ( -9.999999999999998224, 5.773502691896259087, -142.7500000040967905 ) ) ;
#35750=ORIENTED_EDGE ( 'NONE', *, *, #31975, .T. ) ;
#35753=CARTESIAN_POINT ( 'NONE',  ( 10.81189881249999729, 0.000000000000000000, -193.5312500020484094 ) ) ;
#35757=CARTESIAN_POINT ( 'NONE',  ( -9.999999999999998224, 1.224646799147353059E-15, -59.74999999999997158 ) ) ;
#35759=CARTESIAN_POINT ( 'NONE',  ( -10.00000000000000000, -5.773502691896251982, -75.00000000409677625 ) ) ;
#35761=CARTESIAN_POINT ( 'NONE',  ( -9.999999999999479527, -5.773502691896549521, -145.1250000000000000 ) ) ;
#35763=CARTESIAN_POINT ( 'NONE',  ( 10.81189881249999729, 0.000000000000000000, -69.03125000204838102 ) ) ;
#35767=CARTESIAN_POINT ( 'NONE',  ( 10.81189881249999907, 6.242252689847868297, -196.4062500020484379 ) ) ;
#35769=CARTESIAN_POINT ( 'NONE',  ( 10.81189881249999551, -6.242252689847874514, -1.468750002048354819 ) ) ;
#35770=DIRECTION ( 'NONE',  ( -0.000000000000000000, -0.000000000000000000, 1.000000000000000000 ) ) ;
#35771=FACE_OUTER_BOUND ( 'NONE', #41722, .T. ) ;
#35772=CARTESIAN_POINT ( 'NONE',  ( -23.09401076758503280, 0.000000000000000000, 45.00000000000009237 ) ) ;
#35773=CARTESIAN_POINT ( 'NONE',  ( 7.070501591499377789E-16, 11.54700538379251284, -171.1250000000000000 ) ) ;
#35775=CARTESIAN_POINT ( 'NONE',  ( -2.293366432827344421E-15, -12.48450537969573659, -105.4062500020483810 ) ) ;
#35776=ORIENTED_EDGE ( 'NONE', *, *, #5401, .F. ) ;
#35778=ORIENTED_EDGE ( 'NONE', *, *, #7449, .T. ) ;
#35779=EDGE_LOOP ( 'NONE', ( #3608, #5945, #6356, #24689 ) ) ;
#35780=CARTESIAN_POINT ( 'NONE',  ( 5.405949406249999534, 9.363379034771803333, -32.59375000204836681 ) ) ;
#35781=CARTESIAN_POINT ( 'NONE',  ( 10.81189881249999907, 6.242252689847868297, -29.90625000204836326 ) ) ;
#35783=AXIS2_PLACEMENT_3D ( 'NONE', #36426, #30600, #13316 ) ;
#35784=CARTESIAN_POINT ( 'NONE',  ( 5.405949406249999534, 9.363379034771803333, -80.59375000204838102 ) ) ;
#35786=CARTESIAN_POINT ( 'NONE',  ( -2.293366432827344421E-15, -12.48450537969573659, -198.2187500020484379 ) ) ;
#35790=CARTESIAN_POINT ( 'NONE',  ( -2.121150477449813534E-15, -11.54700538379251284, -8.750000004096753159 ) ) ;
#35791=CARTESIAN_POINT ( 'NONE',  ( -9.999999999999998224, 1.224646799147353059E-15, -103.6250000040967763 ) ) ;
#35792=EDGE_CURVE ( 'NONE', #41070, #41327, #17806, .T. ) ;
#35793=CARTESIAN_POINT ( 'NONE',  ( -10.81189881249999729, 1.324075727343319199E-15, -129.5937500020483810 ) ) ;
#35794=CARTESIAN_POINT ( 'NONE',  ( -10.81189881249999729, 6.242252689847871849, -99.90625000204838102 ) ) ;
#35795=CARTESIAN_POINT ( 'NONE',  ( -2.293366432827344421E-15, -12.48450537969573659, -108.2187500020483668 ) ) ;
#35798=CARTESIAN_POINT ( 'NONE',  ( -9.999999999999998224, 5.773502691896259087, -172.7500000040967905 ) ) ;
#35799=CARTESIAN_POINT ( 'NONE',  ( 0.000000000000000000, 0.000000000000000000, -200.0000000000000000 ) ) ;
#35805=CARTESIAN_POINT ( 'NONE',  ( 9.999999999999998224, 0.000000000000000000, -59.37500000409676204 ) ) ;
#35807=CARTESIAN_POINT ( 'NONE',  ( 10.00000000000000000, 5.773502691896255534, -87.37499999999998579 ) ) ;
#35809=CARTESIAN_POINT ( 'NONE',  ( -9.999999999999998224, 5.773502691896259087, -97.75000000409677625 ) ) ;
#35810=CYLINDRICAL_SURFACE ( 'NONE', #27213, 9.999999999999998224 ) ;
#35812=CARTESIAN_POINT ( 'NONE',  ( -10.81189881249999729, 6.242252689847871849, -93.90625000204838102 ) ) ;
#35817=ORIENTED_EDGE ( 'NONE', *, *, #31517, .T. ) ;
#35818=CARTESIAN_POINT ( 'NONE',  ( -9.999999999999998224, 1.224646799147353059E-15, -16.24999999999995737 ) ) ;
#35819=VECTOR ( 'NONE', #38731, 1000.000000000000000 ) ;
#35820=CARTESIAN_POINT ( 'NONE',  ( -10.00000000000000000, -5.773502691896251982, -154.1250000000000284 ) ) ;
#35823=CARTESIAN_POINT ( 'NONE',  ( 10.81189881249999551, -6.242252689847874514, -129.1562500020483810 ) ) ;
#35825=CARTESIAN_POINT ( 'NONE',  ( -10.00000000000051337, 5.773502691895962435, -89.87499999999998579 ) ) ;
#35827=ORIENTED_EDGE ( 'NONE', *, *, #23291, .T. ) ;
#35828=CARTESIAN_POINT ( 'NONE',  ( -5.405949406249996869, 9.363379034771805109, -55.03125000204836681 ) ) ;
#35830=CARTESIAN_POINT ( 'NONE',  ( 5.405949406249992428, -9.363379034771808662, -100.5937500020483810 ) ) ;
#35832=ORIENTED_EDGE ( 'NONE', *, *, #28465, .F. ) ;
#35833=CARTESIAN_POINT ( 'NONE',  ( -9.999999999999998224, 1.224646799147353059E-15, -77.74999999999998579 ) ) ;
#35835=CARTESIAN_POINT ( 'NONE',  ( -5.405949406249996869, 9.363379034771805109, -2.343750002048366810 ) ) ;
#35837=AXIS2_PLACEMENT_3D ( 'NONE', #9432, #39415, #38569 ) ;
#35838=CARTESIAN_POINT ( 'NONE',  ( 10.81189881249999729, 6.242252689847867408, -128.7187500020483810 ) ) ;
#35840=CARTESIAN_POINT ( 'NONE',  ( 9.999999999999742428, 5.773502691896404748, -116.2500000040967620 ) ) ;
#35842=CARTESIAN_POINT ( 'NONE',  ( 9.999999999999998224, 0.000000000000000000, -197.3750000040967905 ) ) ;
#35844=CARTESIAN_POINT ( 'NONE',  ( -5.405949406249996869, 9.363379034771805109, -184.0312500020484094 ) ) ;
#35845=DIRECTION ( 'NONE',  ( -0.5000000000000003331, 0.8660254037844383745, 0.000000000000000000 ) ) ;
#35848=CARTESIAN_POINT ( 'NONE',  ( 10.81189881249999729, 0.000000000000000000, -65.84375000204836681 ) ) ;
#35849=CARTESIAN_POINT ( 'NONE',  ( 10.81189881249999729, 0.000000000000000000, -47.84375000204838102 ) ) ;
#35851=CARTESIAN_POINT ( 'NONE',  ( 5.405949406249992428, -9.363379034771808662, -24.28125000204836681 ) ) ;
#35855=CARTESIAN_POINT ( 'NONE',  ( 9.999999999999996447, -5.773502691896262640, -110.1250000000000000 ) ) ;
#35856=CARTESIAN_POINT ( 'NONE',  ( 9.999999999999742428, 5.773502691896404748, -163.8750000000000284 ) ) ;
#35859=CARTESIAN_POINT ( 'NONE',  ( -10.81189881249999729, -6.242252689847864744, -113.1562500020483952 ) ) ;
#35860=EDGE_CURVE ( 'NONE', #39730, #30625, #22243, .T. ) ;
#35861=ORIENTED_EDGE ( 'NONE', *, *, #8579, .T. ) ;
#35862=CARTESIAN_POINT ( 'NONE',  ( -9.999999999999998224, 1.224646799147353059E-15, -160.6250000040967905 ) ) ;
#35864=DIRECTION ( 'NONE',  ( 0.5000000000000007772, -0.8660254037844381525, -0.000000000000000000 ) ) ;
#35866=VERTEX_POINT ( 'NONE', #20649 ) ;
#35867=CARTESIAN_POINT ( 'NONE',  ( -10.00000000000000000, -5.773502691896251982, -41.62499999999997158 ) ) ;
#35868=CARTESIAN_POINT ( 'NONE',  ( 4.999999999999992006, -8.660254037844389075, -19.12500000409675494 ) ) ;
#35869=CARTESIAN_POINT ( 'NONE',  ( -10.81189881249999729, 1.324075727343319199E-15, -42.78125000204838102 ) ) ;
#35872=( BOUNDED_CURVE ( )  B_SPLINE_CURVE ( 2, ( #42417, #22584, #9418, #13056, #38777, #3369, #42207 ),
 .UNSPECIFIED., .F., .F. ) 
 B_SPLINE_CURVE_WITH_KNOTS ( ( 3, 2, 2, 3 ),
 ( 0.9253731343283585487, 0.9266169154228859339, 0.9278606965174133192, 0.9291044776119405935 ),
 .UNSPECIFIED. ) 
 CURVE ( )  GEOMETRIC_REPRESENTATION_ITEM ( )  RATIONAL_B_SPLINE_CURVE ( ( 0.9999999999999641398, 0.8660254037844745678, 1.000000000000000000, 0.8660254037844387076, 1.000000000000000000, 0.8660254037844028474, 1.000000000000035971 ) ) 
 REPRESENTATION_ITEM ( '' )  );
#35873=DIRECTION ( 'NONE',  ( -0.000000000000000000, -0.000000000000000000, 1.000000000000000000 ) ) ;
#35874=CARTESIAN_POINT ( 'NONE',  ( -10.81189881249999729, 6.242252689847871849, -137.4062500020484094 ) ) ;
#35875=CARTESIAN_POINT ( 'NONE',  ( 5.405949406249999534, 9.363379034771803333, -151.2812500020484094 ) ) ;
#35877=VERTEX_POINT ( 'NONE', #40078 ) ;
#35878=( BOUNDED_CURVE ( )  B_SPLINE_CURVE ( 2, ( #12380, #22329, #5931, #5290, #19082, #41534, #29021 ),
 .UNSPECIFIED., .F., .F. ) 
 B_SPLINE_CURVE_WITH_KNOTS ( ( 3, 2, 2, 3 ),
 ( 0.07462686567164185381, 0.07587064676616922521, 0.07711442786069658273, 0.07835820895522395413 ),
 .UNSPECIFIED. ) 
 CURVE ( )  GEOMETRIC_REPRESENTATION_ITEM ( )  RATIONAL_B_SPLINE_CURVE ( ( 0.9999999999999925615, 0.8660254037844461461, 1.000000000000000000, 0.8660254037844387076, 1.000000000000000000, 0.8660254037844312691, 1.000000000000007550 ) ) 
 REPRESENTATION_ITEM ( '' )  );
#35879=ORIENTED_EDGE ( 'NONE', *, *, #18294, .F. ) ;
#35881=CARTESIAN_POINT ( 'NONE',  ( 7.644554776091147741E-16, 12.48450537969573659, -174.9687500020484094 ) ) ;
#35882=CARTESIAN_POINT ( 'NONE',  ( 10.81189881249999907, 6.242252689847868297, -22.21875000204837036 ) ) ;
#35883=CARTESIAN_POINT ( 'NONE',  ( -9.999999999999998224, 1.224646799147353059E-15, -61.62500000409676204 ) ) ;
#35884=CARTESIAN_POINT ( 'NONE',  ( -10.81189881249999729, 6.242252689847871849, -161.2187500020483810 ) ) ;
#35885=CARTESIAN_POINT ( 'NONE',  ( 5.405949406249999534, 9.363379034771803333, -142.0937500020483810 ) ) ;
#35889=CARTESIAN_POINT ( 'NONE',  ( 5.405949406249992428, -9.363379034771808662, -15.09375000204835082 ) ) ;
#35892=DIRECTION ( 'NONE',  ( -0.000000000000000000, -0.000000000000000000, 1.000000000000000000 ) ) ;
#35894=CARTESIAN_POINT ( 'NONE',  ( -10.00000000000000000, -5.773502691896252870, -168.0000000040968189 ) ) ;
#35895=VECTOR ( 'NONE', #42013, 1000.000000000000000 ) ;
#35896=CARTESIAN_POINT ( 'NONE',  ( 5.405949406249999534, 9.363379034771803333, -76.09375000204838102 ) ) ;
#35897=CARTESIAN_POINT ( 'NONE',  ( 10.81189881249999551, -6.242252689847874514, -51.15625000204838813 ) ) ;
#35901=CARTESIAN_POINT ( 'NONE',  ( -10.00000000000000000, -5.773502691896251982, -139.1250000000000000 ) ) ;
#35902=CARTESIAN_POINT ( 'NONE',  ( -5.405949406249996869, 9.363379034771805109, -139.0312500020484094 ) ) ;
#35904=CARTESIAN_POINT ( 'NONE',  ( -9.999999999999998224, 5.773502691896259087, -114.2500000040967905 ) ) ;
#35906=VERTEX_POINT ( 'NONE', #10509 ) ;
#35909=FACE_OUTER_BOUND ( 'NONE', #15781, .T. ) ;
#35910=CARTESIAN_POINT ( 'NONE',  ( 5.405949406249999534, 9.363379034771803333, -175.2812500020484094 ) ) ;
#35911=CARTESIAN_POINT ( 'NONE',  ( -9.999999999999998224, 1.224646799147353059E-15, -40.62500000409677625 ) ) ;
#35915=CARTESIAN_POINT ( 'NONE',  ( -10.00000000000051337, 5.773502691895962435, -73.37499999999995737 ) ) ;
#35916=CARTESIAN_POINT ( 'NONE',  ( 5.405949406249992428, -9.363379034771808662, -159.2812500020484094 ) ) ;
#35917=CARTESIAN_POINT ( 'NONE',  ( -5.405949406249996869, 9.363379034771805109, -140.3437500020484094 ) ) ;
#35918=ORIENTED_EDGE ( 'NONE', *, *, #22174, .T. ) ;
#35919=CARTESIAN_POINT ( 'NONE',  ( 10.00000000000154010, -5.773502691895370020, -30.62499999999991118 ) ) ;
#35921=CARTESIAN_POINT ( 'NONE',  ( 10.81189881249999551, -6.242252689847874514, -70.65625000204839523 ) ) ;
#35923=CARTESIAN_POINT ( 'NONE',  ( -5.405949406250003975, -9.363379034771801557, -121.8437500020483952 ) ) ;
#35924=EDGE_LOOP ( 'NONE', ( #40834, #17211, #29777, #36581 ) ) ;
#35925=EDGE_LOOP ( 'NONE', ( #20499, #11210, #6416, #15472 ) ) ;
#35926=CARTESIAN_POINT ( 'NONE',  ( 10.81189881249999729, 6.242252689847867408, -26.71875000204837391 ) ) ;
#35927=CARTESIAN_POINT ( 'NONE',  ( -10.81189881249999729, 6.242252689847871849, -0.9062500020483681418 ) ) ;
#35928=CARTESIAN_POINT ( 'NONE',  ( -2.293366432827344421E-15, -12.48450537969573659, -45.21875000204836681 ) ) ;
#35930=CARTESIAN_POINT ( 'NONE',  ( -10.81189881249999729, -6.242252689847864744, -190.9687500020484094 ) ) ;
#35931=CARTESIAN_POINT ( 'NONE',  ( 10.81189881249999551, -6.242252689847874514, -172.4687500020484094 ) ) ;
#35932=( BOUNDED_CURVE ( )  B_SPLINE_CURVE ( 2, ( #9088, #18369, #11886, #25294, #35216, #25082, #8881 ),
 .UNSPECIFIED., .F., .F. ) 
 B_SPLINE_CURVE_WITH_KNOTS ( ( 3, 2, 2, 3 ),
 ( 0.9589552238805971740, 0.9601990049751244483, 0.9614427860696519446, 0.9626865671641793298 ),
 .UNSPECIFIED. ) 
 CURVE ( )  GEOMETRIC_REPRESENTATION_ITEM ( )  RATIONAL_B_SPLINE_CURVE ( ( 0.9999999999999880096, 0.8660254037844506980, 1.000000000000000000, 0.8660254037844387076, 1.000000000000000000, 0.8660254037844148378, 1.000000000000023981 ) ) 
 REPRESENTATION_ITEM ( '' )  );
#35935=CARTESIAN_POINT ( 'NONE',  ( -10.00000000000102496, 5.773502691895664007, -40.75000000409673362 ) ) ;
#35936=CARTESIAN_POINT ( 'NONE',  ( 9.999999999998456346, 5.773502691897149042, -20.25000000409673717 ) ) ;
#35938=CARTESIAN_POINT ( 'NONE',  ( -10.81189881249999729, 1.324075727343319199E-15, -96.59375000204838102 ) ) ;
#35939=CARTESIAN_POINT ( 'NONE',  ( -9.999999999998969713, -5.773502691896847949, -85.12499999999995737 ) ) ;
#35940=CARTESIAN_POINT ( 'NONE',  ( 10.81189881249999907, 6.242252689847868297, -76.40625000204839523 ) ) ;
#35941=CARTESIAN_POINT ( 'NONE',  ( -5.000000000000003553, -8.660254037844383745, -160.0000000000000000 ) ) ;
#35943=CARTESIAN_POINT ( 'NONE',  ( -10.81189881249999729, 6.242252689847871849, -81.71875000204838102 ) ) ;
#35945=CARTESIAN_POINT ( 'NONE',  ( -5.000000000000003553, -8.660254037844383745, -134.8750000040967905 ) ) ;
#35947=VECTOR ( 'NONE', #39062, 1000.000000000000000 ) ;
#35952=CARTESIAN_POINT ( 'NONE',  ( 10.81189881249999907, 6.242252689847868297, -197.9062500020484379 ) ) ;
#35953=CARTESIAN_POINT ( 'NONE',  ( 10.00000000000102318, -5.773502691895667560, -38.12499999999992184 ) ) ;
#35955=ORIENTED_EDGE ( 'NONE', *, *, #23459, .T. ) ;
#35956=CARTESIAN_POINT ( 'NONE',  ( -4.999999999999996447, 8.660254037844387298, -55.49999999999996447 ) ) ;
#35958=CARTESIAN_POINT ( 'NONE',  ( -4.999999999999996447, 8.660254037844387298, -76.87500000409677625 ) ) ;
#35959=ADVANCED_FACE ( 'NONE', ( #33836 ), #1029, .T. ) ;
#35960=CARTESIAN_POINT ( 'NONE',  ( -4.999999999999996447, 8.660254037844387298, -65.99999999999997158 ) ) ;
#35961=FACE_OUTER_BOUND ( 'NONE', #33901, .T. ) ;
#35962=ADVANCED_FACE ( 'NONE', ( #195 ), #26505, .T. ) ;
#35964=CARTESIAN_POINT ( 'NONE',  ( -10.81189881249999729, -6.242252689847864744, -71.15625000204839523 ) ) ;
#35965=ADVANCED_FACE ( 'NONE', ( #1674 ), #31671, .T. ) ;
#35968=DIRECTION ( 'NONE',  ( -0.000000000000000000, -0.000000000000000000, 1.000000000000000000 ) ) ;
#35969=CARTESIAN_POINT ( 'NONE',  ( 5.405949406249999534, 9.363379034771803333, -187.2812500020484094 ) ) ;
#35972=CARTESIAN_POINT ( 'NONE',  ( 7.070501591499376803E-16, 11.54700538379251284, -186.5000000040968189 ) ) ;
#35975=CARTESIAN_POINT ( 'NONE',  ( -9.999999999999998224, 1.224646799147353059E-15, -124.6250000040967763 ) ) ;
#35976=CARTESIAN_POINT ( 'NONE',  ( -10.00000000000000000, -5.773502691896251982, -166.1249999999999716 ) ) ;
#35977=CARTESIAN_POINT ( 'NONE',  ( 10.81189881249999729, 0.000000000000000000, -93.03125000204838102 ) ) ;
#35978=VERTEX_POINT ( 'NONE', #24988 ) ;
#35982=VERTEX_POINT ( 'NONE', #34049 ) ;
#35983=ORIENTED_EDGE ( 'NONE', *, *, #30362, .F. ) ;
#35984=( BOUNDED_CURVE ( )  B_SPLINE_CURVE ( 2, ( #20865, #28434, #12626, #12209, #26032, #35953, #25198 ),
 .UNSPECIFIED., .F., .F. ) 
 B_SPLINE_CURVE_WITH_KNOTS ( ( 3, 2, 2, 3 ),
 ( 0.8022388059701494045, 0.8034825870646766788, 0.8047263681592041751, 0.8059701492537315604 ),
 .UNSPECIFIED. ) 
 CURVE ( )  GEOMETRIC_REPRESENTATION_ITEM ( )  RATIONAL_B_SPLINE_CURVE ( ( 0.9999999999999880096, 0.8660254037844506980, 1.000000000000000000, 0.8660254037844387076, 1.000000000000000000, 0.8660254037844148378, 1.000000000000023981 ) ) 
 REPRESENTATION_ITEM ( '' )  );
#35985=CARTESIAN_POINT ( 'NONE',  ( 5.405949406249992428, -9.363379034771808662, -37.59375000204837391 ) ) ;
#35986=CARTESIAN_POINT ( 'NONE',  ( 5.405949406249999534, 9.363379034771803333, -23.78125000204836681 ) ) ;
#35988=EDGE_CURVE ( 'NONE', #10458, #6, #22748, .T. ) ;
#35989=CARTESIAN_POINT ( 'NONE',  ( -10.81189881249999729, 6.242252689847871849, -75.71875000204836681 ) ) ;
#35990=CARTESIAN_POINT ( 'NONE',  ( -9.999999999999998224, 1.224646799147353059E-15, -174.1250000040968189 ) ) ;
#35991=CARTESIAN_POINT ( 'NONE',  ( 10.81189881249999551, -6.242252689847874514, -196.4687500020484094 ) ) ;
#35992=CARTESIAN_POINT ( 'NONE',  ( -10.00000000000051337, 5.773502691895962435, -72.25000000409674783 ) ) ;
#35993=CARTESIAN_POINT ( 'NONE',  ( -2.121150477449813534E-15, -11.54700538379251284, -143.7500000040967905 ) ) ;
#35995=CARTESIAN_POINT ( 'NONE',  ( -10.00000000000000000, -5.773502691896251982, -6.000000004096739836 ) ) ;
#35997=CARTESIAN_POINT ( 'NONE',  ( 7.644554776091147741E-16, 12.48450537969573659, -117.9687500020483668 ) ) ;
#35998=CARTESIAN_POINT ( 'NONE',  ( 7.644554776091147741E-16, 12.48450537969573659, -100.1562500020483952 ) ) ;
#35999=CARTESIAN_POINT ( 'NONE',  ( 10.81189881249999729, 6.242252689847867408, -104.7187500020483810 ) ) ;
#36000=EDGE_CURVE ( 'NONE', #4655, #22659, #11359, .T. ) ;
#36003=CARTESIAN_POINT ( 'NONE',  ( 4.999999999999992006, -8.660254037844389075, -169.1250000040967905 ) ) ;
#36007=FACE_OUTER_BOUND ( 'NONE', #36665, .T. ) ;
#36009=CARTESIAN_POINT ( 'NONE',  ( -5.000000000000003553, -8.660254037844383745, -59.87500000409676204 ) ) ;
#36011=CARTESIAN_POINT ( 'NONE',  ( 5.000000000000000000, 8.660254037844385522, -84.24999999999997158 ) ) ;
#36013=CARTESIAN_POINT ( 'NONE',  ( 4.999999999999992006, -8.660254037844389075, -95.62500000409677625 ) ) ;
#36014=CARTESIAN_POINT ( 'NONE',  ( -9.999999999999998224, 1.224646799147353059E-15, -200.0000000000000000 ) ) ;
#36016=CARTESIAN_POINT ( 'NONE',  ( -10.81189881249999729, -6.242252689847864744, -89.15625000204836681 ) ) ;
#36017=VERTEX_POINT ( 'NONE', #27782 ) ;
#36018=AXIS2_PLACEMENT_3D ( 'NONE', #34728, #20895, #14403 ) ;
#36020=DIRECTION ( 'NONE',  ( -0.000000000000000000, -0.000000000000000000, 1.000000000000000000 ) ) ;
#36022=ORIENTED_EDGE ( 'NONE', *, *, #34605, .T. ) ;
#36023=CARTESIAN_POINT ( 'NONE',  ( 7.070501591499377789E-16, 11.54700538379251284, -12.12499999999996270 ) ) ;
#36024=CARTESIAN_POINT ( 'NONE',  ( -5.000000000000003553, -8.660254037844383745, -145.0000000000000000 ) ) ;
#36026=AXIS2_PLACEMENT_3D ( 'NONE', #42524, #9312, #12949 ) ;
#36027=CARTESIAN_POINT ( 'NONE',  ( 9.999999999999996447, -5.773502691896262640, -198.6250000000000284 ) ) ;
#36028=ADVANCED_FACE ( 'NONE', ( #27998 ), #14802, .T. ) ;
#36029=CARTESIAN_POINT ( 'NONE',  ( 10.81189881249999907, 6.242252689847868297, -116.9062500020483952 ) ) ;
#36031=DIRECTION ( 'NONE',  ( 1.000000000000000000, 0.000000000000000000, -0.000000000000000000 ) ) ;
#36032=VERTEX_POINT ( 'NONE', #2105 ) ;
#36033=CARTESIAN_POINT ( 'NONE',  ( 10.81189881249999907, 6.242252689847868297, -55.40625000204837391 ) ) ;
#36035=CARTESIAN_POINT ( 'NONE',  ( -10.81189881249999729, 6.242252689847871849, -101.2187500020483810 ) ) ;
#36036=CARTESIAN_POINT ( 'NONE',  ( -5.405949406250003975, -9.363379034771801557, -122.0312500020483952 ) ) ;
#36037=ORIENTED_EDGE ( 'NONE', *, *, #36084, .F. ) ;
#36039=CARTESIAN_POINT ( 'NONE',  ( -9.999999999999479527, -5.773502691896549521, -116.6249999999999574 ) ) ;
#36041=CARTESIAN_POINT ( 'NONE',  ( -2.293366432827344421E-15, -12.48450537969573659, -1.718750002048355929 ) ) ;
#36043=CARTESIAN_POINT ( 'NONE',  ( 10.81189881249999729, 0.000000000000000000, -131.8437500020484094 ) ) ;
#36045=CARTESIAN_POINT ( 'NONE',  ( -5.000000000000003553, -8.660254037844383745, -158.5000000000000000 ) ) ;
#36047=CARTESIAN_POINT ( 'NONE',  ( -9.999999999999998224, 1.224646799147353059E-15, -195.1250000040967905 ) ) ;
#36049=CARTESIAN_POINT ( 'NONE',  ( 7.644554776091147741E-16, 12.48450537969573659, -188.6562500020484094 ) ) ;
#36050=CARTESIAN_POINT ( 'NONE',  ( -9.999999999999998224, 1.224646799147353059E-15, -186.1250000040967905 ) ) ;
#36053=CARTESIAN_POINT ( 'NONE',  ( 10.81189881249999729, 0.000000000000000000, -61.34375000204836681 ) ) ;
#36054=CARTESIAN_POINT ( 'NONE',  ( -2.293366432827344421E-15, -12.48450537969573659, -52.71875000204837391 ) ) ;
#36057=CARTESIAN_POINT ( 'NONE',  ( -10.81189881249999729, 1.324075727343319199E-15, -21.78125000204836326 ) ) ;
#36059=CARTESIAN_POINT ( 'NONE',  ( -9.999999999998456346, -5.773502691897145489, -8.624999999999937828 ) ) ;
#36061=CARTESIAN_POINT ( 'NONE',  ( 7.070501591499377789E-16, 11.54700538379251284, -106.6249999999999716 ) ) ;
#36062=CARTESIAN_POINT ( 'NONE',  ( 9.999999999999998224, 0.000000000000000000, -164.0000000000000000 ) ) ;
#36065=CARTESIAN_POINT ( 'NONE',  ( -5.405949406249996869, 9.363379034771805109, -119.5312500020483952 ) ) ;
#36066=ORIENTED_EDGE ( 'NONE', *, *, #19118, .T. ) ;
#36071=CARTESIAN_POINT ( 'NONE',  ( -4.999999999999996447, 8.660254037844387298, -41.99999999999997868 ) ) ;
#36072=CARTESIAN_POINT ( 'NONE',  ( 10.00000000000000000, 5.773502691896255534, -15.75000000409677270 ) ) ;
#36073=CARTESIAN_POINT ( 'NONE',  ( 7.644554776091147741E-16, 12.48450537969573659, -44.65625000204836681 ) ) ;
#36077=CARTESIAN_POINT ( 'NONE',  ( -10.81189881249999907, -6.242252689847864744, -135.6562500020484094 ) ) ;
#36079=CARTESIAN_POINT ( 'NONE',  ( 10.81189881249999729, 0.000000000000000000, -144.0312500020483810 ) ) ;
#36084=EDGE_CURVE ( 'NONE', #16838, #12159, #27155, .T. ) ;
#36086=CARTESIAN_POINT ( 'NONE',  ( 7.644554776091147741E-16, 12.48450537969573659, -173.4687500020483810 ) ) ;
#36087=CARTESIAN_POINT ( 'NONE',  ( -10.81189881249999907, -6.242252689847864744, -25.96875000204837391 ) ) ;
#36089=CARTESIAN_POINT ( 'NONE',  ( -10.81189881249999729, 6.242252689847871849, -159.7187500020483810 ) ) ;
#36090=CARTESIAN_POINT ( 'NONE',  ( -5.405949406250003975, -9.363379034771801557, -141.3437500020483810 ) ) ;
#36094=( BOUNDED_CURVE ( )  B_SPLINE_CURVE ( 2, ( #41206, #27859, #34771, #14228, #21805, #28289, #11009 ),
 .UNSPECIFIED., .F., .F. ) 
 B_SPLINE_CURVE_WITH_KNOTS ( ( 3, 2, 2, 3 ),
 ( 0.6119402985074627876, 0.6131840796019901729, 0.6144278606965176692, 0.6156716417910449435 ),
 .UNSPECIFIED. ) 
 CURVE ( )  GEOMETRIC_REPRESENTATION_ITEM ( )  RATIONAL_B_SPLINE_CURVE ( ( 0.9999999999999880096, 0.8660254037844506980, 1.000000000000000000, 0.8660254037844387076, 1.000000000000000000, 0.8660254037844148378, 1.000000000000023981 ) ) 
 REPRESENTATION_ITEM ( '' )  );
#36095=CARTESIAN_POINT ( 'NONE',  ( -10.81189881249999907, -6.242252689847864744, -21.46875000204836681 ) ) ;
#36097=CYLINDRICAL_SURFACE ( 'NONE', #14323, 9.999999999999998224 ) ;
#36098=CARTESIAN_POINT ( 'NONE',  ( -9.999999999999998224, 1.224646799147353059E-15, -28.24999999999996803 ) ) ;
#36100=CARTESIAN_POINT ( 'NONE',  ( 9.999999999999998224, 0.000000000000000000, -174.5000000000000284 ) ) ;
#36101=CARTESIAN_POINT ( 'NONE',  ( -10.81189881249999907, -6.242252689847864744, -72.46875000204835260 ) ) ;
#36102=CARTESIAN_POINT ( 'NONE',  ( -10.81189881249999729, 1.324075727343319199E-15, -42.78125000204838102 ) ) ;
#36106=CARTESIAN_POINT ( 'NONE',  ( -9.999999999999998224, 1.224646799147353059E-15, -140.7500000000000000 ) ) ;
#36107=CARTESIAN_POINT ( 'NONE',  ( -2.293366432827344421E-15, -12.48450537969573659, -135.4062500020483810 ) ) ;
#36108=CARTESIAN_POINT ( 'NONE',  ( -5.000000000000003553, -8.660254037844383745, -98.87500000409677625 ) ) ;
#36109=CARTESIAN_POINT ( 'NONE',  ( -4.999999999999996447, 8.660254037844387298, -111.3750000040967763 ) ) ;
#36111=VERTEX_POINT ( 'NONE', #31454 ) ;
#36112=( BOUNDED_CURVE ( )  B_SPLINE_CURVE ( 2, ( #27984, #37473, #41113, #1443, #1017, #14137, #11346 ),
 .UNSPECIFIED., .F., .F. ) 
 B_SPLINE_CURVE_WITH_KNOTS ( ( 3, 2, 2, 3 ),
 ( 0.8843283582089555006, 0.8855721393034827749, 0.8868159203980102712, 0.8880597014925376564 ),
 .UNSPECIFIED. ) 
 CURVE ( )  GEOMETRIC_REPRESENTATION_ITEM ( )  RATIONAL_B_SPLINE_CURVE ( ( 0.9999999999999761302, 0.8660254037844625774, 1.000000000000000000, 0.8660254037844387076, 1.000000000000000000, 0.8660254037844028474, 1.000000000000035971 ) ) 
 REPRESENTATION_ITEM ( '' )  );
#36115=CARTESIAN_POINT ( 'NONE',  ( 10.00000000000051159, -5.773502691895965988, -140.5000000040967620 ) ) ;
#36116=CARTESIAN_POINT ( 'NONE',  ( -10.81189881249999907, -6.242252689847864744, -173.1562500020484094 ) ) ;
#36117=CARTESIAN_POINT ( 'NONE',  ( 10.00000000000000000, 5.773502691896255534, -39.75000000409675494 ) ) ;
#36118=CARTESIAN_POINT ( 'NONE',  ( -5.000000000000003553, -8.660254037844383745, -91.37500000409677625 ) ) ;
#36120=EDGE_CURVE ( 'NONE', #38469, #35463, #31587, .T. ) ;
#36121=( BOUNDED_CURVE ( )  B_SPLINE_CURVE ( 2, ( #12325, #19027, #38881, #8691, #16184, #42315, #15562 ),
 .UNSPECIFIED., .F., .F. ) 
 B_SPLINE_CURVE_WITH_KNOTS ( ( 3, 2, 2, 3 ),
 ( 0.5559701492537315604, 0.5572139303482589456, 0.5584577114427863309, 0.5597014925373136052 ),
 .UNSPECIFIED. ) 
 CURVE ( )  GEOMETRIC_REPRESENTATION_ITEM ( )  RATIONAL_B_SPLINE_CURVE ( ( 0.9999999999999761302, 0.8660254037844625774, 1.000000000000000000, 0.8660254037844387076, 1.000000000000000000, 0.8660254037844148378, 1.000000000000023981 ) ) 
 REPRESENTATION_ITEM ( '' )  );
#36122=CARTESIAN_POINT ( 'NONE',  ( -5.321294541346989426, 5.321294541346989426, -220.0000000000000000 ) ) ;
#36123=CARTESIAN_POINT ( 'NONE',  ( -10.81189881249999907, -6.242252689847864744, -159.6562500020484094 ) ) ;
#36124=CARTESIAN_POINT ( 'NONE',  ( 10.81189881249999551, -6.242252689847874514, -139.4687500020483810 ) ) ;
#36125=CARTESIAN_POINT ( 'NONE',  ( -9.999999999999998224, 1.224646799147353059E-15, -46.24999999999998579 ) ) ;
#36127=VERTEX_POINT ( 'NONE', #40487 ) ;
#36128=CARTESIAN_POINT ( 'NONE',  ( 10.00000000000051159, -5.773502691895965988, -78.62499999999997158 ) ) ;
#36129=CARTESIAN_POINT ( 'NONE',  ( -10.81189881249999729, 1.324075727343319199E-15, -68.28125000204838102 ) ) ;
#36130=ORIENTED_EDGE ( 'NONE', *, *, #9486, .F. ) ;
#36132=CARTESIAN_POINT ( 'NONE',  ( 10.81189881249999907, 6.242252689847868297, -116.7187500020483810 ) ) ;
#36133=ORIENTED_EDGE ( 'NONE', *, *, #25690, .F. ) ;
#36134=VERTEX_POINT ( 'NONE', #10933 ) ;
#36135=CARTESIAN_POINT ( 'NONE',  ( 10.81189881249999729, 6.242252689847867408, -23.71875000204836681 ) ) ;
#36136=CARTESIAN_POINT ( 'NONE',  ( -10.81189881249999729, 1.324075727343319199E-15, -198.5937500020484094 ) ) ;
#36137=CARTESIAN_POINT ( 'NONE',  ( 5.405949406249992428, -9.363379034771808662, -48.09375000204838102 ) ) ;
#36139=EDGE_CURVE ( 'NONE', #14232, #34637, #35984, .T. ) ;
#36141=CARTESIAN_POINT ( 'NONE',  ( -2.293366432827344421E-15, -12.48450537969573659, -177.2187500020484094 ) ) ;
#36142=CARTESIAN_POINT ( 'NONE',  ( 10.81189881249999729, 0.000000000000000000, -170.8437500020484094 ) ) ;
#36145=CARTESIAN_POINT ( 'NONE',  ( -2.121150477449813534E-15, -11.54700538379251284, -104.7500000040967763 ) ) ;
#36147=CARTESIAN_POINT ( 'NONE',  ( -5.405949406249996869, 9.363379034771805109, -93.84375000204838102 ) ) ;
#36148=CARTESIAN_POINT ( 'NONE',  ( -9.999999999999998224, 1.224646799147353059E-15, -108.1250000040967763 ) ) ;
#36149=CARTESIAN_POINT ( 'NONE',  ( -10.81189881249999907, -6.242252689847864744, -71.15625000204839523 ) ) ;
#36150=CARTESIAN_POINT ( 'NONE',  ( 9.999999999999998224, 0.000000000000000000, -4.999999999999976907 ) ) ;
#36152=CARTESIAN_POINT ( 'NONE',  ( 7.644554776091147741E-16, 12.48450537969573659, -161.6562500020484094 ) ) ;
#36154=CARTESIAN_POINT ( 'NONE',  ( 4.999999999999992006, -8.660254037844389075, -140.6250000040967905 ) ) ;
#36163=CARTESIAN_POINT ( 'NONE',  ( -10.00000000000000000, -5.773502691896251982, -58.12499999999998579 ) ) ;
#36165=CARTESIAN_POINT ( 'NONE',  ( -10.00000000000000000, -5.773502691896251982, -67.50000000409679046 ) ) ;
#36167=DIRECTION ( 'NONE',  ( -0.000000000000000000, -0.000000000000000000, 1.000000000000000000 ) ) ;
#36169=CARTESIAN_POINT ( 'NONE',  ( -10.81189881249999729, 6.242252689847871849, -68.40625000204840944 ) ) ;
#36172=CARTESIAN_POINT ( 'NONE',  ( 5.405949406249999534, 9.363379034771803333, -184.2812500020484094 ) ) ;
#36174=CARTESIAN_POINT ( 'NONE',  ( 8.614196012143713332, -6.533971456633876684, 2.775557561562891351E-14 ) ) ;
#36175=CARTESIAN_POINT ( 'NONE',  ( 4.999999999999992006, -8.660254037844389075, -117.7500000000000000 ) ) ;
#36177=CARTESIAN_POINT ( 'NONE',  ( -5.000000000000003553, -8.660254037844383745, -166.0000000000000000 ) ) ;
#36178=CARTESIAN_POINT ( 'NONE',  ( -9.999999999999998224, 1.224646799147353059E-15, -122.7500000000000000 ) ) ;
#36179=CARTESIAN_POINT ( 'NONE',  ( -2.293366432827344421E-15, -12.48450537969573659, -91.90625000204838102 ) ) ;
#36181=LINE ( 'NONE', #39419, #25553 ) ;
#36182=DIRECTION ( 'NONE',  ( -1.000000000000000000, 0.000000000000000000, 0.000000000000000000 ) ) ;
#36183=EDGE_LOOP ( 'NONE', ( #30676, #24950, #4984, #26211 ) ) ;
#36184=( BOUNDED_CURVE ( )  B_SPLINE_CURVE ( 2, ( #42658, #42447, #13082, #35993, #33612, #26069, #39220 ),
 .UNSPECIFIED., .F., .F. ) 
 B_SPLINE_CURVE_WITH_KNOTS ( ( 3, 2, 2, 3 ),
 ( 0.2723880597014926574, 0.2736318407960199872, 0.2748756218905473725, 0.2761194029850747578 ),
 .UNSPECIFIED. ) 
 CURVE ( )  GEOMETRIC_REPRESENTATION_ITEM ( )  RATIONAL_B_SPLINE_CURVE ( ( 0.9999999999999880096, 0.8660254037844506980, 1.000000000000000000, 0.8660254037844387076, 1.000000000000000000, 0.8660254037844267172, 1.000000000000011990 ) ) 
 REPRESENTATION_ITEM ( '' )  );
#36185=EDGE_LOOP ( 'NONE', ( #23509, #25323, #31841, #25221 ) ) ;
#36186=CARTESIAN_POINT ( 'NONE',  ( 7.644554776091147741E-16, 12.48450537969573659, -35.46875000204835260 ) ) ;
#36187=VECTOR ( 'NONE', #40838, 1000.000000000000000 ) ;
#36188=CARTESIAN_POINT ( 'NONE',  ( -10.81189881249999907, -6.242252689847864744, -23.15625000204837747 ) ) ;
#36190=CARTESIAN_POINT ( 'NONE',  ( -5.405949406250003975, -9.363379034771801557, -70.84375000204836681 ) ) ;
#36191=CARTESIAN_POINT ( 'NONE',  ( 9.999999999999479527, 5.773502691896553074, -105.3749999999999716 ) ) ;
#36193=CARTESIAN_POINT ( 'NONE',  ( 10.81189881249999907, 6.242252689847868297, -190.2187500020484094 ) ) ;
#36194=EDGE_CURVE ( 'NONE', #36127, #6564, #28853, .T. ) ;
#36195=CARTESIAN_POINT ( 'NONE',  ( -9.999999999999479527, -5.773502691896549521, -79.50000000409677625 ) ) ;
#36198=CARTESIAN_POINT ( 'NONE',  ( 9.999999999999998224, 0.000000000000000000, -6.875000004096742501 ) ) ;
#36199=CARTESIAN_POINT ( 'NONE',  ( 10.00000000000102318, -5.773502691895667560, -80.12499999999997158 ) ) ;
#36200=CARTESIAN_POINT ( 'NONE',  ( 10.81189881249999551, -6.242252689847874514, -118.4687500020483810 ) ) ;
#36201=CARTESIAN_POINT ( 'NONE',  ( -5.405949406250003975, -9.363379034771801557, -96.53125000204839523 ) ) ;
#36202=CARTESIAN_POINT ( 'NONE',  ( -10.81189881249999729, 6.242252689847871849, -110.2187500020483810 ) ) ;
#36206=CARTESIAN_POINT ( 'NONE',  ( -9.999999999999998224, 1.224646799147353059E-15, -165.1250000040967905 ) ) ;
#36207=CARTESIAN_POINT ( 'NONE',  ( 4.999999999999992006, -8.660254037844389075, -66.74999999999997158 ) ) ;
#36211=CARTESIAN_POINT ( 'NONE',  ( 10.00000000000038369, -5.773502691896038819, -156.6250000000000284 ) ) ;
#36215=CARTESIAN_POINT ( 'NONE',  ( 7.070501591499377789E-16, 11.54700538379251284, -78.12500000000000000 ) ) ;
#36217=CARTESIAN_POINT ( 'NONE',  ( -9.999999999999998224, 5.773502691896259087, -87.25000000409676204 ) ) ;
#36218=EDGE_CURVE ( 'NONE', #21702, #2376, #21938, .T. ) ;
#36219=CARTESIAN_POINT ( 'NONE',  ( 9.999999999999998224, 0.000000000000000000, -150.8750000040967905 ) ) ;
#36221=CARTESIAN_POINT ( 'NONE',  ( -10.81189881249999729, 1.324075727343319199E-15, -95.28125000204838102 ) ) ;
#36222=VERTEX_POINT ( 'NONE', #38975 ) ;
#36224=DIRECTION ( 'NONE',  ( 0.000000000000000000, -1.000000000000000000, 0.000000000000000000 ) ) ;
#36227=CARTESIAN_POINT ( 'NONE',  ( 4.999999999999992006, -8.660254037844389075, -9.749999999999953815 ) ) ;
#36228=ADVANCED_FACE ( 'NONE', ( #12418 ), #16073, .T. ) ;
#36229=CARTESIAN_POINT ( 'NONE',  ( 7.070501591499377789E-16, 11.54700538379251284, -142.6250000000000000 ) ) ;
#36230=CARTESIAN_POINT ( 'NONE',  ( -9.999999999999998224, 1.224646799147353059E-15, -32.74999999999997158 ) ) ;
#36231=EDGE_CURVE ( 'NONE', #4695, #28503, #9411, .T. ) ;
#36233=( BOUNDED_CURVE ( )  B_SPLINE_CURVE ( 2, ( #5957, #15845, #29249, #19305, #8975, #12611, #25804 ),
 .UNSPECIFIED., .F., .F. ) 
 B_SPLINE_CURVE_WITH_KNOTS ( ( 3, 2, 2, 3 ),
 ( 0.3731343283582090331, 0.3743781094527363629, 0.3756218905472638037, 0.3768656716417911334 ),
 .UNSPECIFIED. ) 
 CURVE ( )  GEOMETRIC_REPRESENTATION_ITEM ( )  RATIONAL_B_SPLINE_CURVE ( ( 0.9999999999999940048, 0.8660254037844447028, 1.000000000000000000, 0.8660254037844387076, 1.000000000000000000, 0.8660254037844267172, 1.000000000000011990 ) ) 
 REPRESENTATION_ITEM ( '' )  );
#36234=CARTESIAN_POINT ( 'NONE',  ( -2.121150477449813534E-15, -11.54700538379251284, -192.8750000000000284 ) ) ;
#36235=CARTESIAN_POINT ( 'NONE',  ( 10.81189881249999729, 0.000000000000000000, -120.0312500020483952 ) ) ;
#36237=CARTESIAN_POINT ( 'NONE',  ( -9.999999999999998224, 1.224646799147353059E-15, -22.62500000409675849 ) ) ;
#36238=VECTOR ( 'NONE', #41360, 1000.000000000000000 ) ;
#36241=CARTESIAN_POINT ( 'NONE',  ( -2.293366432827344421E-15, -12.48450537969573659, -48.40625000204837391 ) ) ;
#36243=CARTESIAN_POINT ( 'NONE',  ( 7.644554776091147741E-16, 12.48450537969573659, -93.96875000204838102 ) ) ;
#36244=CARTESIAN_POINT ( 'NONE',  ( -5.405949406249996869, 9.363379034771805109, -121.0312500020483952 ) ) ;
#36245=EDGE_CURVE ( 'NONE', #4845, #4157, #42410, .T. ) ;
#36246=EDGE_LOOP ( 'NONE', ( #27148, #14340, #2706, #26401 ) ) ;
#36247=DIRECTION ( 'NONE',  ( -0.000000000000000000, -0.000000000000000000, 1.000000000000000000 ) ) ;
#36252=EDGE_CURVE ( 'NONE', #13704, #29829, #2088, .T. ) ;
#36253=CARTESIAN_POINT ( 'NONE',  ( -2.293366432827344421E-15, -12.48450537969573659, -135.2187500020483810 ) ) ;
#36258=CARTESIAN_POINT ( 'NONE',  ( -4.999999999999996447, 8.660254037844387298, -183.3750000040967905 ) ) ;
#36260=CARTESIAN_POINT ( 'NONE',  ( 10.81189881249999551, -6.242252689847874514, -183.1562500020484094 ) ) ;
#36261=DIRECTION ( 'NONE',  ( -0.000000000000000000, -0.000000000000000000, 1.000000000000000000 ) ) ;
#36262=CARTESIAN_POINT ( 'NONE',  ( 9.999999999999998224, 0.000000000000000000, -140.0000000000000000 ) ) ;
#36265=CARTESIAN_POINT ( 'NONE',  ( 5.405949406249992428, -9.363379034771808662, -57.09375000204835970 ) ) ;
#36266=CARTESIAN_POINT ( 'NONE',  ( 5.405949406249992428, -9.363379034771808662, -46.59375000204838102 ) ) ;
#36268=CARTESIAN_POINT ( 'NONE',  ( -2.293366432827344421E-15, -12.48450537969573659, -18.40625000204837036 ) ) ;
#36272=CARTESIAN_POINT ( 'NONE',  ( 9.999999999999998224, 0.000000000000000000, -105.4999999999999858 ) ) ;
#36278=CARTESIAN_POINT ( 'NONE',  ( -10.81189881249999729, 6.242252689847871849, -117.9062500020483952 ) ) ;
#36286=CARTESIAN_POINT ( 'NONE',  ( 10.00000000000000000, 5.773502691896255534, -31.87499999999995737 ) ) ;
#36287=CARTESIAN_POINT ( 'NONE',  ( 10.00000000000000000, 5.773502691896255534, -17.25000000409676204 ) ) ;
#36288=CARTESIAN_POINT ( 'NONE',  ( -10.81189881249999729, 1.324075727343319199E-15, -47.28125000204838813 ) ) ;
#36292=CARTESIAN_POINT ( 'NONE',  ( 10.81189881249999551, -6.242252689847874514, -136.6562500020484094 ) ) ;
#36294=CARTESIAN_POINT ( 'NONE',  ( 5.405949406249992428, -9.363379034771808662, -142.7812500020483810 ) ) ;
#36295=CARTESIAN_POINT ( 'NONE',  ( 9.999999999999998224, 0.000000000000000000, -123.5000000000000000 ) ) ;
#36296=EDGE_LOOP ( 'NONE', ( #38739, #30506, #20933, #28855 ) ) ;
#36297=VERTEX_POINT ( 'NONE', #2945 ) ;
#36298=ORIENTED_EDGE ( 'NONE', *, *, #15514, .F. ) ;
#36300=CARTESIAN_POINT ( 'NONE',  ( -10.81189881249999729, 6.242252689847871849, -173.2187500020483810 ) ) ;
#36301=CARTESIAN_POINT ( 'NONE',  ( -10.81189881249999729, 6.242252689847871849, -24.71875000204837036 ) ) ;
#36302=CARTESIAN_POINT ( 'NONE',  ( 9.999999999999998224, 0.000000000000000000, -38.37500000409676915 ) ) ;
#36303=CARTESIAN_POINT ( 'NONE',  ( 10.81189881249999551, -6.242252689847874514, -152.9687500020484094 ) ) ;
#36304=CARTESIAN_POINT ( 'NONE',  ( -10.81189881249999907, -6.242252689847864744, -145.9687500020484094 ) ) ;
#36305=CARTESIAN_POINT ( 'NONE',  ( 10.00000000000154010, -5.773502691895370020, -8.500000004096712303 ) ) ;
#36308=CARTESIAN_POINT ( 'NONE',  ( 10.81189881249999907, 6.242252689847868297, -22.21875000204837036 ) ) ;
#36312=CARTESIAN_POINT ( 'NONE',  ( 9.999999999999998224, 0.000000000000000000, -167.3750000040967905 ) ) ;
#36313=EDGE_CURVE ( 'NONE', #38258, #684, #9619, .T. ) ;
#36314=CARTESIAN_POINT ( 'NONE',  ( -10.81189881249999729, 1.324075727343319199E-15, -71.09375000204836681 ) ) ;
#36315=CARTESIAN_POINT ( 'NONE',  ( 10.81189881249999907, 6.242252689847868297, -46.40625000204835970 ) ) ;
#36319=CARTESIAN_POINT ( 'NONE',  ( 5.000000000000000000, 8.660254037844385522, -129.2499999999999716 ) ) ;
#36320=CARTESIAN_POINT ( 'NONE',  ( -10.81189881249999729, 1.324075727343319199E-15, -137.2812500020483810 ) ) ;
#36322=CARTESIAN_POINT ( 'NONE',  ( 7.070501591499377789E-16, 11.54700538379251284, -117.5000000040967905 ) ) ;
#36324=ORIENTED_EDGE ( 'NONE', *, *, #9661, .F. ) ;
#36328=CARTESIAN_POINT ( 'NONE',  ( 5.405949406249992428, -9.363379034771808662, -160.7812500020484094 ) ) ;
#36329=CARTESIAN_POINT ( 'NONE',  ( 10.00000000000000000, 5.773502691896255534, -41.25000000409676204 ) ) ;
#36332=DIRECTION ( 'NONE',  ( -0.000000000000000000, -0.000000000000000000, 1.000000000000000000 ) ) ;
#36333=CARTESIAN_POINT ( 'NONE',  ( 5.405949406249999534, 9.363379034771803333, -163.2812500020484094 ) ) ;
#36334=CARTESIAN_POINT ( 'NONE',  ( -10.81189881249999729, 1.324075727343319199E-15, -132.5937500020483810 ) ) ;
#36335=LINE ( 'NONE', #6766, #27701 ) ;
#36338=CARTESIAN_POINT ( 'NONE',  ( -9.999999999998969713, -5.773502691896847949, -31.12499999999993250 ) ) ;
#36339=CARTESIAN_POINT ( 'NONE',  ( -10.81189881249999907, -6.242252689847864744, -72.65625000204836681 ) ) ;
#36342=CARTESIAN_POINT ( 'NONE',  ( 5.405949406249999534, 9.363379034771803333, -116.5937500020483810 ) ) ;
#36343=VERTEX_POINT ( 'NONE', #15447 ) ;
#36345=( BOUNDED_CURVE ( )  B_SPLINE_CURVE ( 2, ( #12649, #18717, #9849, #15676, #2755, #31911, #29286 ),
 .UNSPECIFIED., .F., .F. ) 
 B_SPLINE_CURVE_WITH_KNOTS ( ( 3, 2, 2, 3 ),
 ( 0.8097014925373136052, 0.8109452736318409904, 0.8121890547263682647, 0.8134328358208956500 ),
 .UNSPECIFIED. ) 
 CURVE ( )  GEOMETRIC_REPRESENTATION_ITEM ( )  RATIONAL_B_SPLINE_CURVE ( ( 0.9999999999999761302, 0.8660254037844625774, 1.000000000000000000, 0.8660254037844387076, 1.000000000000000000, 0.8660254037844267172, 1.000000000000011990 ) ) 
 REPRESENTATION_ITEM ( '' )  );
#36346=CARTESIAN_POINT ( 'NONE',  ( -5.405949406249996869, 9.363379034771805109, -21.84375000204835615 ) ) ;
#36347=CARTESIAN_POINT ( 'NONE',  ( 10.81189881249999907, 6.242252689847868297, -1.406250002048370584 ) ) ;
#36348=CARTESIAN_POINT ( 'NONE',  ( -10.81189881249999729, 1.324075727343319199E-15, -44.09375000204837391 ) ) ;
#36349=CYLINDRICAL_SURFACE ( 'NONE', #17065, 9.999999999999998224 ) ;
#36351=CARTESIAN_POINT ( 'NONE',  ( 10.81189881249999551, -6.242252689847874514, -181.4687500020484094 ) ) ;
#36352=CARTESIAN_POINT ( 'NONE',  ( -5.405949406249996869, 9.363379034771805109, -170.3437500020484094 ) ) ;
#36358=CARTESIAN_POINT ( 'NONE',  ( -10.81189881249999729, 1.324075727343319199E-15, -99.59375000204838102 ) ) ;
#36360=CARTESIAN_POINT ( 'NONE',  ( 7.644554776091147741E-16, 12.48450537969573659, -62.65625000204838813 ) ) ;
#36361=CARTESIAN_POINT ( 'NONE',  ( 10.00000000000025402, -5.773502691896113426, -159.6250000000000284 ) ) ;
#36363=CARTESIAN_POINT ( 'NONE',  ( -5.405949406249996869, 9.363379034771805109, -119.5312500020483952 ) ) ;
#36364=CARTESIAN_POINT ( 'NONE',  ( 5.405949406249999534, 9.363379034771803333, -161.7812500020484094 ) ) ;
#36366=CARTESIAN_POINT ( 'NONE',  ( -4.999999999999996447, 8.660254037844387298, -135.3750000040967905 ) ) ;
#36368=VERTEX_POINT ( 'NONE', #28645 ) ;
#36371=CYLINDRICAL_SURFACE ( 'NONE', #17853, 9.999999999999998224 ) ;
#36372=CARTESIAN_POINT ( 'NONE',  ( -5.000000000000003553, -8.660254037844383745, -43.37500000409677625 ) ) ;
#36374=AXIS2_PLACEMENT_3D ( 'NONE', #700, #30893, #4133 ) ;
#36375=ORIENTED_EDGE ( 'NONE', *, *, #4854, .F. ) ;
#36376=CARTESIAN_POINT ( 'NONE',  ( -2.121150477449813534E-15, -11.54700538379251284, -54.87499999999997158 ) ) ;
#36378=CARTESIAN_POINT ( 'NONE',  ( 9.999999999999996447, -5.773502691896262640, -65.50000000409677625 ) ) ;
#36380=EDGE_CURVE ( 'NONE', #25635, #6986, #24149, .T. ) ;
#36381=CARTESIAN_POINT ( 'NONE',  ( 7.070501591499376803E-16, 11.54700538379251284, -21.50000000409676559 ) ) ;
#36382=CYLINDRICAL_SURFACE ( 'NONE', #33960, 9.999999999999998224 ) ;
#36384=CARTESIAN_POINT ( 'NONE',  ( 10.81189881249999729, 6.242252689847867408, -61.40625000204838813 ) ) ;
#36387=CARTESIAN_POINT ( 'NONE',  ( -9.999999999999998224, 1.224646799147353059E-15, -160.2500000000000000 ) ) ;
#36388=CARTESIAN_POINT ( 'NONE',  ( 10.81189881249999551, -6.242252689847874514, -189.1562500020484379 ) ) ;
#36390=CARTESIAN_POINT ( 'NONE',  ( 7.070501591499376803E-16, 11.54700538379251284, -40.62499999999996447 ) ) ;
#36393=DIRECTION ( 'NONE',  ( -0.000000000000000000, -0.000000000000000000, 1.000000000000000000 ) ) ;
#36394=CARTESIAN_POINT ( 'NONE',  ( 9.999999999999998224, 0.000000000000000000, -170.0000000000000000 ) ) ;
#36395=CARTESIAN_POINT ( 'NONE',  ( -9.999999999999998224, 1.224646799147353059E-15, -51.12500000409675494 ) ) ;
#36396=CARTESIAN_POINT ( 'NONE',  ( 10.81189881249999907, 6.242252689847868297, -94.40625000204836681 ) ) ;
#36397=ORIENTED_EDGE ( 'NONE', *, *, #10365, .T. ) ;
#36398=CARTESIAN_POINT ( 'NONE',  ( 9.999999999999998224, 0.000000000000000000, -30.87500000409676559 ) ) ;
#36399=ORIENTED_EDGE ( 'NONE', *, *, #39797, .F. ) ;
#36401=CARTESIAN_POINT ( 'NONE',  ( 10.81189881249999907, 6.242252689847868297, -32.71875000204834549 ) ) ;
#36402=CARTESIAN_POINT ( 'NONE',  ( 10.81189881249999729, 0.000000000000000000, -19.53125000204835970 ) ) ;
#36404=CARTESIAN_POINT ( 'NONE',  ( -10.81189881249999729, 1.324075727343319199E-15, -69.59375000204836681 ) ) ;
#36405=CARTESIAN_POINT ( 'NONE',  ( 5.000000000000000000, 8.660254037844385522, -105.2499999999999858 ) ) ;
#36407=CARTESIAN_POINT ( 'NONE',  ( -10.81189881249999729, 1.324075727343319199E-15, -189.5937500020483810 ) ) ;
#36408=CARTESIAN_POINT ( 'NONE',  ( 10.81189881249999551, -6.242252689847874514, -151.4687500020483810 ) ) ;
#36410=CARTESIAN_POINT ( 'NONE',  ( -9.999999999999998224, 1.224646799147353059E-15, -112.2499999999999858 ) ) ;
#36412=CARTESIAN_POINT ( 'NONE',  ( 9.999999999999998224, 0.000000000000000000, -3.875000004096768258 ) ) ;
#36413=CARTESIAN_POINT ( 'NONE',  ( -9.999999999999998224, 1.224646799147353059E-15, -49.62500000409675494 ) ) ;
#36414=CARTESIAN_POINT ( 'NONE',  ( -10.81189881249999907, -6.242252689847864744, -117.4687500020483952 ) ) ;
#36416=CARTESIAN_POINT ( 'NONE',  ( 7.644554776091147741E-16, 12.48450537969573659, -86.65625000204838102 ) ) ;
#36417=CARTESIAN_POINT ( 'NONE',  ( -10.81189881249999729, 1.324075727343319199E-15, -108.5937500020483810 ) ) ;
#36420=CARTESIAN_POINT ( 'NONE',  ( -9.999999999999998224, 5.773502691896259087, -160.7500000040967620 ) ) ;
#36421=DIRECTION ( 'NONE',  ( -0.000000000000000000, -0.000000000000000000, 1.000000000000000000 ) ) ;
#36426=CARTESIAN_POINT ( 'NONE',  ( 0.000000000000000000, 0.000000000000000000, -200.0000000000000000 ) ) ;
#36428=CARTESIAN_POINT ( 'NONE',  ( -2.121150477449813534E-15, -11.54700538379251284, -80.37499999999997158 ) ) ;
#36430=CARTESIAN_POINT ( 'NONE',  ( 7.070501591499377789E-16, 11.54700538379251284, -90.50000000409677625 ) ) ;
#36431=DIRECTION ( 'NONE',  ( 1.000000000000000000, 0.000000000000000000, 0.000000000000000000 ) ) ;
#36433=CARTESIAN_POINT ( 'NONE',  ( 5.405949406249999534, 9.363379034771803333, -85.28125000204838102 ) ) ;
#36434=VERTEX_POINT ( 'NONE', #23431 ) ;
#36436=CARTESIAN_POINT ( 'NONE',  ( 10.81189881249999729, 0.000000000000000000, -199.4375000020484094 ) ) ;
#36439=CARTESIAN_POINT ( 'NONE',  ( 7.070501591499377789E-16, 11.54700538379251284, -6.124999999999965361 ) ) ;
#36440=EDGE_CURVE ( 'NONE', #28824, #10829, #7026, .T. ) ;
#36441=CARTESIAN_POINT ( 'NONE',  ( -10.00000000000000000, -5.773502691896251982, -145.1250000000000284 ) ) ;
#36442=DIRECTION ( 'NONE',  ( -0.000000000000000000, -0.000000000000000000, 1.000000000000000000 ) ) ;
#36443=( BOUNDED_CURVE ( )  B_SPLINE_CURVE ( 2, ( #20475, #31061, #8182, #34518, #1496, #33662, #41165 ),
 .UNSPECIFIED., .F., .F. ) 
 B_SPLINE_CURVE_WITH_KNOTS ( ( 3, 2, 2, 3 ),
 ( 0.7164179104477614857, 0.7176616915422888709, 0.7189054726368161452, 0.7201492537313435305 ),
 .UNSPECIFIED. ) 
 CURVE ( )  GEOMETRIC_REPRESENTATION_ITEM ( )  RATIONAL_B_SPLINE_CURVE ( ( 0.9999999999999641398, 0.8660254037844745678, 1.000000000000000000, 0.8660254037844387076, 1.000000000000000000, 0.8660254037844148378, 1.000000000000023981 ) ) 
 REPRESENTATION_ITEM ( '' )  );
#36445=EDGE_CURVE ( 'NONE', #26792, #11948, #140, .T. ) ;
#36446=CARTESIAN_POINT ( 'NONE',  ( -2.121150477449813534E-15, -11.54700538379251284, -189.8750000000000000 ) ) ;
#36447=CARTESIAN_POINT ( 'NONE',  ( 7.071067811865472841, 7.071067811865472841, -200.0000000000000000 ) ) ;
#36448=CARTESIAN_POINT ( 'NONE',  ( -5.405949406250003975, -9.363379034771801557, -119.0312500020483952 ) ) ;
#36450=FACE_OUTER_BOUND ( 'NONE', #22439, .T. ) ;
#36451=ORIENTED_EDGE ( 'NONE', *, *, #11850, .F. ) ;
#36452=CARTESIAN_POINT ( 'NONE',  ( -5.405949406249996869, 9.363379034771805109, -49.03125000204838813 ) ) ;
#36454=CARTESIAN_POINT ( 'NONE',  ( -10.81189881249999729, 1.324075727343319199E-15, -96.59375000204838102 ) ) ;
#36455=CARTESIAN_POINT ( 'NONE',  ( 10.81189881249999729, 6.242252689847867408, -124.4062500020483810 ) ) ;
#36456=ORIENTED_EDGE ( 'NONE', *, *, #28864, .F. ) ;
#36457=CARTESIAN_POINT ( 'NONE',  ( -2.121150477449813534E-15, -11.54700538379251284, -111.8749999999999858 ) ) ;
#36459=CARTESIAN_POINT ( 'NONE',  ( -10.00000000000102496, 5.773502691895664007, -0.2500000040967191861 ) ) ;
#36460=CARTESIAN_POINT ( 'NONE',  ( 10.81189881249999551, -6.242252689847874514, -133.4687500020483810 ) ) ;
#36462=DIRECTION ( 'NONE',  ( -0.000000000000000000, -0.000000000000000000, 1.000000000000000000 ) ) ;
#36464=CARTESIAN_POINT ( 'NONE',  ( 9.999999999999998224, 0.000000000000000000, -186.8750000040967905 ) ) ;
#36466=CARTESIAN_POINT ( 'NONE',  ( -5.405949406249996869, 9.363379034771805109, -190.0312500020484094 ) ) ;
#36467=CARTESIAN_POINT ( 'NONE',  ( -9.999999999999998224, 1.224646799147353059E-15, -95.74999999999998579 ) ) ;
#36471=CARTESIAN_POINT ( 'NONE',  ( -2.293366432827344421E-15, -12.48450537969573659, -60.21875000204837391 ) ) ;
#36472=VECTOR ( 'NONE', #9824, 1000.000000000000000 ) ;
#36473=CARTESIAN_POINT ( 'NONE',  ( -10.81189881249999729, 6.242252689847871849, -50.21875000204836681 ) ) ;
#36475=CARTESIAN_POINT ( 'NONE',  ( -10.81189881249999729, 6.242252689847871849, -15.90625000204837391 ) ) ;
#36477=CARTESIAN_POINT ( 'NONE',  ( -5.000000000000003553, -8.660254037844383745, -92.87500000409677625 ) ) ;
#36479=CARTESIAN_POINT ( 'NONE',  ( -2.121150477449813534E-15, -11.54700538379251284, -105.8749999999999858 ) ) ;
#36483=CARTESIAN_POINT ( 'NONE',  ( -10.81189881249999729, 6.242252689847871849, -108.9062500020483810 ) ) ;
#36484=ORIENTED_EDGE ( 'NONE', *, *, #29172, .T. ) ;
#36485=( BOUNDED_CURVE ( )  B_SPLINE_CURVE ( 2, ( #31225, #4882, #17591, #37244, #24105, #1651, #20845 ),
 .UNSPECIFIED., .F., .F. ) 
 B_SPLINE_CURVE_WITH_KNOTS ( ( 3, 2, 2, 3 ),
 ( 0.3395522388059703522, 0.3407960199004976820, 0.3420398009950250118, 0.3432835820895522860 ),
 .UNSPECIFIED. ) 
 CURVE ( )  GEOMETRIC_REPRESENTATION_ITEM ( )  RATIONAL_B_SPLINE_CURVE ( ( 0.9999999999999761302, 0.8660254037844625774, 1.000000000000000000, 0.8660254037844387076, 1.000000000000000000, 0.8660254037844327124, 1.000000000000005995 ) ) 
 REPRESENTATION_ITEM ( '' )  );
#36486=AXIS2_PLACEMENT_3D ( 'NONE', #12671, #12464, #32765 ) ;
#36489=ORIENTED_EDGE ( 'NONE', *, *, #40653, .T. ) ;
#36490=CARTESIAN_POINT ( 'NONE',  ( -2.121150477449813534E-15, -11.54700538379251284, -32.37499999999996447 ) ) ;
#36491=CARTESIAN_POINT ( 'NONE',  ( -9.999999999999998224, 5.773502691896259087, -16.75000000409675849 ) ) ;
#36492=EDGE_CURVE ( 'NONE', #39036, #4760, #10122, .T. ) ;
#36493=CARTESIAN_POINT ( 'NONE',  ( 5.405949406249999534, 9.363379034771803333, -46.28125000204838813 ) ) ;
#36494=CARTESIAN_POINT ( 'NONE',  ( -4.999999999999996447, 8.660254037844387298, -34.87500000409676915 ) ) ;
#36497=DIRECTION ( 'NONE',  ( -1.000000000000000000, 0.000000000000000000, 0.000000000000000000 ) ) ;
#36498=CARTESIAN_POINT ( 'NONE',  ( -2.293366432827344421E-15, -12.48450537969573659, -145.9062500020484094 ) ) ;
#36500=CARTESIAN_POINT ( 'NONE',  ( -5.000000000000003553, -8.660254037844383745, -110.4999999999999858 ) ) ;
#36504=CARTESIAN_POINT ( 'NONE',  ( -4.999999999999996447, 8.660254037844387298, -159.0000000000000000 ) ) ;
#36505=CARTESIAN_POINT ( 'NONE',  ( -9.999999999999227285, -5.773502691896698735, -130.1249999999999716 ) ) ;
#36506=CARTESIAN_POINT ( 'NONE',  ( 10.81189881249999907, 6.242252689847868297, -172.2187500020483810 ) ) ;
#36508=CARTESIAN_POINT ( 'NONE',  ( 10.81189881249999907, 6.242252689847868297, -20.71875000204836681 ) ) ;
#36509=CARTESIAN_POINT ( 'NONE',  ( -2.121150477449813534E-15, -11.54700538379251284, -61.25000000409677625 ) ) ;
#36510=CARTESIAN_POINT ( 'NONE',  ( -9.999999999999998224, 1.224646799147353059E-15, -157.6250000040967905 ) ) ;
#36511=CARTESIAN_POINT ( 'NONE',  ( 10.81189881249999729, 0.000000000000000000, -158.8437500020483810 ) ) ;
#36512=CARTESIAN_POINT ( 'NONE',  ( 7.644554776091147741E-16, 12.48450537969573659, -141.9687500020483810 ) ) ;
#36513=CARTESIAN_POINT ( 'NONE',  ( 9.999999999999998224, 0.000000000000000000, -87.87500000409677625 ) ) ;
#36516=CARTESIAN_POINT ( 'NONE',  ( -10.81189881249999729, 1.324075727343319199E-15, -12.59375000204834905 ) ) ;
#36518=DIRECTION ( 'NONE',  ( 1.000000000000000000, 0.000000000000000000, 0.000000000000000000 ) ) ;
#36520=CARTESIAN_POINT ( 'NONE',  ( 9.999999999999998224, 0.000000000000000000, -106.9999999999999858 ) ) ;
#36521=CARTESIAN_POINT ( 'NONE',  ( -5.405949406250003975, -9.363379034771801557, -75.34375000204838102 ) ) ;
#36522=CARTESIAN_POINT ( 'NONE',  ( -5.405949406250003975, -9.363379034771801557, -45.53125000204838102 ) ) ;
#36524=CARTESIAN_POINT ( 'NONE',  ( -2.121150477449813534E-15, -11.54700538379251284, -113.7500000040967763 ) ) ;
#36526=CARTESIAN_POINT ( 'NONE',  ( -9.999999999999998224, 5.773502691896259087, -125.8749999999999858 ) ) ;
#36527=CARTESIAN_POINT ( 'NONE',  ( -2.293366432827344421E-15, -12.48450537969573659, -139.9062500020484094 ) ) ;
#36528=DIRECTION ( 'NONE',  ( -0.000000000000000000, -0.000000000000000000, 1.000000000000000000 ) ) ;
#36529=CARTESIAN_POINT ( 'NONE',  ( 4.999999999999992006, -8.660254037844389075, -113.6250000040967763 ) ) ;
#36531=ORIENTED_EDGE ( 'NONE', *, *, #7995, .F. ) ;
#36536=CARTESIAN_POINT ( 'NONE',  ( 10.81189881249999729, 0.000000000000000000, -168.0312500020484094 ) ) ;
#36537=CARTESIAN_POINT ( 'NONE',  ( 9.999999999999996447, -5.773502691896262640, -43.00000000409676204 ) ) ;
#36538=CYLINDRICAL_SURFACE ( 'NONE', #15230, 9.999999999999998224 ) ;
#36540=FACE_OUTER_BOUND ( 'NONE', #8808, .T. ) ;
#36541=CARTESIAN_POINT ( 'NONE',  ( 5.405949406249992428, -9.363379034771808662, -163.7812500020484094 ) ) ;
#36542=CARTESIAN_POINT ( 'NONE',  ( -10.81189881249999729, 1.324075727343319199E-15, -134.0937500020483810 ) ) ;
#36543=LINE ( 'NONE', #3750, #20116 ) ;
#36544=EDGE_LOOP ( 'NONE', ( #41958, #11012, #10521, #24294 ) ) ;
#36546=EDGE_CURVE ( 'NONE', #1269, #5836, #26243, .T. ) ;
#36547=CARTESIAN_POINT ( 'NONE',  ( -10.81189881249999729, 6.242252689847871849, -66.90625000204839523 ) ) ;
#36548=ORIENTED_EDGE ( 'NONE', *, *, #26621, .T. ) ;
#36550=CARTESIAN_POINT ( 'NONE',  ( 5.405949406249992428, -9.363379034771808662, -120.0937500020483952 ) ) ;
#36551=EDGE_LOOP ( 'NONE', ( #4811, #19023, #1956, #18237 ) ) ;
#36552=CARTESIAN_POINT ( 'NONE',  ( 7.644554776091147741E-16, 12.48450537969573659, -17.46875000204836681 ) ) ;
#36553=CARTESIAN_POINT ( 'NONE',  ( -5.405949406250003975, -9.363379034771801557, -196.8437500020484094 ) ) ;
#36554=CARTESIAN_POINT ( 'NONE',  ( -5.405949406250003975, -9.363379034771801557, -43.84375000204837391 ) ) ;
#36555=CARTESIAN_POINT ( 'NONE',  ( 9.999999999999998224, 0.000000000000000000, -72.49999999999998579 ) ) ;
#36556=CARTESIAN_POINT ( 'NONE',  ( 5.000000000000000000, 8.660254037844385522, -0.2499999999999724665 ) ) ;
#36558=CARTESIAN_POINT ( 'NONE',  ( 5.405949406249999534, 9.363379034771803333, -184.0937500020483810 ) ) ;
#36559=CARTESIAN_POINT ( 'NONE',  ( 10.81189881249999907, 6.242252689847868297, -166.2187500020484094 ) ) ;
#36563=CARTESIAN_POINT ( 'NONE',  ( -10.00000000000012434, 5.773502691896184480, -193.7500000040967620 ) ) ;
#36565=CARTESIAN_POINT ( 'NONE',  ( 10.81189881249999551, -6.242252689847874514, -100.4687500020483952 ) ) ;
#36567=CARTESIAN_POINT ( 'NONE',  ( 7.644554776091147741E-16, 12.48450537969573659, -65.65625000204838102 ) ) ;
#36570=CARTESIAN_POINT ( 'NONE',  ( 10.81189881249999551, -6.242252689847874514, -120.1562500020483810 ) ) ;
#36571=CARTESIAN_POINT ( 'NONE',  ( -5.405949406249996869, 9.363379034771805109, -163.0312500020484094 ) ) ;
#36573=CARTESIAN_POINT ( 'NONE',  ( -9.999999999999998224, 5.773502691896259087, -135.2500000040967905 ) ) ;
#36578=CARTESIAN_POINT ( 'NONE',  ( 10.81189881249999729, 0.000000000000000000, -189.0312500020484094 ) ) ;
#36581=ORIENTED_EDGE ( 'NONE', *, *, #25986, .F. ) ;
#36582=CARTESIAN_POINT ( 'NONE',  ( -10.00000000000000000, -5.773502691896251982, -56.62499999999997868 ) ) ;
#36584=CARTESIAN_POINT ( 'NONE',  ( 9.999999999999998224, 0.000000000000000000, -65.37500000409676204 ) ) ;
#36586=LINE ( 'NONE', #37219, #20839 ) ;
#36588=CARTESIAN_POINT ( 'NONE',  ( -10.81189881249999729, 1.324075727343319199E-15, -60.78125000204836681 ) ) ;
#36592=CARTESIAN_POINT ( 'NONE',  ( -10.81189881249999729, 6.242252689847871849, -188.4062500020484094 ) ) ;
#36598=FACE_OUTER_BOUND ( 'NONE', #36296, .T. ) ;
#36600=CARTESIAN_POINT ( 'NONE',  ( 9.999999999999998224, 0.000000000000000000, -61.99999999999997158 ) ) ;
#36601=CARTESIAN_POINT ( 'NONE',  ( -10.81189881249999907, -6.242252689847864744, -90.65625000204836681 ) ) ;
#36602=ORIENTED_EDGE ( 'NONE', *, *, #4036, .F. ) ;
#36603=CARTESIAN_POINT ( 'NONE',  ( 5.000000000000000000, 8.660254037844385522, -83.12500000409676204 ) ) ;
#36605=EDGE_LOOP ( 'NONE', ( #1356, #27542, #30575, #7953 ) ) ;
#36606=ORIENTED_EDGE ( 'NONE', *, *, #26241, .T. ) ;
#36607=CARTESIAN_POINT ( 'NONE',  ( -5.405949406249996869, 9.363379034771805109, -33.84375000204836681 ) ) ;
#36608=CARTESIAN_POINT ( 'NONE',  ( 5.405949406249999534, 9.363379034771803333, -19.28125000204835970 ) ) ;
#36609=CARTESIAN_POINT ( 'NONE',  ( -10.81189881249999729, 1.324075727343319199E-15, -72.59375000204838102 ) ) ;
#36610=CARTESIAN_POINT ( 'NONE',  ( -9.999999999999998224, 1.224646799147353059E-15, -133.6250000040967620 ) ) ;
#36612=CARTESIAN_POINT ( 'NONE',  ( 10.81189881249999907, 6.242252689847868297, -194.7187500020484094 ) ) ;
#36613=CARTESIAN_POINT ( 'NONE',  ( -10.81189881249999729, 6.242252689847871849, -150.7187500020483810 ) ) ;
#36615=CARTESIAN_POINT ( 'NONE',  ( 7.070501591499376803E-16, 11.54700538379251284, -99.12500000000000000 ) ) ;
#36618=CARTESIAN_POINT ( 'NONE',  ( -4.999999999999996447, 8.660254037844387298, -1.875000004096766260 ) ) ;
#36619=CARTESIAN_POINT ( 'NONE',  ( 0.000000000000000000, 0.000000000000000000, -200.0000000000000000 ) ) ;
#36620=PRODUCT_DEFINITION_FORMATION_WITH_SPECIFIED_SOURCE ( 'ANY', '', #2800, .NOT_KNOWN. ) ;
#36621=CARTESIAN_POINT ( 'NONE',  ( 5.405949406249999534, 9.363379034771803333, -122.5937500020483952 ) ) ;
#36622=FACE_OUTER_BOUND ( 'NONE', #41633, .T. ) ;
#36623=CARTESIAN_POINT ( 'NONE',  ( 10.81189881249999907, 6.242252689847868297, -91.40625000204836681 ) ) ;
#36624=CARTESIAN_POINT ( 'NONE',  ( -10.81189881249999729, -6.242252689847864744, -105.4687500020483668 ) ) ;
#36627=CARTESIAN_POINT ( 'NONE',  ( 4.999999999999992006, -8.660254037844389075, -158.6250000040967905 ) ) ;
#36631=CARTESIAN_POINT ( 'NONE',  ( 0.000000000000000000, 0.000000000000000000, -200.0000000000000000 ) ) ;
#36633=CARTESIAN_POINT ( 'NONE',  ( -5.000000000000003553, -8.660254037844383745, -53.87500000409675494 ) ) ;
#36635=CARTESIAN_POINT ( 'NONE',  ( 9.999999999999996447, -5.773502691896262640, -84.62499999999998579 ) ) ;
#36637=CARTESIAN_POINT ( 'NONE',  ( -4.999999999999996447, 8.660254037844387298, -88.87500000409677625 ) ) ;
#36640=CARTESIAN_POINT ( 'NONE',  ( -5.405949406250003975, -9.363379034771801557, -81.53125000204839523 ) ) ;
#36641=ORIENTED_EDGE ( 'NONE', *, *, #24740, .T. ) ;
#36647=CARTESIAN_POINT ( 'NONE',  ( -10.00000000000000000, -5.773502691896251982, -11.62499999999995914 ) ) ;
#36650=CARTESIAN_POINT ( 'NONE',  ( -10.00000000000000000, -5.773502691896251982, -146.6249999999999716 ) ) ;
#36651=CYLINDRICAL_SURFACE ( 'NONE', #42039, 9.999999999999998224 ) ;
#36654=CARTESIAN_POINT ( 'NONE',  ( -4.999999999999996447, 8.660254037844387298, -190.5000000000000000 ) ) ;
#36655=CARTESIAN_POINT ( 'NONE',  ( 9.999999999999998224, 0.000000000000000000, -47.37500000409677625 ) ) ;
#36656=CARTESIAN_POINT ( 'NONE',  ( -2.293366432827344421E-15, -12.48450537969573659, -117.4062500020483952 ) ) ;
#36657=VERTEX_POINT ( 'NONE', #16978 ) ;
#36658=DIRECTION ( 'NONE',  ( 1.000000000000000000, 1.502314598737160017E-16, 0.000000000000000000 ) ) ;
#36659=VERTEX_POINT ( 'NONE', #26919 ) ;
#36660=CARTESIAN_POINT ( 'NONE',  ( -10.81189881249999907, -6.242252689847864744, -44.15625000204838102 ) ) ;
#36663=CARTESIAN_POINT ( 'NONE',  ( 10.81189881249999907, 6.242252689847868297, -94.21875000204838102 ) ) ;
#36664=CARTESIAN_POINT ( 'NONE',  ( -10.81189881249999729, 1.324075727343319199E-15, -120.7812500020483952 ) ) ;
#36665=EDGE_LOOP ( 'NONE', ( #32488, #27324, #14995, #7511 ) ) ;
#36666=CARTESIAN_POINT ( 'NONE',  ( -9.999999999999998224, 1.224646799147353059E-15, -96.12500000409677625 ) ) ;
#36667=CARTESIAN_POINT ( 'NONE',  ( -9.999999999999998224, 1.224646799147353059E-15, -193.2500000000000000 ) ) ;
#36671=CARTESIAN_POINT ( 'NONE',  ( 10.81189881249999729, 6.242252689847867408, -131.7187500020483810 ) ) ;
#36675=CARTESIAN_POINT ( 'NONE',  ( -10.00000000000000000, -5.773502691896251982, -189.0000000040967905 ) ) ;
#36677=AXIS2_PLACEMENT_3D ( 'NONE', #40895, #40465, #27548 ) ;
#36678=CARTESIAN_POINT ( 'NONE',  ( -10.81189881249999729, 6.242252689847871849, -180.9062500020484094 ) ) ;
#36682=CARTESIAN_POINT ( 'NONE',  ( 5.405949406249992428, -9.363379034771808662, -63.09375000204836681 ) ) ;
#36683=CARTESIAN_POINT ( 'NONE',  ( -10.81189881249999729, 1.324075727343319199E-15, -39.59375000204837391 ) ) ;
#36685=CARTESIAN_POINT ( 'NONE',  ( 5.405949406249992428, -9.363379034771808662, -16.78125000204835970 ) ) ;
#36687=CARTESIAN_POINT ( 'NONE',  ( 4.999999999999992006, -8.660254037844389075, -92.62500000409677625 ) ) ;
#36689=CARTESIAN_POINT ( 'NONE',  ( -5.000000000000003553, -8.660254037844383745, -108.9999999999999858 ) ) ;
#36691=( BOUNDED_CURVE ( )  B_SPLINE_CURVE ( 2, ( #10371, #24424, #4550, #30673, #690, #10580, #20944 ),
 .UNSPECIFIED., .F., .F. ) 
 B_SPLINE_CURVE_WITH_KNOTS ( ( 3, 2, 2, 3 ),
 ( 0.1567164179104477695, 0.1579601990049751270, 0.1592039800995025123, 0.1604477611940298698 ),
 .UNSPECIFIED. ) 
 CURVE ( )  GEOMETRIC_REPRESENTATION_ITEM ( )  RATIONAL_B_SPLINE_CURVE ( ( 1.000000000000000000, 0.8660254037844387076, 1.000000000000000000, 0.8660254037844387076, 1.000000000000000000, 0.8660254037844357100, 1.000000000000003109 ) ) 
 REPRESENTATION_ITEM ( '' )  );
#36692=CARTESIAN_POINT ( 'NONE',  ( -5.000000000000003553, -8.660254037844383745, -26.87500000409676204 ) ) ;
#36695=CARTESIAN_POINT ( 'NONE',  ( -10.81189881249999729, 1.324075727343319199E-15, -110.2812500020483810 ) ) ;
#36696=ORIENTED_EDGE ( 'NONE', *, *, #22279, .F. ) ;
#36700=ORIENTED_EDGE ( 'NONE', *, *, #40000, .F. ) ;
#36701=CARTESIAN_POINT ( 'NONE',  ( 9.999999999999996447, -5.773502691896262640, -33.62499999999997158 ) ) ;
#36702=AXIS2_PLACEMENT_3D ( 'NONE', #17255, #30458, #14004 ) ;
#36703=CARTESIAN_POINT ( 'NONE',  ( 10.81189881249999729, 0.000000000000000000, -34.53125000204837391 ) ) ;
#36704=CARTESIAN_POINT ( 'NONE',  ( 9.999999999999998224, 0.000000000000000000, -29.37500000409676204 ) ) ;
#36706=CARTESIAN_POINT ( 'NONE',  ( 10.00000000000000000, 5.773502691896255534, -133.8750000000000000 ) ) ;
#36707=CARTESIAN_POINT ( 'NONE',  ( -5.405949406250003975, -9.363379034771801557, -141.5312500020483810 ) ) ;
#36709=ORIENTED_EDGE ( 'NONE', *, *, #12040, .F. ) ;
#36710=VERTEX_POINT ( 'NONE', #27567 ) ;
#36712=CARTESIAN_POINT ( 'NONE',  ( -9.999999999999998224, 1.224646799147353059E-15, -121.6250000040967905 ) ) ;
#36713=CARTESIAN_POINT ( 'NONE',  ( -10.81189881249999729, 6.242252689847871849, -167.2187500020483810 ) ) ;
#36715=ADVANCED_FACE ( 'NONE', ( #10508 ), #24344, .T. ) ;
#36716=CARTESIAN_POINT ( 'NONE',  ( 5.405949406249992428, -9.363379034771808662, -19.59375000204835615 ) ) ;
#36717=PLANE ( 'NONE',  #36374 ) ;
#36719=CARTESIAN_POINT ( 'NONE',  ( 5.405949406249999534, 9.363379034771803333, -160.0937500020484094 ) ) ;
#36720=CARTESIAN_POINT ( 'NONE',  ( 5.405949406249999534, 9.363379034771803333, -140.5937500020483810 ) ) ;
#36725=CARTESIAN_POINT ( 'NONE',  ( -2.293366432827344421E-15, -12.48450537969573659, -10.71875000204836681 ) ) ;
#36727=CARTESIAN_POINT ( 'NONE',  ( 9.999999999999998224, 0.000000000000000000, -63.87500000409676915 ) ) ;
#36729=CARTESIAN_POINT ( 'NONE',  ( 9.999999999999742428, 5.773502691896404748, -125.2500000040967478 ) ) ;
#36731=CARTESIAN_POINT ( 'NONE',  ( 10.00000000000154010, -5.773502691895370020, -17.12499999999992895 ) ) ;
#36732=CARTESIAN_POINT ( 'NONE',  ( 7.644554776091147741E-16, 12.48450537969573659, -84.96875000204838102 ) ) ;
#36733=CARTESIAN_POINT ( 'NONE',  ( -5.405949406249996869, 9.363379034771805109, -62.34375000204836681 ) ) ;
#36734=CARTESIAN_POINT ( 'NONE',  ( -10.81189881249999729, 1.324075727343319199E-15, -45.78125000204838813 ) ) ;
#36736=DIRECTION ( 'NONE',  ( -0.000000000000000000, -0.000000000000000000, 1.000000000000000000 ) ) ;
#36738=CARTESIAN_POINT ( 'NONE',  ( -2.121150477449813534E-15, -11.54700538379251284, -126.8749999999999858 ) ) ;
#36739=CARTESIAN_POINT ( 'NONE',  ( 10.81189881249999551, -6.242252689847874514, -141.1562500020484094 ) ) ;
#36740=FACE_OUTER_BOUND ( 'NONE', #36906, .T. ) ;
#36742=CARTESIAN_POINT ( 'NONE',  ( 10.81189881249999729, 0.000000000000000000, -21.03125000204836326 ) ) ;
#36748=CARTESIAN_POINT ( 'NONE',  ( -5.000000000000003553, -8.660254037844383745, -40.37500000409677625 ) ) ;
#36750=CARTESIAN_POINT ( 'NONE',  ( -2.121150477449813534E-15, -11.54700538379251284, -58.25000000409677625 ) ) ;
#36752=CARTESIAN_POINT ( 'NONE',  ( 10.00000000000051159, -5.773502691895965988, -146.1250000000000284 ) ) ;
#36753=CARTESIAN_POINT ( 'NONE',  ( 7.644554776091147741E-16, 12.48450537969573659, -152.6562500020484094 ) ) ;
#36754=EDGE_CURVE ( 'NONE', #42281, #24195, #36853, .T. ) ;
#36755=CARTESIAN_POINT ( 'NONE',  ( -10.81189881249999729, 6.242252689847871849, -137.2187500020483810 ) ) ;
#36756=CARTESIAN_POINT ( 'NONE',  ( -5.000000000000003553, -8.660254037844383745, -23.49999999999996447 ) ) ;
#36758=ADVANCED_FACE ( 'NONE', ( #40702, #37703 ), #31027, .F. ) ;
#36759=ORIENTED_EDGE ( 'NONE', *, *, #21422, .F. ) ;
#36760=CARTESIAN_POINT ( 'NONE',  ( -5.000000000000003553, -8.660254037844383745, -30.99999999999997158 ) ) ;
#36761=CARTESIAN_POINT ( 'NONE',  ( -10.81189881249999907, -6.242252689847864744, -65.15625000204838102 ) ) ;
#36762=EDGE_LOOP ( 'NONE', ( #12963, #26613, #25607, #14770 ) ) ;
#36764=CARTESIAN_POINT ( 'NONE',  ( 10.81189881249999551, -6.242252689847874514, -122.9687500020483810 ) ) ;
#36765=ORIENTED_EDGE ( 'NONE', *, *, #16143, .F. ) ;
#36766=CARTESIAN_POINT ( 'NONE',  ( -10.81189881249999729, -6.242252689847864744, -24.46875000204837036 ) ) ;
#36767=CARTESIAN_POINT ( 'NONE',  ( 5.405949406249999534, 9.363379034771803333, -194.5937500020484094 ) ) ;
#36768=CARTESIAN_POINT ( 'NONE',  ( 5.405949406249992428, -9.363379034771808662, -51.09375000204835260 ) ) ;
#36769=CARTESIAN_POINT ( 'NONE',  ( 10.00000000000038369, -5.773502691896038819, -155.5000000040967905 ) ) ;
#36770=FACE_OUTER_BOUND ( 'NONE', #22497, .T. ) ;
#36771=CARTESIAN_POINT ( 'NONE',  ( 7.644554776091147741E-16, 12.48450537969573659, -183.9687500020484663 ) ) ;
#36772=CARTESIAN_POINT ( 'NONE',  ( -5.405949406250003975, -9.363379034771801557, -162.3437500020484094 ) ) ;
#36775=EDGE_CURVE ( 'NONE', #9067, #35021, #34695, .T. ) ;
#36776=CARTESIAN_POINT ( 'NONE',  ( 4.999999999999992006, -8.660254037844389075, -118.1250000040967905 ) ) ;
#36777=DIRECTION ( 'NONE',  ( -0.000000000000000000, -0.000000000000000000, 1.000000000000000000 ) ) ;
#36779=EDGE_CURVE ( 'NONE', #982, #6545, #37998, .T. ) ;
#36780=CARTESIAN_POINT ( 'NONE',  ( -5.405949406249996869, 9.363379034771805109, -98.34375000204838102 ) ) ;
#36782=CARTESIAN_POINT ( 'NONE',  ( 5.405949406249999534, 9.363379034771803333, -70.28125000204838102 ) ) ;
#36783=CARTESIAN_POINT ( 'NONE',  ( 9.999999999999998224, 0.000000000000000000, -146.3750000040967905 ) ) ;
#36785=CARTESIAN_POINT ( 'NONE',  ( 10.81189881249999729, 0.000000000000000000, -118.5312500020483952 ) ) ;
#36786=CARTESIAN_POINT ( 'NONE',  ( 7.644554776091147741E-16, 12.48450537969573659, -158.6562500020484094 ) ) ;
#36788=CARTESIAN_POINT ( 'NONE',  ( 9.999999999999998224, 0.000000000000000000, -140.3750000040967905 ) ) ;
#36793=CARTESIAN_POINT ( 'NONE',  ( 10.81189881249999551, -6.242252689847874514, -189.1562500020484379 ) ) ;
#36795=VERTEX_POINT ( 'NONE', #38338 ) ;
#36796=CARTESIAN_POINT ( 'NONE',  ( -9.999999999999998224, 1.224646799147353059E-15, -46.24999999999998579 ) ) ;
#36798=CARTESIAN_POINT ( 'NONE',  ( 10.00000000000000000, 5.773502691896255534, -69.75000000409679046 ) ) ;
#36802=CARTESIAN_POINT ( 'NONE',  ( 7.644554776091147741E-16, 12.48450537969573659, -59.65625000204838813 ) ) ;
#36803=ADVANCED_FACE ( 'NONE', ( #28644 ), #18050, .T. ) ;
#36806=CARTESIAN_POINT ( 'NONE',  ( -9.999999999999525713, -2.663671193123883896, -0.06732983108239683212 ) ) ;
#36807=CARTESIAN_POINT ( 'NONE',  ( -5.405949406250003975, -9.363379034771801557, -185.0312500020484094 ) ) ;
#36809=CARTESIAN_POINT ( 'NONE',  ( -2.293366432827344421E-15, -12.48450537969573659, -0.2187500020483489072 ) ) ;
#36810=LINE ( 'NONE', #42636, #8946 ) ;
#36811=( BOUNDED_CURVE ( )  B_SPLINE_CURVE ( 2, ( #2373, #8204, #8842, #11844, #21787, #31945, #21574 ),
 .UNSPECIFIED., .F., .F. ) 
 B_SPLINE_CURVE_WITH_KNOTS ( ( 3, 2, 2, 3 ),
 ( 0.2425373134328359381, 0.2437810945273632957, 0.2450248756218906532, 0.2462686567164180107 ),
 .UNSPECIFIED. ) 
 CURVE ( )  GEOMETRIC_REPRESENTATION_ITEM ( )  RATIONAL_B_SPLINE_CURVE ( ( 0.9999999999999880096, 0.8660254037844506980, 1.000000000000000000, 0.8660254037844387076, 1.000000000000000000, 0.8660254037844267172, 1.000000000000011990 ) ) 
 REPRESENTATION_ITEM ( '' )  );
#36812=CARTESIAN_POINT ( 'NONE',  ( 4.999999999999992006, -8.660254037844389075, -89.24999999999998579 ) ) ;
#36814=CARTESIAN_POINT ( 'NONE',  ( -9.999999999999998224, 1.224646799147353059E-15, -80.74999999999998579 ) ) ;
#36815=CARTESIAN_POINT ( 'NONE',  ( -5.405949406250003975, -9.363379034771801557, -87.53125000204838102 ) ) ;
#36817=CARTESIAN_POINT ( 'NONE',  ( 9.999999999999998224, 0.000000000000000000, -167.3750000040967905 ) ) ;
#36818=ORIENTED_EDGE ( 'NONE', *, *, #16142, .T. ) ;
#36820=CARTESIAN_POINT ( 'NONE',  ( -5.405949406249996869, 9.363379034771805109, -24.84375000204835970 ) ) ;
#36821=CARTESIAN_POINT ( 'NONE',  ( 10.81189881249999907, 6.242252689847868297, -25.40625000204838813 ) ) ;
#36822=CARTESIAN_POINT ( 'NONE',  ( 10.81189881249999907, 6.242252689847868297, -74.71875000204838102 ) ) ;
#36823=CARTESIAN_POINT ( 'NONE',  ( -9.999999999999998224, 1.224646799147353059E-15, -84.12500000409677625 ) ) ;
#36825=CARTESIAN_POINT ( 'NONE',  ( 10.81189881249999729, 0.000000000000000000, -193.3437500020484094 ) ) ;
#36826=CARTESIAN_POINT ( 'NONE',  ( 5.405949406249992428, -9.363379034771808662, -153.0937500020483810 ) ) ;
#36827=CARTESIAN_POINT ( 'NONE',  ( -5.405949406250003975, -9.363379034771801557, -0.3437500020483652552 ) ) ;
#36828=FACE_OUTER_BOUND ( 'NONE', #2842, .T. ) ;
#36829=CARTESIAN_POINT ( 'NONE',  ( 7.070501591499376803E-16, 11.54700538379251284, -112.6249999999999858 ) ) ;
#36830=CARTESIAN_POINT ( 'NONE',  ( -10.00000000000000000, -5.773502691896251982, -3.000000004096758044 ) ) ;
#36831=DIRECTION ( 'NONE',  ( -0.000000000000000000, -0.000000000000000000, 1.000000000000000000 ) ) ;
#36832=CARTESIAN_POINT ( 'NONE',  ( 10.81189881249999551, -6.242252689847874514, -121.4687500020484094 ) ) ;
#36834=CARTESIAN_POINT ( 'NONE',  ( 10.81189881249999729, 0.000000000000000000, -87.03125000204838102 ) ) ;
#36835=CARTESIAN_POINT ( 'NONE',  ( 7.644554776091147741E-16, 12.48450537969573659, -96.96875000204838102 ) ) ;
#36838=CARTESIAN_POINT ( 'NONE',  ( -9.999999999999998224, 5.773502691896259087, -162.2500000040967620 ) ) ;
#36841=EDGE_CURVE ( 'NONE', #2222, #29057, #27997, .T. ) ;
#36842=CARTESIAN_POINT ( 'NONE',  ( -9.999999999999998224, 1.224646799147353059E-15, -200.0000000000000000 ) ) ;
#36844=CARTESIAN_POINT ( 'NONE',  ( 9.999999999999998224, 0.000000000000000000, -53.37500000409675494 ) ) ;
#36847=CARTESIAN_POINT ( 'NONE',  ( -2.121150477449813534E-15, -11.54700538379251284, -78.87500000000000000 ) ) ;
#36849=CARTESIAN_POINT ( 'NONE',  ( -9.999999999999998224, 5.773502691896259087, -88.75000000409677625 ) ) ;
#36850=CARTESIAN_POINT ( 'NONE',  ( 0.000000000000000000, 0.000000000000000000, -200.0000000000000000 ) ) ;
#36852=CARTESIAN_POINT ( 'NONE',  ( -2.293366432827344421E-15, -12.48450537969573659, -81.40625000204838102 ) ) ;
#36853=( BOUNDED_CURVE ( )  B_SPLINE_CURVE ( 2, ( #24126, #37267, #20864, #30807, #4470, #34048, #17612 ),
 .UNSPECIFIED., .F., .F. ) 
 B_SPLINE_CURVE_WITH_KNOTS ( ( 3, 2, 2, 3 ),
 ( 0.2238805970149254365, 0.2251243781094527940, 0.2263681592039801793, 0.2276119402985075368 ),
 .UNSPECIFIED. ) 
 CURVE ( )  GEOMETRIC_REPRESENTATION_ITEM ( )  RATIONAL_B_SPLINE_CURVE ( ( 0.9999999999999940048, 0.8660254037844447028, 1.000000000000000000, 0.8660254037844387076, 1.000000000000000000, 0.8660254037844297148, 1.000000000000008882 ) ) 
 REPRESENTATION_ITEM ( '' )  );
#36857=ORIENTED_EDGE ( 'NONE', *, *, #22229, .T. ) ;
#36858=CARTESIAN_POINT ( 'NONE',  ( -9.999999999999998224, 5.773502691896259087, -8.874999999999976907 ) ) ;
#36860=CARTESIAN_POINT ( 'NONE',  ( -9.999999999999998224, 1.224646799147353059E-15, -143.7500000000000000 ) ) ;
#36864=AXIS2_PLACEMENT_3D ( 'NONE', #36850, #1253, #14377 ) ;
#36865=CARTESIAN_POINT ( 'NONE',  ( 9.999999999999998224, 0.000000000000000000, -194.0000000000000000 ) ) ;
#36866=DIRECTION ( 'NONE',  ( -0.000000000000000000, -0.000000000000000000, 1.000000000000000000 ) ) ;
#36867=CARTESIAN_POINT ( 'NONE',  ( -10.81189881249999729, 1.324075727343319199E-15, -114.7812500020483952 ) ) ;
#36868=ORIENTED_EDGE ( 'NONE', *, *, #37982, .T. ) ;
#36870=ORIENTED_EDGE ( 'NONE', *, *, #10491, .F. ) ;
#36872=CARTESIAN_POINT ( 'NONE',  ( 5.405949406249999534, 9.363379034771803333, -46.28125000204838813 ) ) ;
#36874=CARTESIAN_POINT ( 'NONE',  ( -10.81189881249999729, 6.242252689847871849, -93.71875000204838102 ) ) ;
#36875=CARTESIAN_POINT ( 'NONE',  ( 5.405949406249999534, 9.363379034771803333, -127.2812500020483810 ) ) ;
#36876=EDGE_LOOP ( 'NONE', ( #27646, #15449, #33574, #41300 ) ) ;
#36877=CARTESIAN_POINT ( 'NONE',  ( 4.999999999999992006, -8.660254037844389075, -83.24999999999997158 ) ) ;
#36878=CARTESIAN_POINT ( 'NONE',  ( -10.81189881249999729, 6.242252689847871849, -195.7187500020484379 ) ) ;
#36880=CARTESIAN_POINT ( 'NONE',  ( -9.999999999999227285, -5.773502691896698735, -139.1249999999999716 ) ) ;
#36881=CARTESIAN_POINT ( 'NONE',  ( -10.81189881249999729, -6.242252689847864744, -120.4687500020483952 ) ) ;
#36885=CARTESIAN_POINT ( 'NONE',  ( 9.999999999999996447, -5.773502691896262640, -187.0000000040968189 ) ) ;
#36887=CARTESIAN_POINT ( 'NONE',  ( 7.644554776091147741E-16, 12.48450537969573659, -181.1562500020484379 ) ) ;
#36890=CARTESIAN_POINT ( 'NONE',  ( 9.999999999999479527, 5.773502691896553074, -3.374999999999938716 ) ) ;
#36891=CARTESIAN_POINT ( 'NONE',  ( 5.000000000000000000, 8.660254037844385522, -122.1250000040967905 ) ) ;
#36893=CARTESIAN_POINT ( 'NONE',  ( -5.405949406249996869, 9.363379034771805109, -57.84375000204835970 ) ) ;
#36894=CARTESIAN_POINT ( 'NONE',  ( 7.644554776091147741E-16, 12.48450537969573659, -39.96875000204835970 ) ) ;
#36896=CARTESIAN_POINT ( 'NONE',  ( 7.644554776091147741E-16, 12.48450537969573659, -20.65625000204838102 ) ) ;
#36900=CARTESIAN_POINT ( 'NONE',  ( -9.999999999999998224, 1.224646799147353059E-15, -104.7499999999999858 ) ) ;
#36902=DIRECTION ( 'NONE',  ( -1.000000000000000000, 0.000000000000000000, 0.000000000000000000 ) ) ;
#36905=CARTESIAN_POINT ( 'NONE',  ( 7.644554776091147741E-16, 12.48450537969573659, -107.6562500020483810 ) ) ;
#36906=EDGE_LOOP ( 'NONE', ( #35144, #15349, #8753, #40602 ) ) ;
#36909=FACE_OUTER_BOUND ( 'NONE', #4075, .T. ) ;
#36912=CARTESIAN_POINT ( 'NONE',  ( -5.000000000000003553, -8.660254037844383745, -36.99999999999997868 ) ) ;
#36913=CARTESIAN_POINT ( 'NONE',  ( 10.81189881249999729, 0.000000000000000000, -37.53125000204838102 ) ) ;
#36914=EDGE_CURVE ( 'NONE', #41090, #26035, #19203, .T. ) ;
#36917=AXIS2_PLACEMENT_3D ( 'NONE', #21525, #25000, #5128 ) ;
#36918=VECTOR ( 'NONE', #33386, 1000.000000000000000 ) ;
#36919=CARTESIAN_POINT ( 'NONE',  ( -9.999999999999998224, 1.224646799147353059E-15, -90.12500000409677625 ) ) ;
#36920=CARTESIAN_POINT ( 'NONE',  ( -10.81189881249999729, 1.324075727343319199E-15, -141.7812500020483810 ) ) ;
#36924=ORIENTED_EDGE ( 'NONE', *, *, #31765, .T. ) ;
#36925=CARTESIAN_POINT ( 'NONE',  ( -9.999999999999998224, 1.224646799147353059E-15, -106.6250000040967763 ) ) ;
#36926=CARTESIAN_POINT ( 'NONE',  ( -9.999999999999998224, 1.224646799147353059E-15, -200.0000000000000000 ) ) ;
#36927=CARTESIAN_POINT ( 'NONE',  ( -10.81189881249999729, 1.324075727343319199E-15, -167.0937500020484094 ) ) ;
#36929=CARTESIAN_POINT ( 'NONE',  ( 5.405949406249992428, -9.363379034771808662, -15.09375000204835082 ) ) ;
#36930=DIRECTION ( 'NONE',  ( 1.000000000000000000, 0.000000000000000000, 0.000000000000000000 ) ) ;
#36931=CARTESIAN_POINT ( 'NONE',  ( 5.405949406249992428, -9.363379034771808662, -154.5937500020483810 ) ) ;
#36932=CARTESIAN_POINT ( 'NONE',  ( 5.405949406249999534, 9.363379034771803333, -136.0937500020483810 ) ) ;
#36933=( BOUNDED_CURVE ( )  B_SPLINE_CURVE ( 2, ( #13853, #41899, #5675, #32219, #35456, #38252, #41256 ),
 .UNSPECIFIED., .F., .F. ) 
 B_SPLINE_CURVE_WITH_KNOTS ( ( 3, 2, 2, 3 ),
 ( 0.8731343283582092551, 0.8743781094527366404, 0.8756218905472639147, 0.8768656716417913000 ),
 .UNSPECIFIED. ) 
 CURVE ( )  GEOMETRIC_REPRESENTATION_ITEM ( )  RATIONAL_B_SPLINE_CURVE ( ( 0.9999999999999641398, 0.8660254037844745678, 1.000000000000000000, 0.8660254037844387076, 1.000000000000000000, 0.8660254037844148378, 1.000000000000023981 ) ) 
 REPRESENTATION_ITEM ( '' )  );
#36934=CARTESIAN_POINT ( 'NONE',  ( -5.405949406250003975, -9.363379034771801557, -110.0312500020483810 ) ) ;
#36937=VECTOR ( 'NONE', #26910, 1000.000000000000000 ) ;
#36939=CARTESIAN_POINT ( 'NONE',  ( -10.81189881249999907, -6.242252689847864744, -6.468750002048346381 ) ) ;
#36942=CARTESIAN_POINT ( 'NONE',  ( -9.999999999999998224, 1.224646799147353059E-15, -99.12500000409677625 ) ) ;
#36945=CARTESIAN_POINT ( 'NONE',  ( -5.405949406249996869, 9.363379034771805109, -83.34375000204836681 ) ) ;
#36946=CARTESIAN_POINT ( 'NONE',  ( 5.405949406249999534, 9.363379034771803333, -67.09375000204836681 ) ) ;
#36948=CARTESIAN_POINT ( 'NONE',  ( 10.81189881249999551, -6.242252689847874514, -42.15625000204836681 ) ) ;
#36952=CARTESIAN_POINT ( 'NONE',  ( -4.999999999999996447, 8.660254037844387298, -132.0000000000000000 ) ) ;
#36953=CARTESIAN_POINT ( 'NONE',  ( 5.405949406249992428, -9.363379034771808662, -130.7812500020483810 ) ) ;
#36956=CARTESIAN_POINT ( 'NONE',  ( -10.81189881249999729, -6.242252689847864744, -17.15625000204838102 ) ) ;
#36957=VERTEX_POINT ( 'NONE', #35331 ) ;
#36960=LINE ( 'NONE', #3743, #19463 ) ;
#36961=CARTESIAN_POINT ( 'NONE',  ( -2.121150477449813534E-15, -11.54700538379251284, -35.75000000409675494 ) ) ;
#36964=CARTESIAN_POINT ( 'NONE',  ( 9.999999999999998224, 0.000000000000000000, -76.99999999999998579 ) ) ;
#36965=CARTESIAN_POINT ( 'NONE',  ( 7.644554776091147741E-16, 12.48450537969573659, -149.6562500020484094 ) ) ;
#36966=CARTESIAN_POINT ( 'NONE',  ( -5.405949406250003975, -9.363379034771801557, -132.3437500020484094 ) ) ;
#36967=CARTESIAN_POINT ( 'NONE',  ( 5.000000000000000000, 8.660254037844385522, -144.2500000000000000 ) ) ;
#36968=EDGE_CURVE ( 'NONE', #25614, #4287, #15906, .T. ) ;
#36969=ORIENTED_EDGE ( 'NONE', *, *, #41499, .T. ) ;
#36970=EDGE_CURVE ( 'NONE', #14017, #37834, #23629, .T. ) ;
#36971=FACE_OUTER_BOUND ( 'NONE', #26776, .T. ) ;
#36973=VERTEX_POINT ( 'NONE', #12002 ) ;
#36974=CARTESIAN_POINT ( 'NONE',  ( 7.644554776091147741E-16, 12.48450537969573659, -59.65625000204838813 ) ) ;
#36977=CARTESIAN_POINT ( 'NONE',  ( 5.405949406249999534, 9.363379034771803333, -110.5937500020483810 ) ) ;
#36979=CARTESIAN_POINT ( 'NONE',  ( 10.81189881249999729, 6.242252689847867408, -25.21875000204837036 ) ) ;
#36980=( BOUNDED_CURVE ( )  B_SPLINE_CURVE ( 2, ( #38566, #2546, #28873, #24792, #28455, #34926, #42007 ),
 .UNSPECIFIED., .F., .F. ) 
 B_SPLINE_CURVE_WITH_KNOTS ( ( 3, 2, 2, 3 ),
 ( 0.8022388059701494045, 0.8034825870646766788, 0.8047263681592041751, 0.8059701492537315604 ),
 .UNSPECIFIED. ) 
 CURVE ( )  GEOMETRIC_REPRESENTATION_ITEM ( )  RATIONAL_B_SPLINE_CURVE ( ( 0.9999999999999880096, 0.8660254037844506980, 1.000000000000000000, 0.8660254037844387076, 1.000000000000000000, 0.8660254037844148378, 1.000000000000023981 ) ) 
 REPRESENTATION_ITEM ( '' )  );
#36981=CARTESIAN_POINT ( 'NONE',  ( 5.405949406249992428, -9.363379034771808662, -189.0937500020483810 ) ) ;
#36982=CARTESIAN_POINT ( 'NONE',  ( -10.81189881249999729, 6.242252689847871849, -36.71875000204835970 ) ) ;
#36983=CARTESIAN_POINT ( 'NONE',  ( -8.461552159095841574, -5.381368393490791213, 7.703719777548943412E-31 ) ) ;
#36984=CARTESIAN_POINT ( 'NONE',  ( 9.999999999999998224, 0.000000000000000000, -152.3750000040967905 ) ) ;
#36985=CARTESIAN_POINT ( 'NONE',  ( 5.405949406249999534, 9.363379034771803333, -179.5937500020484094 ) ) ;
#36986=CARTESIAN_POINT ( 'NONE',  ( -5.405949406250003975, -9.363379034771801557, -160.8437500020484094 ) ) ;
#36989=CARTESIAN_POINT ( 'NONE',  ( -5.000000000000003553, -8.660254037844383745, -42.99999999999998579 ) ) ;
#36990=( BOUNDED_CURVE ( )  B_SPLINE_CURVE ( 2, ( #5045, #18190, #14294, #11069, #31382, #7639, #24911 ),
 .UNSPECIFIED., .F., .F. ) 
 B_SPLINE_CURVE_WITH_KNOTS ( ( 3, 2, 2, 3 ),
 ( 0.6082089552238807428, 0.6094527363184080171, 0.6106965174129354024, 0.6119402985074627876 ),
 .UNSPECIFIED. ) 
 CURVE ( )  GEOMETRIC_REPRESENTATION_ITEM ( )  RATIONAL_B_SPLINE_CURVE ( ( 0.9999999999999880096, 0.8660254037844506980, 1.000000000000000000, 0.8660254037844387076, 1.000000000000000000, 0.8660254037844267172, 1.000000000000011990 ) ) 
 REPRESENTATION_ITEM ( '' )  );
#36991=CARTESIAN_POINT ( 'NONE',  ( -9.999999999999998224, 1.224646799147353059E-15, -187.6250000040967905 ) ) ;
#36993=CARTESIAN_POINT ( 'NONE',  ( 10.81189881249999551, -6.242252689847874514, -92.96875000204838102 ) ) ;
#36994=CARTESIAN_POINT ( 'NONE',  ( -9.999999999999998224, 1.224646799147353059E-15, -200.0000000000000000 ) ) ;
#36995=CARTESIAN_POINT ( 'NONE',  ( -10.81189881249999729, 1.324075727343319199E-15, -65.28125000204838102 ) ) ;
#36998=CARTESIAN_POINT ( 'NONE',  ( -10.81189881249999729, 1.324075727343319199E-15, -122.2812500020483952 ) ) ;
#36999=CARTESIAN_POINT ( 'NONE',  ( 10.81189881249999729, 6.242252689847867408, -164.9062500020484094 ) ) ;
#37001=CARTESIAN_POINT ( 'NONE',  ( -10.00000000000000000, -5.773502691896251982, -127.5000000040967905 ) ) ;
#37003=ORIENTED_EDGE ( 'NONE', *, *, #27372, .T. ) ;
#37007=CARTESIAN_POINT ( 'NONE',  ( -5.405949406249996869, 9.363379034771805109, -185.5312500020484094 ) ) ;
#37010=CARTESIAN_POINT ( 'NONE',  ( -4.999999999999996447, 8.660254037844387298, -47.99999999999998579 ) ) ;
#37012=CARTESIAN_POINT ( 'NONE',  ( 9.999999999999998224, 0.000000000000000000, -68.37500000409677625 ) ) ;
#37013=CARTESIAN_POINT ( 'NONE',  ( -9.999999999999998224, 1.224646799147353059E-15, -179.7500000000000284 ) ) ;
#37016=CARTESIAN_POINT ( 'NONE',  ( 10.81189881249999729, 0.000000000000000000, -63.03125000204837391 ) ) ;
#37019=CARTESIAN_POINT ( 'NONE',  ( 9.999999999999998224, 0.000000000000000000, -158.3750000040967905 ) ) ;
#37020=CARTESIAN_POINT ( 'NONE',  ( 10.81189881249999729, 0.000000000000000000, -174.0312500020484094 ) ) ;
#37022=DIRECTION ( 'NONE',  ( -0.000000000000000000, -0.000000000000000000, 1.000000000000000000 ) ) ;
#37025=CARTESIAN_POINT ( 'NONE',  ( -9.999999999999479527, -5.773502691896549521, -89.62499999999997158 ) ) ;
#37026=FACE_OUTER_BOUND ( 'NONE', #2967, .T. ) ;
#37027=ADVANCED_FACE ( 'NONE', ( #29265 ), #36371, .T. ) ;
#37028=LINE ( 'NONE', #14118, #14453 ) ;
#37029=ADVANCED_FACE ( 'NONE', ( #35541 ), #1062, .F. ) ;
#37030=CARTESIAN_POINT ( 'NONE',  ( 10.81189881249999729, 0.000000000000000000, -82.53125000204838102 ) ) ;
#37031=EDGE_LOOP ( 'NONE', ( #27163, #2699, #37177, #41649 ) ) ;
#37032=LINE ( 'NONE', #21266, #11637 ) ;
#37033=ORIENTED_EDGE ( 'NONE', *, *, #15152, .T. ) ;
#37035=ORIENTED_EDGE ( 'NONE', *, *, #25204, .T. ) ;
#37036=CARTESIAN_POINT ( 'NONE',  ( 10.81189881249999907, 6.242252689847868297, -23.71875000204836326 ) ) ;
#37037=CARTESIAN_POINT ( 'NONE',  ( 10.81189881249999907, 6.242252689847868297, -10.40625000204838102 ) ) ;
#37038=CARTESIAN_POINT ( 'NONE',  ( 5.405949406249992428, -9.363379034771808662, -67.59375000204836681 ) ) ;
#37041=CARTESIAN_POINT ( 'NONE',  ( 10.81189881249999907, 6.242252689847868297, -184.2187500020483810 ) ) ;
#37043=CARTESIAN_POINT ( 'NONE',  ( -5.405949406249996869, 9.363379034771805109, -0.8437500020483656993 ) ) ;
#37044=CARTESIAN_POINT ( 'NONE',  ( -10.00000000000154188, 5.773502691895366468, -58.75000000409671941 ) ) ;
#37047=EDGE_CURVE ( 'NONE', #25274, #18020, #3239, .T. ) ;
#37048=CARTESIAN_POINT ( 'NONE',  ( -10.81189881249999729, 6.242252689847871849, -111.7187500020483810 ) ) ;
#37050=CARTESIAN_POINT ( 'NONE',  ( -10.81189881249999729, 1.324075727343319199E-15, -93.78125000204838102 ) ) ;
#37051=CARTESIAN_POINT ( 'NONE',  ( 7.644554776091147741E-16, 12.48450537969573659, -102.9687500020483668 ) ) ;
#37054=CARTESIAN_POINT ( 'NONE',  ( -9.999999999999998224, 1.224646799147353059E-15, -159.1250000040967905 ) ) ;
#37059=CARTESIAN_POINT ( 'NONE',  ( 0.000000000000000000, 0.000000000000000000, -200.0000000000000000 ) ) ;
#37060=CARTESIAN_POINT ( 'NONE',  ( -9.999999999999998224, 5.773502691896259087, -71.87500000000000000 ) ) ;
#37062=CARTESIAN_POINT ( 'NONE',  ( 9.999999999999996447, -5.773502691896262640, -91.00000000409677625 ) ) ;
#37063=( BOUNDED_CURVE ( )  B_SPLINE_CURVE ( 2, ( #17887, #10778, #36692, #31085, #40546, #1085, #7985 ),
 .UNSPECIFIED., .F., .F. ) 
 B_SPLINE_CURVE_WITH_KNOTS ( ( 3, 2, 2, 3 ),
 ( 0.8544776119402988090, 0.8557213930348261943, 0.8569651741293534686, 0.8582089552238808539 ),
 .UNSPECIFIED. ) 
 CURVE ( )  GEOMETRIC_REPRESENTATION_ITEM ( )  RATIONAL_B_SPLINE_CURVE ( ( 0.9999999999999641398, 0.8660254037844745678, 1.000000000000000000, 0.8660254037844387076, 1.000000000000000000, 0.8660254037844148378, 1.000000000000023981 ) ) 
 REPRESENTATION_ITEM ( '' )  );
#37065=CARTESIAN_POINT ( 'NONE',  ( 10.81189881249999729, 0.000000000000000000, -82.53125000204838102 ) ) ;
#37067=CARTESIAN_POINT ( 'NONE',  ( 9.999999999998969713, 5.773502691896851502, -19.87499999999994316 ) ) ;
#37070=CARTESIAN_POINT ( 'NONE',  ( 5.000000000000000000, 8.660254037844385522, -0.2499999999999724665 ) ) ;
#37072=CARTESIAN_POINT ( 'NONE',  ( -10.81189881249999729, 1.324075727343319199E-15, -14.09375000204834905 ) ) ;
#37073=CARTESIAN_POINT ( 'NONE',  ( 9.999999999999998224, 0.000000000000000000, -14.37500000409674961 ) ) ;
#37075=CARTESIAN_POINT ( 'NONE',  ( -10.81189881249999729, 1.324075727343319199E-15, -135.7812500020483810 ) ) ;
#37076=CARTESIAN_POINT ( 'NONE',  ( -2.121150477449813534E-15, -11.54700538379251284, -186.8750000000000284 ) ) ;
#37077=CARTESIAN_POINT ( 'NONE',  ( -10.81189881249999729, 6.242252689847871849, -110.4062500020483810 ) ) ;
#37079=DIRECTION ( 'NONE',  ( -0.000000000000000000, -0.000000000000000000, 1.000000000000000000 ) ) ;
#37081=ORIENTED_EDGE ( 'NONE', *, *, #4042, .T. ) ;
#37082=EDGE_LOOP ( 'NONE', ( #33009, #35827, #8447, #23002 ) ) ;
#37083=CARTESIAN_POINT ( 'NONE',  ( 7.644554776091147741E-16, 12.48450537969573659, -44.65625000204836681 ) ) ;
#37085=EDGE_CURVE ( 'NONE', #16098, #17857, #16365, .T. ) ;
#37086=CARTESIAN_POINT ( 'NONE',  ( 10.81189881249999907, 6.242252689847868297, -97.21875000204836681 ) ) ;
#37087=PLANE ( 'NONE',  #36018 ) ;
#37088=CARTESIAN_POINT ( 'NONE',  ( 10.00000000000012790, 5.773502691896179151, -174.3750000000000000 ) ) ;
#37089=CARTESIAN_POINT ( 'NONE',  ( 10.81189881249999551, -6.242252689847874514, -194.9687500020484094 ) ) ;
#37091=DIRECTION ( 'NONE',  ( -0.000000000000000000, -0.000000000000000000, 1.000000000000000000 ) ) ;
#37092=CARTESIAN_POINT ( 'NONE',  ( 7.644554776091147741E-16, 12.48450537969573659, -123.9687500020483952 ) ) ;
#37094=CARTESIAN_POINT ( 'NONE',  ( -9.999999999998969713, -5.773502691896847949, -44.62499999999995737 ) ) ;
#37096=CARTESIAN_POINT ( 'NONE',  ( -2.121150477449813534E-15, -11.54700538379251284, -185.7500000040967905 ) ) ;
#37098=CARTESIAN_POINT ( 'NONE',  ( 7.644554776091147741E-16, 12.48450537969573659, -176.6562500020484094 ) ) ;
#37099=( BOUNDED_CURVE ( )  B_SPLINE_CURVE ( 2, ( #10142, #27405, #244, #14206, #33260, #10985, #20491 ),
 .UNSPECIFIED., .F., .F. ) 
 B_SPLINE_CURVE_WITH_KNOTS ( ( 3, 2, 2, 3 ),
 ( 0.3694029850746269883, 0.3706467661691543181, 0.3718905472636816478, 0.3731343283582090331 ),
 .UNSPECIFIED. ) 
 CURVE ( )  GEOMETRIC_REPRESENTATION_ITEM ( )  RATIONAL_B_SPLINE_CURVE ( ( 0.9999999999999880096, 0.8660254037844506980, 1.000000000000000000, 0.8660254037844387076, 1.000000000000000000, 0.8660254037844327124, 1.000000000000005995 ) ) 
 REPRESENTATION_ITEM ( '' )  );
#37100=CARTESIAN_POINT ( 'NONE',  ( -9.999999999999998224, 1.224646799147353059E-15, -200.0000000000000000 ) ) ;
#37102=CARTESIAN_POINT ( 'NONE',  ( 5.405949406249992428, -9.363379034771808662, -52.59375000204835260 ) ) ;
#37103=CARTESIAN_POINT ( 'NONE',  ( 7.644554776091147741E-16, 12.48450537969573659, -41.46875000204835260 ) ) ;
#37105=CARTESIAN_POINT ( 'NONE',  ( -5.405949406250003975, -9.363379034771801557, -11.03125000204835438 ) ) ;
#37109=CARTESIAN_POINT ( 'NONE',  ( -10.00000000000000000, -5.773502691896251982, -94.12499999999998579 ) ) ;
#37111=VECTOR ( 'NONE', #30270, 1000.000000000000000 ) ;
#37112=CARTESIAN_POINT ( 'NONE',  ( 4.999999999999992006, -8.660254037844389075, -49.12500000409678336 ) ) ;
#37115=CARTESIAN_POINT ( 'NONE',  ( -5.405949406249996869, 9.363379034771805109, -104.5312500020483810 ) ) ;
#37116=VERTEX_POINT ( 'NONE', #17385 ) ;
#37117=DIRECTION ( 'NONE',  ( -0.000000000000000000, -0.000000000000000000, 1.000000000000000000 ) ) ;
#37119=CARTESIAN_POINT ( 'NONE',  ( 9.999999999999998224, 0.000000000000000000, -75.87500000409677625 ) ) ;
#37121=ORIENTED_EDGE ( 'NONE', *, *, #19564, .F. ) ;
#37122=CARTESIAN_POINT ( 'NONE',  ( -10.00000000000000000, -5.773502691896251982, -34.12499999999997158 ) ) ;
#37123=CARTESIAN_POINT ( 'NONE',  ( 10.81189881249999729, 6.242252689847867408, -38.90625000204835970 ) ) ;
#37124=CARTESIAN_POINT ( 'NONE',  ( 9.999999999999479527, 5.773502691896553074, -35.25000000409674072 ) ) ;
#37126=CARTESIAN_POINT ( 'NONE',  ( 10.81189881249999907, 6.242252689847868297, -131.9062500020484094 ) ) ;
#37128=ORIENTED_EDGE ( 'NONE', *, *, #17476, .F. ) ;
#37131=AXIS2_PLACEMENT_3D ( 'NONE', #33470, #17031, #670 ) ;
#37133=CYLINDRICAL_SURFACE ( 'NONE', #24243, 9.999999999999998224 ) ;
#37134=CARTESIAN_POINT ( 'NONE',  ( 10.81189881249999907, 6.242252689847868297, -166.2187500020484094 ) ) ;
#37136=CARTESIAN_POINT ( 'NONE',  ( 5.405949406249992428, -9.363379034771808662, -13.59375000204834905 ) ) ;
#37137=CARTESIAN_POINT ( 'NONE',  ( 4.999999999999992006, -8.660254037844389075, -157.1250000040967905 ) ) ;
#37138=CARTESIAN_POINT ( 'NONE',  ( -5.405949406250003975, -9.363379034771801557, -150.3437500020483810 ) ) ;
#37139=CARTESIAN_POINT ( 'NONE',  ( -10.81189881249999907, -6.242252689847864744, -136.9687500020483810 ) ) ;
#37140=CARTESIAN_POINT ( 'NONE',  ( 10.81189881249999907, 6.242252689847868297, -104.9062500020483952 ) ) ;
#37144=CARTESIAN_POINT ( 'NONE',  ( 7.644554776091147741E-16, 12.48450537969573659, -11.46875000204836859 ) ) ;
#37146=EDGE_CURVE ( 'NONE', #19338, #14871, #32218, .T. ) ;
#37148=VECTOR ( 'NONE', #21393, 1000.000000000000000 ) ;
#37149=CARTESIAN_POINT ( 'NONE',  ( 9.999999999999998224, 0.000000000000000000, -179.3750000040967905 ) ) ;
#37152=CARTESIAN_POINT ( 'NONE',  ( 7.644554776091147741E-16, 12.48450537969573659, -72.96875000204836681 ) ) ;
#37153=CARTESIAN_POINT ( 'NONE',  ( -10.81189881249999729, 1.324075727343319199E-15, -65.09375000204836681 ) ) ;
#37154=CARTESIAN_POINT ( 'NONE',  ( -5.405949406249996869, 9.363379034771805109, -34.03125000204837391 ) ) ;
#37156=CARTESIAN_POINT ( 'NONE',  ( 10.00000000000025402, -5.773502691896113426, -139.0000000040967905 ) ) ;
#37158=CARTESIAN_POINT ( 'NONE',  ( -5.000000000000003553, -8.660254037844383745, -127.0000000000000000 ) ) ;
#37159=CARTESIAN_POINT ( 'NONE',  ( 10.81189881249999729, 0.000000000000000000, -133.5312500020484094 ) ) ;
#37160=CARTESIAN_POINT ( 'NONE',  ( -10.00000000000051337, 5.773502691895962435, -94.37499999999997158 ) ) ;
#37162=CARTESIAN_POINT ( 'NONE',  ( 5.405949406249999534, 9.363379034771803333, -16.28125000204835970 ) ) ;
#37167=CARTESIAN_POINT ( 'NONE',  ( -10.00000000000000000, -5.773502691896251982, -31.50000000409674783 ) ) ;
#37170=CARTESIAN_POINT ( 'NONE',  ( -4.999999999999996447, 8.660254037844387298, -76.49999999999998579 ) ) ;
#37171=CARTESIAN_POINT ( 'NONE',  ( -5.405949406249996869, 9.363379034771805109, -149.5312500020483810 ) ) ;
#37173=CARTESIAN_POINT ( 'NONE',  ( -10.81189881249999907, -6.242252689847864744, -136.9687500020483810 ) ) ;
#37175=ORIENTED_EDGE ( 'NONE', *, *, #10650, .F. ) ;
#37177=ORIENTED_EDGE ( 'NONE', *, *, #17957, .F. ) ;
#37178=VECTOR ( 'NONE', #16439, 1000.000000000000000 ) ;
#37180=CARTESIAN_POINT ( 'NONE',  ( 10.81189881249999729, 0.000000000000000000, -109.3437500020483810 ) ) ;
#37181=ORIENTED_EDGE ( 'NONE', *, *, #13936, .T. ) ;
#37183=CARTESIAN_POINT ( 'NONE',  ( 5.000000000000000000, 8.660254037844385522, -129.6250000040967620 ) ) ;
#37184=CARTESIAN_POINT ( 'NONE',  ( 10.81189881249999907, 6.242252689847868297, -190.2187500020484094 ) ) ;
#37185=CARTESIAN_POINT ( 'NONE',  ( 10.81189881249999729, 0.000000000000000000, -38.84375000204837391 ) ) ;
#37186=CARTESIAN_POINT ( 'NONE',  ( -0.8693057687019801749, -10.36909276259400237, -5.090678961559013491E-15 ) ) ;
#37187=DIRECTION ( 'NONE',  ( 1.000000000000000000, 0.000000000000000000, 0.000000000000000000 ) ) ;
#37188=CARTESIAN_POINT ( 'NONE',  ( 10.81189881249999729, 0.000000000000000000, -170.8437500020484094 ) ) ;
#37189=CARTESIAN_POINT ( 'NONE',  ( -5.405949406249996869, 9.363379034771805109, -158.3437500020483810 ) ) ;
#37190=CARTESIAN_POINT ( 'NONE',  ( -9.999999999999998224, 1.224646799147353059E-15, -66.12500000409676204 ) ) ;
#37193=CARTESIAN_POINT ( 'NONE',  ( 4.999999999999992006, -8.660254037844389075, -155.2500000000000000 ) ) ;
#37196=VECTOR ( 'NONE', #4702, 1000.000000000000000 ) ;
#37197=CARTESIAN_POINT ( 'NONE',  ( -10.81189881249999907, -6.242252689847864744, -85.96875000204836681 ) ) ;
#37199=CARTESIAN_POINT ( 'NONE',  ( -10.81189881249999907, -6.242252689847864744, -57.65625000204838102 ) ) ;
#37200=CARTESIAN_POINT ( 'NONE',  ( 9.999999999998969713, 5.773502691896851502, -87.75000000409674783 ) ) ;
#37203=CARTESIAN_POINT ( 'NONE',  ( -10.81189881249999907, -6.242252689847864744, -125.1562500020483810 ) ) ;
#37204=CARTESIAN_POINT ( 'NONE',  ( 5.405949406249999534, 9.363379034771803333, -152.7812500020484094 ) ) ;
#37207=CARTESIAN_POINT ( 'NONE',  ( -10.00000000000000000, -5.773502691896251982, -129.0000000040967905 ) ) ;
#37209=VERTEX_POINT ( 'NONE', #804 ) ;
#37213=CARTESIAN_POINT ( 'NONE',  ( 5.405949406249992428, -9.363379034771808662, -192.2812500020484094 ) ) ;
#37214=VERTEX_POINT ( 'NONE', #33610 ) ;
#37215=CARTESIAN_POINT ( 'NONE',  ( 9.999999999999998224, 0.000000000000000000, -52.99999999999996447 ) ) ;
#37217=CARTESIAN_POINT ( 'NONE',  ( -5.000000000000003553, -8.660254037844383745, -61.37500000409676204 ) ) ;
#37218=CARTESIAN_POINT ( 'NONE',  ( 5.000000000000000000, 8.660254037844385522, -153.2500000000000000 ) ) ;
#37219=CARTESIAN_POINT ( 'NONE',  ( 9.999999999999998224, 0.000000000000000000, -200.0000000000000000 ) ) ;
#37221=CARTESIAN_POINT ( 'NONE',  ( -5.405949406249996869, 9.363379034771805109, -49.03125000204838813 ) ) ;
#37225=CARTESIAN_POINT ( 'NONE',  ( -10.81189881249999729, 6.242252689847871849, -180.9062500020484094 ) ) ;
#37227=DIRECTION ( 'NONE',  ( -0.000000000000000000, -0.000000000000000000, 1.000000000000000000 ) ) ;
#37228=CYLINDRICAL_SURFACE ( 'NONE', #2756, 9.999999999999998224 ) ;
#37229=CARTESIAN_POINT ( 'NONE',  ( -5.000000000000003553, -8.660254037844383745, -89.49999999999998579 ) ) ;
#37230=CARTESIAN_POINT ( 'NONE',  ( -2.121150477449813534E-15, -11.54700538379251284, -60.87499999999998579 ) ) ;
#37232=CARTESIAN_POINT ( 'NONE',  ( -9.999999999998456346, -5.773502691897145489, -20.62499999999993250 ) ) ;
#37233=CARTESIAN_POINT ( 'NONE',  ( -5.405949406249996869, 9.363379034771805109, -83.53125000204838102 ) ) ;
#37234=ORIENTED_EDGE ( 'NONE', *, *, #42108, .T. ) ;
#37235=CYLINDRICAL_SURFACE ( 'NONE', #23482, 9.999999999999998224 ) ;
#37237=ORIENTED_EDGE ( 'NONE', *, *, #19158, .F. ) ;
#37239=CARTESIAN_POINT ( 'NONE',  ( -5.405949406250003975, -9.363379034771801557, -39.34375000204837391 ) ) ;
#37240=CARTESIAN_POINT ( 'NONE',  ( -10.81189881249999729, 1.324075727343319199E-15, -29.09375000204836326 ) ) ;
#37241=CARTESIAN_POINT ( 'NONE',  ( -10.81189881249999907, -6.242252689847864744, -15.65625000204837569 ) ) ;
#37242=( BOUNDED_CURVE ( )  B_SPLINE_CURVE ( 2, ( #6610, #30138, #576, #32947, #19550, #23446, #32734 ),
 .UNSPECIFIED., .F., .F. ) 
 B_SPLINE_CURVE_WITH_KNOTS ( ( 3, 2, 2, 3 ),
 ( 0.5671641791044778058, 0.5684079601990051911, 0.5696517412935325764, 0.5708955223880599616 ),
 .UNSPECIFIED. ) 
 CURVE ( )  GEOMETRIC_REPRESENTATION_ITEM ( )  RATIONAL_B_SPLINE_CURVE ( ( 0.9999999999999761302, 0.8660254037844625774, 1.000000000000000000, 0.8660254037844387076, 1.000000000000000000, 0.8660254037844148378, 1.000000000000023981 ) ) 
 REPRESENTATION_ITEM ( '' )  );
#37243=CARTESIAN_POINT ( 'NONE',  ( 10.81189881249999907, 6.242252689847868297, -62.71875000204838813 ) ) ;
#37244=CARTESIAN_POINT ( 'NONE',  ( -2.121150477449813534E-15, -11.54700538379251284, -131.3750000000000000 ) ) ;
#37246=CARTESIAN_POINT ( 'NONE',  ( 10.81189881249999729, 0.000000000000000000, -184.3437500020483810 ) ) ;
#37249=LINE ( 'NONE', #37471, #8814 ) ;
#37252=CARTESIAN_POINT ( 'NONE',  ( 5.405949406249992428, -9.363379034771808662, -112.5937500020483810 ) ) ;
#37253=CARTESIAN_POINT ( 'NONE',  ( -10.00000000000102496, 5.773502691895664007, -14.87499999999994671 ) ) ;
#37254=CARTESIAN_POINT ( 'NONE',  ( 7.644554776091147741E-16, 12.48450537969573659, -88.15625000204838102 ) ) ;
#37255=EDGE_CURVE ( 'NONE', #4745, #982, #8501, .T. ) ;
#37256=CARTESIAN_POINT ( 'NONE',  ( 10.81189881249999729, 0.000000000000000000, -101.8437500020483810 ) ) ;
#37259=EDGE_CURVE ( 'NONE', #18128, #2019, #4453, .T. ) ;
#37261=CARTESIAN_POINT ( 'NONE',  ( -9.999999999999998224, 1.224646799147353059E-15, -154.6250000040967905 ) ) ;
#37263=EDGE_CURVE ( 'NONE', #684, #1542, #16154, .T. ) ;
#37267=CARTESIAN_POINT ( 'NONE',  ( 9.999999999999742428, 5.773502691896404748, -153.7500000040967620 ) ) ;
#37268=CARTESIAN_POINT ( 'NONE',  ( -9.999999999999998224, 1.224646799147353059E-15, -182.7500000000000000 ) ) ;
#37271=CARTESIAN_POINT ( 'NONE',  ( -10.00000000000000000, -5.773502691896251982, -70.12500000000000000 ) ) ;
#37273=CARTESIAN_POINT ( 'NONE',  ( 10.00000000000000000, 5.773502691896255534, -80.25000000409679046 ) ) ;
#37274=CARTESIAN_POINT ( 'NONE',  ( 9.999999999999998224, 0.000000000000000000, -95.37500000409677625 ) ) ;
#37277=CARTESIAN_POINT ( 'NONE',  ( -10.81189881249999729, 1.324075727343319199E-15, -83.28125000204838102 ) ) ;
#37279=CARTESIAN_POINT ( 'NONE',  ( -10.00000000000012434, 5.773502691896184480, -167.8749999999999716 ) ) ;
#37281=ORIENTED_EDGE ( 'NONE', *, *, #34824, .T. ) ;
#37282=CARTESIAN_POINT ( 'NONE',  ( -2.121150477449813534E-15, -11.54700538379251284, -5.374999999999960920 ) ) ;
#37284=CARTESIAN_POINT ( 'NONE',  ( -2.293366432827344421E-15, -12.48450537969573659, -12.21875000204837391 ) ) ;
#37285=CARTESIAN_POINT ( 'NONE',  ( -4.999999999999996447, 8.660254037844387298, -142.5000000000000000 ) ) ;
#37286=EDGE_CURVE ( 'NONE', #14564, #16918, #21061, .T. ) ;
#37288=CARTESIAN_POINT ( 'NONE',  ( -2.293366432827344421E-15, -12.48450537969573659, -132.4062500020483810 ) ) ;
#37290=CARTESIAN_POINT ( 'NONE',  ( -10.00000000000000000, -5.773502691896251982, -182.6250000000000284 ) ) ;
#37291=CARTESIAN_POINT ( 'NONE',  ( -9.999999999999998224, 1.224646799147353059E-15, -184.6250000040967905 ) ) ;
#37292=CARTESIAN_POINT ( 'NONE',  ( 10.81189881249999907, 6.242252689847868297, -109.4062500020483952 ) ) ;
#37293=ORIENTED_EDGE ( 'NONE', *, *, #9486, .T. ) ;
#37294=CARTESIAN_POINT ( 'NONE',  ( -10.00000000000012434, 5.773502691896184480, -194.8750000000000000 ) ) ;
#37295=EDGE_CURVE ( 'NONE', #18719, #32801, #6140, .T. ) ;
#37298=VECTOR ( 'NONE', #13383, 1000.000000000000000 ) ;
#37299=CARTESIAN_POINT ( 'NONE',  ( -5.405949406250003975, -9.363379034771801557, -36.53125000204837391 ) ) ;
#37302=CARTESIAN_POINT ( 'NONE',  ( -10.81189881249999729, 6.242252689847871849, -90.71875000204838102 ) ) ;
#37303=LINE ( 'NONE', #24160, #35314 ) ;
#37304=ADVANCED_FACE ( 'NONE', ( #42645 ), #13703, .T. ) ;
#37305=CARTESIAN_POINT ( 'NONE',  ( -9.999999999999998224, 1.224646799147353059E-15, -200.0000000000000000 ) ) ;
#37308=VECTOR ( 'NONE', #2960, 1000.000000000000114 ) ;
#37309=CARTESIAN_POINT ( 'NONE',  ( 7.070501591499376803E-16, 11.54700538379251284, -58.62499999999999289 ) ) ;
#37310=CARTESIAN_POINT ( 'NONE',  ( 7.644554776091147741E-16, 12.48450537969573659, -122.4687500020483952 ) ) ;
#37311=( BOUNDED_CURVE ( )  B_SPLINE_CURVE ( 2, ( #25033, #27829, #5589, #15284, #31934, #5378, #18529 ),
 .UNSPECIFIED., .F., .F. ) 
 B_SPLINE_CURVE_WITH_KNOTS ( ( 3, 2, 2, 3 ),
 ( 0.6492537313432837909, 0.6504975124378111762, 0.6517412935323385614, 0.6529850746268659467 ),
 .UNSPECIFIED. ) 
 CURVE ( )  GEOMETRIC_REPRESENTATION_ITEM ( )  RATIONAL_B_SPLINE_CURVE ( ( 0.9999999999999761302, 0.8660254037844625774, 1.000000000000000000, 0.8660254037844387076, 1.000000000000000000, 0.8660254037844148378, 1.000000000000023981 ) ) 
 REPRESENTATION_ITEM ( '' )  );
#37313=CARTESIAN_POINT ( 'NONE',  ( -5.405949406249996869, 9.363379034771805109, -4.031250002048375691 ) ) ;
#37314=DIRECTION ( 'NONE',  ( 1.000000000000000000, 0.000000000000000000, 0.000000000000000000 ) ) ;
#37316=CARTESIAN_POINT ( 'NONE',  ( -9.999999999999998224, 5.773502691896259087, -174.2500000040967905 ) ) ;
#37318=CARTESIAN_POINT ( 'NONE',  ( -10.81189881249999729, -6.242252689847864744, -177.6562500020484094 ) ) ;
#37319=CYLINDRICAL_SURFACE ( 'NONE', #32379, 9.999999999999998224 ) ;
#37322=CARTESIAN_POINT ( 'NONE',  ( -5.405949406249996869, 9.363379034771805109, -50.34375000204835260 ) ) ;
#37323=CARTESIAN_POINT ( 'NONE',  ( -5.405949406250003975, -9.363379034771801557, -42.34375000204837391 ) ) ;
#37325=CARTESIAN_POINT ( 'NONE',  ( -10.81189881249999729, 6.242252689847871849, -14.40625000204836859 ) ) ;
#37327=CARTESIAN_POINT ( 'NONE',  ( -4.999999999999996447, 8.660254037844387298, -145.5000000000000000 ) ) ;
#37329=CARTESIAN_POINT ( 'NONE',  ( 4.999999999999992006, -8.660254037844389075, -99.74999999999998579 ) ) ;
#37331=CARTESIAN_POINT ( 'NONE',  ( -4.999999999999996447, 8.660254037844387298, -115.8750000040967905 ) ) ;
#37335=CARTESIAN_POINT ( 'NONE',  ( 7.644554776091147741E-16, 12.48450537969573659, -109.1562500020483810 ) ) ;
#37337=AXIS2_PLACEMENT_3D ( 'NONE', #16089, #17797, #40042 ) ;
#37340=CARTESIAN_POINT ( 'NONE',  ( 9.999999999999479527, 5.773502691896553074, -141.7500000040967620 ) ) ;
#37341=CARTESIAN_POINT ( 'NONE',  ( -2.293366432827344421E-15, -12.48450537969573659, -166.9062500020483810 ) ) ;
#37343=ORIENTED_EDGE ( 'NONE', *, *, #5638, .F. ) ;
#37344=CARTESIAN_POINT ( 'NONE',  ( -9.999999999999998224, 5.773502691896259087, -26.87499999999998579 ) ) ;
#37346=CARTESIAN_POINT ( 'NONE',  ( -10.81189881249999729, 1.324075727343319199E-15, -35.28125000204837391 ) ) ;
#37347=CARTESIAN_POINT ( 'NONE',  ( -5.000000000000003553, -8.660254037844383745, -163.0000000000000000 ) ) ;
#37351=CARTESIAN_POINT ( 'NONE',  ( -10.81189881249999729, 6.242252689847871849, -131.4062500020484094 ) ) ;
#37352=CARTESIAN_POINT ( 'NONE',  ( 9.999999999999998224, 0.000000000000000000, -46.99999999999998579 ) ) ;
#37355=ORIENTED_EDGE ( 'NONE', *, *, #27774, .T. ) ;
#37356=ORIENTED_EDGE ( 'NONE', *, *, #23075, .T. ) ;
#37357=CARTESIAN_POINT ( 'NONE',  ( 9.999999999999998224, 0.000000000000000000, -182.3750000040967905 ) ) ;
#37358=AXIS2_PLACEMENT_3D ( 'NONE', #35362, #38579, #6216 ) ;
#37359=CARTESIAN_POINT ( 'NONE',  ( 0.000000000000000000, 0.000000000000000000, -200.0000000000000000 ) ) ;
#37360=( BOUNDED_CURVE ( )  B_SPLINE_CURVE ( 2, ( #7868, #37200, #20799, #33987, #4408, #17547, #27502 ),
 .UNSPECIFIED., .F., .F. ) 
 B_SPLINE_CURVE_WITH_KNOTS ( ( 3, 2, 2, 3 ),
 ( 0.5522388059701495155, 0.5534825870646767898, 0.5547263681592041751, 0.5559701492537315604 ),
 .UNSPECIFIED. ) 
 CURVE ( )  GEOMETRIC_REPRESENTATION_ITEM ( )  RATIONAL_B_SPLINE_CURVE ( ( 0.9999999999999761302, 0.8660254037844625774, 1.000000000000000000, 0.8660254037844387076, 1.000000000000000000, 0.8660254037844148378, 1.000000000000023981 ) ) 
 REPRESENTATION_ITEM ( '' )  );
#37361=CARTESIAN_POINT ( 'NONE',  ( 7.644554776091147741E-16, 12.48450537969573659, -167.4687500020483810 ) ) ;
#37363=CARTESIAN_POINT ( 'NONE',  ( -5.405949406249996869, 9.363379034771805109, -17.34375000204835260 ) ) ;
#37365=CARTESIAN_POINT ( 'NONE',  ( -10.81189881249999729, -6.242252689847864744, -147.4687500020484094 ) ) ;
#37366=CARTESIAN_POINT ( 'NONE',  ( -10.81189881249999729, 6.242252689847871849, -138.7187500020483810 ) ) ;
#37367=CARTESIAN_POINT ( 'NONE',  ( -10.81189881249999729, 6.242252689847871849, -105.9062500020483810 ) ) ;
#37371=CARTESIAN_POINT ( 'NONE',  ( 10.81189881249999907, 6.242252689847868297, -11.71875000204837214 ) ) ;
#37373=CARTESIAN_POINT ( 'NONE',  ( -5.405949406250003975, -9.363379034771801557, -198.5312500020484094 ) ) ;
#37377=AXIS2_PLACEMENT_3D ( 'NONE', #36436, #36224, #10519 ) ;
#37378=CARTESIAN_POINT ( 'NONE',  ( 5.405949406249999534, 9.363379034771803333, -77.59375000204838102 ) ) ;
#37379=CARTESIAN_POINT ( 'NONE',  ( -5.405949406249996869, 9.363379034771805109, -66.84375000204836681 ) ) ;
#37381=CARTESIAN_POINT ( 'NONE',  ( -10.81189881249999907, -6.242252689847864744, -33.65625000204836681 ) ) ;
#37385=CARTESIAN_POINT ( 'NONE',  ( 10.00000000000000000, 5.773502691896255534, -124.8750000000000000 ) ) ;
#37386=CARTESIAN_POINT ( 'NONE',  ( -10.81189881249999729, 6.242252689847871849, -131.4062500020483810 ) ) ;
#37387=FACE_OUTER_BOUND ( 'NONE', #3388, .T. ) ;
#37389=CARTESIAN_POINT ( 'NONE',  ( 5.405949406249999534, 9.363379034771803333, -14.78125000204835793 ) ) ;
#37390=VERTEX_POINT ( 'NONE', #36817 ) ;
#37395=CARTESIAN_POINT ( 'NONE',  ( 4.999999999999992006, -8.660254037844389075, -32.62500000409676915 ) ) ;
#37396=CARTESIAN_POINT ( 'NONE',  ( 9.999999999999479527, 5.773502691896553074, -148.8749999999999432 ) ) ;
#37398=DIRECTION ( 'NONE',  ( 1.000000000000000000, 0.000000000000000000, 0.000000000000000000 ) ) ;
#37399=CARTESIAN_POINT ( 'NONE',  ( -5.405949406249996869, 9.363379034771805109, -155.5312500020484094 ) ) ;
#37400=CARTESIAN_POINT ( 'NONE',  ( -10.81189881249999729, 1.324075727343319199E-15, -129.5937500020483810 ) ) ;
#37401=CARTESIAN_POINT ( 'NONE',  ( 9.999999999999776179, 5.773502691896386985, -190.8750000000000000 ) ) ;
#37402=EDGE_LOOP ( 'NONE', ( #11733, #17745, #17012, #42540 ) ) ;
#37403=CARTESIAN_POINT ( 'NONE',  ( 9.999999999999998224, 0.000000000000000000, -31.99999999999997158 ) ) ;
#37404=ORIENTED_EDGE ( 'NONE', *, *, #27555, .F. ) ;
#37406=EDGE_LOOP ( 'NONE', ( #373, #737, #20293, #38686 ) ) ;
#37407=CARTESIAN_POINT ( 'NONE',  ( 10.81189881249999551, -6.242252689847874514, -110.9687500020483810 ) ) ;
#37408=VERTEX_POINT ( 'NONE', #6621 ) ;
#37409=CARTESIAN_POINT ( 'NONE',  ( 4.999999999999992006, -8.660254037844389075, -41.62500000409677625 ) ) ;
#37410=CARTESIAN_POINT ( 'NONE',  ( 5.405949406249999534, 9.363379034771803333, -191.5937500020484094 ) ) ;
#37411=CARTESIAN_POINT ( 'NONE',  ( -5.405949406250003975, -9.363379034771801557, -40.84375000204837391 ) ) ;
#37413=FACE_OUTER_BOUND ( 'NONE', #40785, .T. ) ;
#37414=CARTESIAN_POINT ( 'NONE',  ( 10.81189881249999551, -6.242252689847874514, -169.4687500020483810 ) ) ;
#37415=CARTESIAN_POINT ( 'NONE',  ( -10.81189881249999907, -6.242252689847864744, -162.4687500020483526 ) ) ;
#37416=CARTESIAN_POINT ( 'NONE',  ( -9.999999999999998224, 1.224646799147353059E-15, -25.62500000409675849 ) ) ;
#37420=CARTESIAN_POINT ( 'NONE',  ( 9.999999999998969713, 5.773502691896851502, -87.37499999999997158 ) ) ;
#37422=CARTESIAN_POINT ( 'NONE',  ( -10.81189881249999729, 6.242252689847871849, -86.21875000204838102 ) ) ;
#37423=CARTESIAN_POINT ( 'NONE',  ( 9.999999999999998224, 0.000000000000000000, -36.49999999999997868 ) ) ;
#37424=CARTESIAN_POINT ( 'NONE',  ( -5.405949406249996869, 9.363379034771805109, -59.53125000204836681 ) ) ;
#37425=CARTESIAN_POINT ( 'NONE',  ( 9.999999999999998224, 0.000000000000000000, -13.99999999999995737 ) ) ;
#37427=CARTESIAN_POINT ( 'NONE',  ( 10.81189881249999729, 0.000000000000000000, -114.0312500020483952 ) ) ;
#37428=CARTESIAN_POINT ( 'NONE',  ( -2.293366432827344421E-15, -12.48450537969573659, -154.9062500020483810 ) ) ;
#37431=CARTESIAN_POINT ( 'NONE',  ( 5.000000000000000000, 8.660254037844385522, -128.1250000040967620 ) ) ;
#37433=EDGE_CURVE ( 'NONE', #14344, #20834, #35492, .T. ) ;
#37434=ORIENTED_EDGE ( 'NONE', *, *, #25926, .F. ) ;
#37437=CARTESIAN_POINT ( 'NONE',  ( -5.405949406250003975, -9.363379034771801557, -179.0312500020483810 ) ) ;
#37439=CARTESIAN_POINT ( 'NONE',  ( 4.999999999999992006, -8.660254037844389075, -48.74999999999998579 ) ) ;
#37441=CARTESIAN_POINT ( 'NONE',  ( 4.999999999999992006, -8.660254037844389075, -58.12500000409676204 ) ) ;
#37443=CARTESIAN_POINT ( 'NONE',  ( 9.999999999999998224, 0.000000000000000000, -170.3750000040968189 ) ) ;
#37445=CARTESIAN_POINT ( 'NONE',  ( 10.81189881249999729, 6.242252689847867408, -47.90625000204836681 ) ) ;
#37448=CARTESIAN_POINT ( 'NONE',  ( -5.000000000000003553, -8.660254037844383745, -134.8750000040967905 ) ) ;
#37449=CARTESIAN_POINT ( 'NONE',  ( -2.293366432827344421E-15, -12.48450537969573659, -178.9062500020484379 ) ) ;
#37452=CARTESIAN_POINT ( 'NONE',  ( -9.999999999999998224, 1.224646799147353059E-15, -82.24999999999998579 ) ) ;
#37453=CARTESIAN_POINT ( 'NONE',  ( 7.070501591499376803E-16, 11.54700538379251284, -154.6250000000000284 ) ) ;
#37455=CYLINDRICAL_SURFACE ( 'NONE', #6233, 9.999999999999998224 ) ;
#37456=CARTESIAN_POINT ( 'NONE',  ( -10.81189881249999907, -6.242252689847864744, -86.15625000204836681 ) ) ;
#37458=EDGE_CURVE ( 'NONE', #6661, #10829, #38251, .T. ) ;
#37460=ORIENTED_EDGE ( 'NONE', *, *, #18388, .F. ) ;
#37462=CARTESIAN_POINT ( 'NONE',  ( -10.81189881249999729, -6.242252689847864744, -37.96875000204837391 ) ) ;
#37463=CARTESIAN_POINT ( 'NONE',  ( -10.81189881249999729, 1.324075727343319199E-15, -23.09375000204835615 ) ) ;
#37464=CARTESIAN_POINT ( 'NONE',  ( -5.405949406249996869, 9.363379034771805109, -14.53125000204835615 ) ) ;
#37465=CARTESIAN_POINT ( 'NONE',  ( 5.405949406249992428, -9.363379034771808662, -60.09375000204835970 ) ) ;
#37466=CARTESIAN_POINT ( 'NONE',  ( -9.999999999999998224, 1.224646799147353059E-15, -163.6250000040967905 ) ) ;
#37468=CARTESIAN_POINT ( 'NONE',  ( -10.81189881249999729, 1.324075727343319199E-15, -188.0937500020483810 ) ) ;
#37471=CARTESIAN_POINT ( 'NONE',  ( -9.999999999999998224, 1.224646799147353059E-15, -200.0000000000000000 ) ) ;
#37472=CARTESIAN_POINT ( 'NONE',  ( 0.000000000000000000, 0.000000000000000000, -200.0000000000000000 ) ) ;
#37473=CARTESIAN_POINT ( 'NONE',  ( -9.999999999998969713, -5.773502691896847949, -21.00000000409676204 ) ) ;
#37474=DIRECTION ( 'NONE',  ( -0.000000000000000000, -0.000000000000000000, 1.000000000000000000 ) ) ;
#37475=CARTESIAN_POINT ( 'NONE',  ( 7.644554776091147741E-16, 12.48450537969573659, -114.9687500020483668 ) ) ;
#37476=CYLINDRICAL_SURFACE ( 'NONE', #19716, 9.999999999999998224 ) ;
#37477=CARTESIAN_POINT ( 'NONE',  ( -5.405949406249996869, 9.363379034771805109, -85.03125000204838102 ) ) ;
#37478=CARTESIAN_POINT ( 'NONE',  ( 10.81189881249999729, 6.242252689847867408, -101.7187500020483810 ) ) ;
#37481=CARTESIAN_POINT ( 'NONE',  ( -5.000000000000003553, -8.660254037844383745, -151.3750000040967905 ) ) ;
#37483=( BOUNDED_CURVE ( )  B_SPLINE_CURVE ( 2, ( #13496, #33596, #6417, #29502, #19557, #16306, #10060 ),
 .UNSPECIFIED., .F., .F. ) 
 B_SPLINE_CURVE_WITH_KNOTS ( ( 3, 2, 2, 3 ),
 ( 0.08582089552238814090, 0.08706467661691551230, 0.08830845771144288370, 0.08955223880597024122 ),
 .UNSPECIFIED. ) 
 CURVE ( )  GEOMETRIC_REPRESENTATION_ITEM ( )  RATIONAL_B_SPLINE_CURVE ( ( 0.9999999999999910072, 0.8660254037844477004, 1.000000000000000000, 0.8660254037844387076, 1.000000000000000000, 0.8660254037844282715, 1.000000000000010436 ) ) 
 REPRESENTATION_ITEM ( '' )  );
#37488=FACE_OUTER_BOUND ( 'NONE', #8598, .T. ) ;
#37489=CARTESIAN_POINT ( 'NONE',  ( -2.121150477449813534E-15, -11.54700538379251284, -69.87500000000000000 ) ) ;
#37491=CARTESIAN_POINT ( 'NONE',  ( 9.999999999999996447, -5.773502691896262640, -83.50000000409676204 ) ) ;
#37494=CARTESIAN_POINT ( 'NONE',  ( 10.81189881249999729, 0.000000000000000000, -75.03125000204838102 ) ) ;
#37499=VERTEX_POINT ( 'NONE', #18019 ) ;
#37500=CARTESIAN_POINT ( 'NONE',  ( 10.00000000000000000, 5.773502691896255534, -0.3749999999999697464 ) ) ;
#37502=CARTESIAN_POINT ( 'NONE',  ( 5.405949406249999534, 9.363379034771803333, -13.09375000204834905 ) ) ;
#37503=CARTESIAN_POINT ( 'NONE',  ( -9.999999999999998224, 1.224646799147353059E-15, -94.62500000409677625 ) ) ;
#37505=CARTESIAN_POINT ( 'NONE',  ( 7.644554776091147741E-16, 12.48450537969573659, -127.1562500020483952 ) ) ;
#37506=( BOUNDED_CURVE ( )  B_SPLINE_CURVE ( 2, ( #21813, #36039, #22661, #39055, #225, #13347, #26537 ),
 .UNSPECIFIED., .F., .F. ) 
 B_SPLINE_CURVE_WITH_KNOTS ( ( 3, 2, 2, 3 ),
 ( 0.4141791044776120256, 0.4154228855721394109, 0.4166666666666667962, 0.4179104477611941260 ),
 .UNSPECIFIED. ) 
 CURVE ( )  GEOMETRIC_REPRESENTATION_ITEM ( )  RATIONAL_B_SPLINE_CURVE ( ( 0.9999999999999880096, 0.8660254037844506980, 1.000000000000000000, 0.8660254037844387076, 1.000000000000000000, 0.8660254037844267172, 1.000000000000011990 ) ) 
 REPRESENTATION_ITEM ( '' )  );
#37507=CARTESIAN_POINT ( 'NONE',  ( -9.999999999999998224, 5.773502691896259087, -184.3750000000000000 ) ) ;
#37509=CARTESIAN_POINT ( 'NONE',  ( -10.81189881249999907, -6.242252689847864744, -108.6562500020483952 ) ) ;
#37512=EDGE_CURVE ( 'NONE', #19666, #2132, #37032, .T. ) ;
#37513=ORIENTED_EDGE ( 'NONE', *, *, #12588, .T. ) ;
#37515=ORIENTED_EDGE ( 'NONE', *, *, #9473, .F. ) ;
#37516=CARTESIAN_POINT ( 'NONE',  ( -10.81189881249999729, 1.324075727343319199E-15, -38.28125000204838102 ) ) ;
#37518=CARTESIAN_POINT ( 'NONE',  ( -5.405949406250003975, -9.363379034771801557, -85.84375000204836681 ) ) ;
#37519=DIRECTION ( 'NONE',  ( 1.000000000000000000, 0.000000000000000000, 0.000000000000000000 ) ) ;
#37523=CARTESIAN_POINT ( 'NONE',  ( 9.999999999999998224, 0.000000000000000000, -200.0000000000000000 ) ) ;
#37524=EDGE_CURVE ( 'NONE', #41727, #5730, #33592, .T. ) ;
#37525=CARTESIAN_POINT ( 'NONE',  ( 10.81189881249999551, -6.242252689847874514, -125.9687500020483810 ) ) ;
#37527=CARTESIAN_POINT ( 'NONE',  ( 10.81189881249999551, -6.242252689847874514, -1.656250002048371917 ) ) ;
#37530=CARTESIAN_POINT ( 'NONE',  ( -5.000000000000003553, -8.660254037844383745, -175.3750000040967905 ) ) ;
#37532=CARTESIAN_POINT ( 'NONE',  ( -5.405949406249996869, 9.363379034771805109, -175.0312500020484094 ) ) ;
#37534=CARTESIAN_POINT ( 'NONE',  ( -9.999999999999998224, 1.224646799147353059E-15, -121.6250000040967905 ) ) ;
#37536=CARTESIAN_POINT ( 'NONE',  ( -10.81189881249999729, 1.324075727343319199E-15, -48.59375000204838102 ) ) ;
#37538=CARTESIAN_POINT ( 'NONE',  ( 10.81189881249999907, 6.242252689847868297, -8.906250002048375691 ) ) ;
#37540=CARTESIAN_POINT ( 'NONE',  ( -9.999999999999998224, 1.224646799147353059E-15, -193.6250000040967905 ) ) ;
#37542=CARTESIAN_POINT ( 'NONE',  ( 9.999999999999996447, -5.773502691896262640, -95.12499999999998579 ) ) ;
#37544=CARTESIAN_POINT ( 'NONE',  ( 10.00000000000000000, 5.773502691896255534, -107.2500000040967763 ) ) ;
#37545=EDGE_CURVE ( 'NONE', #8658, #40301, #26400, .T. ) ;
#37546=CARTESIAN_POINT ( 'NONE',  ( 0.000000000000000000, 0.000000000000000000, -200.0000000000000000 ) ) ;
#37549=CARTESIAN_POINT ( 'NONE',  ( 10.81189881249999551, -6.242252689847874514, -97.65625000204839523 ) ) ;
#37552=CARTESIAN_POINT ( 'NONE',  ( -10.00000000000051337, 5.773502691895962435, -91.37499999999997158 ) ) ;
#37553=CARTESIAN_POINT ( 'NONE',  ( -10.81189881249999729, 6.242252689847871849, -161.4062500020483810 ) ) ;
#37555=ORIENTED_EDGE ( 'NONE', *, *, #32223, .F. ) ;
#37556=CARTESIAN_POINT ( 'NONE',  ( 9.999999999999998224, 0.000000000000000000, -25.99999999999996803 ) ) ;
#37557=CARTESIAN_POINT ( 'NONE',  ( 5.405949406249992428, -9.363379034771808662, -37.78125000204838102 ) ) ;
#37558=CARTESIAN_POINT ( 'NONE',  ( -5.000000000000003553, -8.660254037844383745, -158.5000000000000000 ) ) ;
#37559=CARTESIAN_POINT ( 'NONE',  ( 10.00000000000051159, -5.773502691895965988, -92.12499999999997158 ) ) ;
#37561=LINE ( 'NONE', #31533, #7745 ) ;
#37562=CARTESIAN_POINT ( 'NONE',  ( 5.405949406249999534, 9.363379034771803333, -136.2812500020483810 ) ) ;
#37563=DIRECTION ( 'NONE',  ( -0.000000000000000000, -0.000000000000000000, 1.000000000000000000 ) ) ;
#37564=EDGE_CURVE ( 'NONE', #18570, #6727, #23883, .T. ) ;
#37566=EDGE_CURVE ( 'NONE', #6715, #7196, #34452, .T. ) ;
#37568=ORIENTED_EDGE ( 'NONE', *, *, #39352, .F. ) ;
#37569=ORIENTED_EDGE ( 'NONE', *, *, #18388, .T. ) ;
#37571=CARTESIAN_POINT ( 'NONE',  ( 9.999999999999998224, 0.000000000000000000, -200.0000000000000000 ) ) ;
#37573=CARTESIAN_POINT ( 'NONE',  ( -5.405949406250003975, -9.363379034771801557, -165.3437500020484094 ) ) ;
#37575=CARTESIAN_POINT ( 'NONE',  ( 10.81189881249999551, -6.242252689847874514, -11.96875000204837214 ) ) ;
#37576=DIRECTION ( 'NONE',  ( -0.4999999999999998890, -0.8660254037844387076, 0.000000000000000000 ) ) ;
#37577=CARTESIAN_POINT ( 'NONE',  ( 7.644554776091147741E-16, 12.48450537969573659, -144.9687500020484094 ) ) ;
#37578=CARTESIAN_POINT ( 'NONE',  ( 10.81189881249999907, 6.242252689847868297, -137.7187500020484094 ) ) ;
#37579=CARTESIAN_POINT ( 'NONE',  ( -5.405949406250003975, -9.363379034771801557, -108.5312500020483810 ) ) ;
#37583=CARTESIAN_POINT ( 'NONE',  ( 5.405949406249992428, -9.363379034771808662, -6.093750002048370362 ) ) ;
#37586=CARTESIAN_POINT ( 'NONE',  ( -9.999999999999998224, 1.224646799147353059E-15, -55.24999999999996447 ) ) ;
#37590=CARTESIAN_POINT ( 'NONE',  ( 10.81189881249999551, -6.242252689847874514, -73.46875000204836681 ) ) ;
#37591=CARTESIAN_POINT ( 'NONE',  ( 5.405949406249999534, 9.363379034771803333, -64.09375000204836681 ) ) ;
#37592=CARTESIAN_POINT ( 'NONE',  ( -5.000000000000003553, -8.660254037844383745, -19.37500000409675494 ) ) ;
#37593=CARTESIAN_POINT ( 'NONE',  ( -10.81189881249999907, -6.242252689847864744, -30.65625000204835260 ) ) ;
#37597=CARTESIAN_POINT ( 'NONE',  ( 9.999999999999996447, -5.773502691896262640, -117.6250000000000000 ) ) ;
#37598=CARTESIAN_POINT ( 'NONE',  ( -10.81189881249999729, 1.324075727343319199E-15, -132.7812500020483810 ) ) ;
#37602=CARTESIAN_POINT ( 'NONE',  ( 10.81189881249999551, -6.242252689847874514, -16.65625000204838102 ) ) ;
#37607=CARTESIAN_POINT ( 'NONE',  ( 5.000000000000000000, 8.660254037844385522, -36.62500000409676915 ) ) ;
#37610=CARTESIAN_POINT ( 'NONE',  ( -10.00000000000025580, 5.773502691896109873, -100.7500000040968047 ) ) ;
#37611=CARTESIAN_POINT ( 'NONE',  ( 5.405949406249999534, 9.363379034771803333, -152.7812500020484094 ) ) ;
#37612=CARTESIAN_POINT ( 'NONE',  ( -5.405949406250003975, -9.363379034771801557, -130.8437500020484094 ) ) ;
#37613=CARTESIAN_POINT ( 'NONE',  ( -10.00000000000051337, 5.773502691895962435, -143.8750000000000000 ) ) ;
#37614=ORIENTED_EDGE ( 'NONE', *, *, #24444, .F. ) ;
#37617=( BOUNDED_CURVE ( )  B_SPLINE_CURVE ( 2, ( #26645, #23631, #13243, #26225, #36776, #13449, #6788 ),
 .UNSPECIFIED., .F., .F. ) 
 B_SPLINE_CURVE_WITH_KNOTS ( ( 3, 2, 2, 3 ),
 ( 0.3992537313432836799, 0.4004975124378110651, 0.4017412935323383949, 0.4029850746268657802 ),
 .UNSPECIFIED. ) 
 CURVE ( )  GEOMETRIC_REPRESENTATION_ITEM ( )  RATIONAL_B_SPLINE_CURVE ( ( 0.9999999999999880096, 0.8660254037844506980, 1.000000000000000000, 0.8660254037844387076, 1.000000000000000000, 0.8660254037844267172, 1.000000000000011990 ) ) 
 REPRESENTATION_ITEM ( '' )  );
#37621=CARTESIAN_POINT ( 'NONE',  ( 9.999999999999998224, 0.000000000000000000, -144.8750000040967905 ) ) ;
#37622=CARTESIAN_POINT ( 'NONE',  ( -10.81189881249999907, -6.242252689847864744, -189.4687500020484094 ) ) ;
#37623=VECTOR ( 'NONE', #26154, 1000.000000000000114 ) ;
#37624=CARTESIAN_POINT ( 'NONE',  ( 10.81189881249999729, 0.000000000000000000, -37.34375000204836681 ) ) ;
#37625=EDGE_CURVE ( 'NONE', #933, #5984, #14772, .T. ) ;
#37626=CARTESIAN_POINT ( 'NONE',  ( -2.544246206568858693, -10.01717225130982492, 6.879861566378983540E-16 ) ) ;
#37627=CARTESIAN_POINT ( 'NONE',  ( 9.999999999999998224, 0.000000000000000000, -73.99999999999998579 ) ) ;
#37628=CARTESIAN_POINT ( 'NONE',  ( 7.644554776091147741E-16, 12.48450537969573659, -170.4687500020483810 ) ) ;
#37630=CARTESIAN_POINT ( 'NONE',  ( 5.405949406249999534, 9.363379034771803333, -158.5937500020483810 ) ) ;
#37631=DIRECTION ( 'NONE',  ( -0.000000000000000000, -0.000000000000000000, 1.000000000000000000 ) ) ;
#37635=CARTESIAN_POINT ( 'NONE',  ( 5.000000000000000000, 8.660254037844385522, -134.1250000040967620 ) ) ;
#37636=CARTESIAN_POINT ( 'NONE',  ( 9.999999999998969713, 5.773502691896851502, -66.75000000409674783 ) ) ;
#37638=CARTESIAN_POINT ( 'NONE',  ( -5.405949406250003975, -9.363379034771801557, -88.84375000204838102 ) ) ;
#37639=CARTESIAN_POINT ( 'NONE',  ( -9.999999999999998224, 1.224646799147353059E-15, -113.7499999999999858 ) ) ;
#37640=CARTESIAN_POINT ( 'NONE',  ( -10.81189881249999907, -6.242252689847864744, -60.65625000204840234 ) ) ;
#37643=CARTESIAN_POINT ( 'NONE',  ( -10.81189881249999729, 6.242252689847871849, -113.4062500020483810 ) ) ;
#37644=CARTESIAN_POINT ( 'NONE',  ( -5.405949406249996869, 9.363379034771805109, -155.5312500020484094 ) ) ;
#37645=CARTESIAN_POINT ( 'NONE',  ( -5.000000000000003553, -8.660254037844383745, -11.49999999999995381 ) ) ;
#37647=CARTESIAN_POINT ( 'NONE',  ( -10.00000000000000000, -5.773502691896251982, -130.5000000040967905 ) ) ;
#37649=ORIENTED_EDGE ( 'NONE', *, *, #15271, .T. ) ;
#37653=CARTESIAN_POINT ( 'NONE',  ( -10.81189881249999907, -6.242252689847864744, -177.6562500020484094 ) ) ;
#37656=CARTESIAN_POINT ( 'NONE',  ( 7.070501591499377789E-16, 11.54700538379251284, -62.00000000409678336 ) ) ;
#37658=CARTESIAN_POINT ( 'NONE',  ( 10.00000000000000000, 5.773502691896255534, -135.7500000040967905 ) ) ;
#37661=CARTESIAN_POINT ( 'NONE',  ( -10.81189881249999729, 6.242252689847871849, -50.40625000204837391 ) ) ;
#37664=CARTESIAN_POINT ( 'NONE',  ( -10.00000000000012434, 5.773502691896184480, -157.7500000040967905 ) ) ;
#37665=CARTESIAN_POINT ( 'NONE',  ( 10.81189881249999729, 0.000000000000000000, -177.0312500020483810 ) ) ;
#37666=CARTESIAN_POINT ( 'NONE',  ( 10.00000000000051159, -5.773502691895965988, -73.00000000409676204 ) ) ;
#37667=CARTESIAN_POINT ( 'NONE',  ( 9.999999999999998224, 0.000000000000000000, -81.49999999999998579 ) ) ;
#37669=DIRECTION ( 'NONE',  ( -0.000000000000000000, -0.000000000000000000, 1.000000000000000000 ) ) ;
#37670=CARTESIAN_POINT ( 'NONE',  ( 9.999999999999227285, 5.773502691896701400, -105.7500000040967620 ) ) ;
#37672=CARTESIAN_POINT ( 'NONE',  ( 7.644554776091147741E-16, 12.48450537969573659, -86.65625000204838102 ) ) ;
#37673=VERTEX_POINT ( 'NONE', #14342 ) ;
#37675=VERTEX_POINT ( 'NONE', #37890 ) ;
#37676=ORIENTED_EDGE ( 'NONE', *, *, #5844, .F. ) ;
#37677=CARTESIAN_POINT ( 'NONE',  ( 10.81189881249999729, 6.242252689847867408, -38.71875000204835970 ) ) ;
#37678=CARTESIAN_POINT ( 'NONE',  ( -2.293366432827344421E-15, -12.48450537969573659, -24.21875000204836326 ) ) ;
#37679=CARTESIAN_POINT ( 'NONE',  ( -10.81189881249999907, -6.242252689847864744, -17.15625000204838102 ) ) ;
#37680=CARTESIAN_POINT ( 'NONE',  ( -5.405949406250003975, -9.363379034771801557, -64.84375000204836681 ) ) ;
#37682=CARTESIAN_POINT ( 'NONE',  ( 4.999999999999992006, -8.660254037844389075, -17.62500000409675138 ) ) ;
#37684=CARTESIAN_POINT ( 'NONE',  ( -5.405949406249996869, 9.363379034771805109, -188.3437500020483810 ) ) ;
#37687=CARTESIAN_POINT ( 'NONE',  ( -9.999999999999998224, 1.224646799147353059E-15, -193.2500000000000000 ) ) ;
#37690=CARTESIAN_POINT ( 'NONE',  ( 10.00000000000102318, -5.773502691895667560, -104.1249999999999432 ) ) ;
#37691=CARTESIAN_POINT ( 'NONE',  ( 9.999999999999998224, 0.000000000000000000, -200.0000000000000000 ) ) ;
#37692=CARTESIAN_POINT ( 'NONE',  ( 5.405949406249999534, 9.363379034771803333, -116.5937500020483810 ) ) ;
#37694=CARTESIAN_POINT ( 'NONE',  ( 10.81189881249999729, 0.000000000000000000, -82.53125000204838102 ) ) ;
#37695=CARTESIAN_POINT ( 'NONE',  ( -10.81189881249999729, -6.242252689847864744, -97.96875000204838102 ) ) ;
#37696=EDGE_CURVE ( 'NONE', #2592, #24037, #24096, .T. ) ;
#37699=CARTESIAN_POINT ( 'NONE',  ( -4.999999999999996447, 8.660254037844387298, -154.8750000040967905 ) ) ;
#37703=FACE_OUTER_BOUND ( 'NONE', #6832, .T. ) ;
#37706=CARTESIAN_POINT ( 'NONE',  ( -10.00000000000102496, 5.773502691895664007, -62.87499999999994316 ) ) ;
#37707=CARTESIAN_POINT ( 'NONE',  ( -10.00000000000000000, -5.773502691896251982, -76.12499999999997158 ) ) ;
#37709=CARTESIAN_POINT ( 'NONE',  ( 4.999999999999992006, -8.660254037844389075, -79.12500000409677625 ) ) ;
#37710=CARTESIAN_POINT ( 'NONE',  ( 11.54700538379253416, -19.99999999999999289, 49.99999999999998579 ) ) ;
#37712=CARTESIAN_POINT ( 'NONE',  ( 7.644554776091147741E-16, 12.48450537969573659, -77.65625000204838102 ) ) ;
#37714=CARTESIAN_POINT ( 'NONE',  ( -4.999999999999996447, 8.660254037844387298, -168.0000000000000000 ) ) ;
#37716=VERTEX_POINT ( 'NONE', #1217 ) ;
#37717=CARTESIAN_POINT ( 'NONE',  ( -10.00000000000000000, -5.773502691896251982, -1.124999999999973355 ) ) ;
#37719=CARTESIAN_POINT ( 'NONE',  ( -10.81189881249999729, -6.242252689847864744, -16.96875000204836681 ) ) ;
#37723=CARTESIAN_POINT ( 'NONE',  ( 10.81189881249999907, 6.242252689847868297, -127.4062500020483810 ) ) ;
#37724=CARTESIAN_POINT ( 'NONE',  ( -4.999999999999996447, 8.660254037844387298, -184.5000000000000000 ) ) ;
#37725=CARTESIAN_POINT ( 'NONE',  ( 0.000000000000000000, 0.000000000000000000, -200.0000000000000000 ) ) ;
#37726=CARTESIAN_POINT ( 'NONE',  ( 10.81189881249999729, 0.000000000000000000, -108.0312500020483810 ) ) ;
#37727=ORIENTED_EDGE ( 'NONE', *, *, #10791, .F. ) ;
#37728=CARTESIAN_POINT ( 'NONE',  ( -9.999999999999998224, 1.224646799147353059E-15, -138.1250000040967620 ) ) ;
#37731=CARTESIAN_POINT ( 'NONE',  ( 10.81189881249999551, -6.242252689847874514, -34.65625000204836681 ) ) ;
#37733=CARTESIAN_POINT ( 'NONE',  ( -5.405949406250003975, -9.363379034771801557, -90.34375000204838102 ) ) ;
#37736=( BOUNDED_CURVE ( )  B_SPLINE_CURVE ( 2, ( #5937, #19085, #28822, #32271, #8749, #5509, #35084 ),
 .UNSPECIFIED., .F., .F. ) 
 B_SPLINE_CURVE_WITH_KNOTS ( ( 3, 2, 2, 3 ),
 ( 0.3059701492537313383, 0.3072139303482587791, 0.3084577114427861644, 0.3097014925373136052 ),
 .UNSPECIFIED. ) 
 CURVE ( )  GEOMETRIC_REPRESENTATION_ITEM ( )  RATIONAL_B_SPLINE_CURVE ( ( 1.000000000000000000, 0.8660254037844387076, 1.000000000000000000, 0.8660254037844387076, 1.000000000000000000, 0.8660254037844207220, 1.000000000000017986 ) ) 
 REPRESENTATION_ITEM ( '' )  );
#37737=CARTESIAN_POINT ( 'NONE',  ( 7.070501591499376803E-16, 11.54700538379251284, -123.1249999999999858 ) ) ;
#37739=CARTESIAN_POINT ( 'NONE',  ( 9.999999999999994671, -5.773502691896262640, -138.6250000000000000 ) ) ;
#37740=CARTESIAN_POINT ( 'NONE',  ( -5.405949406250003975, -9.363379034771801557, -124.8437500020483810 ) ) ;
#37742=CARTESIAN_POINT ( 'NONE',  ( -9.999999999999998224, 1.224646799147353059E-15, -171.1250000040968189 ) ) ;
#37745=CARTESIAN_POINT ( 'NONE',  ( -10.00000000000000000, -5.773502691896251982, -175.5000000040967905 ) ) ;
#37746=CARTESIAN_POINT ( 'NONE',  ( 10.81189881249999551, -6.242252689847874514, -171.1562500020484094 ) ) ;
#37747=CARTESIAN_POINT ( 'NONE',  ( -5.000000000000003553, -8.660254037844383745, -1.375000004096765815 ) ) ;
#37750=CARTESIAN_POINT ( 'NONE',  ( -10.81189881249999729, -6.242252689847864744, -51.46875000204837391 ) ) ;
#37752=CARTESIAN_POINT ( 'NONE',  ( -10.81189881249999729, 1.324075727343319199E-15, -11.28125000204835438 ) ) ;
#37756=CARTESIAN_POINT ( 'NONE',  ( -4.999999999999996447, 8.660254037844387298, -100.4999999999999858 ) ) ;
#37758=CARTESIAN_POINT ( 'NONE',  ( -5.000000000000003553, -8.660254037844383745, -104.8750000040967763 ) ) ;
#37760=EDGE_CURVE ( 'NONE', #33065, #35463, #8114, .T. ) ;
#37763=CARTESIAN_POINT ( 'NONE',  ( 5.405949406249992428, -9.363379034771808662, -96.28125000204838102 ) ) ;
#37766=CARTESIAN_POINT ( 'NONE',  ( 4.999999999999992006, -8.660254037844389075, -166.1250000040967905 ) ) ;
#37767=CARTESIAN_POINT ( 'NONE',  ( -5.405949406250003975, -9.363379034771801557, -167.0312500020484094 ) ) ;
#37769=ORIENTED_EDGE ( 'NONE', *, *, #37524, .T. ) ;
#37770=CARTESIAN_POINT ( 'NONE',  ( -10.00000000000000000, -5.773502691896251982, -22.12499999999997868 ) ) ;
#37771=AXIS2_PLACEMENT_3D ( 'NONE', #3719, #20738, #36930 ) ;
#37772=CARTESIAN_POINT ( 'NONE',  ( -5.405949406250003975, -9.363379034771801557, -29.03125000204837036 ) ) ;
#37773=CARTESIAN_POINT ( 'NONE',  ( -5.000000000000003553, -8.660254037844383745, -161.5000000000000000 ) ) ;
#37774=CARTESIAN_POINT ( 'NONE',  ( 4.999999999999992006, -8.660254037844389075, -92.24999999999998579 ) ) ;
#37776=CARTESIAN_POINT ( 'NONE',  ( 0.000000000000000000, 0.000000000000000000, -200.0000000000000000 ) ) ;
#37777=CARTESIAN_POINT ( 'NONE',  ( -5.405949406249996869, 9.363379034771805109, -131.5312500020484094 ) ) ;
#37778=CARTESIAN_POINT ( 'NONE',  ( 1.915001621468759074, 10.12637373387462780, 1.028787474604546119E-14 ) ) ;
#37779=CARTESIAN_POINT ( 'NONE',  ( -2.121150477449813534E-15, -11.54700538379251284, -188.3750000000000284 ) ) ;
#37780=ORIENTED_EDGE ( 'NONE', *, *, #15145, .T. ) ;
#37781=CARTESIAN_POINT ( 'NONE',  ( 10.81189881249999551, -6.242252689847874514, -61.65625000204838813 ) ) ;
#37783=ORIENTED_EDGE ( 'NONE', *, *, #10764, .T. ) ;
#37784=EDGE_LOOP ( 'NONE', ( #28406, #37569, #13121, #26526 ) ) ;
#37786=CARTESIAN_POINT ( 'NONE',  ( 9.999999999999998224, 0.000000000000000000, -54.87500000409675494 ) ) ;
#37787=CARTESIAN_POINT ( 'NONE',  ( 10.81189881249999551, -6.242252689847874514, -158.9687500020484094 ) ) ;
#37789=CARTESIAN_POINT ( 'NONE',  ( -10.81189881249999729, 1.324075727343319199E-15, -17.09375000204835260 ) ) ;
#37790=CYLINDRICAL_SURFACE ( 'NONE', #6732, 9.999999999999998224 ) ;
#37791=CARTESIAN_POINT ( 'NONE',  ( 10.81189881249999551, -6.242252689847874514, -148.4687500020484094 ) ) ;
#37792=CARTESIAN_POINT ( 'NONE',  ( 10.81189881249999729, 0.000000000000000000, -125.8437500020483952 ) ) ;
#37793=CARTESIAN_POINT ( 'NONE',  ( 10.81189881249999729, 0.000000000000000000, -103.5312500020483810 ) ) ;
#37795=DIRECTION ( 'NONE',  ( -0.000000000000000000, -0.000000000000000000, 1.000000000000000000 ) ) ;
#37797=CARTESIAN_POINT ( 'NONE',  ( 7.644554776091147741E-16, 12.48450537969573659, -2.468750002048359704 ) ) ;
#37799=CARTESIAN_POINT ( 'NONE',  ( 10.81189881249999729, 6.242252689847867408, -191.9062500020484094 ) ) ;
#37800=CARTESIAN_POINT ( 'NONE',  ( 9.999999999999998224, 0.000000000000000000, -12.49999999999995559 ) ) ;
#37803=CARTESIAN_POINT ( 'NONE',  ( -5.405949406250003975, -9.363379034771801557, -79.84375000204838102 ) ) ;
#37804=CARTESIAN_POINT ( 'NONE',  ( 5.405949406249992428, -9.363379034771808662, -54.09375000204835970 ) ) ;
#37805=CARTESIAN_POINT ( 'NONE',  ( -5.000000000000003553, -8.660254037844383745, -116.8750000040967905 ) ) ;
#37806=CARTESIAN_POINT ( 'NONE',  ( -10.81189881249999907, -6.242252689847864744, -35.15625000204837391 ) ) ;
#37808=CARTESIAN_POINT ( 'NONE',  ( 10.00000000000000000, 5.773502691896255534, -136.8750000000000000 ) ) ;
#37811=EDGE_CURVE ( 'NONE', #7087, #19666, #42169, .T. ) ;
#37812=CARTESIAN_POINT ( 'NONE',  ( -2.121150477449813534E-15, -11.54700538379251284, -125.3749999999999858 ) ) ;
#37813=EDGE_CURVE ( 'NONE', #22008, #23394, #1321, .T. ) ;
#37816=CARTESIAN_POINT ( 'NONE',  ( 5.405949406249992428, -9.363379034771808662, -9.281250002048352599 ) ) ;
#37817=EDGE_CURVE ( 'NONE', #5974, #38843, #27792, .T. ) ;
#37818=ORIENTED_EDGE ( 'NONE', *, *, #35439, .T. ) ;
#37821=CARTESIAN_POINT ( 'NONE',  ( -9.999999999999998224, 1.224646799147353059E-15, -200.0000000000000000 ) ) ;
#37823=CARTESIAN_POINT ( 'NONE',  ( 10.00000000000000000, 5.773502691896255534, -30.75000000409674428 ) ) ;
#37824=CARTESIAN_POINT ( 'NONE',  ( 5.000000000000000000, 8.660254037844385522, -61.74999999999997158 ) ) ;
#37827=CARTESIAN_POINT ( 'NONE',  ( 0.000000000000000000, 0.000000000000000000, -200.0000000000000000 ) ) ;
#37828=CARTESIAN_POINT ( 'NONE',  ( 10.81189881249999729, 0.000000000000000000, -142.5312500020483810 ) ) ;
#37829=CARTESIAN_POINT ( 'NONE',  ( 7.644554776091147741E-16, 12.48450537969573659, -123.9687500020483952 ) ) ;
#37830=CARTESIAN_POINT ( 'NONE',  ( -4.999999999999996447, 8.660254037844387298, -3.375000004096767370 ) ) ;
#37831=AXIS2_PLACEMENT_3D ( 'NONE', #15291, #21130, #18536 ) ;
#37832=( BOUNDED_CURVE ( )  B_SPLINE_CURVE ( 2, ( #6308, #23347, #36500, #266, #25950, #19454, #39098 ),
 .UNSPECIFIED., .F., .F. ) 
 B_SPLINE_CURVE_WITH_KNOTS ( ( 3, 2, 2, 3 ),
 ( 0.4440298507462688282, 0.4452736318407962135, 0.4465174129353234878, 0.4477611940298508730 ),
 .UNSPECIFIED. ) 
 CURVE ( )  GEOMETRIC_REPRESENTATION_ITEM ( )  RATIONAL_B_SPLINE_CURVE ( ( 0.9999999999999820144, 0.8660254037844566932, 1.000000000000000000, 0.8660254037844387076, 1.000000000000000000, 0.8660254037844267172, 1.000000000000011990 ) ) 
 REPRESENTATION_ITEM ( '' )  );
#37833=LINE ( 'NONE', #17103, #25236 ) ;
#37834=VERTEX_POINT ( 'NONE', #31860 ) ;
#37835=EDGE_CURVE ( 'NONE', #36368, #14677, #10373, .T. ) ;
#37837=ORIENTED_EDGE ( 'NONE', *, *, #31800, .T. ) ;
#37839=CARTESIAN_POINT ( 'NONE',  ( 5.405949406249992428, -9.363379034771808662, -193.5937500020484094 ) ) ;
#37840=CARTESIAN_POINT ( 'NONE',  ( -5.405949406249996869, 9.363379034771805109, -36.84375000204836681 ) ) ;
#37841=CARTESIAN_POINT ( 'NONE',  ( 9.999999999999998224, 0.000000000000000000, -200.0000000000000000 ) ) ;
#37842=CARTESIAN_POINT ( 'NONE',  ( 9.999999999999998224, 0.000000000000000000, -140.0000000000000000 ) ) ;
#37843=CARTESIAN_POINT ( 'NONE',  ( 5.405949406249999534, 9.363379034771803333, -172.0937500020484094 ) ) ;
#37844=CARTESIAN_POINT ( 'NONE',  ( -10.81189881249999907, -6.242252689847864744, -154.9687500020484094 ) ) ;
#37845=EDGE_CURVE ( 'NONE', #25379, #37675, #25032, .T. ) ;
#37850=CARTESIAN_POINT ( 'NONE',  ( -4.999999999999996447, 8.660254037844387298, -70.49999999999998579 ) ) ;
#37852=CARTESIAN_POINT ( 'NONE',  ( 10.81189881249999551, -6.242252689847874514, -86.96875000204838102 ) ) ;
#37853=CARTESIAN_POINT ( 'NONE',  ( 4.999999999999992006, -8.660254037844389075, -113.2499999999999858 ) ) ;
#37854=CARTESIAN_POINT ( 'NONE',  ( -5.405949406250003975, -9.363379034771801557, -54.53125000204836681 ) ) ;
#37857=CARTESIAN_POINT ( 'NONE',  ( -5.405949406249996869, 9.363379034771805109, -113.5312500020483952 ) ) ;
#37858=CARTESIAN_POINT ( 'NONE',  ( -10.81189881249999729, 6.242252689847871849, -156.9062500020483526 ) ) ;
#37861=CARTESIAN_POINT ( 'NONE',  ( -4.999999999999996447, 8.660254037844387298, -129.3750000040967905 ) ) ;
#37863=ORIENTED_EDGE ( 'NONE', *, *, #15782, .F. ) ;
#37866=VECTOR ( 'NONE', #8988, 1000.000000000000000 ) ;
#37867=CARTESIAN_POINT ( 'NONE',  ( 5.405949406249992428, -9.363379034771808662, -178.7812500020484094 ) ) ;
#37870=CARTESIAN_POINT ( 'NONE',  ( 5.000000000000000000, 8.660254037844385522, -60.62500000409676204 ) ) ;
#37872=FACE_OUTER_BOUND ( 'NONE', #16946, .T. ) ;
#37874=CARTESIAN_POINT ( 'NONE',  ( -10.81189881249999729, -6.242252689847864744, -53.15625000204838102 ) ) ;
#37875=( BOUNDED_CURVE ( )  B_SPLINE_CURVE ( 2, ( #16104, #15273, #25439, #25646, #5792, #15893, #32344 ),
 .UNSPECIFIED., .F., .F. ) 
 B_SPLINE_CURVE_WITH_KNOTS ( ( 3, 2, 2, 3 ),
 ( 0.3395522388059703522, 0.3407960199004976820, 0.3420398009950250118, 0.3432835820895522860 ),
 .UNSPECIFIED. ) 
 CURVE ( )  GEOMETRIC_REPRESENTATION_ITEM ( )  RATIONAL_B_SPLINE_CURVE ( ( 0.9999999999999761302, 0.8660254037844625774, 1.000000000000000000, 0.8660254037844387076, 1.000000000000000000, 0.8660254037844327124, 1.000000000000005995 ) ) 
 REPRESENTATION_ITEM ( '' )  );
#37877=AXIS2_PLACEMENT_3D ( 'NONE', #15908, #4840, #27722 ) ;
#37879=CARTESIAN_POINT ( 'NONE',  ( 9.999999999999998224, 0.000000000000000000, -88.99999999999998579 ) ) ;
#37880=CARTESIAN_POINT ( 'NONE',  ( -2.293366432827344421E-15, -12.48450537969573659, -175.9062500020483810 ) ) ;
#37881=EDGE_CURVE ( 'NONE', #7438, #38628, #40994, .T. ) ;
#37882=CARTESIAN_POINT ( 'NONE',  ( 5.000000000000000000, 8.660254037844385522, -198.2500000000000000 ) ) ;
#37883=ORIENTED_EDGE ( 'NONE', *, *, #39352, .T. ) ;
#37884=CARTESIAN_POINT ( 'NONE',  ( 5.000000000000000000, 8.660254037844385522, -84.62500000409677625 ) ) ;
#37886=CARTESIAN_POINT ( 'NONE',  ( -2.121150477449813534E-15, -11.54700538379251284, -20.37499999999996803 ) ) ;
#37887=CARTESIAN_POINT ( 'NONE',  ( -5.405949406250003975, -9.363379034771801557, -75.53125000204838102 ) ) ;
#37889=DIRECTION ( 'NONE',  ( 1.000000000000000000, 0.000000000000000000, 0.000000000000000000 ) ) ;
#37890=CARTESIAN_POINT ( 'NONE',  ( -9.999999999999998224, 1.224646799147353059E-15, -29.74999999999997158 ) ) ;
#37891=ORIENTED_EDGE ( 'NONE', *, *, #14409, .T. ) ;
#37892=EDGE_LOOP ( 'NONE', ( #7847, #18118, #15149, #31324 ) ) ;
#37893=CARTESIAN_POINT ( 'NONE',  ( -5.405949406250003975, -9.363379034771801557, -40.84375000204837391 ) ) ;
#37895=CARTESIAN_POINT ( 'NONE',  ( 7.644554776091147741E-16, 12.48450537969573659, -14.65625000204836859 ) ) ;
#37896=VECTOR ( 'NONE', #18177, 1000.000000000000000 ) ;
#37897=CARTESIAN_POINT ( 'NONE',  ( 10.81189881249999729, 0.000000000000000000, -59.84375000204835970 ) ) ;
#37898=VERTEX_POINT ( 'NONE', #2292 ) ;
#37899=CYLINDRICAL_SURFACE ( 'NONE', #33249, 9.999999999999998224 ) ;
#37901=CARTESIAN_POINT ( 'NONE',  ( -10.81189881249999729, -6.242252689847864744, -192.4687500020484094 ) ) ;
#37902=CARTESIAN_POINT ( 'NONE',  ( 10.81189881249999907, 6.242252689847868297, -173.7187500020484094 ) ) ;
#37905=CARTESIAN_POINT ( 'NONE',  ( -9.999999999999834799, -5.773502691896343464, -193.1250000000000000 ) ) ;
#37908=CARTESIAN_POINT ( 'NONE',  ( -10.81189881249999907, -6.242252689847864744, -109.9687500020483668 ) ) ;
#37909=CARTESIAN_POINT ( 'NONE',  ( -9.999999999999998224, 1.224646799147353059E-15, -87.12500000409677625 ) ) ;
#37910=CARTESIAN_POINT ( 'NONE',  ( -5.405949406249996869, 9.363379034771805109, -83.53125000204838102 ) ) ;
#37911=CARTESIAN_POINT ( 'NONE',  ( 10.81189881249999551, -6.242252689847874514, -92.96875000204838102 ) ) ;
#37914=CARTESIAN_POINT ( 'NONE',  ( -4.999999999999996447, 8.660254037844387298, -157.8750000040967905 ) ) ;
#37918=CARTESIAN_POINT ( 'NONE',  ( -5.000000000000003553, -8.660254037844383745, -13.37500000409674783 ) ) ;
#37919=DIRECTION ( 'NONE',  ( -0.000000000000000000, -0.000000000000000000, 1.000000000000000000 ) ) ;
#37922=CARTESIAN_POINT ( 'NONE',  ( -2.121150477449813534E-15, -11.54700538379251284, -77.37499999999997158 ) ) ;
#37924=CARTESIAN_POINT ( 'NONE',  ( 9.999999999999998224, 0.000000000000000000, -84.87500000409677625 ) ) ;
#37927=CARTESIAN_POINT ( 'NONE',  ( -10.81189881249999729, 1.324075727343319199E-15, -72.78125000204838102 ) ) ;
#37929=CARTESIAN_POINT ( 'NONE',  ( 10.00000000000102318, -5.773502691895667560, -59.12499999999996447 ) ) ;
#37931=ORIENTED_EDGE ( 'NONE', *, *, #4965, .T. ) ;
#37932=CARTESIAN_POINT ( 'NONE',  ( -2.121150477449813534E-15, -11.54700538379251284, -0.8749999999999721334 ) ) ;
#37935=CARTESIAN_POINT ( 'NONE',  ( -10.81189881249999729, -6.242252689847864744, -10.96875000204836859 ) ) ;
#37937=CARTESIAN_POINT ( 'NONE',  ( -10.81189881249999729, 6.242252689847871849, -143.2187500020484094 ) ) ;
#37940=CARTESIAN_POINT ( 'NONE',  ( 10.81189881249999551, -6.242252689847874514, -132.1562500020484094 ) ) ;
#37941=CARTESIAN_POINT ( 'NONE',  ( -10.00000000000000000, -5.773502691896251982, -185.6250000000000284 ) ) ;
#37942=CYLINDRICAL_SURFACE ( 'NONE', #18610, 9.999999999999998224 ) ;
#37943=CARTESIAN_POINT ( 'NONE',  ( 10.81189881249999907, 6.242252689847868297, -107.9062500020483668 ) ) ;
#37944=VERTEX_POINT ( 'NONE', #41746 ) ;
#37945=CARTESIAN_POINT ( 'NONE',  ( 0.000000000000000000, 0.000000000000000000, -200.0000000000000000 ) ) ;
#37946=ORIENTED_EDGE ( 'NONE', *, *, #18751, .T. ) ;
#37949=CARTESIAN_POINT ( 'NONE',  ( 5.405949406249992428, -9.363379034771808662, -40.78125000204838102 ) ) ;
#37951=CARTESIAN_POINT ( 'NONE',  ( 5.405949406249992428, -9.363379034771808662, -84.09375000204836681 ) ) ;
#37955=CARTESIAN_POINT ( 'NONE',  ( 4.999999999999992006, -8.660254037844389075, -86.24999999999998579 ) ) ;
#37958=CARTESIAN_POINT ( 'NONE',  ( 10.81189881249999551, -6.242252689847874514, -118.4687500020483810 ) ) ;
#37960=CARTESIAN_POINT ( 'NONE',  ( -5.405949406249996869, 9.363379034771805109, -5.531250002048376579 ) ) ;
#37963=CARTESIAN_POINT ( 'NONE',  ( 7.070501591499377789E-16, 11.54700538379251284, -179.0000000040967905 ) ) ;
#37964=CARTESIAN_POINT ( 'NONE',  ( 5.405949406249992428, -9.363379034771808662, -169.7812500020484094 ) ) ;
#37968=CARTESIAN_POINT ( 'NONE',  ( 10.81189881249999729, 6.242252689847867408, -55.21875000204836681 ) ) ;
#37971=CARTESIAN_POINT ( 'NONE',  ( -10.81189881249999729, 1.324075727343319199E-15, -5.281250002048376579 ) ) ;
#37975=CARTESIAN_POINT ( 'NONE',  ( -5.000000000000003553, -8.660254037844383745, -101.5000000000000000 ) ) ;
#37977=CARTESIAN_POINT ( 'NONE',  ( 4.999999999999992006, -8.660254037844389075, -103.1250000040967763 ) ) ;
#37980=CARTESIAN_POINT ( 'NONE',  ( -5.405949406250003975, -9.363379034771801557, -98.03125000204839523 ) ) ;
#37982=EDGE_CURVE ( 'NONE', #36710, #1760, #26466, .T. ) ;
#37985=CARTESIAN_POINT ( 'NONE',  ( -2.293366432827344421E-15, -12.48450537969573659, -157.9062500020483810 ) ) ;
#37988=CARTESIAN_POINT ( 'NONE',  ( -5.000000000000003553, -8.660254037844383745, -29.49999999999997158 ) ) ;
#37989=CARTESIAN_POINT ( 'NONE',  ( -10.81189881249999729, -6.242252689847864744, -30.65625000204835260 ) ) ;
#37990=CARTESIAN_POINT ( 'NONE',  ( -9.999999999999998224, 1.224646799147353059E-15, -161.7500000000000000 ) ) ;
#37991=CARTESIAN_POINT ( 'NONE',  ( -9.999999999999479527, -5.773502691896549521, -103.1249999999999858 ) ) ;
#37993=DIRECTION ( 'NONE',  ( -0.000000000000000000, -0.000000000000000000, 1.000000000000000000 ) ) ;
#37994=CARTESIAN_POINT ( 'NONE',  ( 10.81189881249999907, 6.242252689847868297, -137.9062500020483810 ) ) ;
#37995=CARTESIAN_POINT ( 'NONE',  ( 10.55761814654026232, 2.340415281005872039, -2.775557561562896400E-14 ) ) ;
#37996=CARTESIAN_POINT ( 'NONE',  ( 10.00000000000025402, -5.773502691896113426, -188.1250000000000284 ) ) ;
#37998=( BOUNDED_CURVE ( )  B_SPLINE_CURVE ( 2, ( #41775, #15446, #8145, #1458, #21293, #11567, #8364 ),
 .UNSPECIFIED., .F., .F. ) 
 B_SPLINE_CURVE_WITH_KNOTS ( ( 3, 2, 2, 3 ),
 ( 0.1231343283582089221, 0.1243781094527362935, 0.1256218905472636649, 0.1268656716417910224 ),
 .UNSPECIFIED. ) 
 CURVE ( )  GEOMETRIC_REPRESENTATION_ITEM ( )  RATIONAL_B_SPLINE_CURVE ( ( 1.000000000000002887, 0.8660254037844355990, 1.000000000000000000, 0.8660254037844387076, 1.000000000000000000, 0.8660254037844417052, 0.9999999999999970024 ) ) 
 REPRESENTATION_ITEM ( '' )  );
#37999=CARTESIAN_POINT ( 'NONE',  ( 5.405949406249999534, 9.363379034771803333, -64.28125000204836681 ) ) ;
#38002=ORIENTED_EDGE ( 'NONE', *, *, #32327, .F. ) ;
#38006=CARTESIAN_POINT ( 'NONE',  ( 7.644554776091147741E-16, 12.48450537969573659, -158.4687500020483810 ) ) ;
#38008=CARTESIAN_POINT ( 'NONE',  ( -10.81189881249999729, 6.242252689847871849, -6.718750002048347270 ) ) ;
#38009=CARTESIAN_POINT ( 'NONE',  ( -5.405949406250003975, -9.363379034771801557, -145.8437500020483810 ) ) ;
#38010=CARTESIAN_POINT ( 'NONE',  ( -5.405949406250003975, -9.363379034771801557, -95.03125000204838102 ) ) ;
#38012=DIRECTION ( 'NONE',  ( 1.000000000000000000, 0.000000000000000000, 0.000000000000000000 ) ) ;
#38014=CARTESIAN_POINT ( 'NONE',  ( 7.644554776091147741E-16, 12.48450537969573659, -5.468750002048341941 ) ) ;
#38017=CARTESIAN_POINT ( 'NONE',  ( -10.81189881249999729, -6.242252689847864744, -191.1562500020484094 ) ) ;
#38018=CARTESIAN_POINT ( 'NONE',  ( 9.999999999999998224, 0.000000000000000000, -165.8750000040967905 ) ) ;
#38022=CARTESIAN_POINT ( 'NONE',  ( -5.405949406250003975, -9.363379034771801557, -73.84375000204838102 ) ) ;
#38023=CARTESIAN_POINT ( 'NONE',  ( -5.405949406249996869, 9.363379034771805109, -57.84375000204835970 ) ) ;
#38025=CARTESIAN_POINT ( 'NONE',  ( -10.81189881249999729, 6.242252689847871849, -30.90625000204834905 ) ) ;
#38029=CARTESIAN_POINT ( 'NONE',  ( -9.999999999999998224, 1.224646799147353059E-15, -121.2500000000000000 ) ) ;
#38032=CARTESIAN_POINT ( 'NONE',  ( -10.81189881249999729, -6.242252689847864744, -12.65625000204835970 ) ) ;
#38036=DIRECTION ( 'NONE',  ( -0.000000000000000000, -0.000000000000000000, 1.000000000000000000 ) ) ;
#38038=AXIS2_PLACEMENT_3D ( 'NONE', #10376, #33921, #30475 ) ;
#38039=CARTESIAN_POINT ( 'NONE',  ( 5.000000000000000000, 8.660254037844385522, -24.62500000409675849 ) ) ;
#38040=CARTESIAN_POINT ( 'NONE',  ( -2.121150477449813534E-15, -11.54700538379251284, -14.37499999999997335 ) ) ;
#38042=DIRECTION ( 'NONE',  ( -0.000000000000000000, -0.000000000000000000, 1.000000000000000000 ) ) ;
#38043=CARTESIAN_POINT ( 'NONE',  ( 10.81189881249999729, 0.000000000000000000, -147.0312500020483810 ) ) ;
#38044=CARTESIAN_POINT ( 'NONE',  ( 5.405949406249992428, -9.363379034771808662, -129.0937500020483810 ) ) ;
#38045=CARTESIAN_POINT ( 'NONE',  ( -4.999999999999996447, 8.660254037844387298, -50.99999999999996447 ) ) ;
#38046=CARTESIAN_POINT ( 'NONE',  ( -9.999999999999227285, -5.773502691896698735, -127.5000000040967763 ) ) ;
#38047=ORIENTED_EDGE ( 'NONE', *, *, #29337, .T. ) ;
#38050=ORIENTED_EDGE ( 'NONE', *, *, #4231, .F. ) ;
#38052=LINE ( 'NONE', #21645, #9766 ) ;
#38053=CARTESIAN_POINT ( 'NONE',  ( -10.81189881249999729, 1.324075727343319199E-15, -180.5937500020484094 ) ) ;
#38054=CARTESIAN_POINT ( 'NONE',  ( 10.81189881249999729, 0.000000000000000000, -32.84375000204836681 ) ) ;
#38055=DIRECTION ( 'NONE',  ( -0.000000000000000000, -0.000000000000000000, 1.000000000000000000 ) ) ;
#38056=CARTESIAN_POINT ( 'NONE',  ( -5.405949406249996869, 9.363379034771805109, -171.8437500020484094 ) ) ;
#38057=CARTESIAN_POINT ( 'NONE',  ( -10.81189881249999729, 6.242252689847871849, -152.2187500020483526 ) ) ;
#38061=DIRECTION ( 'NONE',  ( -0.000000000000000000, -0.000000000000000000, 1.000000000000000000 ) ) ;
#38062=CARTESIAN_POINT ( 'NONE',  ( 9.999999999999998224, 0.000000000000000000, -183.5000000000000000 ) ) ;
#38064=CARTESIAN_POINT ( 'NONE',  ( 7.644554776091147741E-16, 12.48450537969573659, -78.96875000204839523 ) ) ;
#38065=CARTESIAN_POINT ( 'NONE',  ( 0.000000000000000000, 0.000000000000000000, -200.0000000000000000 ) ) ;
#38066=CARTESIAN_POINT ( 'NONE',  ( 10.81189881249999551, -6.242252689847874514, -58.65625000204838813 ) ) ;
#38070=CARTESIAN_POINT ( 'NONE',  ( -5.405949406250003975, -9.363379034771801557, -117.5312500020483952 ) ) ;
#38071=CARTESIAN_POINT ( 'NONE',  ( -10.81189881249999729, -6.242252689847864744, -147.6562500020483810 ) ) ;
#38074=CARTESIAN_POINT ( 'NONE',  ( -5.000000000000003553, -8.660254037844383745, -118.3750000040967905 ) ) ;
#38076=ORIENTED_EDGE ( 'NONE', *, *, #20022, .F. ) ;
#38079=CARTESIAN_POINT ( 'NONE',  ( -10.81189881249999729, 6.242252689847871849, -183.9062500020484094 ) ) ;
#38080=ORIENTED_EDGE ( 'NONE', *, *, #25981, .T. ) ;
#38082=CARTESIAN_POINT ( 'NONE',  ( -10.00000000000000000, -5.773502691896251982, -57.00000000409676915 ) ) ;
#38083=EDGE_CURVE ( 'NONE', #31273, #12182, #36810, .T. ) ;
#38084=( BOUNDED_CURVE ( )  B_SPLINE_CURVE ( 2, ( #8442, #15315, #18127, #37779, #8861, #37996, #31962 ),
 .UNSPECIFIED., .F., .F. ) 
 B_SPLINE_CURVE_WITH_KNOTS ( ( 3, 2, 2, 3 ),
 ( 0.05597014925373139382, 0.05721393034825875828, 0.05845771144278612275, 0.05970149253731348721 ),
 .UNSPECIFIED. ) 
 CURVE ( )  GEOMETRIC_REPRESENTATION_ITEM ( )  RATIONAL_B_SPLINE_CURVE ( ( 0.9999999999999947820, 0.8660254037844439257, 1.000000000000000000, 0.8660254037844387076, 1.000000000000000000, 0.8660254037844327124, 1.000000000000005995 ) ) 
 REPRESENTATION_ITEM ( '' )  );
#38085=CARTESIAN_POINT ( 'NONE',  ( 0.000000000000000000, 0.000000000000000000, -200.0000000000000000 ) ) ;
#38089=DIRECTION ( 'NONE',  ( 1.000000000000000000, 0.000000000000000000, 0.000000000000000000 ) ) ;
#38090=CARTESIAN_POINT ( 'NONE',  ( 10.81189881249999551, -6.242252689847874514, -172.6562500020484379 ) ) ;
#38094=CARTESIAN_POINT ( 'NONE',  ( -4.999999999999996447, 8.660254037844387298, -16.87500000409675138 ) ) ;
#38095=DIRECTION ( 'NONE',  ( 0.4999999999999998335, 0.8660254037844387076, 0.000000000000000000 ) ) ;
#38096=CARTESIAN_POINT ( 'NONE',  ( 4.999999999999992006, -8.660254037844389075, -163.1250000040967905 ) ) ;
#38097=CARTESIAN_POINT ( 'NONE',  ( -5.405949406250003975, -9.363379034771801557, -74.03125000204838102 ) ) ;
#38098=VERTEX_POINT ( 'NONE', #27103 ) ;
#38100=ORIENTED_EDGE ( 'NONE', *, *, #33639, .F. ) ;
#38102=EDGE_CURVE ( 'NONE', #32122, #14673, #1583, .T. ) ;
#38103=CARTESIAN_POINT ( 'NONE',  ( 5.405949406249999534, 9.363379034771803333, -35.59375000204836681 ) ) ;
#38104=CARTESIAN_POINT ( 'NONE',  ( -9.999999999999998224, 1.224646799147353059E-15, -171.1250000040968189 ) ) ;
#38105=CARTESIAN_POINT ( 'NONE',  ( -5.405949406250003975, -9.363379034771801557, -9.531250002048352599 ) ) ;
#38106=CARTESIAN_POINT ( 'NONE',  ( 5.405949406249992428, -9.363379034771808662, -64.59375000204836681 ) ) ;
#38107=EDGE_LOOP ( 'NONE', ( #28188, #4072, #29910, #41483 ) ) ;
#38108=EDGE_CURVE ( 'NONE', #21458, #25114, #2701, .T. ) ;
#38111=CARTESIAN_POINT ( 'NONE',  ( -10.81189881249999729, -6.242252689847864744, -198.4687500020484094 ) ) ;
#38112=CARTESIAN_POINT ( 'NONE',  ( -2.293366432827344421E-15, -12.48450537969573659, -177.2187500020484094 ) ) ;
#38115=CARTESIAN_POINT ( 'NONE',  ( 10.00000000000051159, -5.773502691895965988, -75.62499999999998579 ) ) ;
#38118=CARTESIAN_POINT ( 'NONE',  ( 7.644554776091147741E-16, 12.48450537969573659, -102.9687500020483952 ) ) ;
#38120=CARTESIAN_POINT ( 'NONE',  ( -10.81189881249999907, -6.242252689847864744, -86.15625000204836681 ) ) ;
#38121=CARTESIAN_POINT ( 'NONE',  ( -10.81189881249999729, 1.324075727343319199E-15, -90.59375000204838102 ) ) ;
#38123=CARTESIAN_POINT ( 'NONE',  ( -10.00000000000000000, -5.773502691896251982, -156.0000000040967905 ) ) ;
#38125=ADVANCED_FACE ( 'NONE', ( #3378 ), #13276, .T. ) ;
#38126=( BOUNDED_CURVE ( )  B_SPLINE_CURVE ( 2, ( #23950, #37094, #445, #26753, #24167, #3672, #10336 ),
 .UNSPECIFIED., .F., .F. ) 
 B_SPLINE_CURVE_WITH_KNOTS ( ( 3, 2, 2, 3 ),
 ( 0.7723880597014927130, 0.7736318407960200982, 0.7748756218905473725, 0.7761194029850747578 ),
 .UNSPECIFIED. ) 
 CURVE ( )  GEOMETRIC_REPRESENTATION_ITEM ( )  RATIONAL_B_SPLINE_CURVE ( ( 0.9999999999999761302, 0.8660254037844625774, 1.000000000000000000, 0.8660254037844387076, 1.000000000000000000, 0.8660254037844267172, 1.000000000000011990 ) ) 
 REPRESENTATION_ITEM ( '' )  );
#38129=CARTESIAN_POINT ( 'NONE',  ( -5.000000000000003553, -8.660254037844383745, -39.99999999999997868 ) ) ;
#38130=CARTESIAN_POINT ( 'NONE',  ( 4.999999999999992006, -8.660254037844389075, -182.2500000000000000 ) ) ;
#38132=ORIENTED_EDGE ( 'NONE', *, *, #36313, .F. ) ;
#38133=CARTESIAN_POINT ( 'NONE',  ( 9.999999999999998224, 0.000000000000000000, -66.49999999999997158 ) ) ;
#38135=CARTESIAN_POINT ( 'NONE',  ( 7.070501591499377789E-16, 11.54700538379251284, -80.00000000409679046 ) ) ;
#38136=CARTESIAN_POINT ( 'NONE',  ( -9.999999999999998224, 1.224646799147353059E-15, -142.6250000040967905 ) ) ;
#38139=CARTESIAN_POINT ( 'NONE',  ( -5.405949406249996869, 9.363379034771805109, -76.03125000204838102 ) ) ;
#38140=( BOUNDED_CURVE ( )  B_SPLINE_CURVE ( 2, ( #37416, #11496, #7858, #4399, #28143, #34196, #24699 ),
 .UNSPECIFIED., .F., .F. ) 
 B_SPLINE_CURVE_WITH_KNOTS ( ( 3, 2, 2, 3 ),
 ( 0.8619402985074630097, 0.8631840796019903950, 0.8644278606965177802, 0.8656716417910450545 ),
 .UNSPECIFIED. ) 
 CURVE ( )  GEOMETRIC_REPRESENTATION_ITEM ( )  RATIONAL_B_SPLINE_CURVE ( ( 0.9999999999999641398, 0.8660254037844745678, 1.000000000000000000, 0.8660254037844387076, 1.000000000000000000, 0.8660254037844028474, 1.000000000000035971 ) ) 
 REPRESENTATION_ITEM ( '' )  );
#38142=CARTESIAN_POINT ( 'NONE',  ( -9.999999999999998224, 1.224646799147353059E-15, -200.0000000000000000 ) ) ;
#38144=ORIENTED_EDGE ( 'NONE', *, *, #16628, .F. ) ;
#38145=CARTESIAN_POINT ( 'NONE',  ( -10.81189881249999729, 6.242252689847871849, -189.9062500020484379 ) ) ;
#38147=CARTESIAN_POINT ( 'NONE',  ( 5.405949406249999534, 9.363379034771803333, -7.093750002048371250 ) ) ;
#38148=CARTESIAN_POINT ( 'NONE',  ( 7.070501591499376803E-16, 11.54700538379251284, -142.6250000000000000 ) ) ;
#38149=CARTESIAN_POINT ( 'NONE',  ( 5.405949406249999534, 9.363379034771803333, -145.0937500020483810 ) ) ;
#38151=DIRECTION ( 'NONE',  ( -0.000000000000000000, -0.000000000000000000, 1.000000000000000000 ) ) ;
#38152=CARTESIAN_POINT ( 'NONE',  ( -9.999999999999998224, 1.224646799147353059E-15, -179.7500000000000284 ) ) ;
#38153=CARTESIAN_POINT ( 'NONE',  ( -9.999999999999998224, 1.224646799147353059E-15, -106.2499999999999858 ) ) ;
#38154=CARTESIAN_POINT ( 'NONE',  ( 10.81189881249999729, 0.000000000000000000, -105.0312500020483810 ) ) ;
#38156=CARTESIAN_POINT ( 'NONE',  ( 9.999999999999998224, 0.000000000000000000, -161.3750000040967905 ) ) ;
#38157=ORIENTED_EDGE ( 'NONE', *, *, #15107, .F. ) ;
#38158=ORIENTED_EDGE ( 'NONE', *, *, #33597, .F. ) ;
#38159=CARTESIAN_POINT ( 'NONE',  ( 5.405949406249999534, 9.363379034771803333, -28.28125000204837036 ) ) ;
#38161=CARTESIAN_POINT ( 'NONE',  ( 10.81189881249999907, 6.242252689847868297, -83.71875000204836681 ) ) ;
#38162=CARTESIAN_POINT ( 'NONE',  ( -9.999999999999998224, 1.224646799147353059E-15, -127.6250000040967620 ) ) ;
#38163=CARTESIAN_POINT ( 'NONE',  ( 7.644554776091147741E-16, 12.48450537969573659, -198.9687500020484094 ) ) ;
#38165=CARTESIAN_POINT ( 'NONE',  ( -5.000000000000003553, -8.660254037844383745, -11.87500000409674783 ) ) ;
#38166=CARTESIAN_POINT ( 'NONE',  ( -9.999999999999998224, 1.224646799147353059E-15, -199.2500000000000000 ) ) ;
#38168=CARTESIAN_POINT ( 'NONE',  ( 10.81189881249999729, 6.242252689847867408, -115.2187500020483810 ) ) ;
#38170=CARTESIAN_POINT ( 'NONE',  ( -5.405949406250003975, -9.363379034771801557, -2.031250002048373915 ) ) ;
#38173=CARTESIAN_POINT ( 'NONE',  ( 9.999999999999998224, 0.000000000000000000, -174.8750000040967905 ) ) ;
#38174=CARTESIAN_POINT ( 'NONE',  ( -5.405949406249996869, 9.363379034771805109, -169.0312500020484094 ) ) ;
#38178=CARTESIAN_POINT ( 'NONE',  ( 10.81189881249999551, -6.242252689847874514, -46.46875000204838102 ) ) ;
#38180=CARTESIAN_POINT ( 'NONE',  ( 10.81189881249999907, 6.242252689847868297, -5.906250002048359704 ) ) ;
#38182=CARTESIAN_POINT ( 'NONE',  ( 7.070501591499376803E-16, 11.54700538379251284, -54.12499999999997158 ) ) ;
#38184=CARTESIAN_POINT ( 'NONE',  ( -9.999999999999998224, 1.224646799147353059E-15, -88.24999999999998579 ) ) ;
#38186=CARTESIAN_POINT ( 'NONE',  ( -10.00000000000000000, -5.773502691896251982, -106.5000000040967763 ) ) ;
#38187=CARTESIAN_POINT ( 'NONE',  ( 9.999999999999998224, 0.000000000000000000, -143.3750000040967905 ) ) ;
#38190=CARTESIAN_POINT ( 'NONE',  ( 10.81189881249999551, -6.242252689847874514, -103.6562500020483810 ) ) ;
#38192=VERTEX_POINT ( 'NONE', #21472 ) ;
#38195=CARTESIAN_POINT ( 'NONE',  ( 10.81189881249999729, 0.000000000000000000, -157.5312500020484094 ) ) ;
#38197=ORIENTED_EDGE ( 'NONE', *, *, #3804, .F. ) ;
#38198=CARTESIAN_POINT ( 'NONE',  ( 10.00000000000000000, 5.773502691896255534, -28.87499999999997868 ) ) ;
#38199=CARTESIAN_POINT ( 'NONE',  ( 10.81189881249999729, 6.242252689847867408, -28.40625000204838813 ) ) ;
#38200=CARTESIAN_POINT ( 'NONE',  ( -9.999999999999998224, 1.224646799147353059E-15, -152.7500000000000000 ) ) ;
#38202=CARTESIAN_POINT ( 'NONE',  ( 4.999999999999992006, -8.660254037844389075, -80.62500000409677625 ) ) ;
#38203=CARTESIAN_POINT ( 'NONE',  ( 10.81189881249999907, 6.242252689847868297, -122.9062500020484094 ) ) ;
#38204=CARTESIAN_POINT ( 'NONE',  ( 9.999999999999227285, 5.773502691896701400, -111.3749999999999432 ) ) ;
#38205=( BOUNDED_CURVE ( )  B_SPLINE_CURVE ( 2, ( #29700, #38981, #9417, #146, #8995, #15659, #40032 ),
 .UNSPECIFIED., .F., .F. ) 
 B_SPLINE_CURVE_WITH_KNOTS ( ( 3, 2, 2, 3 ),
 ( 0.4850746268656717652, 0.4863184079601990950, 0.4875621890547264248, 0.4888059701492538101 ),
 .UNSPECIFIED. ) 
 CURVE ( )  GEOMETRIC_REPRESENTATION_ITEM ( )  RATIONAL_B_SPLINE_CURVE ( ( 0.9999999999999880096, 0.8660254037844506980, 1.000000000000000000, 0.8660254037844387076, 1.000000000000000000, 0.8660254037844327124, 1.000000000000005995 ) ) 
 REPRESENTATION_ITEM ( '' )  );
#38206=CARTESIAN_POINT ( 'NONE',  ( -9.999999999999479527, -5.773502691896549521, -45.00000000409674783 ) ) ;
#38207=ORIENTED_EDGE ( 'NONE', *, *, #18057, .T. ) ;
#38208=CARTESIAN_POINT ( 'NONE',  ( -5.405949406249996869, 9.363379034771805109, -64.03125000204836681 ) ) ;
#38210=CARTESIAN_POINT ( 'NONE',  ( 10.81189881249999907, 6.242252689847868297, -107.7187500020483810 ) ) ;
#38212=ORIENTED_EDGE ( 'NONE', *, *, #41656, .T. ) ;
#38214=CARTESIAN_POINT ( 'NONE',  ( 10.00000000000031619, -5.773502691896077010, -183.6249999999999716 ) ) ;
#38215=CARTESIAN_POINT ( 'NONE',  ( 10.81189881249999729, 0.000000000000000000, -154.3437500020483810 ) ) ;
#38216=ADVANCED_FACE ( 'NONE', ( #14334 ), #34445, .T. ) ;
#38218=CARTESIAN_POINT ( 'NONE',  ( 10.81189881249999551, -6.242252689847874514, -8.968750002048359704 ) ) ;
#38219=CARTESIAN_POINT ( 'NONE',  ( 10.81189881249999729, 0.000000000000000000, -136.3437500020484094 ) ) ;
#38220=CARTESIAN_POINT ( 'NONE',  ( 5.405949406249999534, 9.363379034771803333, -100.2812500020483952 ) ) ;
#38222=CARTESIAN_POINT ( 'NONE',  ( -10.00000000000025580, 5.773502691896109873, -187.3750000000000284 ) ) ;
#38224=CARTESIAN_POINT ( 'NONE',  ( 9.999999999999998224, 0.000000000000000000, -198.8750000040967905 ) ) ;
#38226=CARTESIAN_POINT ( 'NONE',  ( 5.405949406249992428, -9.363379034771808662, -190.7812500020484094 ) ) ;
#38230=CARTESIAN_POINT ( 'NONE',  ( -5.405949406250003975, -9.363379034771801557, -70.84375000204836681 ) ) ;
#38231=CARTESIAN_POINT ( 'NONE',  ( 10.81189881249999551, -6.242252689847874514, -55.46875000204837391 ) ) ;
#38233=CARTESIAN_POINT ( 'NONE',  ( -10.81189881249999729, 1.324075727343319199E-15, -26.28125000204836681 ) ) ;
#38235=CARTESIAN_POINT ( 'NONE',  ( -9.999999999999998224, 1.224646799147353059E-15, -94.62500000409677625 ) ) ;
#38237=CARTESIAN_POINT ( 'NONE',  ( 5.000000000000000000, 8.660254037844385522, -118.7500000000000000 ) ) ;
#38238=EDGE_CURVE ( 'NONE', #15716, #8658, #20574, .T. ) ;
#38242=CARTESIAN_POINT ( 'NONE',  ( -5.405949406250003975, -9.363379034771801557, -12.53125000204835615 ) ) ;
#38243=VERTEX_POINT ( 'NONE', #30567 ) ;
#38248=CARTESIAN_POINT ( 'NONE',  ( -4.999999999999996447, 8.660254037844387298, -49.49999999999998579 ) ) ;
#38249=CARTESIAN_POINT ( 'NONE',  ( -9.999999999999998224, 1.224646799147353059E-15, -24.12500000409675849 ) ) ;
#38251=( BOUNDED_CURVE ( )  B_SPLINE_CURVE ( 2, ( #10270, #3607, #7051, #17373, #14988, #4232, #20836 ),
 .UNSPECIFIED., .F., .F. ) 
 B_SPLINE_CURVE_WITH_KNOTS ( ( 3, 2, 2, 3 ),
 ( 0.6455223880597016350, 0.6467661691542290203, 0.6480099502487564056, 0.6492537313432837909 ),
 .UNSPECIFIED. ) 
 CURVE ( )  GEOMETRIC_REPRESENTATION_ITEM ( )  RATIONAL_B_SPLINE_CURVE ( ( 0.9999999999999880096, 0.8660254037844506980, 1.000000000000000000, 0.8660254037844387076, 1.000000000000000000, 0.8660254037844148378, 1.000000000000023981 ) ) 
 REPRESENTATION_ITEM ( '' )  );
#38252=CARTESIAN_POINT ( 'NONE',  ( -10.00000000000102496, 5.773502691895664007, -23.87499999999995381 ) ) ;
#38253=CARTESIAN_POINT ( 'NONE',  ( 7.644554776091147741E-16, 12.48450537969573659, -142.1562500020483810 ) ) ;
#38254=CARTESIAN_POINT ( 'NONE',  ( -10.81189881249999907, -6.242252689847864744, -129.4687500020483810 ) ) ;
#38256=EDGE_LOOP ( 'NONE', ( #16140, #34869, #35199, #4707 ) ) ;
#38258=VERTEX_POINT ( 'NONE', #24735 ) ;
#38259=ORIENTED_EDGE ( 'NONE', *, *, #34944, .T. ) ;
#38260=CARTESIAN_POINT ( 'NONE',  ( 0.000000000000000000, 0.000000000000000000, -200.0000000000000000 ) ) ;
#38261=CARTESIAN_POINT ( 'NONE',  ( -5.405949406250003975, -9.363379034771801557, -178.8437500020483810 ) ) ;
#38262=CARTESIAN_POINT ( 'NONE',  ( -5.405949406250003975, -9.363379034771801557, -30.34375000204836326 ) ) ;
#38263=CARTESIAN_POINT ( 'NONE',  ( -9.999999999999998224, 1.224646799147353059E-15, -109.6250000040967763 ) ) ;
#38264=CARTESIAN_POINT ( 'NONE',  ( -5.405949406250003975, -9.363379034771801557, -160.8437500020484094 ) ) ;
#38265=CARTESIAN_POINT ( 'NONE',  ( 5.405949406249999534, 9.363379034771803333, -157.0937500020483810 ) ) ;
#38266=CARTESIAN_POINT ( 'NONE',  ( -9.999999999999998224, 1.224646799147353059E-15, -200.0000000000000000 ) ) ;
#38268=AXIS2_PLACEMENT_3D ( 'NONE', #33028, #32034, #16593 ) ;
#38271=CARTESIAN_POINT ( 'NONE',  ( 9.999999999999742428, 5.773502691896404748, -135.3750000000000000 ) ) ;
#38272=CARTESIAN_POINT ( 'NONE',  ( -4.999999999999996447, 8.660254037844387298, -10.87500000409674605 ) ) ;
#38274=CARTESIAN_POINT ( 'NONE',  ( -10.81189881249999729, 6.242252689847871849, -78.71875000204838102 ) ) ;
#38276=CARTESIAN_POINT ( 'NONE',  ( 10.81189881249999907, 6.242252689847868297, -49.40625000204837391 ) ) ;
#38277=CARTESIAN_POINT ( 'NONE',  ( 0.000000000000000000, 0.000000000000000000, -200.0000000000000000 ) ) ;
#38279=CARTESIAN_POINT ( 'NONE',  ( 10.81189881249999729, 0.000000000000000000, -117.0312500020483952 ) ) ;
#38280=CARTESIAN_POINT ( 'NONE',  ( 5.405949406249999534, 9.363379034771803333, -143.7812500020483810 ) ) ;
#38281=CARTESIAN_POINT ( 'NONE',  ( 9.999999999999998224, 0.000000000000000000, -138.5000000000000000 ) ) ;
#38283=CARTESIAN_POINT ( 'NONE',  ( 9.999999999999998224, 0.000000000000000000, -122.3750000040967905 ) ) ;
#38285=ORIENTED_EDGE ( 'NONE', *, *, #38893, .F. ) ;
#38290=CARTESIAN_POINT ( 'NONE',  ( 5.405949406249999534, 9.363379034771803333, -176.7812500020484094 ) ) ;
#38291=ORIENTED_EDGE ( 'NONE', *, *, #27809, .F. ) ;
#38293=CARTESIAN_POINT ( 'NONE',  ( -5.000000000000003553, -8.660254037844383745, -53.87500000409675494 ) ) ;
#38294=EDGE_CURVE ( 'NONE', #33541, #16838, #35243, .T. ) ;
#38295=CYLINDRICAL_SURFACE ( 'NONE', #9729, 9.999999999999998224 ) ;
#38298=CARTESIAN_POINT ( 'NONE',  ( 7.070501591499376803E-16, 11.54700538379251284, -84.12499999999997158 ) ) ;
#38299=CARTESIAN_POINT ( 'NONE',  ( -5.405949406249996869, 9.363379034771805109, -167.5312500020484094 ) ) ;
#38300=CARTESIAN_POINT ( 'NONE',  ( -10.00000000000102496, 5.773502691895664007, -1.750000004096726069 ) ) ;
#38301=CARTESIAN_POINT ( 'NONE',  ( 9.999999999998969713, 5.773502691896851502, -64.87499999999997158 ) ) ;
#38302=ORIENTED_EDGE ( 'NONE', *, *, #42405, .F. ) ;
#38303=DIRECTION ( 'NONE',  ( -0.000000000000000000, -0.000000000000000000, 1.000000000000000000 ) ) ;
#38307=DIRECTION ( 'NONE',  ( -0.000000000000000000, -0.000000000000000000, 1.000000000000000000 ) ) ;
#38308=CARTESIAN_POINT ( 'NONE',  ( -10.81189881249999729, 6.242252689847871849, -81.90625000204838102 ) ) ;
#38309=ORIENTED_EDGE ( 'NONE', *, *, #382, .F. ) ;
#38310=CARTESIAN_POINT ( 'NONE',  ( 10.00000000000025402, -5.773502691896113426, -188.5000000040968473 ) ) ;
#38311=ORIENTED_EDGE ( 'NONE', *, *, #13771, .T. ) ;
#38312=AXIS2_PLACEMENT_3D ( 'NONE', #7465, #20615, #33802 ) ;
#38313=ORIENTED_EDGE ( 'NONE', *, *, #34824, .F. ) ;
#38314=CARTESIAN_POINT ( 'NONE',  ( 5.405949406249992428, -9.363379034771808662, -33.09375000204836681 ) ) ;
#38315=CARTESIAN_POINT ( 'NONE',  ( 10.00000000000102318, -5.773502691895667560, -53.12499999999995737 ) ) ;
#38316=CARTESIAN_POINT ( 'NONE',  ( -10.81189881249999729, 6.242252689847871849, -3.906250002048350822 ) ) ;
#38317=CARTESIAN_POINT ( 'NONE',  ( -2.293366432827344421E-15, -12.48450537969573659, -54.21875000204838102 ) ) ;
#38319=CARTESIAN_POINT ( 'NONE',  ( -9.999999999999998224, 1.224646799147353059E-15, -28.24999999999996803 ) ) ;
#38321=CARTESIAN_POINT ( 'NONE',  ( -5.405949406250003975, -9.363379034771801557, -198.3437500020484094 ) ) ;
#38322=CARTESIAN_POINT ( 'NONE',  ( 7.644554776091147741E-16, 12.48450537969573659, -177.9687500020483810 ) ) ;
#38325=CARTESIAN_POINT ( 'NONE',  ( 9.999999999999998224, 0.000000000000000000, -200.0000000000000000 ) ) ;
#38327=CARTESIAN_POINT ( 'NONE',  ( -10.81189881249999907, -6.242252689847864744, -102.4687500020483810 ) ) ;
#38328=DIRECTION ( 'NONE',  ( -0.000000000000000000, -0.000000000000000000, 1.000000000000000000 ) ) ;
#38329=CARTESIAN_POINT ( 'NONE',  ( 5.405949406249992428, -9.363379034771808662, -82.78125000204838102 ) ) ;
#38330=CARTESIAN_POINT ( 'NONE',  ( -5.405949406250003975, -9.363379034771801557, -88.84375000204838102 ) ) ;
#38331=( BOUNDED_CURVE ( )  B_SPLINE_CURVE ( 2, ( #10221, #3974, #36556, #10855, #7420 ),
 .UNSPECIFIED., .F., .F. ) 
 B_SPLINE_CURVE_WITH_KNOTS ( ( 3, 2, 3 ),
 ( 0.9925373134328360214, 0.9937810945273632957, 0.9950248756218905699 ),
 .UNSPECIFIED. ) 
 CURVE ( )  GEOMETRIC_REPRESENTATION_ITEM ( )  RATIONAL_B_SPLINE_CURVE ( ( 0.9999999999999761302, 0.8660254037844625774, 1.000000000000000000, 0.8660254037844387076, 1.000000000000000000 ) ) 
 REPRESENTATION_ITEM ( '' )  );
#38333=CARTESIAN_POINT ( 'NONE',  ( -2.121150477449813534E-15, -11.54700538379251284, -146.7500000040968189 ) ) ;
#38338=CARTESIAN_POINT ( 'NONE',  ( -9.999999999999998224, 1.224646799147353059E-15, -147.1250000040967905 ) ) ;
#38339=DIRECTION ( 'NONE',  ( -0.000000000000000000, -0.000000000000000000, 1.000000000000000000 ) ) ;
#38341=ORIENTED_EDGE ( 'NONE', *, *, #42513, .T. ) ;
#38342=CARTESIAN_POINT ( 'NONE',  ( 4.999999999999992006, -8.660254037844389075, -63.74999999999997158 ) ) ;
#38344=CARTESIAN_POINT ( 'NONE',  ( -9.999999999999998224, 5.773502691896259087, -75.25000000409677625 ) ) ;
#38346=CARTESIAN_POINT ( 'NONE',  ( 9.999999999999998224, 0.000000000000000000, -141.8750000040967905 ) ) ;
#38349=CARTESIAN_POINT ( 'NONE',  ( -10.81189881249999729, -6.242252689847864744, -75.65625000204836681 ) ) ;
#38352=DIRECTION ( 'NONE',  ( -0.000000000000000000, -0.000000000000000000, 1.000000000000000000 ) ) ;
#38354=VERTEX_POINT ( 'NONE', #27745 ) ;
#38355=CARTESIAN_POINT ( 'NONE',  ( 10.81189881249999729, 0.000000000000000000, -196.5312500020484094 ) ) ;
#38356=EDGE_CURVE ( 'NONE', #19091, #18719, #28177, .T. ) ;
#38358=CARTESIAN_POINT ( 'NONE',  ( 5.405949406249999534, 9.363379034771803333, -4.093750002048368586 ) ) ;
#38360=CARTESIAN_POINT ( 'NONE',  ( -2.121150477449813534E-15, -11.54700538379251284, -50.37499999999998579 ) ) ;
#38362=DIRECTION ( 'NONE',  ( -0.5000000000000003331, 0.8660254037844383745, 0.000000000000000000 ) ) ;
#38363=CARTESIAN_POINT ( 'NONE',  ( -5.000000000000003553, -8.660254037844383745, -175.0000000000000284 ) ) ;
#38364=FACE_OUTER_BOUND ( 'NONE', #35924, .T. ) ;
#38365=CARTESIAN_POINT ( 'NONE',  ( 7.644554776091147741E-16, 12.48450537969573659, -101.6562500020483952 ) ) ;
#38367=CARTESIAN_POINT ( 'NONE',  ( 10.00000000000025402, -5.773502691896113426, -164.1250000000000284 ) ) ;
#38368=ORIENTED_EDGE ( 'NONE', *, *, #35354, .F. ) ;
#38369=ORIENTED_EDGE ( 'NONE', *, *, #13936, .F. ) ;
#38370=CARTESIAN_POINT ( 'NONE',  ( 5.405949406249992428, -9.363379034771808662, -28.78125000204837036 ) ) ;
#38373=CARTESIAN_POINT ( 'NONE',  ( -10.81189881249999729, 1.324075727343319199E-15, -78.59375000204838102 ) ) ;
#38379=CARTESIAN_POINT ( 'NONE',  ( 5.000000000000000000, 8.660254037844385522, -14.12500000409674961 ) ) ;
#38381=CARTESIAN_POINT ( 'NONE',  ( 5.405949406249999534, 9.363379034771803333, -118.0937500020483810 ) ) ;
#38385=CARTESIAN_POINT ( 'NONE',  ( -4.999999999999996447, 8.660254037844387298, -166.8750000040967905 ) ) ;
#38386=CARTESIAN_POINT ( 'NONE',  ( 10.81189881249999551, -6.242252689847874514, -174.1562500020484094 ) ) ;
#38387=( BOUNDED_CURVE ( )  B_SPLINE_CURVE ( 2, ( #40498, #37067, #13953, #7509, #27362, #31038, #17412 ),
 .UNSPECIFIED., .F., .F. ) 
 B_SPLINE_CURVE_WITH_KNOTS ( ( 3, 2, 2, 3 ),
 ( 0.8955223880597017461, 0.8967661691542291313, 0.8980099502487565166, 0.8992537313432839019 ),
 .UNSPECIFIED. ) 
 CURVE ( )  GEOMETRIC_REPRESENTATION_ITEM ( )  RATIONAL_B_SPLINE_CURVE ( ( 0.9999999999999761302, 0.8660254037844625774, 1.000000000000000000, 0.8660254037844387076, 1.000000000000000000, 0.8660254037844028474, 1.000000000000035971 ) ) 
 REPRESENTATION_ITEM ( '' )  );
#38388=CARTESIAN_POINT ( 'NONE',  ( 9.999999999999998224, 0.000000000000000000, -69.87500000409677625 ) ) ;
#38391=CARTESIAN_POINT ( 'NONE',  ( -10.81189881249999729, 6.242252689847871849, -44.21875000204835970 ) ) ;
#38393=CARTESIAN_POINT ( 'NONE',  ( 7.644554776091147741E-16, 12.48450537969573659, -1.156250002048369474 ) ) ;
#38395=CARTESIAN_POINT ( 'NONE',  ( 10.00000000000038369, -5.773502691896038819, -152.5000000040967620 ) ) ;
#38397=CARTESIAN_POINT ( 'NONE',  ( -9.999999999999998224, 1.224646799147353059E-15, -86.74999999999998579 ) ) ;
#38399=CARTESIAN_POINT ( 'NONE',  ( -9.999999999999998224, 5.773502691896259087, -103.7500000040967620 ) ) ;
#38402=CARTESIAN_POINT ( 'NONE',  ( 10.81189881249999729, 0.000000000000000000, -103.5312500020483810 ) ) ;
#38403=ORIENTED_EDGE ( 'NONE', *, *, #19995, .T. ) ;
#38405=CARTESIAN_POINT ( 'NONE',  ( -9.999999999999998224, 1.224646799147353059E-15, -71.74999999999998579 ) ) ;
#38406=CARTESIAN_POINT ( 'NONE',  ( 5.405949406249999534, 9.363379034771803333, -154.2812500020484094 ) ) ;
#38409=CARTESIAN_POINT ( 'NONE',  ( 10.00000000000000000, 5.773502691896255534, -21.37499999999997513 ) ) ;
#38410=CLOSED_SHELL ( 'NONE', ( #16408, #17058, #21132, #27122, #36228, #3984, #3027, #25445, #21070, #27156, #6917, #41268, #35145, #27272, #182, #24201, #38415, #35959, #25875, #39532, #8274, #1424, #3496, #28983, #29625, #36715, #6741, #31536, #25154, #16839, #32268, #12610, #39671, #24682, #14997, #4647, #26695, #8488, #42541, #5406, #39960, #38754, #3808, #40896, #28321, #27531, #12062, #19354, #41853, #40837, #14571, #778, #21002, #40435, #6206, #40404, #19495, #26208, #19460, #11712, #27215, #10094, #17289, #1173, #23316, #22225, #29334, #25692, #10675, #21680, #18319, #29657, #17731, #26743, #32925, #1794, #20964, #33477, #23238, #13224, #35965, #22286, #35962, #28685, #21553, #31796, #10249, #10740, #36803, #12090, #39884, #34726, #30415, #35219, #29827, #6057, #37304, #6202, #34391, #9221, #38583, #14367, #29795, #2737, #54, #649, #38125, #7366, #4817, #21971, #40524, #25158, #18940, #137, #26577, #29019, #25751, #1368, #14544, #21321, #14837, #11681, #6695, #42034, #6682, #6988, #22398, #29620, #4881, #23053, #30994, #17417, #15806, #24691, #4201, #3559, #12872, #33164, #8013, #41492, #11621, #39640, #38624, #42014, #29013, #21803, #16158, #10363, #33043, #42690, #10126, #18130, #22783, #16096, #10362, #19732, #33088, #12449, #16928, #6803, #359, #12485, #39347, #36028, #7619, #905, #15750, #39368, #12642, #42570, #24379, #23543, #34008, #16386, #2333, #16190, #41221, #594, #35460, #678, #3777, #12452, #25185, #33756, #42438, #15141, #13811, #40198, #8833, #41258, #19885, #22334, #34776, #32809, #30172, #32687, #3537, #5728, #38503, #40950, #5363, #30472, #37027, #18810, #28270, #14231, #25392, #23876, #6310, #10843, #13456, #24508, #2977, #14335, #24132, #9438, #31275, #4899, #24623, #32507, #30855, #30166, #40606, #3013, #14459, #5074, #22503, #1490, #2467, #11138, #13297, #13993, #5132, #26812, #30197, #5670, #5019, #25292, #25639, #31604, #42464, #33940, #35443, #28612, #20642, #13280, #10718, #7694, #39902, #12398, #28616, #19870, #13047, #9617, #20583, #25178, #6040, #40719, #21358, #34480, #11263, #10118, #8774, #40178, #23426, #17472, #20028, #114, #29226, #24794, #6383, #27107, #12489, #2442, #894, #3055, #9540, #36758, #41738, #13869, #28813, #37029, #16574, #21889, #18879, #15032, #38216, #27803, #24640, #11194, #14602, #6719, #18006, #3329, #15690, #39382, #26047 ) ) ;
#38411=CARTESIAN_POINT ( 'NONE',  ( 10.81189881249999551, -6.242252689847874514, -27.15625000204838102 ) ) ;
#38412=CARTESIAN_POINT ( 'NONE',  ( 10.00000000000000000, 5.773502691896255534, -153.3750000000000000 ) ) ;
#38414=CARTESIAN_POINT ( 'NONE',  ( 5.000000000000000000, 8.660254037844385522, -198.2500000000000000 ) ) ;
#38415=ADVANCED_FACE ( 'NONE', ( #1853 ), #37228, .T. ) ;
#38416=CARTESIAN_POINT ( 'NONE',  ( 5.405949406249992428, -9.363379034771808662, -123.2812500020483952 ) ) ;
#38418=LINE ( 'NONE', #29775, #5557 ) ;
#38419=CARTESIAN_POINT ( 'NONE',  ( -9.999999999999998224, 1.224646799147353059E-15, -45.12500000409677625 ) ) ;
#38420=ORIENTED_EDGE ( 'NONE', *, *, #41768, .T. ) ;
#38421=CARTESIAN_POINT ( 'NONE',  ( -10.81189881249999907, -6.242252689847864744, -56.15625000204837391 ) ) ;
#38423=CARTESIAN_POINT ( 'NONE',  ( -10.81189881249999729, 6.242252689847871849, -110.2187500020483810 ) ) ;
#38424=ORIENTED_EDGE ( 'NONE', *, *, #38102, .T. ) ;
#38426=CARTESIAN_POINT ( 'NONE',  ( 9.999999999999998224, 0.000000000000000000, -83.37500000409677625 ) ) ;
#38428=CARTESIAN_POINT ( 'NONE',  ( -10.81189881249999907, -6.242252689847864744, -159.4687500020484094 ) ) ;
#38430=CARTESIAN_POINT ( 'NONE',  ( -5.405949406249996869, 9.363379034771805109, -6.843750002048371250 ) ) ;
#38431=CARTESIAN_POINT ( 'NONE',  ( 5.405949406249992428, -9.363379034771808662, -142.5937500020483810 ) ) ;
#38435=CARTESIAN_POINT ( 'NONE',  ( 5.000000000000000000, 8.660254037844385522, -198.6250000040967905 ) ) ;
#38437=CARTESIAN_POINT ( 'NONE',  ( 5.405949406249992428, -9.363379034771808662, -198.2812500020484094 ) ) ;
#38440=CARTESIAN_POINT ( 'NONE',  ( -5.405949406250003975, -9.363379034771801557, -67.84375000204836681 ) ) ;
#38441=CARTESIAN_POINT ( 'NONE',  ( -2.293366432827344421E-15, -12.48450537969573659, -60.21875000204837391 ) ) ;
#38443=CARTESIAN_POINT ( 'NONE',  ( 5.405949406249999534, 9.363379034771803333, -25.28125000204836681 ) ) ;
#38444=AXIS2_PLACEMENT_3D ( 'NONE', #23254, #19786, #3623 ) ;
#38446=CARTESIAN_POINT ( 'NONE',  ( -4.999999999999996447, 8.660254037844387298, -31.87500000409676559 ) ) ;
#38448=CARTESIAN_POINT ( 'NONE',  ( 9.999999999999996447, -5.773502691896262640, -113.1250000000000000 ) ) ;
#38449=VECTOR ( 'NONE', #2090, 1000.000000000000000 ) ;
#38453=CARTESIAN_POINT ( 'NONE',  ( -10.81189881249999729, 6.242252689847871849, -9.906250002048379244 ) ) ;
#38454=ORIENTED_EDGE ( 'NONE', *, *, #13812, .F. ) ;
#38455=CARTESIAN_POINT ( 'NONE',  ( -9.999999999999998224, 1.224646799147353059E-15, -50.74999999999996447 ) ) ;
#38457=CARTESIAN_POINT ( 'NONE',  ( -2.121150477449813534E-15, -11.54700538379251284, -128.3750000000000000 ) ) ;
#38459=CARTESIAN_POINT ( 'NONE',  ( -5.000000000000003553, -8.660254037844383745, -41.49999999999997868 ) ) ;
#38460=CARTESIAN_POINT ( 'NONE',  ( 5.000000000000000000, 8.660254037844385522, -26.12500000409675849 ) ) ;
#38464=CARTESIAN_POINT ( 'NONE',  ( 9.999999999999998224, 0.000000000000000000, -80.37500000409677625 ) ) ;
#38465=CARTESIAN_POINT ( 'NONE',  ( -10.81189881249999907, -6.242252689847864744, -144.6562500020484094 ) ) ;
#38466=CARTESIAN_POINT ( 'NONE',  ( 10.81189881249999729, 0.000000000000000000, -147.0312500020483810 ) ) ;
#38467=CARTESIAN_POINT ( 'NONE',  ( 9.999999999999998224, 0.000000000000000000, -126.8750000040967905 ) ) ;
#38468=ORIENTED_EDGE ( 'NONE', *, *, #34188, .F. ) ;
#38469=VERTEX_POINT ( 'NONE', #11532 ) ;
#38471=ORIENTED_EDGE ( 'NONE', *, *, #30471, .F. ) ;
#38472=EDGE_CURVE ( 'NONE', #17679, #107, #2963, .T. ) ;
#38474=CARTESIAN_POINT ( 'NONE',  ( 7.644554776091147741E-16, 12.48450537969573659, -177.9687500020483810 ) ) ;
#38475=CARTESIAN_POINT ( 'NONE',  ( 7.644554776091147741E-16, 12.48450537969573659, -32.46875000204835970 ) ) ;
#38476=CYLINDRICAL_SURFACE ( 'NONE', #28135, 9.999999999999998224 ) ;
#38477=CARTESIAN_POINT ( 'NONE',  ( -5.405949406249996869, 9.363379034771805109, -164.3437500020484094 ) ) ;
#38478=CARTESIAN_POINT ( 'NONE',  ( -10.81189881249999729, 1.324075727343319199E-15, -155.0937500020483810 ) ) ;
#38479=DIRECTION ( 'NONE',  ( -0.000000000000000000, -0.000000000000000000, 1.000000000000000000 ) ) ;
#38482=CARTESIAN_POINT ( 'NONE',  ( 9.999999999999998224, 0.000000000000000000, -3.499999999999975131 ) ) ;
#38484=LINE ( 'NONE', #18849, #28168 ) ;
#38485=CARTESIAN_POINT ( 'NONE',  ( 9.999999999999479527, 5.773502691896553074, -33.75000000409673362 ) ) ;
#38487=CARTESIAN_POINT ( 'NONE',  ( 5.405949406249999534, 9.363379034771803333, -77.59375000204838102 ) ) ;
#38489=CARTESIAN_POINT ( 'NONE',  ( -5.405949406249996869, 9.363379034771805109, -52.03125000204835970 ) ) ;
#38492=CARTESIAN_POINT ( 'NONE',  ( 9.999999999999998224, 0.000000000000000000, -140.0000000000000000 ) ) ;
#38493=CARTESIAN_POINT ( 'NONE',  ( -10.81189881249999729, 6.242252689847871849, -143.4062500020484094 ) ) ;
#38494=CYLINDRICAL_SURFACE ( 'NONE', #20632, 9.999999999999998224 ) ;
#38496=CARTESIAN_POINT ( 'NONE',  ( 9.999999999999998224, 0.000000000000000000, -120.8750000040967905 ) ) ;
#38498=( BOUNDED_CURVE ( )  B_SPLINE_CURVE ( 2, ( #6649, #7079, #36633, #16979, #3844, #9883, #36844 ),
 .UNSPECIFIED., .F., .F. ) 
 B_SPLINE_CURVE_WITH_KNOTS ( ( 3, 2, 2, 3 ),
 ( 0.7201492537313435305, 0.7213930348258709158, 0.7226368159203983010, 0.7238805970149256863 ),
 .UNSPECIFIED. ) 
 CURVE ( )  GEOMETRIC_REPRESENTATION_ITEM ( )  RATIONAL_B_SPLINE_CURVE ( ( 0.9999999999999761302, 0.8660254037844625774, 1.000000000000000000, 0.8660254037844387076, 1.000000000000000000, 0.8660254037844028474, 1.000000000000035971 ) ) 
 REPRESENTATION_ITEM ( '' )  );
#38499=EDGE_LOOP ( 'NONE', ( #42260, #35721, #17134, #32715 ) ) ;
#38502=DIRECTION ( 'NONE',  ( -0.000000000000000000, -0.000000000000000000, 1.000000000000000000 ) ) ;
#38503=ADVANCED_FACE ( 'NONE', ( #25997 ), #42370, .T. ) ;
#38504=CARTESIAN_POINT ( 'NONE',  ( 5.405949406249999534, 9.363379034771803333, -170.7812500020484094 ) ) ;
#38505=CARTESIAN_POINT ( 'NONE',  ( 9.999999999999996447, -5.773502691896262640, -52.00000000409676915 ) ) ;
#38508=CARTESIAN_POINT ( 'NONE',  ( 7.070501591499376803E-16, 11.54700538379251284, -9.500000004096756712 ) ) ;
#38509=CARTESIAN_POINT ( 'NONE',  ( -10.81189881249999907, -6.242252689847864744, -167.1562500020483810 ) ) ;
#38510=CARTESIAN_POINT ( 'NONE',  ( 9.999999999999998224, 0.000000000000000000, -7.999999999999952038 ) ) ;
#38511=CARTESIAN_POINT ( 'NONE',  ( 9.999999999999998224, 0.000000000000000000, -33.87500000409676915 ) ) ;
#38512=VERTEX_POINT ( 'NONE', #9579 ) ;
#38514=CARTESIAN_POINT ( 'NONE',  ( 7.070501591499376803E-16, 11.54700538379251284, -123.5000000040967905 ) ) ;
#38515=FACE_OUTER_BOUND ( 'NONE', #33238, .T. ) ;
#38516=CARTESIAN_POINT ( 'NONE',  ( -10.81189881249999729, 1.324075727343319199E-15, -81.78125000204839523 ) ) ;
#38519=CARTESIAN_POINT ( 'NONE',  ( -9.999999999999998224, 1.224646799147353059E-15, -143.7500000000000000 ) ) ;
#38520=ORIENTED_EDGE ( 'NONE', *, *, #15084, .F. ) ;
#38521=ORIENTED_EDGE ( 'NONE', *, *, #9018, .T. ) ;
#38522=CARTESIAN_POINT ( 'NONE',  ( 5.405949406249999534, 9.363379034771803333, -31.09375000204836326 ) ) ;
#38523=CARTESIAN_POINT ( 'NONE',  ( 9.999999999999998224, 0.000000000000000000, -52.99999999999996447 ) ) ;
#38524=CARTESIAN_POINT ( 'NONE',  ( -2.293366432827344421E-15, -12.48450537969573659, -6.406250002048362369 ) ) ;
#38525=CARTESIAN_POINT ( 'NONE',  ( 10.81189881249999551, -6.242252689847874514, -53.96875000204838102 ) ) ;
#38526=ORIENTED_EDGE ( 'NONE', *, *, #9068, .F. ) ;
#38527=EDGE_CURVE ( 'NONE', #17561, #17891, #34987, .T. ) ;
#38529=CARTESIAN_POINT ( 'NONE',  ( -10.81189881249999729, 6.242252689847871849, -189.7187500020484379 ) ) ;
#38530=CARTESIAN_POINT ( 'NONE',  ( -5.405949406250003975, -9.363379034771801557, -178.8437500020483810 ) ) ;
#38533=CARTESIAN_POINT ( 'NONE',  ( -9.999999999999998224, 1.224646799147353059E-15, -72.12500000409677625 ) ) ;
#38537=CARTESIAN_POINT ( 'NONE',  ( -5.405949406249996869, 9.363379034771805109, -101.3437500020483810 ) ) ;
#38538=CARTESIAN_POINT ( 'NONE',  ( 9.999999999998969713, 5.773502691896851502, -18.37499999999995026 ) ) ;
#38539=CARTESIAN_POINT ( 'NONE',  ( -10.81189881249999729, 1.324075727343319199E-15, -75.78125000204838102 ) ) ;
#38540=CARTESIAN_POINT ( 'NONE',  ( -5.405949406249996869, 9.363379034771805109, -90.84375000204838102 ) ) ;
#38542=CARTESIAN_POINT ( 'NONE',  ( 5.000000000000000000, 8.660254037844385522, -149.1250000040967905 ) ) ;
#38548=CARTESIAN_POINT ( 'NONE',  ( 10.00000000000102318, -5.773502691895667560, -51.62499999999995737 ) ) ;
#38551=CARTESIAN_POINT ( 'NONE',  ( 9.999999999999998224, 0.000000000000000000, -61.99999999999997158 ) ) ;
#38553=CARTESIAN_POINT ( 'NONE',  ( -5.000000000000003553, -8.660254037844383745, -71.87500000409677625 ) ) ;
#38554=DIRECTION ( 'NONE',  ( -0.000000000000000000, -0.000000000000000000, -1.000000000000000000 ) ) ;
#38555=CYLINDRICAL_SURFACE ( 'NONE', #4503, 9.999999999999998224 ) ;
#38557=CARTESIAN_POINT ( 'NONE',  ( 5.405949406249999534, 9.363379034771803333, -67.28125000204838102 ) ) ;
#38559=CARTESIAN_POINT ( 'NONE',  ( -2.121150477449813534E-15, -11.54700538379251284, -77.75000000409677625 ) ) ;
#38561=VERTEX_POINT ( 'NONE', #34868 ) ;
#38562=CARTESIAN_POINT ( 'NONE',  ( 10.81189881249999729, 0.000000000000000000, -193.5312500020484094 ) ) ;
#38564=CARTESIAN_POINT ( 'NONE',  ( -5.405949406250003975, -9.363379034771801557, -9.343750002048345493 ) ) ;
#38566=CARTESIAN_POINT ( 'NONE',  ( -9.999999999999998224, 1.224646799147353059E-15, -37.62500000409676915 ) ) ;
#38567=CARTESIAN_POINT ( 'NONE',  ( 9.999999999999998224, 0.000000000000000000, -147.5000000000000000 ) ) ;
#38568=CARTESIAN_POINT ( 'NONE',  ( 9.999999999999996447, -5.773502691896262640, -173.1250000000000000 ) ) ;
#38569=DIRECTION ( 'NONE',  ( 1.000000000000000000, 0.000000000000000000, 0.000000000000000000 ) ) ;
#38571=CARTESIAN_POINT ( 'NONE',  ( 10.81189881249999551, -6.242252689847874514, -105.1562500020483810 ) ) ;
#38573=DIRECTION ( 'NONE',  ( -0.000000000000000000, -0.000000000000000000, 1.000000000000000000 ) ) ;
#38574=ORIENTED_EDGE ( 'NONE', *, *, #42648, .T. ) ;
#38575=ORIENTED_EDGE ( 'NONE', *, *, #8798, .T. ) ;
#38577=CARTESIAN_POINT ( 'NONE',  ( -5.405949406250003975, -9.363379034771801557, -27.53125000204836681 ) ) ;
#38578=CARTESIAN_POINT ( 'NONE',  ( 7.644554776091147741E-16, 12.48450537969573659, -80.46875000204838102 ) ) ;
#38579=DIRECTION ( 'NONE',  ( -0.000000000000000000, -0.000000000000000000, 1.000000000000000000 ) ) ;
#38580=EDGE_CURVE ( 'NONE', #27810, #17561, #41734, .T. ) ;
#38582=( BOUNDED_CURVE ( )  B_SPLINE_CURVE ( 2, ( #20772, #33961, #17734, #17310, #40392, #36752, #940 ),
 .UNSPECIFIED., .F., .F. ) 
 B_SPLINE_CURVE_WITH_KNOTS ( ( 3, 2, 2, 3 ),
 ( 0.2649253731343284568, 0.2661691542288558421, 0.2674129353233831718, 0.2686567164179105571 ),
 .UNSPECIFIED. ) 
 CURVE ( )  GEOMETRIC_REPRESENTATION_ITEM ( )  RATIONAL_B_SPLINE_CURVE ( ( 0.9999999999999880096, 0.8660254037844506980, 1.000000000000000000, 0.8660254037844387076, 1.000000000000000000, 0.8660254037844267172, 1.000000000000011990 ) ) 
 REPRESENTATION_ITEM ( '' )  );
#38583=ADVANCED_FACE ( 'NONE', ( #15407 ), #12173, .T. ) ;
#38584=EDGE_CURVE ( 'NONE', #5784, #5415, #32057, .T. ) ;
#38586=CARTESIAN_POINT ( 'NONE',  ( -4.999999999999996447, 8.660254037844387298, -30.37500000409676204 ) ) ;
#38588=CARTESIAN_POINT ( 'NONE',  ( 4.999999999999992006, -8.660254037844389075, -8.625000004096744277 ) ) ;
#38589=CARTESIAN_POINT ( 'NONE',  ( -9.999999999998969713, -5.773502691896847949, -86.62499999999995737 ) ) ;
#38590=CARTESIAN_POINT ( 'NONE',  ( -10.81189881249999907, -6.242252689847864744, -129.4687500020483810 ) ) ;
#38591=CARTESIAN_POINT ( 'NONE',  ( 10.81189881249999729, 0.000000000000000000, -119.8437500020483810 ) ) ;
#38595=CARTESIAN_POINT ( 'NONE',  ( -9.999999999999998224, 5.773502691896259087, -171.2500000040967905 ) ) ;
#38596=CARTESIAN_POINT ( 'NONE',  ( -2.293366432827344421E-15, -12.48450537969573659, -171.4062500020484379 ) ) ;
#38597=CARTESIAN_POINT ( 'NONE',  ( 9.999999999999998224, 0.000000000000000000, -132.8750000040967905 ) ) ;
#38600=CARTESIAN_POINT ( 'NONE',  ( -10.81189881249999729, -6.242252689847864744, -45.46875000204837391 ) ) ;
#38601=VECTOR ( 'NONE', #13912, 1000.000000000000000 ) ;
#38603=CARTESIAN_POINT ( 'NONE',  ( -10.00000000000102496, 5.773502691895664007, -85.75000000409671941 ) ) ;
#38607=CARTESIAN_POINT ( 'NONE',  ( 4.999999999999992006, -8.660254037844389075, -87.74999999999998579 ) ) ;
#38609=CARTESIAN_POINT ( 'NONE',  ( 9.999999999999998224, 0.000000000000000000, -99.87500000409679046 ) ) ;
#38610=EDGE_CURVE ( 'NONE', #3867, #5197, #14775, .T. ) ;
#38613=CARTESIAN_POINT ( 'NONE',  ( -10.81189881249999729, 1.324075727343319199E-15, -87.78125000204838102 ) ) ;
#38614=ORIENTED_EDGE ( 'NONE', *, *, #37259, .F. ) ;
#38616=CARTESIAN_POINT ( 'NONE',  ( 9.999999999998969713, 5.773502691896851502, -4.874999999999934275 ) ) ;
#38617=CARTESIAN_POINT ( 'NONE',  ( -10.81189881249999729, 1.324075727343319199E-15, -159.7812500020484094 ) ) ;
#38619=ORIENTED_EDGE ( 'NONE', *, *, #19334, .T. ) ;
#38620=EDGE_CURVE ( 'NONE', #34021, #35538, #26153, .T. ) ;
#38621=CARTESIAN_POINT ( 'NONE',  ( 7.070501591499377789E-16, 11.54700538379251284, -13.62499999999996803 ) ) ;
#38622=CARTESIAN_POINT ( 'NONE',  ( 7.644554776091147741E-16, 12.48450537969573659, -25.15625000204838813 ) ) ;
#38623=CARTESIAN_POINT ( 'NONE',  ( 10.00000000000000000, 5.773502691896255534, -150.3750000000000000 ) ) ;
#38624=ADVANCED_FACE ( 'NONE', ( #5932 ), #15825, .T. ) ;
#38626=CARTESIAN_POINT ( 'NONE',  ( -9.999999999999998224, 1.224646799147353059E-15, -197.7500000000000000 ) ) ;
#38627=CARTESIAN_POINT ( 'NONE',  ( 5.405949406249999534, 9.363379034771803333, -127.2812500020483810 ) ) ;
#38628=VERTEX_POINT ( 'NONE', #29022 ) ;
#38629=CARTESIAN_POINT ( 'NONE',  ( 7.070501591499376803E-16, 11.54700538379251284, -65.00000000409677625 ) ) ;
#38630=EDGE_CURVE ( 'NONE', #1539, #16629, #11760, .T. ) ;
#38632=( BOUNDED_CURVE ( )  B_SPLINE_CURVE ( 2, ( #21414, #35028, #28124, #40607, #5457, #31579, #18607 ),
 .UNSPECIFIED., .F., .F. ) 
 B_SPLINE_CURVE_WITH_KNOTS ( ( 3, 2, 2, 3 ),
 ( 0.9738805970149255753, 0.9751243781094529606, 0.9763681592039802348, 0.9776119402985076201 ),
 .UNSPECIFIED. ) 
 CURVE ( )  GEOMETRIC_REPRESENTATION_ITEM ( )  RATIONAL_B_SPLINE_CURVE ( ( 0.9999999999999761302, 0.8660254037844625774, 1.000000000000000000, 0.8660254037844387076, 1.000000000000000000, 0.8660254037844267172, 1.000000000000011990 ) ) 
 REPRESENTATION_ITEM ( '' )  );
#38633=CARTESIAN_POINT ( 'NONE',  ( -5.405949406250003975, -9.363379034771801557, -51.53125000204835970 ) ) ;
#38636=CARTESIAN_POINT ( 'NONE',  ( 7.644554776091147741E-16, 12.48450537969573659, -104.4687500020483668 ) ) ;
#38637=ORIENTED_EDGE ( 'NONE', *, *, #33743, .F. ) ;
#38640=CARTESIAN_POINT ( 'NONE',  ( -9.999999999999982236, -5.773502691896262640, -198.0000000040968473 ) ) ;
#38641=CARTESIAN_POINT ( 'NONE',  ( -10.81189881249999729, 1.324075727343319199E-15, -156.5937500020483810 ) ) ;
#38642=EDGE_CURVE ( 'NONE', #4750, #27209, #6557, .T. ) ;
#38643=( BOUNDED_CURVE ( )  B_SPLINE_CURVE ( 2, ( #19285, #42369, #32684, #29868, #22752, #12801, #309 ),
 .UNSPECIFIED., .F., .F. ) 
 B_SPLINE_CURVE_WITH_KNOTS ( ( 3, 2, 2, 3 ),
 ( 0.4925373134328359104, 0.4937810945273632957, 0.4950248756218906809, 0.4962686567164180107 ),
 .UNSPECIFIED. ) 
 CURVE ( )  GEOMETRIC_REPRESENTATION_ITEM ( )  RATIONAL_B_SPLINE_CURVE ( ( 0.9999999999999880096, 0.8660254037844506980, 1.000000000000000000, 0.8660254037844387076, 1.000000000000000000, 0.8660254037844267172, 1.000000000000011990 ) ) 
 REPRESENTATION_ITEM ( '' )  );
#38645=CARTESIAN_POINT ( 'NONE',  ( -5.405949406249996869, 9.363379034771805109, -3.843750002048368586 ) ) ;
#38646=CARTESIAN_POINT ( 'NONE',  ( 10.81189881249999551, -6.242252689847874514, -139.4687500020483810 ) ) ;
#38648=DIRECTION ( 'NONE',  ( -0.08682659386424779191, -0.08682659386424779191, 0.9924325091389669673 ) ) ;
#38650=CARTESIAN_POINT ( 'NONE',  ( 10.00000000000000000, 5.773502691896255534, -195.7500000040968189 ) ) ;
#38652=CARTESIAN_POINT ( 'NONE',  ( 10.81189881249999551, -6.242252689847874514, -198.1562500020484379 ) ) ;
#38653=DIRECTION ( 'NONE',  ( 1.000000000000000000, 0.000000000000000000, 0.000000000000000000 ) ) ;
#38656=CARTESIAN_POINT ( 'NONE',  ( 10.81189881249999551, -6.242252689847874514, -71.96875000204836681 ) ) ;
#38657=CARTESIAN_POINT ( 'NONE',  ( -10.81189881249999729, 1.324075727343319199E-15, -56.09375000204835970 ) ) ;
#38659=CARTESIAN_POINT ( 'NONE',  ( 7.644554776091147741E-16, 12.48450537969573659, -28.15625000204838457 ) ) ;
#38663=CARTESIAN_POINT ( 'NONE',  ( 10.00000000000000000, 5.773502691896255534, -111.3749999999999858 ) ) ;
#38667=CARTESIAN_POINT ( 'NONE',  ( -10.81189881249999729, 1.324075727343319199E-15, -8.281250002048350822 ) ) ;
#38668=EDGE_CURVE ( 'NONE', #22389, #2291, #39617, .T. ) ;
#38669=ORIENTED_EDGE ( 'NONE', *, *, #40135, .F. ) ;
#38670=CARTESIAN_POINT ( 'NONE',  ( 7.071067811865472841, -7.071067811865472841, -200.0000000000000000 ) ) ;
#38674=CARTESIAN_POINT ( 'NONE',  ( -9.999999999999998224, 1.224646799147353059E-15, -38.74999999999997868 ) ) ;
#38676=CARTESIAN_POINT ( 'NONE',  ( 10.00000000000000000, 5.773502691896255534, -24.75000000409676559 ) ) ;
#38677=CARTESIAN_POINT ( 'NONE',  ( 10.81189881249999729, 6.242252689847867408, -55.40625000204837391 ) ) ;
#38680=CARTESIAN_POINT ( 'NONE',  ( 10.00000000000051159, -5.773502691895965988, -105.6249999999999858 ) ) ;
#38681=CARTESIAN_POINT ( 'NONE',  ( 5.405949406249999534, 9.363379034771803333, -146.7812500020483810 ) ) ;
#38682=CARTESIAN_POINT ( 'NONE',  ( 10.81189881249999551, -6.242252689847874514, -150.1562500020484094 ) ) ;
#38683=CARTESIAN_POINT ( 'NONE',  ( -9.999999999999998224, 1.224646799147353059E-15, -78.12500000409677625 ) ) ;
#38684=CARTESIAN_POINT ( 'NONE',  ( -9.999999999999998224, 1.224646799147353059E-15, -58.24999999999997158 ) ) ;
#38686=ORIENTED_EDGE ( 'NONE', *, *, #18971, .F. ) ;
#38687=VERTEX_POINT ( 'NONE', #3325 ) ;
#38688=VECTOR ( 'NONE', #6979, 1000.000000000000000 ) ;
#38689=DIRECTION ( 'NONE',  ( -0.000000000000000000, -0.000000000000000000, 1.000000000000000000 ) ) ;
#38690=CARTESIAN_POINT ( 'NONE',  ( -5.405949406250003975, -9.363379034771801557, -184.8437500020483810 ) ) ;
#38692=CARTESIAN_POINT ( 'NONE',  ( -10.81189881249999729, 6.242252689847871849, -29.21875000204835615 ) ) ;
#38693=CARTESIAN_POINT ( 'NONE',  ( 0.000000000000000000, 0.000000000000000000, -200.0000000000000000 ) ) ;
#38694=CARTESIAN_POINT ( 'NONE',  ( 10.81189881249999551, -6.242252689847874514, -161.9687500020484094 ) ) ;
#38695=CARTESIAN_POINT ( 'NONE',  ( -10.81189881249999729, 1.324075727343319199E-15, -152.0937500020483810 ) ) ;
#38696=CARTESIAN_POINT ( 'NONE',  ( 10.82102786788851212, -1.350150063679357304, 1.152242674263551442E-14 ) ) ;
#38699=CARTESIAN_POINT ( 'NONE',  ( -10.81189881249999907, -6.242252689847864744, -16.96875000204836681 ) ) ;
#38702=CARTESIAN_POINT ( 'NONE',  ( -9.999999999999998224, 1.224646799147353059E-15, -10.62500000409674605 ) ) ;
#38705=CARTESIAN_POINT ( 'NONE',  ( 7.644554776091147741E-16, 12.48450537969573659, -83.46875000204838102 ) ) ;
#38707=CARTESIAN_POINT ( 'NONE',  ( 10.81189881249999907, 6.242252689847868297, -52.40625000204838813 ) ) ;
#38709=CARTESIAN_POINT ( 'NONE',  ( -9.999999999999998224, 1.224646799147353059E-15, -16.62500000409675138 ) ) ;
#38711=CARTESIAN_POINT ( 'NONE',  ( 7.070501591499377789E-16, 11.54700538379251284, -139.6250000000000000 ) ) ;
#38712=CARTESIAN_POINT ( 'NONE',  ( -5.405949406249996869, 9.363379034771805109, -146.5312500020483810 ) ) ;
#38713=( BOUNDED_CURVE ( )  B_SPLINE_CURVE ( 2, ( #36062, #35856, #16605, #42308, #32831, #2838, #12730 ),
 .UNSPECIFIED., .F., .F. ) 
 B_SPLINE_CURVE_WITH_KNOTS ( ( 3, 2, 2, 3 ),
 ( 0.1791044776119403437, 0.1803482587064677289, 0.1815920398009950587, 0.1828358208955224162 ),
 .UNSPECIFIED. ) 
 CURVE ( )  GEOMETRIC_REPRESENTATION_ITEM ( )  RATIONAL_B_SPLINE_CURVE ( ( 0.9999999999999940048, 0.8660254037844447028, 1.000000000000000000, 0.8660254037844387076, 1.000000000000000000, 0.8660254037844357100, 1.000000000000003109 ) ) 
 REPRESENTATION_ITEM ( '' )  );
#38714=CYLINDRICAL_SURFACE ( 'NONE', #10995, 9.999999999999998224 ) ;
#38716=CARTESIAN_POINT ( 'NONE',  ( -9.999999999999998224, 5.773502691896259087, -121.7500000040967905 ) ) ;
#38718=ORIENTED_EDGE ( 'NONE', *, *, #42040, .T. ) ;
#38721=CYLINDRICAL_SURFACE ( 'NONE', #27743, 9.999999999999998224 ) ;
#38722=CARTESIAN_POINT ( 'NONE',  ( 10.81189881249999729, 0.000000000000000000, -169.5312500020484094 ) ) ;
#38723=CARTESIAN_POINT ( 'NONE',  ( -4.999999999999996447, 8.660254037844387298, -48.37500000409677625 ) ) ;
#38726=EDGE_CURVE ( 'NONE', #12739, #41070, #7365, .T. ) ;
#38729=CARTESIAN_POINT ( 'NONE',  ( -10.81189881249999729, 6.242252689847871849, -171.9062500020484094 ) ) ;
#38730=CARTESIAN_POINT ( 'NONE',  ( -9.999999999999998224, 1.224646799147353059E-15, -7.249999999999978684 ) ) ;
#38731=DIRECTION ( 'NONE',  ( -0.000000000000000000, -0.000000000000000000, 1.000000000000000000 ) ) ;
#38732=ORIENTED_EDGE ( 'NONE', *, *, #8828, .F. ) ;
#38733=CYLINDRICAL_SURFACE ( 'NONE', #5914, 9.999999999999998224 ) ;
#38734=CARTESIAN_POINT ( 'NONE',  ( -4.999999999999996447, 8.660254037844387298, -26.99999999999996803 ) ) ;
#38735=CARTESIAN_POINT ( 'NONE',  ( 7.644554776091147741E-16, 12.48450537969573659, -80.65625000204839523 ) ) ;
#38736=VERTEX_POINT ( 'NONE', #17099 ) ;
#38739=ORIENTED_EDGE ( 'NONE', *, *, #25430, .T. ) ;
#38740=VERTEX_POINT ( 'NONE', #26626 ) ;
#38741=CARTESIAN_POINT ( 'NONE',  ( -2.293366432827344421E-15, -12.48450537969573659, -28.71875000204835615 ) ) ;
#38743=CARTESIAN_POINT ( 'NONE',  ( -5.405949406250003975, -9.363379034771801557, -8.031250002048350822 ) ) ;
#38744=CARTESIAN_POINT ( 'NONE',  ( -10.81189881249999907, -6.242252689847864744, -54.46875000204838102 ) ) ;
#38746=FACE_OUTER_BOUND ( 'NONE', #6128, .T. ) ;
#38748=CARTESIAN_POINT ( 'NONE',  ( 10.81189881249999551, -6.242252689847874514, -188.9687500020484094 ) ) ;
#38749=CARTESIAN_POINT ( 'NONE',  ( 10.81189881249999551, -6.242252689847874514, -173.9687500020484094 ) ) ;
#38751=AXIS2_PLACEMENT_3D ( 'NONE', #30790, #4661, #4024 ) ;
#38752=( BOUNDED_CURVE ( )  B_SPLINE_CURVE ( 2, ( #18804, #21183, #31781, #25302, #38446, #31992, #34373 ),
 .UNSPECIFIED., .F., .F. ) 
 B_SPLINE_CURVE_WITH_KNOTS ( ( 3, 2, 2, 3 ),
 ( 0.8283582089552240513, 0.8296019900497514366, 0.8308457711442787108, 0.8320895522388060961 ),
 .UNSPECIFIED. ) 
 CURVE ( )  GEOMETRIC_REPRESENTATION_ITEM ( )  RATIONAL_B_SPLINE_CURVE ( ( 0.9999999999999761302, 0.8660254037844625774, 1.000000000000000000, 0.8660254037844387076, 1.000000000000000000, 0.8660254037844267172, 1.000000000000011990 ) ) 
 REPRESENTATION_ITEM ( '' )  );
#38754=ADVANCED_FACE ( 'NONE', ( #22753 ), #13009, .T. ) ;
#38755=CARTESIAN_POINT ( 'NONE',  ( 5.000000000000000000, 8.660254037844385522, -41.12500000409677625 ) ) ;
#38758=CARTESIAN_POINT ( 'NONE',  ( -10.81189881249999907, -6.242252689847864744, -103.9687500020483668 ) ) ;
#38759=CARTESIAN_POINT ( 'NONE',  ( -9.999999999999998224, 1.224646799147353059E-15, -200.0000000000000000 ) ) ;
#38760=CARTESIAN_POINT ( 'NONE',  ( -10.81189881249999729, 1.324075727343319199E-15, -72.78125000204838102 ) ) ;
#38761=CARTESIAN_POINT ( 'NONE',  ( 5.405949406249999534, 9.363379034771803333, -95.59375000204838102 ) ) ;
#38763=CARTESIAN_POINT ( 'NONE',  ( 9.999999999999996447, -5.773502691896262640, -148.0000000040968189 ) ) ;
#38765=ORIENTED_EDGE ( 'NONE', *, *, #34438, .T. ) ;
#38768=VECTOR ( 'NONE', #14708, 1000.000000000000000 ) ;
#38769=DIRECTION ( 'NONE',  ( 1.000000000000000000, 0.000000000000000000, 0.000000000000000000 ) ) ;
#38772=VERTEX_POINT ( 'NONE', #26413 ) ;
#38773=CARTESIAN_POINT ( 'NONE',  ( 10.00000000000000000, 5.773502691896255534, -69.37499999999998579 ) ) ;
#38775=CARTESIAN_POINT ( 'NONE',  ( 5.000000000000000000, 8.660254037844385522, -74.12500000409677625 ) ) ;
#38776=CARTESIAN_POINT ( 'NONE',  ( -9.999999999999998224, 1.224646799147353059E-15, -122.7500000000000000 ) ) ;
#38777=CARTESIAN_POINT ( 'NONE',  ( -4.999999999999996447, 8.660254037844387298, -12.37500000409674783 ) ) ;
#38779=CARTESIAN_POINT ( 'NONE',  ( -5.405949406250003975, -9.363379034771801557, -69.53125000204838102 ) ) ;
#38781=CARTESIAN_POINT ( 'NONE',  ( -4.999999999999996447, 8.660254037844387298, -93.37500000409677625 ) ) ;
#38783=CARTESIAN_POINT ( 'NONE',  ( -9.999999999999998224, 1.224646799147353059E-15, -46.62500000409677625 ) ) ;
#38784=CARTESIAN_POINT ( 'NONE',  ( -5.405949406249996869, 9.363379034771805109, -190.0312500020484094 ) ) ;
#38786=EDGE_CURVE ( 'NONE', #2188, #35877, #24783, .T. ) ;
#38787=CARTESIAN_POINT ( 'NONE',  ( 5.405949406249992428, -9.363379034771808662, -4.593750002048368586 ) ) ;
#38788=CYLINDRICAL_SURFACE ( 'NONE', #14490, 9.999999999999998224 ) ;
#38790=CARTESIAN_POINT ( 'NONE',  ( -9.999999999999998224, 1.224646799147353059E-15, -200.0000000000000000 ) ) ;
#38791=CARTESIAN_POINT ( 'NONE',  ( 5.000000000000000000, 8.660254037844385522, -171.2500000000000000 ) ) ;
#38792=DIRECTION ( 'NONE',  ( -0.000000000000000000, -0.000000000000000000, 1.000000000000000000 ) ) ;
#38793=CARTESIAN_POINT ( 'NONE',  ( 5.405949406249999534, 9.363379034771803333, -98.78125000204839523 ) ) ;
#38794=ORIENTED_EDGE ( 'NONE', *, *, #22573, .T. ) ;
#38795=CARTESIAN_POINT ( 'NONE',  ( 9.999999999998969713, 5.773502691896851502, -37.87499999999992895 ) ) ;
#38797=EDGE_LOOP ( 'NONE', ( #28778, #27196, #23668, #20091 ) ) ;
#38798=CARTESIAN_POINT ( 'NONE',  ( -2.293366432827344421E-15, -12.48450537969573659, -30.40625000204834905 ) ) ;
#38800=CARTESIAN_POINT ( 'NONE',  ( -5.405949406250003975, -9.363379034771801557, -78.34375000204838102 ) ) ;
#38804=LINE ( 'NONE', #19365, #39106 ) ;
#38806=CARTESIAN_POINT ( 'NONE',  ( -5.000000000000003553, -8.660254037844383745, -7.375000004096743389 ) ) ;
#38807=CARTESIAN_POINT ( 'NONE',  ( -9.999999999999998224, 1.224646799147353059E-15, -150.1250000040967905 ) ) ;
#38808=CARTESIAN_POINT ( 'NONE',  ( 5.405949406249999534, 9.363379034771803333, -133.0937500020483810 ) ) ;
#38809=CARTESIAN_POINT ( 'NONE',  ( 10.81189881249999729, 6.242252689847867408, -113.7187500020483952 ) ) ;
#38812=CARTESIAN_POINT ( 'NONE',  ( -9.999999999999998224, 1.224646799147353059E-15, -166.6250000040967905 ) ) ;
#38813=CARTESIAN_POINT ( 'NONE',  ( -9.999999999999998224, 1.224646799147353059E-15, -133.6250000040967620 ) ) ;
#38816=CARTESIAN_POINT ( 'NONE',  ( 5.405949406249999534, 9.363379034771803333, -47.59375000204838102 ) ) ;
#38818=CARTESIAN_POINT ( 'NONE',  ( -10.81189881249999907, -6.242252689847864744, -0.6562500020483670315 ) ) ;
#38821=CARTESIAN_POINT ( 'NONE',  ( 5.000000000000000000, 8.660254037844385522, -91.74999999999998579 ) ) ;
#38823=CARTESIAN_POINT ( 'NONE',  ( -10.00000000000000000, -5.773502691896251982, -94.50000000409677625 ) ) ;
#38824=CARTESIAN_POINT ( 'NONE',  ( -9.999999999999998224, 1.224646799147353059E-15, -94.24999999999998579 ) ) ;
#38826=CARTESIAN_POINT ( 'NONE',  ( -10.81189881249999729, -6.242252689847864744, -90.65625000204836681 ) ) ;
#38832=CARTESIAN_POINT ( 'NONE',  ( 4.999999999999992006, -8.660254037844389075, -15.74999999999995914 ) ) ;
#38834=CARTESIAN_POINT ( 'NONE',  ( -5.405949406250003975, -9.363379034771801557, -23.03125000204836326 ) ) ;
#38835=CARTESIAN_POINT ( 'NONE',  ( -10.00000000000000000, -5.773502691896251982, -149.6250000000000284 ) ) ;
#38838=CARTESIAN_POINT ( 'NONE',  ( 10.00000000000000000, 5.773502691896255534, -195.3750000000000284 ) ) ;
#38839=CARTESIAN_POINT ( 'NONE',  ( -5.405949406250003975, -9.363379034771801557, -123.5312500020483952 ) ) ;
#38841=CARTESIAN_POINT ( 'NONE',  ( -9.999999999999998224, 1.224646799147353059E-15, -89.74999999999998579 ) ) ;
#38842=( BOUNDED_CURVE ( )  B_SPLINE_CURVE ( 2, ( #4867, #31419, #14117, #1857, #14983, #10684, #23878 ),
 .UNSPECIFIED., .F., .F. ) 
 B_SPLINE_CURVE_WITH_KNOTS ( ( 3, 2, 2, 3 ),
 ( 0.2276119402985075368, 0.2288557213930349221, 0.2300995024875622796, 0.2313432835820896372 ),
 .UNSPECIFIED. ) 
 CURVE ( )  GEOMETRIC_REPRESENTATION_ITEM ( )  RATIONAL_B_SPLINE_CURVE ( ( 0.9999999999999910072, 0.8660254037844477004, 1.000000000000000000, 0.8660254037844387076, 1.000000000000000000, 0.8660254037844297148, 1.000000000000008882 ) ) 
 REPRESENTATION_ITEM ( '' )  );
#38843=VERTEX_POINT ( 'NONE', #39774 ) ;
#38844=CARTESIAN_POINT ( 'NONE',  ( -10.81189881249999729, 1.324075727343319199E-15, -53.28125000204836681 ) ) ;
#38846=CARTESIAN_POINT ( 'NONE',  ( -5.405949406250003975, -9.363379034771801557, -102.3437500020483810 ) ) ;
#38847=ORIENTED_EDGE ( 'NONE', *, *, #25204, .F. ) ;
#38848=ORIENTED_EDGE ( 'NONE', *, *, #23044, .F. ) ;
#38850=CYLINDRICAL_SURFACE ( 'NONE', #3551, 9.999999999999998224 ) ;
#38851=CARTESIAN_POINT ( 'NONE',  ( 10.81189881249999907, 6.242252689847868297, -148.2187500020484094 ) ) ;
#38853=CARTESIAN_POINT ( 'NONE',  ( -5.405949406249996869, 9.363379034771805109, -9.843750002048345493 ) ) ;
#38854=CARTESIAN_POINT ( 'NONE',  ( 9.999999999999742428, 5.773502691896404748, -139.8749999999999716 ) ) ;
#38855=EDGE_CURVE ( 'NONE', #27592, #12865, #42380, .T. ) ;
#38856=CARTESIAN_POINT ( 'NONE',  ( 10.81189881249999729, 0.000000000000000000, -139.3437500020484094 ) ) ;
#38859=CARTESIAN_POINT ( 'NONE',  ( -9.999999999999998224, 5.773502691896259087, -195.2500000040967905 ) ) ;
#38861=CARTESIAN_POINT ( 'NONE',  ( -10.81189881249999729, -6.242252689847864744, -183.6562500020484094 ) ) ;
#38865=CARTESIAN_POINT ( 'NONE',  ( -10.81189881249999729, 1.324075727343319199E-15, -68.09375000204836681 ) ) ;
#38866=CARTESIAN_POINT ( 'NONE',  ( -2.293366432827344421E-15, -12.48450537969573659, -45.21875000204836681 ) ) ;
#38868=CARTESIAN_POINT ( 'NONE',  ( -5.405949406250003975, -9.363379034771801557, -23.03125000204836326 ) ) ;
#38872=CARTESIAN_POINT ( 'NONE',  ( 5.000000000000000000, 8.660254037844385522, -114.2499999999999858 ) ) ;
#38876=CARTESIAN_POINT ( 'NONE',  ( 10.81189881249999551, -6.242252689847874514, -114.1562500020483952 ) ) ;
#38877=( BOUNDED_CURVE ( )  B_SPLINE_CURVE ( 2, ( #36178, #371, #999, #40044, #4014, #20198, #27106 ),
 .UNSPECIFIED., .F., .F. ) 
 B_SPLINE_CURVE_WITH_KNOTS ( ( 3, 2, 2, 3 ),
 ( 0.3843283582089552786, 0.3855721393034826638, 0.3868159203980099936, 0.3880597014925373789 ),
 .UNSPECIFIED. ) 
 CURVE ( )  GEOMETRIC_REPRESENTATION_ITEM ( )  RATIONAL_B_SPLINE_CURVE ( ( 0.9999999999999940048, 0.8660254037844447028, 1.000000000000000000, 0.8660254037844387076, 1.000000000000000000, 0.8660254037844327124, 1.000000000000005995 ) ) 
 REPRESENTATION_ITEM ( '' )  );
#38878=ORIENTED_EDGE ( 'NONE', *, *, #5501, .T. ) ;
#38881=CARTESIAN_POINT ( 'NONE',  ( -5.000000000000003553, -8.660254037844383745, -86.87500000409677625 ) ) ;
#38883=CARTESIAN_POINT ( 'NONE',  ( 7.070501591499377789E-16, 11.54700538379251284, -37.62499999999995737 ) ) ;
#38884=CARTESIAN_POINT ( 'NONE',  ( -5.000000000000003553, -8.660254037844383745, -29.87500000409676204 ) ) ;
#38885=EDGE_CURVE ( 'NONE', #5998, #17896, #1588, .T. ) ;
#38886=CARTESIAN_POINT ( 'NONE',  ( 10.81189881249999551, -6.242252689847874514, -42.15625000204838102 ) ) ;
#38889=EDGE_CURVE ( 'NONE', #16629, #38687, #10840, .T. ) ;
#38892=CARTESIAN_POINT ( 'NONE',  ( 10.81189881249999551, -6.242252689847874514, -133.6562500020483810 ) ) ;
#38893=EDGE_CURVE ( 'NONE', #7682, #6043, #39873, .T. ) ;
#38894=CARTESIAN_POINT ( 'NONE',  ( 10.81189881249999551, -6.242252689847874514, -151.6562500020484094 ) ) ;
#38895=CARTESIAN_POINT ( 'NONE',  ( 9.999999999999998224, 0.000000000000000000, -60.49999999999997158 ) ) ;
#38903=CARTESIAN_POINT ( 'NONE',  ( 10.81189881249999907, 6.242252689847868297, -170.7187500020483810 ) ) ;
#38904=CARTESIAN_POINT ( 'NONE',  ( 10.81189881249999729, 0.000000000000000000, -29.84375000204836326 ) ) ;
#38905=CARTESIAN_POINT ( 'NONE',  ( 9.999999999999998224, 0.000000000000000000, -200.0000000000000000 ) ) ;
#38906=CARTESIAN_POINT ( 'NONE',  ( -10.81189881249999729, -6.242252689847864744, -165.4687500020483526 ) ) ;
#38907=CARTESIAN_POINT ( 'NONE',  ( 10.81189881249999729, 0.000000000000000000, -142.3437500020483810 ) ) ;
#38911=CARTESIAN_POINT ( 'NONE',  ( -5.405949406249996869, 9.363379034771805109, -17.34375000204835260 ) ) ;
#38913=CARTESIAN_POINT ( 'NONE',  ( 9.999999999999742428, 5.773502691896404748, -129.3750000000000000 ) ) ;
#38914=CARTESIAN_POINT ( 'NONE',  ( 9.999999999999479527, 5.773502691896553074, -120.3749999999999716 ) ) ;
#38916=CARTESIAN_POINT ( 'NONE',  ( 5.405949406249999534, 9.363379034771803333, -82.09375000204836681 ) ) ;
#38917=CARTESIAN_POINT ( 'NONE',  ( 10.81189881249999729, 0.000000000000000000, -49.53125000204838813 ) ) ;
#38921=CARTESIAN_POINT ( 'NONE',  ( -9.999999999999998224, 5.773502691896259087, -139.3750000000000000 ) ) ;
#38922=CARTESIAN_POINT ( 'NONE',  ( -5.405949406250003975, -9.363379034771801557, -149.0312500020483810 ) ) ;
#38923=CARTESIAN_POINT ( 'NONE',  ( -5.000000000000003553, -8.660254037844383745, -23.87500000409675849 ) ) ;
#38924=CARTESIAN_POINT ( 'NONE',  ( -4.999999999999996447, 8.660254037844387298, -121.8750000040967905 ) ) ;
#38926=EDGE_LOOP ( 'NONE', ( #40431, #9693, #24686, #949 ) ) ;
#38930=CARTESIAN_POINT ( 'NONE',  ( -10.81189881249999729, 1.324075727343319199E-15, -174.7812500020484094 ) ) ;
#38931=CARTESIAN_POINT ( 'NONE',  ( -5.000000000000003553, -8.660254037844383745, -50.87500000409675494 ) ) ;
#38932=LINE ( 'NONE', #2687, #6989 ) ;
#38934=AXIS2_PLACEMENT_3D ( 'NONE', #33211, #10514, #23701 ) ;
#38935=FACE_OUTER_BOUND ( 'NONE', #34971, .T. ) ;
#38936=CARTESIAN_POINT ( 'NONE',  ( -5.405949406250003975, -9.363379034771801557, -171.5312500020484094 ) ) ;
#38937=CARTESIAN_POINT ( 'NONE',  ( 10.81189881249999729, 0.000000000000000000, -142.3437500020483810 ) ) ;
#38938=CARTESIAN_POINT ( 'NONE',  ( 9.999999999999998224, 0.000000000000000000, -20.37500000409675494 ) ) ;
#38939=CARTESIAN_POINT ( 'NONE',  ( 9.999999999999998224, 0.000000000000000000, -80.37500000409677625 ) ) ;
#38940=VERTEX_POINT ( 'NONE', #943 ) ;
#38941=CARTESIAN_POINT ( 'NONE',  ( 4.999999999999992006, -8.660254037844389075, -194.2500000000000000 ) ) ;
#38943=CARTESIAN_POINT ( 'NONE',  ( 5.405949406249992428, -9.363379034771808662, -66.28125000204838102 ) ) ;
#38944=ORIENTED_EDGE ( 'NONE', *, *, #15445, .T. ) ;
#38946=CARTESIAN_POINT ( 'NONE',  ( 10.00000000000051159, -5.773502691895965988, -143.1250000000000000 ) ) ;
#38948=ORIENTED_EDGE ( 'NONE', *, *, #32830, .F. ) ;
#38949=CARTESIAN_POINT ( 'NONE',  ( -10.81189881249999729, 6.242252689847871849, -32.21875000204835970 ) ) ;
#38950=CYLINDRICAL_SURFACE ( 'NONE', #3162, 9.999999999999998224 ) ;
#38951=CARTESIAN_POINT ( 'NONE',  ( 5.405949406249992428, -9.363379034771808662, -4.781250002048375691 ) ) ;
#38952=CARTESIAN_POINT ( 'NONE',  ( -10.81189881249999729, 1.324075727343319199E-15, -51.59375000204835260 ) ) ;
#38953=EDGE_LOOP ( 'NONE', ( #14311, #20814, #20619, #13857 ) ) ;
#38954=CARTESIAN_POINT ( 'NONE',  ( -5.000000000000003553, -8.660254037844383745, -3.999999999999976019 ) ) ;
#38956=CARTESIAN_POINT ( 'NONE',  ( 7.644554776091147741E-16, 12.48450537969573659, -185.4687500020484094 ) ) ;
#38957=CARTESIAN_POINT ( 'NONE',  ( 7.644554776091147741E-16, 12.48450537969573659, -171.9687500020483810 ) ) ;
#38958=( BOUNDED_CURVE ( )  B_SPLINE_CURVE ( 2, ( #34466, #33822, #30586, #8350, #20633, #40471, #30375 ),
 .UNSPECIFIED., .F., .F. ) 
 B_SPLINE_CURVE_WITH_KNOTS ( ( 3, 2, 2, 3 ),
 ( 0.6343283582089553896, 0.6355721393034826638, 0.6368159203980100491, 0.6380597014925374344 ),
 .UNSPECIFIED. ) 
 CURVE ( )  GEOMETRIC_REPRESENTATION_ITEM ( )  RATIONAL_B_SPLINE_CURVE ( ( 0.9999999999999880096, 0.8660254037844506980, 1.000000000000000000, 0.8660254037844387076, 1.000000000000000000, 0.8660254037844267172, 1.000000000000011990 ) ) 
 REPRESENTATION_ITEM ( '' )  );
#38961=CARTESIAN_POINT ( 'NONE',  ( -10.00000000000154188, 5.773502691895366468, -18.25000000409673007 ) ) ;
#38962=CARTESIAN_POINT ( 'NONE',  ( -9.999999999999834799, -5.773502691896343464, -192.0000000040968189 ) ) ;
#38964=CARTESIAN_POINT ( 'NONE',  ( -2.293366432827344421E-15, -12.48450537969573659, -105.2187500020483952 ) ) ;
#38965=CARTESIAN_POINT ( 'NONE',  ( 5.405949406249999534, 9.363379034771803333, -74.78125000204838102 ) ) ;
#38966=CARTESIAN_POINT ( 'NONE',  ( 4.999999999999992006, -8.660254037844389075, -5.249999999999976907 ) ) ;
#38967=CARTESIAN_POINT ( 'NONE',  ( -10.81189881249999729, 6.242252689847871849, -87.71875000204836681 ) ) ;
#38969=CARTESIAN_POINT ( 'NONE',  ( -5.000000000000003553, -8.660254037844383745, -143.8750000040967905 ) ) ;
#38971=VERTEX_POINT ( 'NONE', #14498 ) ;
#38974=CARTESIAN_POINT ( 'NONE',  ( -10.81189881249999729, 6.242252689847871849, -194.4062500020484094 ) ) ;
#38975=CARTESIAN_POINT ( 'NONE',  ( 9.999999999999998224, 0.000000000000000000, -112.9999999999999858 ) ) ;
#38978=CARTESIAN_POINT ( 'NONE',  ( 7.070501591499377789E-16, 11.54700538379251284, -64.62499999999998579 ) ) ;
#38980=CARTESIAN_POINT ( 'NONE',  ( -2.121150477449813534E-15, -11.54700538379251284, -77.75000000409677625 ) ) ;
#38981=CARTESIAN_POINT ( 'NONE',  ( 9.999999999999479527, 5.773502691896553074, -102.3749999999999858 ) ) ;
#38984=CARTESIAN_POINT ( 'NONE',  ( -10.81189881249999729, 1.324075727343319199E-15, -66.78125000204838102 ) ) ;
#38987=ORIENTED_EDGE ( 'NONE', *, *, #23902, .F. ) ;
#38988=CARTESIAN_POINT ( 'NONE',  ( -10.81189881249999729, 1.324075727343319199E-15, -195.7812500020484094 ) ) ;
#38990=CARTESIAN_POINT ( 'NONE',  ( 10.81189881249999729, 0.000000000000000000, -4.343750002048368586 ) ) ;
#38994=CARTESIAN_POINT ( 'NONE',  ( 9.999999999999998224, 0.000000000000000000, -114.8750000040967905 ) ) ;
#38995=CARTESIAN_POINT ( 'NONE',  ( 7.070501591499377789E-16, 11.54700538379251284, -178.6250000000000000 ) ) ;
#38997=CARTESIAN_POINT ( 'NONE',  ( -5.405949406249996869, 9.363379034771805109, -104.5312500020483810 ) ) ;
#38998=EDGE_LOOP ( 'NONE', ( #5997, #11426, #27378, #42595 ) ) ;
#38999=CARTESIAN_POINT ( 'NONE',  ( -9.999999999999998224, 1.224646799147353059E-15, -37.24999999999997868 ) ) ;
#39000=ORIENTED_EDGE ( 'NONE', *, *, #41110, .T. ) ;
#39001=ORIENTED_EDGE ( 'NONE', *, *, #9860, .T. ) ;
#39002=( BOUNDED_CURVE ( )  B_SPLINE_CURVE ( 2, ( #40260, #10697, #23891, #4238, #7690, #14130, #37466 ),
 .UNSPECIFIED., .F., .F. ) 
 B_SPLINE_CURVE_WITH_KNOTS ( ( 3, 2, 2, 3 ),
 ( 0.1716417910447761430, 0.1728855721393035005, 0.1741293532338308858, 0.1753731343283582433 ),
 .UNSPECIFIED. ) 
 CURVE ( )  GEOMETRIC_REPRESENTATION_ITEM ( )  RATIONAL_B_SPLINE_CURVE ( ( 0.9999999999999970024, 0.8660254037844417052, 1.000000000000000000, 0.8660254037844387076, 1.000000000000000000, 0.8660254037844357100, 1.000000000000003109 ) ) 
 REPRESENTATION_ITEM ( '' )  );
#39003=CARTESIAN_POINT ( 'NONE',  ( -10.81189881249999729, 6.242252689847871849, -32.21875000204835970 ) ) ;
#39004=CARTESIAN_POINT ( 'NONE',  ( -10.81189881249999729, 1.324075727343319199E-15, -27.78125000204837036 ) ) ;
#39006=CARTESIAN_POINT ( 'NONE',  ( -5.405949406250003975, -9.363379034771801557, -82.84375000204836681 ) ) ;
#39007=CARTESIAN_POINT ( 'NONE',  ( -10.00000000000076916, 5.773502691895813221, -127.7500000040967763 ) ) ;
#39008=CARTESIAN_POINT ( 'NONE',  ( 5.405949406249992428, -9.363379034771808662, -198.0937500020484094 ) ) ;
#39009=EDGE_CURVE ( 'NONE', #10480, #39684, #21735, .T. ) ;
#39013=CARTESIAN_POINT ( 'NONE',  ( 4.999999999999992006, -8.660254037844389075, -14.62500000409674961 ) ) ;
#39015=CARTESIAN_POINT ( 'NONE',  ( -2.293366432827344421E-15, -12.48450537969573659, -126.2187500020483952 ) ) ;
#39016=CARTESIAN_POINT ( 'NONE',  ( 10.81189881249999551, -6.242252689847874514, -94.65625000204838102 ) ) ;
#39017=CARTESIAN_POINT ( 'NONE',  ( -10.81189881249999729, 1.324075727343319199E-15, -111.5937500020483810 ) ) ;
#39018=AXIS2_PLACEMENT_3D ( 'NONE', #29786, #13769, #6894 ) ;
#39021=CARTESIAN_POINT ( 'NONE',  ( 4.999999999999992006, -8.660254037844389075, -172.1250000040968189 ) ) ;
#39022=CYLINDRICAL_SURFACE ( 'NONE', #19251, 9.999999999999998224 ) ;
#39026=DIRECTION ( 'NONE',  ( 1.000000000000000000, 0.000000000000000000, 0.000000000000000000 ) ) ;
#39028=CARTESIAN_POINT ( 'NONE',  ( -2.121150477449813534E-15, -11.54700538379251284, -126.8749999999999858 ) ) ;
#39030=CARTESIAN_POINT ( 'NONE',  ( -9.999999999999998224, 1.224646799147353059E-15, -91.24999999999998579 ) ) ;
#39032=CARTESIAN_POINT ( 'NONE',  ( -2.121150477449813534E-15, -11.54700538379251284, -95.75000000409677625 ) ) ;
#39035=CARTESIAN_POINT ( 'NONE',  ( 7.644554776091147741E-16, 12.48450537969573659, -91.15625000204838102 ) ) ;
#39036=VERTEX_POINT ( 'NONE', #34179 ) ;
#39038=FACE_OUTER_BOUND ( 'NONE', #23008, .T. ) ;
#39040=VERTEX_POINT ( 'NONE', #34390 ) ;
#39041=CARTESIAN_POINT ( 'NONE',  ( 7.070501591499377789E-16, 11.54700538379251284, -19.62499999999997868 ) ) ;
#39042=CARTESIAN_POINT ( 'NONE',  ( 5.000000000000000000, 8.660254037844385522, -154.7500000000000000 ) ) ;
#39045=CARTESIAN_POINT ( 'NONE',  ( 5.405949406249992428, -9.363379034771808662, -126.2812500020483668 ) ) ;
#39046=ORIENTED_EDGE ( 'NONE', *, *, #31628, .T. ) ;
#39047=CARTESIAN_POINT ( 'NONE',  ( -5.000000000000003553, -8.660254037844383745, -12.99999999999995559 ) ) ;
#39048=ORIENTED_EDGE ( 'NONE', *, *, #15615, .T. ) ;
#39049=CARTESIAN_POINT ( 'NONE',  ( 10.81189881249999551, -6.242252689847874514, -57.15625000204837391 ) ) ;
#39051=CARTESIAN_POINT ( 'NONE',  ( -10.81189881249999729, 6.242252689847871849, -102.7187500020483810 ) ) ;
#39053=VERTEX_POINT ( 'NONE', #14716 ) ;
#39054=CYLINDRICAL_SURFACE ( 'NONE', #21801, 9.999999999999998224 ) ;
#39055=CARTESIAN_POINT ( 'NONE',  ( -2.121150477449813534E-15, -11.54700538379251284, -116.3749999999999858 ) ) ;
#39057=CARTESIAN_POINT ( 'NONE',  ( -9.999999999999868550, 5.773502691896333694, -175.3750000000000000 ) ) ;
#39058=DIRECTION ( 'NONE',  ( 0.5000000000000003331, -0.8660254037844383745, 0.000000000000000000 ) ) ;
#39059=EDGE_CURVE ( 'NONE', #20204, #5974, #39362, .T. ) ;
#39060=CARTESIAN_POINT ( 'NONE',  ( -10.81189881249999729, 1.324075727343319199E-15, -137.0937500020483810 ) ) ;
#39062=DIRECTION ( 'NONE',  ( -0.000000000000000000, -0.000000000000000000, 1.000000000000000000 ) ) ;
#39064=CARTESIAN_POINT ( 'NONE',  ( -4.999999999999996447, 8.660254037844387298, -196.8750000040967905 ) ) ;
#39066=CARTESIAN_POINT ( 'NONE',  ( -10.81189881249999729, 6.242252689847871849, -185.4062500020484094 ) ) ;
#39067=LINE ( 'NONE', #29362, #41271 ) ;
#39070=CARTESIAN_POINT ( 'NONE',  ( 10.81189881249999729, 0.000000000000000000, -70.34375000204836681 ) ) ;
#39071=CARTESIAN_POINT ( 'NONE',  ( 10.81189881249999729, 0.000000000000000000, -52.34375000204835260 ) ) ;
#39074=CARTESIAN_POINT ( 'NONE',  ( 10.81189881249999907, 6.242252689847868297, -25.40625000204838813 ) ) ;
#39078=CARTESIAN_POINT ( 'NONE',  ( 9.999999999999998224, 0.000000000000000000, -111.4999999999999858 ) ) ;
#39082=CARTESIAN_POINT ( 'NONE',  ( -5.405949406249996869, 9.363379034771805109, -116.5312500020483952 ) ) ;
#39089=CARTESIAN_POINT ( 'NONE',  ( -5.000000000000003553, -8.660254037844383745, -42.99999999999998579 ) ) ;
#39090=CARTESIAN_POINT ( 'NONE',  ( -2.121150477449813534E-15, -11.54700538379251284, -20.75000000409677980 ) ) ;
#39091=CARTESIAN_POINT ( 'NONE',  ( -10.81189881249999729, 1.324075727343319199E-15, -41.28125000204838102 ) ) ;
#39095=CARTESIAN_POINT ( 'NONE',  ( -9.999999999999998224, 1.224646799147353059E-15, -156.1250000040967905 ) ) ;
#39096=CARTESIAN_POINT ( 'NONE',  ( -5.405949406249996869, 9.363379034771805109, -136.0312500020484094 ) ) ;
#39097=CARTESIAN_POINT ( 'NONE',  ( -5.405949406250003975, -9.363379034771801557, -146.0312500020483810 ) ) ;
#39098=CARTESIAN_POINT ( 'NONE',  ( 9.999999999999998224, 0.000000000000000000, -109.9999999999999858 ) ) ;
#39103=CARTESIAN_POINT ( 'NONE',  ( -2.293366432827344421E-15, -12.48450537969573659, -171.2187500020484094 ) ) ;
#39104=CARTESIAN_POINT ( 'NONE',  ( -5.405949406249996869, 9.363379034771805109, -23.34375000204835970 ) ) ;
#39106=VECTOR ( 'NONE', #32551, 1000.000000000000000 ) ;
#39108=CARTESIAN_POINT ( 'NONE',  ( -2.293366432827344421E-15, -12.48450537969573659, -166.7187500020483810 ) ) ;
#39109=CARTESIAN_POINT ( 'NONE',  ( -10.81189881249999907, -6.242252689847864744, -142.9687500020484094 ) ) ;
#39110=EDGE_CURVE ( 'NONE', #11539, #3816, #5734, .T. ) ;
#39111=LINE ( 'NONE', #32234, #30053 ) ;
#39114=( BOUNDED_CURVE ( )  B_SPLINE_CURVE ( 2, ( #27161, #13754, #3868, #20461, #847, #16353, #30414 ),
 .UNSPECIFIED., .F., .F. ) 
 B_SPLINE_CURVE_WITH_KNOTS ( ( 3, 2, 2, 3 ),
 ( 0.8059701492537315604, 0.8072139303482589456, 0.8084577114427863309, 0.8097014925373136052 ),
 .UNSPECIFIED. ) 
 CURVE ( )  GEOMETRIC_REPRESENTATION_ITEM ( )  RATIONAL_B_SPLINE_CURVE ( ( 0.9999999999999761302, 0.8660254037844625774, 1.000000000000000000, 0.8660254037844387076, 1.000000000000000000, 0.8660254037844148378, 1.000000000000023981 ) ) 
 REPRESENTATION_ITEM ( '' )  );
#39115=CARTESIAN_POINT ( 'NONE',  ( -10.81189881249999729, 6.242252689847871849, -21.71875000204837036 ) ) ;
#39117=EDGE_CURVE ( 'NONE', #33917, #1371, #28046, .T. ) ;
#39121=CARTESIAN_POINT ( 'NONE',  ( -5.000000000000003553, -8.660254037844383745, -17.49999999999996092 ) ) ;
#39122=CARTESIAN_POINT ( 'NONE',  ( -10.81189881249999729, 6.242252689847871849, -75.71875000204836681 ) ) ;
#39123=CARTESIAN_POINT ( 'NONE',  ( -10.81189881249999729, 6.242252689847871849, -47.40625000204835970 ) ) ;
#39127=CARTESIAN_POINT ( 'NONE',  ( 9.999999999999996447, -5.773502691896262640, -140.1250000000000000 ) ) ;
#39128=CARTESIAN_POINT ( 'NONE',  ( 10.81189881249999729, 6.242252689847867408, -137.9062500020484094 ) ) ;
#39131=CARTESIAN_POINT ( 'NONE',  ( 9.999999999999998224, 0.000000000000000000, -110.3750000040967763 ) ) ;
#39133=ORIENTED_EDGE ( 'NONE', *, *, #20719, .T. ) ;
#39134=( BOUNDED_CURVE ( )  B_SPLINE_CURVE ( 2, ( #12735, #31789, #15768, #9310, #25310, #19025, #15560 ),
 .UNSPECIFIED., .F., .F. ) 
 B_SPLINE_CURVE_WITH_KNOTS ( ( 3, 2, 2, 3 ),
 ( 0.3880597014925373789, 0.3893034825870647087, 0.3905472636815920939, 0.3917910447761194792 ),
 .UNSPECIFIED. ) 
 CURVE ( )  GEOMETRIC_REPRESENTATION_ITEM ( )  RATIONAL_B_SPLINE_CURVE ( ( 0.9999999999999940048, 0.8660254037844447028, 1.000000000000000000, 0.8660254037844387076, 1.000000000000000000, 0.8660254037844327124, 1.000000000000005995 ) ) 
 REPRESENTATION_ITEM ( '' )  );
#39137=DIRECTION ( 'NONE',  ( 1.000000000000000000, 0.000000000000000000, 0.000000000000000000 ) ) ;
#39138=CARTESIAN_POINT ( 'NONE',  ( 10.81189881249999907, 6.242252689847868297, -169.4062500020484094 ) ) ;
#39139=CARTESIAN_POINT ( 'NONE',  ( -10.00000000000000000, -5.773502691896251982, -49.50000000409676915 ) ) ;
#39141=DIRECTION ( 'NONE',  ( -0.000000000000000000, -0.000000000000000000, 1.000000000000000000 ) ) ;
#39143=CARTESIAN_POINT ( 'NONE',  ( 9.999999999999998224, 0.000000000000000000, -200.0000000000000000 ) ) ;
#39144=CARTESIAN_POINT ( 'NONE',  ( -10.81189881249999729, 6.242252689847871849, -159.9062500020483810 ) ) ;
#39145=EDGE_CURVE ( 'NONE', #39053, #41888, #31584, .T. ) ;
#39146=CARTESIAN_POINT ( 'NONE',  ( 10.81189881249999907, 6.242252689847868297, -145.2187500020484094 ) ) ;
#39148=CYLINDRICAL_SURFACE ( 'NONE', #10470, 9.999999999999998224 ) ;
#39149=CARTESIAN_POINT ( 'NONE',  ( 0.000000000000000000, 0.000000000000000000, -200.0000000000000000 ) ) ;
#39150=ORIENTED_EDGE ( 'NONE', *, *, #37255, .F. ) ;
#39151=CARTESIAN_POINT ( 'NONE',  ( -9.999999999999998224, 1.224646799147353059E-15, -31.24999999999997158 ) ) ;
#39152=CARTESIAN_POINT ( 'NONE',  ( -10.81189881249999729, 1.324075727343319199E-15, -72.78125000204838102 ) ) ;
#39153=ORIENTED_EDGE ( 'NONE', *, *, #39350, .F. ) ;
#39154=CARTESIAN_POINT ( 'NONE',  ( -5.405949406249996869, 9.363379034771805109, -119.3437500020483810 ) ) ;
#39155=ORIENTED_EDGE ( 'NONE', *, *, #20669, .T. ) ;
#39156=EDGE_CURVE ( 'NONE', #7656, #34021, #5991, .T. ) ;
#39157=EDGE_LOOP ( 'NONE', ( #38718, #22859, #3384, #13207 ) ) ;
#39158=CARTESIAN_POINT ( 'NONE',  ( -5.405949406249996869, 9.363379034771805109, -27.84375000204836326 ) ) ;
#39159=CARTESIAN_POINT ( 'NONE',  ( -10.81189881249999729, 6.242252689847871849, -194.2187500020483810 ) ) ;
#39160=CARTESIAN_POINT ( 'NONE',  ( -10.81189881249999907, -6.242252689847864744, -58.96875000204836681 ) ) ;
#39163=CARTESIAN_POINT ( 'NONE',  ( -5.405949406249996869, 9.363379034771805109, -191.3437500020484094 ) ) ;
#39164=CARTESIAN_POINT ( 'NONE',  ( -10.81189881249999729, 6.242252689847871849, -171.7187500020483810 ) ) ;
#39170=CARTESIAN_POINT ( 'NONE',  ( 7.644554776091147741E-16, 12.48450537969573659, -98.46875000204839523 ) ) ;
#39171=CARTESIAN_POINT ( 'NONE',  ( -9.999999999999479527, -5.773502691896549521, -48.00000000409674783 ) ) ;
#39172=CARTESIAN_POINT ( 'NONE',  ( 10.81189881249999729, 0.000000000000000000, -75.03125000204838102 ) ) ;
#39175=CARTESIAN_POINT ( 'NONE',  ( 10.81189881249999729, 6.242252689847867408, -82.21875000204836681 ) ) ;
#39178=CARTESIAN_POINT ( 'NONE',  ( 4.999999999999992006, -8.660254037844389075, -145.1250000040967905 ) ) ;
#39184=DIRECTION ( 'NONE',  ( -0.000000000000000000, -0.000000000000000000, 1.000000000000000000 ) ) ;
#39188=CARTESIAN_POINT ( 'NONE',  ( 4.999999999999992006, -8.660254037844389075, -57.74999999999997158 ) ) ;
#39190=CARTESIAN_POINT ( 'NONE',  ( 9.999999999999998224, 0.000000000000000000, -71.37500000409677625 ) ) ;
#39191=CARTESIAN_POINT ( 'NONE',  ( 0.000000000000000000, 0.000000000000000000, -200.0000000000000000 ) ) ;
#39194=CARTESIAN_POINT ( 'NONE',  ( -5.405949406250003975, -9.363379034771801557, -71.03125000204838102 ) ) ;
#39197=CARTESIAN_POINT ( 'NONE',  ( -2.121150477449813534E-15, -11.54700538379251284, -151.2500000040968189 ) ) ;
#39198=CARTESIAN_POINT ( 'NONE',  ( 10.81189881249999907, 6.242252689847868297, -181.4062500020484379 ) ) ;
#39200=CARTESIAN_POINT ( 'NONE',  ( -9.999999999999998224, 1.224646799147353059E-15, -200.0000000000000000 ) ) ;
#39203=CARTESIAN_POINT ( 'NONE',  ( -2.121150477449813534E-15, -11.54700538379251284, -137.3750000000000000 ) ) ;
#39204=CARTESIAN_POINT ( 'NONE',  ( -10.00000000000000000, -5.773502691896251982, -176.6250000000000284 ) ) ;
#39205=CARTESIAN_POINT ( 'NONE',  ( -9.999999999999998224, 1.224646799147353059E-15, -97.24999999999998579 ) ) ;
#39206=CARTESIAN_POINT ( 'NONE',  ( 7.644554776091147741E-16, 12.48450537969573659, -94.15625000204839523 ) ) ;
#39207=ORIENTED_EDGE ( 'NONE', *, *, #26621, .F. ) ;
#39210=( BOUNDED_CURVE ( )  B_SPLINE_CURVE ( 2, ( #28839, #38962, #15004, #5529, #19108, #25598, #35103 ),
 .UNSPECIFIED., .F., .F. ) 
 B_SPLINE_CURVE_WITH_KNOTS ( ( 3, 2, 2, 3 ),
 ( 0.03358208955223884046, 0.03482587064676620492, 0.03606965174129356938, 0.03731343283582092690 ),
 .UNSPECIFIED. ) 
 CURVE ( )  GEOMETRIC_REPRESENTATION_ITEM ( )  RATIONAL_B_SPLINE_CURVE ( ( 0.9999999999999963363, 0.8660254037844424824, 1.000000000000000000, 0.8660254037844387076, 1.000000000000000000, 0.8660254037844349329, 1.000000000000003775 ) ) 
 REPRESENTATION_ITEM ( '' )  );
#39212=CARTESIAN_POINT ( 'NONE',  ( -10.81189881249999729, 1.324075727343319199E-15, -35.09375000204836681 ) ) ;
#39213=CARTESIAN_POINT ( 'NONE',  ( 10.81189881249999729, 0.000000000000000000, -18.03125000204835970 ) ) ;
#39215=CARTESIAN_POINT ( 'NONE',  ( -5.405949406249996869, 9.363379034771805109, -77.34375000204838102 ) ) ;
#39216=LINE ( 'NONE', #42654, #23607 ) ;
#39217=CARTESIAN_POINT ( 'NONE',  ( -2.293366432827344421E-15, -12.48450537969573659, -193.7187500020484094 ) ) ;
#39218=LINE ( 'NONE', #22191, #9518 ) ;
#39219=AXIS2_PLACEMENT_3D ( 'NONE', #42087, #19215, #35845 ) ;
#39220=CARTESIAN_POINT ( 'NONE',  ( 9.999999999999998224, 0.000000000000000000, -143.3750000040967905 ) ) ;
#39222=CARTESIAN_POINT ( 'NONE',  ( -4.999999999999996447, 8.660254037844387298, -0.3750000040967649273 ) ) ;
#39224=CARTESIAN_POINT ( 'NONE',  ( -2.293366432827344421E-15, -12.48450537969573659, -123.2187500020483952 ) ) ;
#39225=CARTESIAN_POINT ( 'NONE',  ( -10.81189881249999907, -6.242252689847864744, -101.1562500020483952 ) ) ;
#39226=CARTESIAN_POINT ( 'NONE',  ( -10.81189881249999729, 1.324075727343319199E-15, -105.5937500020483810 ) ) ;
#39229=CARTESIAN_POINT ( 'NONE',  ( 9.999999999999998224, 0.000000000000000000, -170.3750000040968189 ) ) ;
#39230=CARTESIAN_POINT ( 'NONE',  ( 9.999999999999998224, 0.000000000000000000, -81.87500000409676204 ) ) ;
#39236=CARTESIAN_POINT ( 'NONE',  ( 9.999999999999479527, 5.773502691896553074, -127.8749999999999858 ) ) ;
#39238=CARTESIAN_POINT ( 'NONE',  ( 9.999999999999996447, -5.773502691896262640, -81.62499999999998579 ) ) ;
#39240=CARTESIAN_POINT ( 'NONE',  ( 5.000000000000000000, 8.660254037844385522, -98.12500000409677625 ) ) ;
#39241=CARTESIAN_POINT ( 'NONE',  ( 0.000000000000000000, 0.000000000000000000, -200.0000000000000000 ) ) ;
#39243=CARTESIAN_POINT ( 'NONE',  ( 10.81189881249999729, 0.000000000000000000, -93.03125000204838102 ) ) ;
#39244=ORIENTED_EDGE ( 'NONE', *, *, #8166, .T. ) ;
#39248=ORIENTED_EDGE ( 'NONE', *, *, #25954, .T. ) ;
#39249=CARTESIAN_POINT ( 'NONE',  ( -9.999999999999998224, 1.224646799147353059E-15, -17.74999999999996092 ) ) ;
#39250=VECTOR ( 'NONE', #1367, 1000.000000000000000 ) ;
#39251=CARTESIAN_POINT ( 'NONE',  ( 9.999999999999998224, 0.000000000000000000, -143.0000000000000000 ) ) ;
#39253=EDGE_CURVE ( 'NONE', #17857, #33970, #4338, .T. ) ;
#39254=( BOUNDED_CURVE ( )  B_SPLINE_CURVE ( 2, ( #33401, #42656, #26487, #10492, #3190, #35992, #30158 ),
 .UNSPECIFIED., .F., .F. ) 
 B_SPLINE_CURVE_WITH_KNOTS ( ( 3, 2, 2, 3 ),
 ( 0.6268656716417911889, 0.6281094527363185742, 0.6293532338308458485, 0.6305970149253732338 ),
 .UNSPECIFIED. ) 
 CURVE ( )  GEOMETRIC_REPRESENTATION_ITEM ( )  RATIONAL_B_SPLINE_CURVE ( ( 0.9999999999999880096, 0.8660254037844506980, 1.000000000000000000, 0.8660254037844387076, 1.000000000000000000, 0.8660254037844267172, 1.000000000000011990 ) ) 
 REPRESENTATION_ITEM ( '' )  );
#39256=CARTESIAN_POINT ( 'NONE',  ( -5.000000000000003553, -8.660254037844383745, -197.5000000000000000 ) ) ;
#39257=CARTESIAN_POINT ( 'NONE',  ( -10.81189881249999907, -6.242252689847864744, -120.6562500020483810 ) ) ;
#39259=CARTESIAN_POINT ( 'NONE',  ( 5.000000000000000000, 8.660254037844385522, -65.12500000409676204 ) ) ;
#39260=ORIENTED_EDGE ( 'NONE', *, *, #8656, .T. ) ;
#39261=CARTESIAN_POINT ( 'NONE',  ( 10.81189881249999729, 0.000000000000000000, -52.53125000204835970 ) ) ;
#39263=CARTESIAN_POINT ( 'NONE',  ( 10.81189881249999551, -6.242252689847874514, -106.4687500020483810 ) ) ;
#39265=CARTESIAN_POINT ( 'NONE',  ( -2.121150477449813534E-15, -11.54700538379251284, -83.37499999999997158 ) ) ;
#39268=CARTESIAN_POINT ( 'NONE',  ( 5.405949406249999534, 9.363379034771803333, 0.4062499979516354109 ) ) ;
#39271=CARTESIAN_POINT ( 'NONE',  ( -10.81189881249999729, 6.242252689847871849, -134.2187500020483810 ) ) ;
#39273=FACE_OUTER_BOUND ( 'NONE', #22877, .T. ) ;
#39275=CARTESIAN_POINT ( 'NONE',  ( 5.000000000000000000, 8.660254037844385522, -197.1250000040967905 ) ) ;
#39277=CARTESIAN_POINT ( 'NONE',  ( 10.81189881249999729, 6.242252689847867408, -185.9062500020484094 ) ) ;
#39278=EDGE_CURVE ( 'NONE', #29829, #23935, #29429, .T. ) ;
#39279=CYLINDRICAL_SURFACE ( 'NONE', #30988, 9.999999999999998224 ) ;
#39282=CARTESIAN_POINT ( 'NONE',  ( 7.644554776091147741E-16, 12.48450537969573659, -63.96875000204838102 ) ) ;
#39283=CARTESIAN_POINT ( 'NONE',  ( -10.81189881249999729, 1.324075727343319199E-15, -50.09375000204835260 ) ) ;
#39285=CARTESIAN_POINT ( 'NONE',  ( -10.81189881249999729, 6.242252689847871849, -17.40625000204838457 ) ) ;
#39288=CARTESIAN_POINT ( 'NONE',  ( 5.000000000000000000, 8.660254037844385522, -102.2500000000000000 ) ) ;
#39289=DIRECTION ( 'NONE',  ( -0.000000000000000000, -0.000000000000000000, 1.000000000000000000 ) ) ;
#39292=CARTESIAN_POINT ( 'NONE',  ( -10.81189881249999729, 6.242252689847871849, -113.4062500020483952 ) ) ;
#39293=ORIENTED_EDGE ( 'NONE', *, *, #31002, .F. ) ;
#39297=VERTEX_POINT ( 'NONE', #2016 ) ;
#39298=CARTESIAN_POINT ( 'NONE',  ( -5.000000000000003553, -8.660254037844383745, -39.99999999999997868 ) ) ;
#39299=CARTESIAN_POINT ( 'NONE',  ( -9.999999999999998224, 1.224646799147353059E-15, -16.62500000409675138 ) ) ;
#39300=CARTESIAN_POINT ( 'NONE',  ( -5.405949406250003975, -9.363379034771801557, -44.03125000204838102 ) ) ;
#39305=CARTESIAN_POINT ( 'NONE',  ( 10.81189881249999729, 0.000000000000000000, -135.0312500020484094 ) ) ;
#39306=CARTESIAN_POINT ( 'NONE',  ( -10.81189881249999729, 1.324075727343319199E-15, -147.7812500020483810 ) ) ;
#39309=ORIENTED_EDGE ( 'NONE', *, *, #12220, .T. ) ;
#39312=CARTESIAN_POINT ( 'NONE',  ( -2.121150477449813534E-15, -11.54700538379251284, -129.8750000000000000 ) ) ;
#39313=CARTESIAN_POINT ( 'NONE',  ( 5.405949406249999534, 9.363379034771803333, -175.0937500020484094 ) ) ;
#39314=CARTESIAN_POINT ( 'NONE',  ( -10.81189881249999729, 1.324075727343319199E-15, -24.59375000204835970 ) ) ;
#39316=CARTESIAN_POINT ( 'NONE',  ( 10.81189881249999729, 6.242252689847867408, -155.7187500020483810 ) ) ;
#39317=CARTESIAN_POINT ( 'NONE',  ( 5.405949406249999534, 9.363379034771803333, -145.0937500020483810 ) ) ;
#39320=CARTESIAN_POINT ( 'NONE',  ( 10.81189881249999551, -6.242252689847874514, -19.46875000204837391 ) ) ;
#39323=CARTESIAN_POINT ( 'NONE',  ( 0.000000000000000000, 0.000000000000000000, -200.0000000000000000 ) ) ;
#39325=CARTESIAN_POINT ( 'NONE',  ( -9.999999999999998224, 1.224646799147353059E-15, -200.0000000000000000 ) ) ;
#39327=CARTESIAN_POINT ( 'NONE',  ( -10.81189881249999907, -6.242252689847864744, -75.46875000204836681 ) ) ;
#39328=CARTESIAN_POINT ( 'NONE',  ( 7.644554776091147741E-16, 12.48450537969573659, -38.65625000204835260 ) ) ;
#39330=LINE ( 'NONE', #19266, #632 ) ;
#39332=AXIS2_PLACEMENT_3D ( 'NONE', #6820, #19761, #13484 ) ;
#39333=CARTESIAN_POINT ( 'NONE',  ( 10.00000000000000000, 5.773502691896255534, -135.3750000000000000 ) ) ;
#39334=CARTESIAN_POINT ( 'NONE',  ( 10.81189881249999729, 0.000000000000000000, -135.0312500020484094 ) ) ;
#39335=CARTESIAN_POINT ( 'NONE',  ( 9.999999999999998224, 0.000000000000000000, -200.0000000000000000 ) ) ;
#39336=CARTESIAN_POINT ( 'NONE',  ( 10.00000000000000000, 5.773502691896255534, -116.2500000040967905 ) ) ;
#39338=ORIENTED_EDGE ( 'NONE', *, *, #34657, .F. ) ;
#39341=CARTESIAN_POINT ( 'NONE',  ( -9.999999999998969713, -5.773502691896847949, -22.50000000409674783 ) ) ;
#39342=CARTESIAN_POINT ( 'NONE',  ( -10.81189881249999729, 6.242252689847871849, -173.4062500020483810 ) ) ;
#39343=CARTESIAN_POINT ( 'NONE',  ( -9.999999999999998224, 1.224646799147353059E-15, -45.12500000409677625 ) ) ;
#39345=CARTESIAN_POINT ( 'NONE',  ( 0.000000000000000000, 0.000000000000000000, -200.0000000000000000 ) ) ;
#39346=CARTESIAN_POINT ( 'NONE',  ( 7.644554776091147741E-16, 12.48450537969573659, -161.6562500020484379 ) ) ;
#39347=ADVANCED_FACE ( 'NONE', ( #41902 ), #25534, .T. ) ;
#39348=CARTESIAN_POINT ( 'NONE',  ( 7.644554776091147741E-16, 12.48450537969573659, -141.9687500020483810 ) ) ;
#39350=EDGE_CURVE ( 'NONE', #36973, #7623, #14516, .T. ) ;
#39351=ORIENTED_EDGE ( 'NONE', *, *, #14112, .T. ) ;
#39352=EDGE_CURVE ( 'NONE', #37499, #10842, #6881, .T. ) ;
#39353=CARTESIAN_POINT ( 'NONE',  ( 7.070501591499376803E-16, 11.54700538379251284, -189.5000000040968189 ) ) ;
#39354=VECTOR ( 'NONE', #16619, 1000.000000000000000 ) ;
#39356=CARTESIAN_POINT ( 'NONE',  ( -10.81189881249999729, 6.242252689847871849, -71.40625000204838102 ) ) ;
#39357=ORIENTED_EDGE ( 'NONE', *, *, #5309, .T. ) ;
#39359=CARTESIAN_POINT ( 'NONE',  ( 10.81189881249999729, 0.000000000000000000, -122.8437500020483952 ) ) ;
#39362=( BOUNDED_CURVE ( )  B_SPLINE_CURVE ( 2, ( #24466, #21419, #36967, #24251, #27476, #37613, #30517 ),
 .UNSPECIFIED., .F., .F. ) 
 B_SPLINE_CURVE_WITH_KNOTS ( ( 3, 2, 2, 3 ),
 ( 0.2761194029850747578, 0.2773631840796020875, 0.2786069651741294728, 0.2798507462686568026 ),
 .UNSPECIFIED. ) 
 CURVE ( )  GEOMETRIC_REPRESENTATION_ITEM ( )  RATIONAL_B_SPLINE_CURVE ( ( 0.9999999999999880096, 0.8660254037844506980, 1.000000000000000000, 0.8660254037844387076, 1.000000000000000000, 0.8660254037844267172, 1.000000000000011990 ) ) 
 REPRESENTATION_ITEM ( '' )  );
#39363=CARTESIAN_POINT ( 'NONE',  ( 5.405949406249992428, -9.363379034771808662, -24.09375000204835970 ) ) ;
#39364=CARTESIAN_POINT ( 'NONE',  ( 10.81189881249999729, 0.000000000000000000, -197.8437500020484094 ) ) ;
#39365=CARTESIAN_POINT ( 'NONE',  ( -2.293366432827344421E-15, -12.48450537969573659, -46.71875000204835970 ) ) ;
#39368=ADVANCED_FACE ( 'NONE', ( #40299 ), #10319, .T. ) ;
#39369=CARTESIAN_POINT ( 'NONE',  ( -10.81189881249999729, 6.242252689847871849, -183.7187500020484379 ) ) ;
#39370=CARTESIAN_POINT ( 'NONE',  ( -2.293366432827344421E-15, -12.48450537969573659, -165.2187500020484094 ) ) ;
#39376=CARTESIAN_POINT ( 'NONE',  ( 10.81189881249999551, -6.242252689847874514, -94.46875000204838102 ) ) ;
#39377=LINE ( 'NONE', #38759, #11393 ) ;
#39378=CARTESIAN_POINT ( 'NONE',  ( 10.81189881249999907, 6.242252689847868297, -71.90625000204836681 ) ) ;
#39379=CARTESIAN_POINT ( 'NONE',  ( 7.070501591499376803E-16, 11.54700538379251284, -89.00000000409679046 ) ) ;
#39381=EDGE_CURVE ( 'NONE', #20180, #24638, #33227, .T. ) ;
#39382=ADVANCED_FACE ( 'NONE', ( #30411 ), #10109, .T. ) ;
#39383=CARTESIAN_POINT ( 'NONE',  ( 10.81189881249999729, 0.000000000000000000, -165.0312500020484094 ) ) ;
#39385=CARTESIAN_POINT ( 'NONE',  ( 4.999999999999992006, -8.660254037844389075, -136.1250000040967620 ) ) ;
#39391=CARTESIAN_POINT ( 'NONE',  ( -2.293366432827344421E-15, -12.48450537969573659, -198.4062500020484094 ) ) ;
#39392=CARTESIAN_POINT ( 'NONE',  ( 9.999999999999998224, 0.000000000000000000, -200.0000000000000000 ) ) ;
#39394=VERTEX_POINT ( 'NONE', #36655 ) ;
#39395=CARTESIAN_POINT ( 'NONE',  ( -4.999999999999996447, 8.660254037844387298, -61.49999999999997158 ) ) ;
#39397=CARTESIAN_POINT ( 'NONE',  ( 10.00000000000000000, 5.773502691896255534, -62.25000000409677625 ) ) ;
#39398=CARTESIAN_POINT ( 'NONE',  ( -10.00000000000102496, 5.773502691895664007, -65.87499999999995737 ) ) ;
#39399=DIRECTION ( 'NONE',  ( 1.000000000000000000, 0.000000000000000000, 0.000000000000000000 ) ) ;
#39401=CARTESIAN_POINT ( 'NONE',  ( 5.405949406249999534, 9.363379034771803333, -70.28125000204838102 ) ) ;
#39404=CARTESIAN_POINT ( 'NONE',  ( -4.999999999999996447, 8.660254037844387298, -37.87500000409676915 ) ) ;
#39405=CARTESIAN_POINT ( 'NONE',  ( 10.81189881249999907, 6.242252689847868297, -184.4062500020484094 ) ) ;
#39406=AXIS2_PLACEMENT_3D ( 'NONE', #6267, #10121, #29561 ) ;
#39408=CARTESIAN_POINT ( 'NONE',  ( 9.999999999999998224, 0.000000000000000000, -40.99999999999997868 ) ) ;
#39409=CARTESIAN_POINT ( 'NONE',  ( -10.00000000000012434, 5.773502691896184480, -164.8749999999999716 ) ) ;
#39410=EDGE_CURVE ( 'NONE', #4655, #18018, #8754, .T. ) ;
#39414=CARTESIAN_POINT ( 'NONE',  ( 9.999999999999996447, -5.773502691896262640, -168.6250000000000000 ) ) ;
#39415=DIRECTION ( 'NONE',  ( -0.000000000000000000, -0.000000000000000000, 1.000000000000000000 ) ) ;
#39417=CARTESIAN_POINT ( 'NONE',  ( -10.81189881249999907, -6.242252689847864744, -96.65625000204839523 ) ) ;
#39418=ORIENTED_EDGE ( 'NONE', *, *, #32437, .F. ) ;
#39419=CARTESIAN_POINT ( 'NONE',  ( -11.54700538379250396, -20.00000000000000355, 49.99999999999998579 ) ) ;
#39421=ORIENTED_EDGE ( 'NONE', *, *, #4231, .T. ) ;
#39422=ORIENTED_EDGE ( 'NONE', *, *, #10150, .T. ) ;
#39424=CARTESIAN_POINT ( 'NONE',  ( 5.405949406249999534, 9.363379034771803333, -31.09375000204836326 ) ) ;
#39425=CARTESIAN_POINT ( 'NONE',  ( -5.405949406250003975, -9.363379034771801557, -20.03125000204836326 ) ) ;
#39427=CARTESIAN_POINT ( 'NONE',  ( -5.405949406249996869, 9.363379034771805109, -71.34375000204836681 ) ) ;
#39428=CARTESIAN_POINT ( 'NONE',  ( -9.999999999998969713, -5.773502691896847949, -84.00000000409676204 ) ) ;
#39429=CARTESIAN_POINT ( 'NONE',  ( -5.405949406250003975, -9.363379034771801557, -192.3437500020484094 ) ) ;
#39430=EDGE_CURVE ( 'NONE', #5733, #41070, #23713, .T. ) ;
#39434=CARTESIAN_POINT ( 'NONE',  ( 10.00000000000000000, 5.773502691896255534, -2.250000004096754491 ) ) ;
#39435=CARTESIAN_POINT ( 'NONE',  ( 7.070501591499376803E-16, 11.54700538379251284, -50.00000000409675494 ) ) ;
#39436=CARTESIAN_POINT ( 'NONE',  ( -5.405949406249996869, 9.363379034771805109, -122.3437500020483952 ) ) ;
#39437=CARTESIAN_POINT ( 'NONE',  ( -10.81189881249999729, 1.324075727343319199E-15, -99.78125000204839523 ) ) ;
#39438=CARTESIAN_POINT ( 'NONE',  ( -5.405949406249996869, 9.363379034771805109, -111.8437500020483810 ) ) ;
#39441=CARTESIAN_POINT ( 'NONE',  ( -10.00000000000000000, -5.773502691896251982, -159.0000000040967905 ) ) ;
#39442=DIRECTION ( 'NONE',  ( -0.000000000000000000, -0.000000000000000000, 1.000000000000000000 ) ) ;
#39446=CARTESIAN_POINT ( 'NONE',  ( 4.999999999999992006, -8.660254037844389075, -156.7500000000000000 ) ) ;
#39448=CYLINDRICAL_SURFACE ( 'NONE', #15072, 9.999999999999998224 ) ;
#39450=CARTESIAN_POINT ( 'NONE',  ( -10.00000000000000000, -5.773502691896251982, -85.12499999999997158 ) ) ;
#39452=CARTESIAN_POINT ( 'NONE',  ( -9.999999999999998224, 5.773502691896259087, -96.25000000409677625 ) ) ;
#39453=FACE_OUTER_BOUND ( 'NONE', #23987, .T. ) ;
#39455=CARTESIAN_POINT ( 'NONE',  ( 5.405949406249992428, -9.363379034771808662, -94.78125000204838102 ) ) ;
#39456=ORIENTED_EDGE ( 'NONE', *, *, #42575, .F. ) ;
#39457=AXIS2_PLACEMENT_3D ( 'NONE', #2740, #29274, #12848 ) ;
#39459=PLANE ( 'NONE',  #37377 ) ;
#39461=ORIENTED_EDGE ( 'NONE', *, *, #836, .F. ) ;
#39462=CARTESIAN_POINT ( 'NONE',  ( -4.999999999999996447, 8.660254037844387298, -8.999999999999952038 ) ) ;
#39463=CARTESIAN_POINT ( 'NONE',  ( 5.000000000000000000, 8.660254037844385522, -144.2500000000000000 ) ) ;
#39464=( BOUNDED_CURVE ( )  B_SPLINE_CURVE ( 2, ( #27490, #957, #4396, #30736, #17535, #23408, #7207 ),
 .UNSPECIFIED., .F., .F. ) 
 B_SPLINE_CURVE_WITH_KNOTS ( ( 3, 2, 2, 3 ),
 ( 0.9365671641791047941, 0.9378109452736321794, 0.9390547263681594536, 0.9402985074626868389 ),
 .UNSPECIFIED. ) 
 CURVE ( )  GEOMETRIC_REPRESENTATION_ITEM ( )  RATIONAL_B_SPLINE_CURVE ( ( 0.9999999999999641398, 0.8660254037844745678, 1.000000000000000000, 0.8660254037844387076, 1.000000000000000000, 0.8660254037844148378, 1.000000000000023981 ) ) 
 REPRESENTATION_ITEM ( '' )  );
#39466=CARTESIAN_POINT ( 'NONE',  ( -5.000000000000003553, -8.660254037844383745, -194.5000000000000000 ) ) ;
#39467=CARTESIAN_POINT ( 'NONE',  ( -2.293366432827344421E-15, -12.48450537969573659, -121.9062500020483952 ) ) ;
#39468=ORIENTED_EDGE ( 'NONE', *, *, #39278, .F. ) ;
#39470=ORIENTED_EDGE ( 'NONE', *, *, #9783, .T. ) ;
#39471=CARTESIAN_POINT ( 'NONE',  ( 5.405949406249999534, 9.363379034771803333, -44.78125000204838102 ) ) ;
#39474=CARTESIAN_POINT ( 'NONE',  ( -10.81189881249999907, -6.242252689847864744, -100.9687500020483810 ) ) ;
#39475=CARTESIAN_POINT ( 'NONE',  ( 10.81189881249999729, 6.242252689847867408, -127.4062500020483810 ) ) ;
#39476=ORIENTED_EDGE ( 'NONE', *, *, #41442, .T. ) ;
#39477=CARTESIAN_POINT ( 'NONE',  ( -8.675003188131697129, -4.974413003141672895, -0.0003472602639886801512 ) ) ;
#39480=CARTESIAN_POINT ( 'NONE',  ( 10.81189881249999907, 6.242252689847868297, 0.2812499979516534521 ) ) ;
#39482=CARTESIAN_POINT ( 'NONE',  ( 5.405949406249999534, 9.363379034771803333, -130.0937500020483810 ) ) ;
#39484=CARTESIAN_POINT ( 'NONE',  ( 5.000000000000000000, 8.660254037844385522, -116.1250000040967905 ) ) ;
#39486=CARTESIAN_POINT ( 'NONE',  ( -10.00000000000000000, -5.773502691896251982, -184.5000000040968189 ) ) ;
#39488=CARTESIAN_POINT ( 'NONE',  ( 5.405949406249992428, -9.363379034771808662, -187.7812500020484094 ) ) ;
#39489=CARTESIAN_POINT ( 'NONE',  ( 9.999999999999998224, 0.000000000000000000, -94.99999999999998579 ) ) ;
#39490=CARTESIAN_POINT ( 'NONE',  ( 0.000000000000000000, 0.000000000000000000, -200.0000000000000000 ) ) ;
#39493=CARTESIAN_POINT ( 'NONE',  ( 10.81189881249999551, -6.242252689847874514, -59.96875000204837391 ) ) ;
#39494=CARTESIAN_POINT ( 'NONE',  ( -2.293366432827344421E-15, -12.48450537969573659, -48.21875000204836681 ) ) ;
#39496=CARTESIAN_POINT ( 'NONE',  ( -10.81189881249999729, 1.324075727343319199E-15, -15.78125000204835793 ) ) ;
#39498=DIRECTION ( 'NONE',  ( 0.5000000000000002220, -0.8660254037844384856, 0.000000000000000000 ) ) ;
#39500=CARTESIAN_POINT ( 'NONE',  ( 9.999999999999998224, 0.000000000000000000, -106.9999999999999858 ) ) ;
#39505=CARTESIAN_POINT ( 'NONE',  ( -10.81189881249999729, -6.242252689847864744, -116.1562500020483952 ) ) ;
#39507=( BOUNDED_CURVE ( )  B_SPLINE_CURVE ( 2, ( #37687, #37905, #8129, #40470, #8349, #21500, #24111 ),
 .UNSPECIFIED., .F., .F. ) 
 B_SPLINE_CURVE_WITH_KNOTS ( ( 3, 2, 2, 3 ),
 ( 0.03358208955223884046, 0.03482587064676620492, 0.03606965174129356938, 0.03731343283582092690 ),
 .UNSPECIFIED. ) 
 CURVE ( )  GEOMETRIC_REPRESENTATION_ITEM ( )  RATIONAL_B_SPLINE_CURVE ( ( 0.9999999999999963363, 0.8660254037844424824, 1.000000000000000000, 0.8660254037844387076, 1.000000000000000000, 0.8660254037844349329, 1.000000000000003775 ) ) 
 REPRESENTATION_ITEM ( '' )  );
#39508=CARTESIAN_POINT ( 'NONE',  ( -9.999999999999479527, -5.773502691896549521, -7.124999999999955591 ) ) ;
#39513=CARTESIAN_POINT ( 'NONE',  ( -10.00000000000000000, -5.773502691896251982, -29.62499999999995026 ) ) ;
#39514=CARTESIAN_POINT ( 'NONE',  ( 9.999999999999998224, 0.000000000000000000, -20.37500000409675494 ) ) ;
#39515=CARTESIAN_POINT ( 'NONE',  ( 10.81189881249999551, -6.242252689847874514, -43.65625000204838102 ) ) ;
#39516=CARTESIAN_POINT ( 'NONE',  ( -5.000000000000003553, -8.660254037844383745, -2.499999999999974243 ) ) ;
#39518=( BOUNDED_CURVE ( )  B_SPLINE_CURVE ( 2, ( #19676, #23574, #30264, #16638, #40162, #6950, #3081 ),
 .UNSPECIFIED., .F., .F. ) 
 B_SPLINE_CURVE_WITH_KNOTS ( ( 3, 2, 2, 3 ),
 ( 0.6567164179104479915, 0.6579601990049753768, 0.6592039800995028731, 0.6604477611940301474 ),
 .UNSPECIFIED. ) 
 CURVE ( )  GEOMETRIC_REPRESENTATION_ITEM ( )  RATIONAL_B_SPLINE_CURVE ( ( 0.9999999999999761302, 0.8660254037844625774, 1.000000000000000000, 0.8660254037844387076, 1.000000000000000000, 0.8660254037844028474, 1.000000000000035971 ) ) 
 REPRESENTATION_ITEM ( '' )  );
#39519=DIRECTION ( 'NONE',  ( -0.000000000000000000, -0.000000000000000000, 1.000000000000000000 ) ) ;
#39520=CARTESIAN_POINT ( 'NONE',  ( 10.81189881249999907, 6.242252689847868297, -140.9062500020484094 ) ) ;
#39521=CARTESIAN_POINT ( 'NONE',  ( -10.81189881249999729, 6.242252689847871849, -138.9062500020484094 ) ) ;
#39522=ORIENTED_EDGE ( 'NONE', *, *, #34438, .F. ) ;
#39524=VERTEX_POINT ( 'NONE', #27374 ) ;
#39525=EDGE_LOOP ( 'NONE', ( #30305, #646, #29231, #37727 ) ) ;
#39527=CARTESIAN_POINT ( 'NONE',  ( -10.81189881249999729, 6.242252689847871849, -177.7187500020483810 ) ) ;
#39528=CARTESIAN_POINT ( 'NONE',  ( 10.81189881249999551, -6.242252689847874514, -25.46875000204837391 ) ) ;
#39529=CARTESIAN_POINT ( 'NONE',  ( 0.000000000000000000, 0.000000000000000000, -200.0000000000000000 ) ) ;
#39530=CARTESIAN_POINT ( 'NONE',  ( -10.81189881249999729, -6.242252689847864744, -153.4687500020484094 ) ) ;
#39531=CARTESIAN_POINT ( 'NONE',  ( 5.405949406249992428, -9.363379034771808662, -144.0937500020483810 ) ) ;
#39532=ADVANCED_FACE ( 'NONE', ( #38364 ), #34288, .T. ) ;
#39533=CARTESIAN_POINT ( 'NONE',  ( -5.000000000000003553, -8.660254037844383745, -9.999999999999953815 ) ) ;
#39536=CARTESIAN_POINT ( 'NONE',  ( 10.81189881249999907, 6.242252689847868297, -17.71875000204836681 ) ) ;
#39541=CARTESIAN_POINT ( 'NONE',  ( -5.405949406250003975, -9.363379034771801557, -76.84375000204838102 ) ) ;
#39542=CARTESIAN_POINT ( 'NONE',  ( -10.81189881249999729, 6.242252689847871849, -45.90625000204836681 ) ) ;
#39546=CARTESIAN_POINT ( 'NONE',  ( 9.999999999999996447, -5.773502691896262640, -131.1250000000000000 ) ) ;
#39547=CARTESIAN_POINT ( 'NONE',  ( -10.81189881249999729, 6.242252689847871849, -141.9062500020484094 ) ) ;
#39548=CYLINDRICAL_SURFACE ( 'NONE', #27943, 9.999999999999998224 ) ;
#39549=CARTESIAN_POINT ( 'NONE',  ( 5.000000000000000000, 8.660254037844385522, -116.1250000040967905 ) ) ;
#39555=CARTESIAN_POINT ( 'NONE',  ( -5.405949406249996869, 9.363379034771805109, -161.5312500020484094 ) ) ;
#39556=CARTESIAN_POINT ( 'NONE',  ( -4.999999999999996447, 8.660254037844387298, -40.87500000409677625 ) ) ;
#39557=DIRECTION ( 'NONE',  ( 1.000000000000000000, 0.000000000000000000, 0.000000000000000000 ) ) ;
#39559=DIRECTION ( 'NONE',  ( 0.8660254037844439257, 0.000000000000000000, 0.4999999999999907296 ) ) ;
#39560=CARTESIAN_POINT ( 'NONE',  ( -5.405949406250003975, -9.363379034771801557, -162.5312500020484094 ) ) ;
#39561=CARTESIAN_POINT ( 'NONE',  ( 10.81189881249999551, -6.242252689847874514, -133.4687500020483810 ) ) ;
#39562=DIRECTION ( 'NONE',  ( -0.000000000000000000, -0.000000000000000000, 1.000000000000000000 ) ) ;
#39564=ORIENTED_EDGE ( 'NONE', *, *, #2242, .T. ) ;
#39565=CARTESIAN_POINT ( 'NONE',  ( 9.999999999999479527, 5.773502691896553074, -114.7500000040967620 ) ) ;
#39566=CARTESIAN_POINT ( 'NONE',  ( 5.405949406249992428, -9.363379034771808662, -67.78125000204838102 ) ) ;
#39567=ORIENTED_EDGE ( 'NONE', *, *, #24757, .T. ) ;
#39569=CARTESIAN_POINT ( 'NONE',  ( 10.81189881249999907, 6.242252689847868297, -122.7187500020483810 ) ) ;
#39570=VERTEX_POINT ( 'NONE', #31049 ) ;
#39572=CARTESIAN_POINT ( 'NONE',  ( -10.81189881249999729, -6.242252689847864744, -19.96875000204837747 ) ) ;
#39573=CARTESIAN_POINT ( 'NONE',  ( 7.644554776091147741E-16, 12.48450537969573659, -197.4687500020484094 ) ) ;
#39574=CARTESIAN_POINT ( 'NONE',  ( 10.81189881249999551, -6.242252689847874514, -47.96875000204836681 ) ) ;
#39575=CARTESIAN_POINT ( 'NONE',  ( -2.121150477449813534E-15, -11.54700538379251284, -71.75000000409676204 ) ) ;
#39577=CARTESIAN_POINT ( 'NONE',  ( 7.644554776091147741E-16, 12.48450537969573659, -179.4687500020484094 ) ) ;
#39578=CARTESIAN_POINT ( 'NONE',  ( -5.405949406250003975, -9.363379034771801557, -168.3437500020484094 ) ) ;
#39582=CARTESIAN_POINT ( 'NONE',  ( -9.999999999999998224, 1.224646799147353059E-15, -193.2500000000000000 ) ) ;
#39584=CARTESIAN_POINT ( 'NONE',  ( -5.405949406250003975, -9.363379034771801557, -97.84375000204838102 ) ) ;
#39585=CARTESIAN_POINT ( 'NONE',  ( 9.999999999999479527, 5.773502691896553074, -34.87499999999994316 ) ) ;
#39586=CARTESIAN_POINT ( 'NONE',  ( -2.293366432827344421E-15, -12.48450537969573659, -63.40625000204838102 ) ) ;
#39587=EDGE_CURVE ( 'NONE', #8170, #12734, #21985, .T. ) ;
#39589=CARTESIAN_POINT ( 'NONE',  ( -10.81189881249999907, -6.242252689847864744, -122.1562500020484094 ) ) ;
#39590=CARTESIAN_POINT ( 'NONE',  ( -5.405949406249996869, 9.363379034771805109, -164.5312500020484094 ) ) ;
#39591=EDGE_CURVE ( 'NONE', #6518, #25484, #3840, .T. ) ;
#39593=CARTESIAN_POINT ( 'NONE',  ( 5.000000000000000000, 8.660254037844385522, -135.6250000040967620 ) ) ;
#39595=ORIENTED_EDGE ( 'NONE', *, *, #10920, .T. ) ;
#39598=CARTESIAN_POINT ( 'NONE',  ( -2.293366432827344421E-15, -12.48450537969573659, -195.4062500020484094 ) ) ;
#39601=ORIENTED_EDGE ( 'NONE', *, *, #17172, .F. ) ;
#39602=CARTESIAN_POINT ( 'NONE',  ( 4.999999999999992006, -8.660254037844389075, -54.74999999999996447 ) ) ;
#39604=CARTESIAN_POINT ( 'NONE',  ( -9.999999999999998224, 5.773502691896259087, -63.25000000409679757 ) ) ;
#39605=FACE_OUTER_BOUND ( 'NONE', #5920, .T. ) ;
#39608=CARTESIAN_POINT ( 'NONE',  ( -2.293366432827344421E-15, -12.48450537969573659, -57.40625000204838102 ) ) ;
#39611=CARTESIAN_POINT ( 'NONE',  ( 4.999999999999992006, -8.660254037844389075, -151.1250000040967905 ) ) ;
#39612=CARTESIAN_POINT ( 'NONE',  ( 10.81189881249999729, 0.000000000000000000, -183.0312500020484094 ) ) ;
#39616=CARTESIAN_POINT ( 'NONE',  ( 0.000000000000000000, 0.000000000000000000, -200.0000000000000000 ) ) ;
#39617=( BOUNDED_CURVE ( )  B_SPLINE_CURVE ( 2, ( #26202, #30299, #16885, #6985, #10418, #3960, #19500 ),
 .UNSPECIFIED., .F., .F. ) 
 B_SPLINE_CURVE_WITH_KNOTS ( ( 3, 2, 2, 3 ),
 ( 0.4141791044776120256, 0.4154228855721394109, 0.4166666666666667962, 0.4179104477611941260 ),
 .UNSPECIFIED. ) 
 CURVE ( )  GEOMETRIC_REPRESENTATION_ITEM ( )  RATIONAL_B_SPLINE_CURVE ( ( 0.9999999999999880096, 0.8660254037844506980, 1.000000000000000000, 0.8660254037844387076, 1.000000000000000000, 0.8660254037844267172, 1.000000000000011990 ) ) 
 REPRESENTATION_ITEM ( '' )  );
#39618=CARTESIAN_POINT ( 'NONE',  ( 9.999999999999996447, -5.773502691896262640, -170.1250000000000000 ) ) ;
#39620=CARTESIAN_POINT ( 'NONE',  ( 5.405949406249999534, 9.363379034771803333, -95.78125000204838102 ) ) ;
#39621=VERTEX_POINT ( 'NONE', #31694 ) ;
#39622=CARTESIAN_POINT ( 'NONE',  ( -10.00000000000025580, 5.773502691896109873, -161.8749999999999716 ) ) ;
#39623=ORIENTED_EDGE ( 'NONE', *, *, #28102, .F. ) ;
#39624=EDGE_LOOP ( 'NONE', ( #42275, #24900, #12551, #9583 ) ) ;
#39625=CARTESIAN_POINT ( 'NONE',  ( -2.293366432827344421E-15, -12.48450537969573659, -34.71875000204835260 ) ) ;
#39626=CARTESIAN_POINT ( 'NONE',  ( -10.81189881249999729, 1.324075727343319199E-15, -21.78125000204836326 ) ) ;
#39628=CARTESIAN_POINT ( 'NONE',  ( 7.644554776091147741E-16, 12.48450537969573659, -71.46875000204838102 ) ) ;
#39629=CARTESIAN_POINT ( 'NONE',  ( -9.999999999999998224, 1.224646799147353059E-15, -165.1250000040967905 ) ) ;
#39630=CARTESIAN_POINT ( 'NONE',  ( -10.81189881249999729, 1.324075727343319199E-15, -197.0937500020484094 ) ) ;
#39631=CARTESIAN_POINT ( 'NONE',  ( -5.405949406250003975, -9.363379034771801557, -153.3437500020483810 ) ) ;
#39632=DIRECTION ( 'NONE',  ( -0.000000000000000000, -0.000000000000000000, 1.000000000000000000 ) ) ;
#39633=CARTESIAN_POINT ( 'NONE',  ( 9.999999999999998224, 0.000000000000000000, -112.9999999999999858 ) ) ;
#39635=CARTESIAN_POINT ( 'NONE',  ( 9.999999999999998224, 0.000000000000000000, 0.6249999959032359609 ) ) ;
#39636=CARTESIAN_POINT ( 'NONE',  ( -9.999999999999998224, 1.224646799147353059E-15, -143.7500000000000000 ) ) ;
#39637=CARTESIAN_POINT ( 'NONE',  ( -2.293366432827344421E-15, -12.48450537969573659, -120.2187500020483952 ) ) ;
#39639=CARTESIAN_POINT ( 'NONE',  ( -10.81189881249999907, -6.242252689847864744, -87.65625000204836681 ) ) ;
#39640=ADVANCED_FACE ( 'NONE', ( #14616 ), #40936, .T. ) ;
#39641=CARTESIAN_POINT ( 'NONE',  ( -5.405949406249996869, 9.363379034771805109, -110.3437500020483810 ) ) ;
#39644=CARTESIAN_POINT ( 'NONE',  ( -9.999999999999998224, 5.773502691896259087, -163.7500000040967905 ) ) ;
#39652=CARTESIAN_POINT ( 'NONE',  ( 0.000000000000000000, 0.000000000000000000, -200.0000000000000000 ) ) ;
#39654=CARTESIAN_POINT ( 'NONE',  ( 10.00000000000000000, 5.773502691896255534, -84.37499999999998579 ) ) ;
#39656=CARTESIAN_POINT ( 'NONE',  ( 9.999999999999998224, 0.000000000000000000, -87.87500000409677625 ) ) ;
#39657=VECTOR ( 'NONE', #10630, 1000.000000000000114 ) ;
#39661=CARTESIAN_POINT ( 'NONE',  ( 5.405949406249992428, -9.363379034771808662, -79.78125000204838102 ) ) ;
#39667=CARTESIAN_POINT ( 'NONE',  ( 5.000000000000000000, 8.660254037844385522, -6.249999999999977796 ) ) ;
#39668=CARTESIAN_POINT ( 'NONE',  ( 9.999999999999998224, 0.000000000000000000, -146.0000000000000000 ) ) ;
#39669=CARTESIAN_POINT ( 'NONE',  ( 4.999999999999992006, -8.660254037844389075, -32.24999999999997158 ) ) ;
#39671=ADVANCED_FACE ( 'NONE', ( #1480 ), #37942, .T. ) ;
#39672=CARTESIAN_POINT ( 'NONE',  ( 4.999999999999992006, -8.660254037844389075, -186.7500000000000000 ) ) ;
#39673=CARTESIAN_POINT ( 'NONE',  ( 9.999999999999998224, 0.000000000000000000, -200.0000000000000000 ) ) ;
#39674=CARTESIAN_POINT ( 'NONE',  ( -10.81189881249999729, 6.242252689847871849, -119.4062500020483952 ) ) ;
#39679=VECTOR ( 'NONE', #38362, 1000.000000000000114 ) ;
#39680=CARTESIAN_POINT ( 'NONE',  ( 10.81189881249999907, 6.242252689847868297, -49.40625000204837391 ) ) ;
#39682=CARTESIAN_POINT ( 'NONE',  ( 10.81189881249999729, 0.000000000000000000, -98.84375000204838102 ) ) ;
#39683=CARTESIAN_POINT ( 'NONE',  ( -10.81189881249999729, 6.242252689847871849, -126.9062500020483810 ) ) ;
#39684=VERTEX_POINT ( 'NONE', #8596 ) ;
#39685=AXIS2_PLACEMENT_3D ( 'NONE', #29884, #33344, #24046 ) ;
#39686=CARTESIAN_POINT ( 'NONE',  ( -2.121150477449813534E-15, -11.54700538379251284, -132.8750000000000000 ) ) ;
#39687=FACE_OUTER_BOUND ( 'NONE', #3179, .T. ) ;
#39690=CARTESIAN_POINT ( 'NONE',  ( -10.81189881249999729, 6.242252689847871849, -128.2187500020483810 ) ) ;
#39692=CARTESIAN_POINT ( 'NONE',  ( -9.999999999999872102, -5.773502691896326589, -158.6250000000000284 ) ) ;
#39694=CARTESIAN_POINT ( 'NONE',  ( -5.000000000000003553, -8.660254037844383745, -187.3750000040967905 ) ) ;
#39696=CARTESIAN_POINT ( 'NONE',  ( -5.405949406250003975, -9.363379034771801557, -189.5312500020484094 ) ) ;
#39697=CARTESIAN_POINT ( 'NONE',  ( -5.000000000000003553, -8.660254037844383745, -95.49999999999998579 ) ) ;
#39701=CARTESIAN_POINT ( 'NONE',  ( -5.405949406250003975, -9.363379034771801557, -61.84375000204836681 ) ) ;
#39702=CARTESIAN_POINT ( 'NONE',  ( -5.405949406249996869, 9.363379034771805109, -51.84375000204835260 ) ) ;
#39704=CARTESIAN_POINT ( 'NONE',  ( 10.81189881249999551, -6.242252689847874514, -18.15625000204837036 ) ) ;
#39707=CARTESIAN_POINT ( 'NONE',  ( -10.00000000000000000, -5.773502691896251982, -101.6249999999999858 ) ) ;
#39709=( BOUNDED_CURVE ( )  B_SPLINE_CURVE ( 2, ( #17063, #26800, #30046, #23995, #27012, #20955, #30261 ),
 .UNSPECIFIED., .F., .F. ) 
 B_SPLINE_CURVE_WITH_KNOTS ( ( 3, 2, 2, 3 ),
 ( 0.1417910447761193959, 0.1430348258706467535, 0.1442786069651741387, 0.1455223880597014963 ),
 .UNSPECIFIED. ) 
 CURVE ( )  GEOMETRIC_REPRESENTATION_ITEM ( )  RATIONAL_B_SPLINE_CURVE ( ( 1.000000000000000000, 0.8660254037844387076, 1.000000000000000000, 0.8660254037844387076, 1.000000000000000000, 0.8660254037844387076, 1.000000000000000000 ) ) 
 REPRESENTATION_ITEM ( '' )  );
#39710=CARTESIAN_POINT ( 'NONE',  ( 10.00000000000051159, -5.773502691895965988, -114.6249999999999574 ) ) ;
#39714=CARTESIAN_POINT ( 'NONE',  ( -10.81189881249999729, 6.242252689847871849, -111.9062500020483810 ) ) ;
#39715=ORIENTED_EDGE ( 'NONE', *, *, #4039, .T. ) ;
#39716=DIRECTION ( 'NONE',  ( -0.000000000000000000, -0.000000000000000000, 1.000000000000000000 ) ) ;
#39718=LINE ( 'NONE', #23335, #31207 ) ;
#39721=CARTESIAN_POINT ( 'NONE',  ( -10.00000000000000000, -5.773502691896251982, -35.62499999999996447 ) ) ;
#39722=EDGE_CURVE ( 'NONE', #30518, #33970, #21101, .T. ) ;
#39723=CARTESIAN_POINT ( 'NONE',  ( 5.000000000000000000, 8.660254037844385522, -21.62500000409675494 ) ) ;
#39724=CARTESIAN_POINT ( 'NONE',  ( 10.81189881249999551, -6.242252689847874514, -45.15625000204836681 ) ) ;
#39725=CARTESIAN_POINT ( 'NONE',  ( 4.999999999999992006, -8.660254037844389075, -2.249999999999974243 ) ) ;
#39728=CARTESIAN_POINT ( 'NONE',  ( 7.644554776091147741E-16, 12.48450537969573659, -143.6562500020484094 ) ) ;
#39730=VERTEX_POINT ( 'NONE', #17852 ) ;
#39731=VERTEX_POINT ( 'NONE', #34505 ) ;
#39732=ORIENTED_EDGE ( 'NONE', *, *, #23539, .F. ) ;
#39733=CARTESIAN_POINT ( 'NONE',  ( 7.070501591499376803E-16, 11.54700538379251284, -159.1250000000000284 ) ) ;
#39734=FACE_OUTER_BOUND ( 'NONE', #37082, .T. ) ;
#39735=CARTESIAN_POINT ( 'NONE',  ( -10.81189881249999729, 6.242252689847871849, -170.2187500020483810 ) ) ;
#39736=CARTESIAN_POINT ( 'NONE',  ( 9.999999999999996447, -5.773502691896262640, -192.6250000000000284 ) ) ;
#39737=CARTESIAN_POINT ( 'NONE',  ( -5.405949406250003975, -9.363379034771801557, -21.34375000204835615 ) ) ;
#39738=DIRECTION ( 'NONE',  ( -0.000000000000000000, -0.000000000000000000, 1.000000000000000000 ) ) ;
#39739=CARTESIAN_POINT ( 'NONE',  ( -5.405949406249996869, 9.363379034771805109, -159.8437500020484094 ) ) ;
#39740=CARTESIAN_POINT ( 'NONE',  ( -10.81189881249999729, 1.324075727343319199E-15, -144.5937500020483810 ) ) ;
#39741=CARTESIAN_POINT ( 'NONE',  ( -9.999999999999996447, 5.773502691896259975, -172.7500000040967905 ) ) ;
#39744=CARTESIAN_POINT ( 'NONE',  ( 5.405949406249992428, -9.363379034771808662, -9.093750002048345493 ) ) ;
#39747=( BOUNDED_CURVE ( )  B_SPLINE_CURVE ( 2, ( #8240, #34571, #28527, #5002, #8457, #31339, #21608 ),
 .UNSPECIFIED., .F., .F. ) 
 B_SPLINE_CURVE_WITH_KNOTS ( ( 3, 2, 2, 3 ),
 ( 0.1902985074626866169, 0.1915422885572139744, 0.1927860696517413319, 0.1940298507462686894 ),
 .UNSPECIFIED. ) 
 CURVE ( )  GEOMETRIC_REPRESENTATION_ITEM ( )  RATIONAL_B_SPLINE_CURVE ( ( 0.9999999999999940048, 0.8660254037844447028, 1.000000000000000000, 0.8660254037844387076, 1.000000000000000000, 0.8660254037844357100, 1.000000000000003109 ) ) 
 REPRESENTATION_ITEM ( '' )  );
#39748=CARTESIAN_POINT ( 'NONE',  ( 7.070501591499376803E-16, 11.54700538379251284, -44.00000000409676204 ) ) ;
#39751=CARTESIAN_POINT ( 'NONE',  ( -10.81189881249999729, 1.324075727343319199E-15, -77.09375000204838102 ) ) ;
#39752=CARTESIAN_POINT ( 'NONE',  ( 5.405949406249992428, -9.363379034771808662, -39.28125000204838102 ) ) ;
#39754=CARTESIAN_POINT ( 'NONE',  ( -9.999999999999227285, -5.773502691896698735, -114.0000000040967478 ) ) ;
#39756=CARTESIAN_POINT ( 'NONE',  ( -9.999999999999998224, 1.224646799147353059E-15, -130.2499999999999716 ) ) ;
#39757=CARTESIAN_POINT ( 'NONE',  ( 5.405949406249999534, 9.363379034771803333, -136.2812500020483810 ) ) ;
#39759=CARTESIAN_POINT ( 'NONE',  ( 5.000000000000000000, 8.660254037844385522, -114.6250000040967763 ) ) ;
#39765=CARTESIAN_POINT ( 'NONE',  ( -9.999999999999998224, 1.224646799147353059E-15, -200.0000000000000000 ) ) ;
#39766=CARTESIAN_POINT ( 'NONE',  ( 7.644554776091147741E-16, 12.48450537969573659, -161.6562500020484379 ) ) ;
#39767=CARTESIAN_POINT ( 'NONE',  ( -4.999999999999996447, 8.660254037844387298, -39.37500000409676915 ) ) ;
#39768=CARTESIAN_POINT ( 'NONE',  ( -4.999999999999996447, 8.660254037844387298, -154.8750000040967905 ) ) ;
#39770=CARTESIAN_POINT ( 'NONE',  ( -2.121150477449813534E-15, -11.54700538379251284, -63.87499999999998579 ) ) ;
#39771=CARTESIAN_POINT ( 'NONE',  ( -10.81189881249999729, 6.242252689847871849, -162.9062500020484094 ) ) ;
#39772=CARTESIAN_POINT ( 'NONE',  ( 10.81189881249999729, 0.000000000000000000, -136.3437500020484094 ) ) ;
#39773=CARTESIAN_POINT ( 'NONE',  ( 9.999999999999998224, 0.000000000000000000, -60.87500000409676204 ) ) ;
#39774=CARTESIAN_POINT ( 'NONE',  ( 9.999999999999998224, 0.000000000000000000, -143.0000000000000000 ) ) ;
#39775=ORIENTED_EDGE ( 'NONE', *, *, #30548, .F. ) ;
#39777=EDGE_CURVE ( 'NONE', #40396, #12739, #2127, .T. ) ;
#39778=CARTESIAN_POINT ( 'NONE',  ( 10.81189881249999551, -6.242252689847874514, -67.65625000204838102 ) ) ;
#39779=VERTEX_POINT ( 'NONE', #18075 ) ;
#39780=CARTESIAN_POINT ( 'NONE',  ( -5.405949406249996869, 9.363379034771805109, -122.3437500020483952 ) ) ;
#39782=ORIENTED_EDGE ( 'NONE', *, *, #42588, .T. ) ;
#39783=CARTESIAN_POINT ( 'NONE',  ( 7.644554776091147741E-16, 12.48450537969573659, -24.96875000204837036 ) ) ;
#39785=CARTESIAN_POINT ( 'NONE',  ( -10.81189881249999729, 1.324075727343319199E-15, -195.5937500020484094 ) ) ;
#39786=CARTESIAN_POINT ( 'NONE',  ( 10.81189881249999551, -6.242252689847874514, -49.46875000204835970 ) ) ;
#39787=CARTESIAN_POINT ( 'NONE',  ( -9.999999999999998224, 1.224646799147353059E-15, -200.0000000000000000 ) ) ;
#39789=CARTESIAN_POINT ( 'NONE',  ( -5.405949406250003975, -9.363379034771801557, -177.3437500020483810 ) ) ;
#39790=CARTESIAN_POINT ( 'NONE',  ( -5.405949406250003975, -9.363379034771801557, -171.3437500020484094 ) ) ;
#39796=CARTESIAN_POINT ( 'NONE',  ( -2.293366432827344421E-15, -12.48450537969573659, -99.21875000204839523 ) ) ;
#39797=EDGE_CURVE ( 'NONE', #8336, #2222, #15663, .T. ) ;
#39799=CARTESIAN_POINT ( 'NONE',  ( 10.81189881249999551, -6.242252689847874514, -67.65625000204838102 ) ) ;
#39800=CARTESIAN_POINT ( 'NONE',  ( -9.999999999999998224, 1.224646799147353059E-15, -5.749999999999976907 ) ) ;
#39802=CARTESIAN_POINT ( 'NONE',  ( 10.81189881249999551, -6.242252689847874514, -124.6562500020483952 ) ) ;
#39803=CARTESIAN_POINT ( 'NONE',  ( 10.81189881249999729, 0.000000000000000000, -160.5312500020484094 ) ) ;
#39805=CARTESIAN_POINT ( 'NONE',  ( 5.000000000000000000, 8.660254037844385522, -138.6250000040967905 ) ) ;
#39807=ORIENTED_EDGE ( 'NONE', *, *, #29664, .F. ) ;
#39810=CARTESIAN_POINT ( 'NONE',  ( -2.293366432827344421E-15, -12.48450537969573659, -192.4062500020484094 ) ) ;
#39811=CARTESIAN_POINT ( 'NONE',  ( -9.999999999998969713, -5.773502691896847949, -43.50000000409674783 ) ) ;
#39814=CARTESIAN_POINT ( 'NONE',  ( -9.999999999999998224, 5.773502691896259087, -56.87499999999998579 ) ) ;
#39816=CARTESIAN_POINT ( 'NONE',  ( 5.000000000000000000, 8.660254037844385522, -63.62500000409676204 ) ) ;
#39817=VECTOR ( 'NONE', #41810, 1000.000000000000000 ) ;
#39818=CARTESIAN_POINT ( 'NONE',  ( -4.999999999999996447, 8.660254037844387298, -21.37500000409675494 ) ) ;
#39819=CARTESIAN_POINT ( 'NONE',  ( 9.999999999999612754, 5.773502691896477579, -179.2500000040967905 ) ) ;
#39821=CARTESIAN_POINT ( 'NONE',  ( -10.81189881249999729, -6.242252689847864744, -56.15625000204837391 ) ) ;
#39824=CARTESIAN_POINT ( 'NONE',  ( 9.999999999999998224, 0.000000000000000000, -137.3750000040967905 ) ) ;
#39825=CARTESIAN_POINT ( 'NONE',  ( -5.405949406250003975, -9.363379034771801557, -183.5312500020484094 ) ) ;
#39827=CARTESIAN_POINT ( 'NONE',  ( 7.070501591499376803E-16, 11.54700538379251284, -79.62500000000000000 ) ) ;
#39829=( BOUNDED_CURVE ( )  B_SPLINE_CURVE ( 2, ( #7131, #24404, #23749, #1518, #37112, #3900, #26771 ),
 .UNSPECIFIED., .F., .F. ) 
 B_SPLINE_CURVE_WITH_KNOTS ( ( 3, 2, 2, 3 ),
 ( 0.7425373134328361324, 0.7437810945273634067, 0.7450248756218907920, 0.7462686567164180662 ),
 .UNSPECIFIED. ) 
 CURVE ( )  GEOMETRIC_REPRESENTATION_ITEM ( )  RATIONAL_B_SPLINE_CURVE ( ( 0.9999999999999641398, 0.8660254037844745678, 1.000000000000000000, 0.8660254037844387076, 1.000000000000000000, 0.8660254037844267172, 1.000000000000011990 ) ) 
 REPRESENTATION_ITEM ( '' )  );
#39832=CARTESIAN_POINT ( 'NONE',  ( 10.00000000000000000, 5.773502691896255534, -166.8750000000000000 ) ) ;
#39834=CARTESIAN_POINT ( 'NONE',  ( -5.405949406249996869, 9.363379034771805109, -91.03125000204838102 ) ) ;
#39836=DIRECTION ( 'NONE',  ( -0.000000000000000000, -0.000000000000000000, 1.000000000000000000 ) ) ;
#39838=CARTESIAN_POINT ( 'NONE',  ( 7.070501591499376803E-16, 11.54700538379251284, -162.1250000000000284 ) ) ;
#39841=CARTESIAN_POINT ( 'NONE',  ( -10.81189881249999729, 6.242252689847871849, -33.71875000204835260 ) ) ;
#39842=CARTESIAN_POINT ( 'NONE',  ( 10.81189881249999551, -6.242252689847874514, -18.15625000204837036 ) ) ;
#39843=CARTESIAN_POINT ( 'NONE',  ( -5.405949406250003975, -9.363379034771801557, -73.84375000204838102 ) ) ;
#39845=CARTESIAN_POINT ( 'NONE',  ( 5.405949406249992428, -9.363379034771808662, -195.0937500020484094 ) ) ;
#39846=CARTESIAN_POINT ( 'NONE',  ( -5.405949406250003975, -9.363379034771801557, -151.8437500020483810 ) ) ;
#39847=CARTESIAN_POINT ( 'NONE',  ( -2.121150477449813534E-15, -11.54700538379251284, -79.25000000409677625 ) ) ;
#39850=CARTESIAN_POINT ( 'NONE',  ( 10.00000000000000000, 5.773502691896255534, -6.750000004096744277 ) ) ;
#39851=CARTESIAN_POINT ( 'NONE',  ( -2.121150477449813534E-15, -11.54700538379251284, -103.2500000040967763 ) ) ;
#39852=CARTESIAN_POINT ( 'NONE',  ( -10.81189881249999729, 6.242252689847871849, -122.2187500020483810 ) ) ;
#39853=LINE ( 'NONE', #10707, #12805 ) ;
#39854=CARTESIAN_POINT ( 'NONE',  ( -10.81189881249999729, 6.242252689847871849, -90.90625000204838102 ) ) ;
#39855=CARTESIAN_POINT ( 'NONE',  ( 10.81189881249999551, -6.242252689847874514, -106.4687500020483810 ) ) ;
#39858=CARTESIAN_POINT ( 'NONE',  ( 4.999999999999992006, -8.660254037844389075, -161.6250000040967905 ) ) ;
#39862=CYLINDRICAL_SURFACE ( 'NONE', #28432, 9.999999999999998224 ) ;
#39866=CARTESIAN_POINT ( 'NONE',  ( 9.999999999999998224, 0.000000000000000000, -81.49999999999998579 ) ) ;
#39868=CARTESIAN_POINT ( 'NONE',  ( 9.999999999999998224, 0.000000000000000000, -86.37500000409677625 ) ) ;
#39869=CARTESIAN_POINT ( 'NONE',  ( 9.999999999999998224, 0.000000000000000000, -107.3750000040967763 ) ) ;
#39871=CARTESIAN_POINT ( 'NONE',  ( 10.81189881249999729, 6.242252689847867408, -86.90625000204836681 ) ) ;
#39873=( BOUNDED_CURVE ( )  B_SPLINE_CURVE ( 2, ( #7622, #41039, #11482, #40828, #24684, #20557, #14062 ),
 .UNSPECIFIED., .F., .F. ) 
 B_SPLINE_CURVE_WITH_KNOTS ( ( 3, 2, 2, 3 ),
 ( 0.4701492537313434195, 0.4713930348258707492, 0.4726368159203981900, 0.4738805970149255198 ),
 .UNSPECIFIED. ) 
 CURVE ( )  GEOMETRIC_REPRESENTATION_ITEM ( )  RATIONAL_B_SPLINE_CURVE ( ( 0.9999999999999880096, 0.8660254037844506980, 1.000000000000000000, 0.8660254037844387076, 1.000000000000000000, 0.8660254037844207220, 1.000000000000017986 ) ) 
 REPRESENTATION_ITEM ( '' )  );
#39877=ORIENTED_EDGE ( 'NONE', *, *, #7199, .F. ) ;
#39878=CARTESIAN_POINT ( 'NONE',  ( 9.999999999999998224, 0.000000000000000000, -9.499999999999953815 ) ) ;
#39879=CARTESIAN_POINT ( 'NONE',  ( -4.999999999999996447, 8.660254037844387298, -142.5000000000000000 ) ) ;
#39880=CARTESIAN_POINT ( 'NONE',  ( -9.999999999998969713, -5.773502691896847949, -15.00000000409674072 ) ) ;
#39883=CARTESIAN_POINT ( 'NONE',  ( -5.000000000000003553, -8.660254037844383745, -191.5000000000000000 ) ) ;
#39884=ADVANCED_FACE ( 'NONE', ( #2965 ), #26264, .T. ) ;
#39885=CARTESIAN_POINT ( 'NONE',  ( -9.999999999999998224, 1.224646799147353059E-15, -95.74999999999998579 ) ) ;
#39886=CARTESIAN_POINT ( 'NONE',  ( -5.405949406249996869, 9.363379034771805109, -115.0312500020483952 ) ) ;
#39887=ORIENTED_EDGE ( 'NONE', *, *, #35386, .F. ) ;
#39889=EDGE_CURVE ( 'NONE', #19247, #13498, #28931, .T. ) ;
#39891=ORIENTED_EDGE ( 'NONE', *, *, #33336, .T. ) ;
#39892=EDGE_CURVE ( 'NONE', #36657, #23120, #36345, .T. ) ;
#39893=CARTESIAN_POINT ( 'NONE',  ( -10.81189881249999729, 6.242252689847871849, -44.40625000204836681 ) ) ;
#39895=CARTESIAN_POINT ( 'NONE',  ( -10.81189881249999729, 6.242252689847871849, -95.21875000204838102 ) ) ;
#39896=CARTESIAN_POINT ( 'NONE',  ( 5.405949406249999534, 9.363379034771803333, -125.7812500020483668 ) ) ;
#39898=CARTESIAN_POINT ( 'NONE',  ( 9.999999999998969713, 5.773502691896851502, -51.75000000409674783 ) ) ;
#39901=DIRECTION ( 'NONE',  ( -0.000000000000000000, -0.000000000000000000, 1.000000000000000000 ) ) ;
#39902=ADVANCED_FACE ( 'NONE', ( #6414 ), #32118, .T. ) ;
#39903=CARTESIAN_POINT ( 'NONE',  ( -5.405949406250003975, -9.363379034771801557, -132.3437500020484094 ) ) ;
#39905=LINE ( 'NONE', #7537, #3573 ) ;
#39907=CARTESIAN_POINT ( 'NONE',  ( -10.00000000000000000, -5.773502691896251982, -183.0000000040967905 ) ) ;
#39909=CARTESIAN_POINT ( 'NONE',  ( -5.405949406250003975, -9.363379034771801557, -179.0312500020483810 ) ) ;
#39913=EDGE_CURVE ( 'NONE', #7881, #36957, #12439, .T. ) ;
#39914=CARTESIAN_POINT ( 'NONE',  ( -5.405949406249996869, 9.363379034771805109, -62.34375000204836681 ) ) ;
#39915=CARTESIAN_POINT ( 'NONE',  ( -2.293366432827344421E-15, -12.48450537969573659, -40.71875000204835260 ) ) ;
#39917=CARTESIAN_POINT ( 'NONE',  ( 5.405949406249992428, -9.363379034771808662, -21.28125000204836326 ) ) ;
#39921=CARTESIAN_POINT ( 'NONE',  ( 10.00000000000000000, 5.773502691896255534, -103.8750000000000000 ) ) ;
#39923=EDGE_CURVE ( 'NONE', #39570, #40457, #31707, .T. ) ;
#39927=CARTESIAN_POINT ( 'NONE',  ( 5.405949406249992428, -9.363379034771808662, -108.2812500020483810 ) ) ;
#39933=ORIENTED_EDGE ( 'NONE', *, *, #17095, .F. ) ;
#39934=CARTESIAN_POINT ( 'NONE',  ( 9.999999999999996447, -5.773502691896262640, -30.62499999999995381 ) ) ;
#39935=CARTESIAN_POINT ( 'NONE',  ( 10.81189881249999551, -6.242252689847874514, -36.15625000204835970 ) ) ;
#39937=CARTESIAN_POINT ( 'NONE',  ( 5.405949406249999534, 9.363379034771803333, -142.2812500020483810 ) ) ;
#39939=ORIENTED_EDGE ( 'NONE', *, *, #37085, .T. ) ;
#39940=EDGE_CURVE ( 'NONE', #8113, #7578, #29083, .T. ) ;
#39942=EDGE_CURVE ( 'NONE', #31108, #41855, #20086, .T. ) ;
#39945=FACE_OUTER_BOUND ( 'NONE', #32227, .T. ) ;
#39946=CARTESIAN_POINT ( 'NONE',  ( -5.405949406250003975, -9.363379034771801557, -168.3437500020484094 ) ) ;
#39948=CARTESIAN_POINT ( 'NONE',  ( 5.405949406249999534, 9.363379034771803333, -22.09375000204835615 ) ) ;
#39951=CARTESIAN_POINT ( 'NONE',  ( -10.81189881249999729, 1.324075727343319199E-15, -155.0937500020483810 ) ) ;
#39952=CARTESIAN_POINT ( 'NONE',  ( 10.81189881249999907, 6.242252689847868297, -140.7187500020483810 ) ) ;
#39954=CARTESIAN_POINT ( 'NONE',  ( -5.000000000000003553, -8.660254037844383745, -8.875000004096744277 ) ) ;
#39958=CARTESIAN_POINT ( 'NONE',  ( -5.405949406249996869, 9.363379034771805109, -8.343750002048345493 ) ) ;
#39960=ADVANCED_FACE ( 'NONE', ( #5780 ), #22814, .T. ) ;
#39962=CARTESIAN_POINT ( 'NONE',  ( 9.999999999998969713, 5.773502691896851502, -5.250000004096743389 ) ) ;
#39964=LINE ( 'NONE', #39325, #14978 ) ;
#39965=CARTESIAN_POINT ( 'NONE',  ( 5.405949406249999534, 9.363379034771803333, -86.59375000204836681 ) ) ;
#39966=CARTESIAN_POINT ( 'NONE',  ( -2.293366432827344421E-15, -12.48450537969573659, -64.71875000204838102 ) ) ;
#39967=CARTESIAN_POINT ( 'NONE',  ( 5.405949406249992428, -9.363379034771808662, -40.78125000204838102 ) ) ;
#39969=CARTESIAN_POINT ( 'NONE',  ( 4.999999999999992006, -8.660254037844389075, -139.1250000040967905 ) ) ;
#39971=CARTESIAN_POINT ( 'NONE',  ( -4.999999999999996447, 8.660254037844387298, -130.5000000000000000 ) ) ;
#39972=CARTESIAN_POINT ( 'NONE',  ( 5.405949406249999534, 9.363379034771803333, -137.7812500020483810 ) ) ;
#39975=CARTESIAN_POINT ( 'NONE',  ( -5.405949406249996869, 9.363379034771805109, -20.53125000204836326 ) ) ;
#39976=VERTEX_POINT ( 'NONE', #5993 ) ;
#39981=CARTESIAN_POINT ( 'NONE',  ( -5.000000000000003553, -8.660254037844383745, -43.37500000409677625 ) ) ;
#39984=CARTESIAN_POINT ( 'NONE',  ( 7.644554776091147741E-16, 12.48450537969573659, -158.6562500020484094 ) ) ;
#39985=CARTESIAN_POINT ( 'NONE',  ( -10.81189881249999907, -6.242252689847864744, -138.4687500020484094 ) ) ;
#39987=CARTESIAN_POINT ( 'NONE',  ( 7.070501591499376803E-16, 11.54700538379251284, -151.6250000000000000 ) ) ;
#39988=ORIENTED_EDGE ( 'NONE', *, *, #7202, .T. ) ;
#39989=CARTESIAN_POINT ( 'NONE',  ( 4.999999999999992006, -8.660254037844389075, -78.74999999999998579 ) ) ;
#39990=CARTESIAN_POINT ( 'NONE',  ( -2.293366432827344421E-15, -12.48450537969573659, -64.90625000204838102 ) ) ;
#39991=ORIENTED_EDGE ( 'NONE', *, *, #28811, .F. ) ;
#39993=CARTESIAN_POINT ( 'NONE',  ( 10.81189881249999907, 6.242252689847868297, -121.2187500020483952 ) ) ;
#39994=ORIENTED_EDGE ( 'NONE', *, *, #20835, .T. ) ;
#39995=CARTESIAN_POINT ( 'NONE',  ( 5.405949406249992428, -9.363379034771808662, -21.09375000204835615 ) ) ;
#39997=CARTESIAN_POINT ( 'NONE',  ( 5.405949406249992428, -9.363379034771808662, -195.0937500020484094 ) ) ;
#39998=AXIS2_PLACEMENT_3D ( 'NONE', #24743, #11112, #37889 ) ;
#39999=CARTESIAN_POINT ( 'NONE',  ( -10.81189881249999729, 1.324075727343319199E-15, -50.09375000204835260 ) ) ;
#40000=EDGE_CURVE ( 'NONE', #9954, #26056, #24519, .T. ) ;
#40002=CYLINDRICAL_SURFACE ( 'NONE', #39685, 9.999999999999998224 ) ;
#40004=CARTESIAN_POINT ( 'NONE',  ( -5.405949406249996869, 9.363379034771805109, -180.8437500020483810 ) ) ;
#40005=CARTESIAN_POINT ( 'NONE',  ( -10.81189881249999729, 1.324075727343319199E-15, -158.0937500020483810 ) ) ;
#40009=( BOUNDED_CURVE ( )  B_SPLINE_CURVE ( 2, ( #13487, #12856, #20194, #13064, #26676, #13275, #26259 ),
 .UNSPECIFIED., .F., .F. ) 
 B_SPLINE_CURVE_WITH_KNOTS ( ( 3, 2, 2, 3 ),
 ( 0.1305970149253731227, 0.1318407960199005080, 0.1330845771144278378, 0.1343283582089551953 ),
 .UNSPECIFIED. ) 
 CURVE ( )  GEOMETRIC_REPRESENTATION_ITEM ( )  RATIONAL_B_SPLINE_CURVE ( ( 1.000000000000000000, 0.8660254037844387076, 1.000000000000000000, 0.8660254037844387076, 1.000000000000000000, 0.8660254037844417052, 0.9999999999999970024 ) ) 
 REPRESENTATION_ITEM ( '' )  );
#40010=CARTESIAN_POINT ( 'NONE',  ( -9.999999999999998224, 1.224646799147353059E-15, -187.6250000040967905 ) ) ;
#40012=CARTESIAN_POINT ( 'NONE',  ( 10.81189881249999729, 0.000000000000000000, -97.34375000204838102 ) ) ;
#40013=CARTESIAN_POINT ( 'NONE',  ( 0.000000000000000000, 0.000000000000000000, -200.0000000000000000 ) ) ;
#40014=CARTESIAN_POINT ( 'NONE',  ( -2.293366432827344421E-15, -12.48450537969573659, -67.90625000204840944 ) ) ;
#40015=CARTESIAN_POINT ( 'NONE',  ( -2.121150477449813534E-15, -11.54700538379251284, -97.25000000409677625 ) ) ;
#40017=CARTESIAN_POINT ( 'NONE',  ( 5.405949406249992428, -9.363379034771808662, -118.7812500020483952 ) ) ;
#40018=CARTESIAN_POINT ( 'NONE',  ( -10.81189881249999729, 6.242252689847871849, -162.9062500020483810 ) ) ;
#40020=CARTESIAN_POINT ( 'NONE',  ( -2.121150477449813534E-15, -11.54700538379251284, -140.7500000040967905 ) ) ;
#40022=EDGE_CURVE ( 'NONE', #18615, #40773, #37028, .T. ) ;
#40023=VERTEX_POINT ( 'NONE', #36395 ) ;
#40026=CARTESIAN_POINT ( 'NONE',  ( 10.81189881249999551, -6.242252689847874514, -192.1562500020484094 ) ) ;
#40029=CARTESIAN_POINT ( 'NONE',  ( 9.999999999999996447, -5.773502691896262640, -50.12499999999998579 ) ) ;
#40031=CARTESIAN_POINT ( 'NONE',  ( 9.999999999999998224, 0.000000000000000000, -66.87500000409676204 ) ) ;
#40032=CARTESIAN_POINT ( 'NONE',  ( -9.999999999999998224, 1.224646799147353059E-15, -101.7500000000000000 ) ) ;
#40035=CARTESIAN_POINT ( 'NONE',  ( 5.405949406249999534, 9.363379034771803333, -56.78125000204836681 ) ) ;
#40038=CARTESIAN_POINT ( 'NONE',  ( 0.000000000000000000, 0.000000000000000000, -200.0000000000000000 ) ) ;
#40039=CARTESIAN_POINT ( 'NONE',  ( -10.81189881249999729, 1.324075727343319199E-15, -186.7812500020484094 ) ) ;
#40041=CARTESIAN_POINT ( 'NONE',  ( -10.81189881249999729, 1.324075727343319199E-15, -0.5937500020483654772 ) ) ;
#40042=DIRECTION ( 'NONE',  ( -0.08715574274765837404, 0.000000000000000000, -0.9961946980917455452 ) ) ;
#40044=CARTESIAN_POINT ( 'NONE',  ( -2.121150477449813534E-15, -11.54700538379251284, -122.3749999999999858 ) ) ;
#40045=CARTESIAN_POINT ( 'NONE',  ( -2.293366432827344421E-15, -12.48450537969573659, -90.40625000204838102 ) ) ;
#40049=ORIENTED_EDGE ( 'NONE', *, *, #15782, .T. ) ;
#40051=EDGE_CURVE ( 'NONE', #14981, #311, #27265, .T. ) ;
#40052=CARTESIAN_POINT ( 'NONE',  ( 10.81189881249999551, -6.242252689847874514, -29.96875000204834549 ) ) ;
#40053=CARTESIAN_POINT ( 'NONE',  ( -10.81189881249999729, 6.242252689847871849, -23.40625000204837747 ) ) ;
#40055=CARTESIAN_POINT ( 'NONE',  ( 5.405949406249999534, 9.363379034771803333, -74.59375000204838102 ) ) ;
#40058=CARTESIAN_POINT ( 'NONE',  ( 10.81189881249999551, -6.242252689847874514, -191.9687500020484379 ) ) ;
#40059=CARTESIAN_POINT ( 'NONE',  ( -10.81189881249999729, 6.242252689847871849, -147.7187500020484094 ) ) ;
#40063=CARTESIAN_POINT ( 'NONE',  ( 9.999999999999996447, -5.773502691896262640, -2.500000004096755823 ) ) ;
#40064=LINE ( 'NONE', #10496, #14280 ) ;
#40066=CARTESIAN_POINT ( 'NONE',  ( 7.644554776091147741E-16, 12.48450537969573659, -120.9687500020483952 ) ) ;
#40067=CYLINDRICAL_SURFACE ( 'NONE', #20390, 9.999999999999998224 ) ;
#40068=CARTESIAN_POINT ( 'NONE',  ( -10.81189881249999729, 6.242252689847871849, -89.40625000204838102 ) ) ;
#40069=CARTESIAN_POINT ( 'NONE',  ( -10.81189881249999729, 6.242252689847871849, -99.71875000204838102 ) ) ;
#40070=EDGE_CURVE ( 'NONE', #18513, #24472, #789, .T. ) ;
#40073=CARTESIAN_POINT ( 'NONE',  ( 7.070501591499377789E-16, 11.54700538379251284, -161.0000000040967905 ) ) ;
#40076=CARTESIAN_POINT ( 'NONE',  ( -9.999999999999998224, 1.224646799147353059E-15, -184.2500000000000000 ) ) ;
#40078=CARTESIAN_POINT ( 'NONE',  ( 9.999999999999998224, 0.000000000000000000, -195.5000000000000000 ) ) ;
#40080=CARTESIAN_POINT ( 'NONE',  ( 9.999999999999996447, -5.773502691896262640, -83.12499999999998579 ) ) ;
#40082=CARTESIAN_POINT ( 'NONE',  ( -4.999999999999996447, 8.660254037844387298, -87.37500000409677625 ) ) ;
#40083=( BOUNDED_CURVE ( )  B_SPLINE_CURVE ( 2, ( #26137, #9723, #33, #19858, #26562, #26349, #10146 ),
 .UNSPECIFIED., .F., .F. ) 
 B_SPLINE_CURVE_WITH_KNOTS ( ( 3, 2, 2, 3 ),
 ( 0.8544776119402988090, 0.8557213930348261943, 0.8569651741293534686, 0.8582089552238808539 ),
 .UNSPECIFIED. ) 
 CURVE ( )  GEOMETRIC_REPRESENTATION_ITEM ( )  RATIONAL_B_SPLINE_CURVE ( ( 0.9999999999999641398, 0.8660254037844745678, 1.000000000000000000, 0.8660254037844387076, 1.000000000000000000, 0.8660254037844148378, 1.000000000000023981 ) ) 
 REPRESENTATION_ITEM ( '' )  );
#40084=CYLINDRICAL_SURFACE ( 'NONE', #38934, 9.999999999999998224 ) ;
#40086=CARTESIAN_POINT ( 'NONE',  ( 7.644554776091147741E-16, 12.48450537969573659, -80.65625000204838102 ) ) ;
#40090=ORIENTED_EDGE ( 'NONE', *, *, #3754, .F. ) ;
#40091=CARTESIAN_POINT ( 'NONE',  ( 9.999999999999998224, 0.000000000000000000, -12.49999999999995559 ) ) ;
#40093=CARTESIAN_POINT ( 'NONE',  ( -9.999999999999998224, 5.773502691896259087, -148.3750000000000000 ) ) ;
#40094=CARTESIAN_POINT ( 'NONE',  ( -11.54700538379251817, 20.00000000000000355, 0.000000000000000000 ) ) ;
#40097=CARTESIAN_POINT ( 'NONE',  ( -2.121150477449813534E-15, -11.54700538379251284, -194.3750000000000284 ) ) ;
#40099=CARTESIAN_POINT ( 'NONE',  ( 10.81189881249999729, 0.000000000000000000, -118.5312500020483952 ) ) ;
#40100=ORIENTED_EDGE ( 'NONE', *, *, #31744, .F. ) ;
#40101=CARTESIAN_POINT ( 'NONE',  ( 5.000000000000000000, 8.660254037844385522, -13.74999999999995737 ) ) ;
#40103=ORIENTED_EDGE ( 'NONE', *, *, #5361, .F. ) ;
#40104=CARTESIAN_POINT ( 'NONE',  ( 10.81189881249999729, 0.000000000000000000, -49.53125000204838813 ) ) ;
#40106=CARTESIAN_POINT ( 'NONE',  ( -5.405949406249996869, 9.363379034771805109, -92.34375000204838102 ) ) ;
#40107=CARTESIAN_POINT ( 'NONE',  ( 5.405949406249999534, 9.363379034771803333, -119.7812500020483952 ) ) ;
#40109=CARTESIAN_POINT ( 'NONE',  ( 5.405949406249992428, -9.363379034771808662, -196.5937500020484094 ) ) ;
#40112=CARTESIAN_POINT ( 'NONE',  ( -5.405949406249996869, 9.363379034771805109, -120.8437500020483952 ) ) ;
#40116=CARTESIAN_POINT ( 'NONE',  ( -5.000000000000003553, -8.660254037844383745, -182.8750000040967905 ) ) ;
#40118=VECTOR ( 'NONE', #7287, 1000.000000000000000 ) ;
#40119=CARTESIAN_POINT ( 'NONE',  ( -2.293366432827344421E-15, -12.48450537969573659, -180.4062500020484379 ) ) ;
#40124=CARTESIAN_POINT ( 'NONE',  ( -5.405949406250003975, -9.363379034771801557, -58.84375000204835970 ) ) ;
#40125=CARTESIAN_POINT ( 'NONE',  ( 10.81189881249999551, -6.242252689847874514, -40.46875000204835260 ) ) ;
#40127=CARTESIAN_POINT ( 'NONE',  ( 7.644554776091147741E-16, 12.48450537969573659, -16.15625000204837747 ) ) ;
#40131=EDGE_CURVE ( 'NONE', #12962, #41098, #38877, .T. ) ;
#40132=CARTESIAN_POINT ( 'NONE',  ( 5.000000000000000000, 8.660254037844385522, -105.2499999999999858 ) ) ;
#40134=DIRECTION ( 'NONE',  ( 0.000000000000000000, 0.000000000000000000, -1.000000000000000000 ) ) ;
#40135=EDGE_CURVE ( 'NONE', #40345, #6396, #4228, .T. ) ;
#40138=CARTESIAN_POINT ( 'NONE',  ( 10.81189881249999729, 6.242252689847867408, -109.4062500020483952 ) ) ;
#40139=ORIENTED_EDGE ( 'NONE', *, *, #34683, .F. ) ;
#40140=CARTESIAN_POINT ( 'NONE',  ( -2.121150477449813534E-15, -11.54700538379251284, -6.874999999999968914 ) ) ;
#40144=ORIENTED_EDGE ( 'NONE', *, *, #2158, .T. ) ;
#40145=CARTESIAN_POINT ( 'NONE',  ( -9.999999999999998224, 1.224646799147353059E-15, -37.24999999999997868 ) ) ;
#40147=CARTESIAN_POINT ( 'NONE',  ( -5.405949406249996869, 9.363379034771805109, -35.53125000204837391 ) ) ;
#40149=CARTESIAN_POINT ( 'NONE',  ( 7.070501591499376803E-16, 11.54700538379251284, -161.0000000040968189 ) ) ;
#40150=CARTESIAN_POINT ( 'NONE',  ( -10.81189881249999729, 1.324075727343319199E-15, -140.2812500020483810 ) ) ;
#40151=CARTESIAN_POINT ( 'NONE',  ( 9.999999999999479527, 5.773502691896553074, -174.7500000040967905 ) ) ;
#40154=CARTESIAN_POINT ( 'NONE',  ( -9.999999999999998224, 1.224646799147353059E-15, -113.7499999999999858 ) ) ;
#40156=CARTESIAN_POINT ( 'NONE',  ( 5.405949406249992428, -9.363379034771808662, -168.0937500020484094 ) ) ;
#40158=CARTESIAN_POINT ( 'NONE',  ( -10.81189881249999907, -6.242252689847864744, -15.46875000204835793 ) ) ;
#40159=CARTESIAN_POINT ( 'NONE',  ( 9.999999999999998224, 0.000000000000000000, -62.37500000409676204 ) ) ;
#40160=CARTESIAN_POINT ( 'NONE',  ( 10.81189881249999729, 0.000000000000000000, -157.3437500020483810 ) ) ;
#40161=CARTESIAN_POINT ( 'NONE',  ( 5.405949406249992428, -9.363379034771808662, -136.5937500020483810 ) ) ;
#40162=CARTESIAN_POINT ( 'NONE',  ( -4.999999999999996447, 8.660254037844387298, -67.49999999999997158 ) ) ;
#40166=CARTESIAN_POINT ( 'NONE',  ( -10.81189881249999907, -6.242252689847864744, -12.46875000204837391 ) ) ;
#40168=CARTESIAN_POINT ( 'NONE',  ( 7.644554776091147741E-16, 12.48450537969573659, -199.1562500020484379 ) ) ;
#40169=CARTESIAN_POINT ( 'NONE',  ( -9.999999999999998224, 1.224646799147353059E-15, -97.24999999999998579 ) ) ;
#40172=CARTESIAN_POINT ( 'NONE',  ( 5.405949406249992428, -9.363379034771808662, -85.59375000204836681 ) ) ;
#40173=CARTESIAN_POINT ( 'NONE',  ( 7.644554776091147741E-16, 12.48450537969573659, -66.96875000204838102 ) ) ;
#40174=CARTESIAN_POINT ( 'NONE',  ( -2.293366432827344421E-15, -12.48450537969573659, -45.40625000204837391 ) ) ;
#40176=FACE_OUTER_BOUND ( 'NONE', #6517, .T. ) ;
#40178=ADVANCED_FACE ( 'NONE', ( #30570 ), #27320, .T. ) ;
#40179=CARTESIAN_POINT ( 'NONE',  ( 7.070501591499377789E-16, 11.54700538379251284, -129.1250000000000000 ) ) ;
#40180=CARTESIAN_POINT ( 'NONE',  ( -5.405949406250003975, -9.363379034771801557, -129.5312500020484094 ) ) ;
#40183=CARTESIAN_POINT ( 'NONE',  ( -5.405949406250003975, -9.363379034771801557, -17.03125000204835970 ) ) ;
#40189=EDGE_CURVE ( 'NONE', #29348, #23986, #27534, .T. ) ;
#40190=CARTESIAN_POINT ( 'NONE',  ( 9.999999999999996447, -5.773502691896262640, -41.50000000409674783 ) ) ;
#40191=CARTESIAN_POINT ( 'NONE',  ( 9.999999999999998224, 0.000000000000000000, -68.37500000409677625 ) ) ;
#40194=CARTESIAN_POINT ( 'NONE',  ( -9.999999999999998224, 1.224646799147353059E-15, -76.24999999999998579 ) ) ;
#40195=CARTESIAN_POINT ( 'NONE',  ( 10.81189881249999907, 6.242252689847868297, -149.9062500020484094 ) ) ;
#40196=CARTESIAN_POINT ( 'NONE',  ( 10.81189881249999907, 6.242252689847868297, -139.2187500020484094 ) ) ;
#40197=CARTESIAN_POINT ( 'NONE',  ( 9.999999999999998224, 0.000000000000000000, -195.5000000000000000 ) ) ;
#40198=ADVANCED_FACE ( 'NONE', ( #7047 ), #3809, .T. ) ;
#40200=DIRECTION ( 'NONE',  ( -0.000000000000000000, -0.000000000000000000, 1.000000000000000000 ) ) ;
#40201=CARTESIAN_POINT ( 'NONE',  ( -10.81189881249999907, -6.242252689847864744, -60.65625000204840234 ) ) ;
#40202=ORIENTED_EDGE ( 'NONE', *, *, #33406, .T. ) ;
#40204=CARTESIAN_POINT ( 'NONE',  ( 10.81189881249999907, 6.242252689847868297, -115.2187500020483810 ) ) ;
#40205=ORIENTED_EDGE ( 'NONE', *, *, #18829, .T. ) ;
#40206=( BOUNDED_CURVE ( )  B_SPLINE_CURVE ( 2, ( #27741, #10678, #41086, #17793, #11529, #30990, #23871 ),
 .UNSPECIFIED., .F., .F. ) 
 B_SPLINE_CURVE_WITH_KNOTS ( ( 3, 2, 2, 3 ),
 ( 0.8395522388059704078, 0.8407960199004976820, 0.8420398009950251783, 0.8432835820895525636 ),
 .UNSPECIFIED. ) 
 CURVE ( )  GEOMETRIC_REPRESENTATION_ITEM ( )  RATIONAL_B_SPLINE_CURVE ( ( 0.9999999999999761302, 0.8660254037844625774, 1.000000000000000000, 0.8660254037844387076, 1.000000000000000000, 0.8660254037844028474, 1.000000000000035971 ) ) 
 REPRESENTATION_ITEM ( '' )  );
#40207=CARTESIAN_POINT ( 'NONE',  ( 5.405949406249999534, 9.363379034771803333, -20.59375000204835615 ) ) ;
#40208=CARTESIAN_POINT ( 'NONE',  ( -2.293366432827344421E-15, -12.48450537969573659, -193.7187500020484094 ) ) ;
#40209=CARTESIAN_POINT ( 'NONE',  ( 5.405949406249999534, 9.363379034771803333, -47.59375000204838102 ) ) ;
#40210=CARTESIAN_POINT ( 'NONE',  ( 10.81189881249999729, 0.000000000000000000, -181.3437500020483810 ) ) ;
#40211=CARTESIAN_POINT ( 'NONE',  ( 5.405949406249992428, -9.363379034771808662, -162.0937500020484094 ) ) ;
#40215=CARTESIAN_POINT ( 'NONE',  ( 0.000000000000000000, 0.000000000000000000, -200.0000000000000000 ) ) ;
#40217=CARTESIAN_POINT ( 'NONE',  ( -2.293366432827344421E-15, -12.48450537969573659, -88.71875000204838102 ) ) ;
#40219=CARTESIAN_POINT ( 'NONE',  ( -10.81189881249999729, 6.242252689847871849, -69.90625000204839523 ) ) ;
#40222=CARTESIAN_POINT ( 'NONE',  ( -10.81189881249999907, -6.242252689847864744, -123.6562500020484094 ) ) ;
#40223=CARTESIAN_POINT ( 'NONE',  ( -10.81189881249999729, 1.324075727343319199E-15, -165.7812500020484094 ) ) ;
#40225=CARTESIAN_POINT ( 'NONE',  ( 5.000000000000000000, 8.660254037844385522, -131.1250000040967620 ) ) ;
#40230=CARTESIAN_POINT ( 'NONE',  ( 5.405949406249992428, -9.363379034771808662, -186.2812500020484094 ) ) ;
#40232=ORIENTED_EDGE ( 'NONE', *, *, #38083, .F. ) ;
#40233=CARTESIAN_POINT ( 'NONE',  ( -9.999999999999998224, 1.224646799147353059E-15, -50.74999999999996447 ) ) ;
#40235=CARTESIAN_POINT ( 'NONE',  ( -2.121150477449813534E-15, -11.54700538379251284, -62.75000000409679046 ) ) ;
#40236=CARTESIAN_POINT ( 'NONE',  ( -9.999999999999998224, 1.224646799147353059E-15, -178.6250000040968189 ) ) ;
#40238=CARTESIAN_POINT ( 'NONE',  ( -5.405949406250003975, -9.363379034771801557, -59.03125000204836681 ) ) ;
#40241=CARTESIAN_POINT ( 'NONE',  ( -9.999999999999998224, 1.224646799147353059E-15, -88.24999999999998579 ) ) ;
#40242=CARTESIAN_POINT ( 'NONE',  ( 10.81189881249999551, -6.242252689847874514, -180.1562500020484379 ) ) ;
#40243=EDGE_CURVE ( 'NONE', #4916, #3061, #13698, .T. ) ;
#40246=CARTESIAN_POINT ( 'NONE',  ( 9.999999999999998224, 0.000000000000000000, -165.5000000000000000 ) ) ;
#40247=CARTESIAN_POINT ( 'NONE',  ( -4.999999999999996447, 8.660254037844387298, -154.5000000000000000 ) ) ;
#40248=CARTESIAN_POINT ( 'NONE',  ( 9.999999999999998224, 0.000000000000000000, -200.0000000000000000 ) ) ;
#40249=( BOUNDED_CURVE ( )  B_SPLINE_CURVE ( 2, ( #41080, #37658, #8098, #21249, #17998, #14757, #19078 ),
 .UNSPECIFIED., .F., .F. ) 
 B_SPLINE_CURVE_WITH_KNOTS ( ( 3, 2, 2, 3 ),
 ( 0.3134328358208955390, 0.3146766169154229242, 0.3159203980099503650, 0.3171641791044778058 ),
 .UNSPECIFIED. ) 
 CURVE ( )  GEOMETRIC_REPRESENTATION_ITEM ( )  RATIONAL_B_SPLINE_CURVE ( ( 1.000000000000000000, 0.8660254037844387076, 1.000000000000000000, 0.8660254037844387076, 1.000000000000000000, 0.8660254037844207220, 1.000000000000017986 ) ) 
 REPRESENTATION_ITEM ( '' )  );
#40251=CARTESIAN_POINT ( 'NONE',  ( -10.81189881249999907, -6.242252689847864744, -84.65625000204836681 ) ) ;
#40253=CARTESIAN_POINT ( 'NONE',  ( 7.070501591499376803E-16, 11.54700538379251284, -81.12500000000000000 ) ) ;
#40254=ORIENTED_EDGE ( 'NONE', *, *, #26163, .F. ) ;
#40256=CARTESIAN_POINT ( 'NONE',  ( -10.81189881249999729, 1.324075727343319199E-15, -26.09375000204835970 ) ) ;
#40257=CARTESIAN_POINT ( 'NONE',  ( 10.81189881249999551, -6.242252689847874514, -16.65625000204837747 ) ) ;
#40259=CARTESIAN_POINT ( 'NONE',  ( -10.81189881249999729, 1.324075727343319199E-15, -74.09375000204838102 ) ) ;
#40260=CARTESIAN_POINT ( 'NONE',  ( 9.999999999999998224, 0.000000000000000000, -164.3750000040967905 ) ) ;
#40262=CARTESIAN_POINT ( 'NONE',  ( 5.405949406249999534, 9.363379034771803333, -187.0937500020483810 ) ) ;
#40264=CARTESIAN_POINT ( 'NONE',  ( 5.000000000000000000, 8.660254037844385522, -175.7500000000000284 ) ) ;
#40265=LINE ( 'NONE', #4029, #8138 ) ;
#40268=DIRECTION ( 'NONE',  ( -0.000000000000000000, -0.000000000000000000, 1.000000000000000000 ) ) ;
#40269=CARTESIAN_POINT ( 'NONE',  ( 5.405949406249992428, -9.363379034771808662, -117.0937500020483810 ) ) ;
#40270=LINE ( 'NONE', #23904, #36937 ) ;
#40271=CARTESIAN_POINT ( 'NONE',  ( 7.644554776091147741E-16, 12.48450537969573659, -92.65625000204839523 ) ) ;
#40272=CARTESIAN_POINT ( 'NONE',  ( -5.405949406250003975, -9.363379034771801557, -96.34375000204838102 ) ) ;
#40275=CARTESIAN_POINT ( 'NONE',  ( -2.121150477449813534E-15, -11.54700538379251284, -164.7500000040967620 ) ) ;
#40281=CYLINDRICAL_SURFACE ( 'NONE', #40353, 9.999999999999998224 ) ;
#40282=CARTESIAN_POINT ( 'NONE',  ( 10.00000000000000000, 5.773502691896255534, -73.87499999999995737 ) ) ;
#40284=CARTESIAN_POINT ( 'NONE',  ( -10.00000000000000000, -5.773502691896251982, -91.50000000409677625 ) ) ;
#40285=CARTESIAN_POINT ( 'NONE',  ( 9.999999999999994671, -5.773502691896262640, -171.6250000000000000 ) ) ;
#40287=CARTESIAN_POINT ( 'NONE',  ( -5.405949406249996869, 9.363379034771805109, -83.53125000204838102 ) ) ;
#40289=CARTESIAN_POINT ( 'NONE',  ( 7.070501591499376803E-16, 11.54700538379251284, -21.12499999999997513 ) ) ;
#40291=ORIENTED_EDGE ( 'NONE', *, *, #42405, .T. ) ;
#40292=CARTESIAN_POINT ( 'NONE',  ( -2.121150477449813534E-15, -11.54700538379251284, -12.87499999999996447 ) ) ;
#40294=CARTESIAN_POINT ( 'NONE',  ( -10.81189881249999729, -6.242252689847864744, -9.468750002048361480 ) ) ;
#40296=CARTESIAN_POINT ( 'NONE',  ( 5.405949406249992428, -9.363379034771808662, -139.7812500020483810 ) ) ;
#40297=AXIS2_PLACEMENT_3D ( 'NONE', #31625, #7885, #1627 ) ;
#40298=CARTESIAN_POINT ( 'NONE',  ( -5.000000000000003553, -8.660254037844383745, -187.0000000000000000 ) ) ;
#40299=FACE_OUTER_BOUND ( 'NONE', #2055, .T. ) ;
#40300=CARTESIAN_POINT ( 'NONE',  ( 5.405949406249992428, -9.363379034771808662, -112.7812500020483952 ) ) ;
#40301=VERTEX_POINT ( 'NONE', #36814 ) ;
#40302=LINE ( 'NONE', #13337, #22805 ) ;
#40303=ORIENTED_EDGE ( 'NONE', *, *, #9375, .F. ) ;
#40304=ORIENTED_EDGE ( 'NONE', *, *, #17490, .F. ) ;
#40306=CARTESIAN_POINT ( 'NONE',  ( -5.405949406250003975, -9.363379034771801557, -45.53125000204838102 ) ) ;
#40308=CARTESIAN_POINT ( 'NONE',  ( 10.81189881249999729, 0.000000000000000000, -97.34375000204838102 ) ) ;
#40309=CARTESIAN_POINT ( 'NONE',  ( 4.999999999999992006, -8.660254037844389075, -167.2500000000000000 ) ) ;
#40310=CARTESIAN_POINT ( 'NONE',  ( -9.999999999999998224, 1.224646799147353059E-15, -19.24999999999996092 ) ) ;
#40312=CARTESIAN_POINT ( 'NONE',  ( 5.405949406249992428, -9.363379034771808662, -193.5937500020484094 ) ) ;
#40314=CARTESIAN_POINT ( 'NONE',  ( 9.999999999999998224, 0.000000000000000000, -138.5000000000000000 ) ) ;
#40315=CARTESIAN_POINT ( 'NONE',  ( 10.81189881249999729, 6.242252689847867408, -125.7187500020483810 ) ) ;
#40316=( BOUNDED_CURVE ( )  B_SPLINE_CURVE ( 2, ( #8829, #21775, #1935, #8619, #35163, #5163, #41820 ),
 .UNSPECIFIED., .F., .F. ) 
 B_SPLINE_CURVE_WITH_KNOTS ( ( 3, 2, 2, 3 ),
 ( 0.4776119402985076756, 0.4788557213930350054, 0.4800995024875623352, 0.4813432835820896649 ),
 .UNSPECIFIED. ) 
 CURVE ( )  GEOMETRIC_REPRESENTATION_ITEM ( )  RATIONAL_B_SPLINE_CURVE ( ( 0.9999999999999761302, 0.8660254037844625774, 1.000000000000000000, 0.8660254037844387076, 1.000000000000000000, 0.8660254037844267172, 1.000000000000011990 ) ) 
 REPRESENTATION_ITEM ( '' )  );
#40318=FACE_OUTER_BOUND ( 'NONE', #8278, .T. ) ;
#40320=CARTESIAN_POINT ( 'NONE',  ( -9.999999999999998224, 1.224646799147353059E-15, -187.6250000040967905 ) ) ;
#40322=CARTESIAN_POINT ( 'NONE',  ( 10.81189881249999729, 6.242252689847867408, -178.4062500020484094 ) ) ;
#40324=CARTESIAN_POINT ( 'NONE',  ( 9.999999999999612754, 5.773502691896477579, -180.3750000000000000 ) ) ;
#40327=CARTESIAN_POINT ( 'NONE',  ( -2.293366432827344421E-15, -12.48450537969573659, -55.71875000204837391 ) ) ;
#40328=CARTESIAN_POINT ( 'NONE',  ( 5.405949406249999534, 9.363379034771803333, -38.59375000204837391 ) ) ;
#40330=CARTESIAN_POINT ( 'NONE',  ( 10.81189881249999729, 0.000000000000000000, -7.531250002048350822 ) ) ;
#40334=CARTESIAN_POINT ( 'NONE',  ( -9.999999999999998224, 1.224646799147353059E-15, -95.74999999999998579 ) ) ;
#40339=CARTESIAN_POINT ( 'NONE',  ( 10.81189881249999551, -6.242252689847874514, -105.1562500020483810 ) ) ;
#40341=CARTESIAN_POINT ( 'NONE',  ( -9.999999999999998224, 1.224646799147353059E-15, -200.0000000000000000 ) ) ;
#40343=CARTESIAN_POINT ( 'NONE',  ( -9.999999999999872102, -5.773502691896326589, -166.5000000040967905 ) ) ;
#40345=VERTEX_POINT ( 'NONE', #17579 ) ;
#40346=CARTESIAN_POINT ( 'NONE',  ( -4.999999999999996447, 8.660254037844387298, -34.49999999999997158 ) ) ;
#40347=CARTESIAN_POINT ( 'NONE',  ( -10.81189881249999729, -6.242252689847864744, -33.65625000204836681 ) ) ;
#40348=CARTESIAN_POINT ( 'NONE',  ( 9.999999999999998224, 0.000000000000000000, -1.999999999999973799 ) ) ;
#40350=VECTOR ( 'NONE', #30466, 1000.000000000000000 ) ;
#40352=CARTESIAN_POINT ( 'NONE',  ( -2.293366432827344421E-15, -12.48450537969573659, -138.4062500020483810 ) ) ;
#40353=AXIS2_PLACEMENT_3D ( 'NONE', #37059, #21082, #13945 ) ;
#40354=CARTESIAN_POINT ( 'NONE',  ( 7.070501591499376803E-16, 11.54700538379251284, -162.5000000040967905 ) ) ;
#40356=EDGE_CURVE ( 'NONE', #42118, #2342, #17049, .T. ) ;
#40357=ORIENTED_EDGE ( 'NONE', *, *, #486, .F. ) ;
#40358=CARTESIAN_POINT ( 'NONE',  ( 0.000000000000000000, 0.000000000000000000, -200.0000000000000000 ) ) ;
#40360=CARTESIAN_POINT ( 'NONE',  ( 10.81189881249999907, 6.242252689847868297, -167.7187500020483810 ) ) ;
#40362=CARTESIAN_POINT ( 'NONE',  ( 10.81189881249999907, 6.242252689847868297, -13.21875000204836148 ) ) ;
#40363=CARTESIAN_POINT ( 'NONE',  ( 0.000000000000000000, 0.000000000000000000, -200.0000000000000000 ) ) ;
#40364=CARTESIAN_POINT ( 'NONE',  ( -10.81189881249999729, 6.242252689847871849, -147.7187500020484094 ) ) ;
#40365=CARTESIAN_POINT ( 'NONE',  ( 7.644554776091147741E-16, 12.48450537969573659, -140.4687500020483810 ) ) ;
#40366=CARTESIAN_POINT ( 'NONE',  ( -5.405949406250003975, -9.363379034771801557, -102.5312500020483952 ) ) ;
#40370=CARTESIAN_POINT ( 'NONE',  ( 10.81189881249999907, 6.242252689847868297, -10.21875000204836326 ) ) ;
#40372=DIRECTION ( 'NONE',  ( -0.000000000000000000, -0.000000000000000000, 1.000000000000000000 ) ) ;
#40375=CARTESIAN_POINT ( 'NONE',  ( -5.405949406249996869, 9.363379034771805109, -86.34375000204836681 ) ) ;
#40376=CARTESIAN_POINT ( 'NONE',  ( 7.644554776091147741E-16, 12.48450537969573659, -62.46875000204839523 ) ) ;
#40378=CARTESIAN_POINT ( 'NONE',  ( 10.81189881249999551, -6.242252689847874514, -33.15625000204835970 ) ) ;
#40380=DIRECTION ( 'NONE',  ( -0.000000000000000000, -0.000000000000000000, 1.000000000000000000 ) ) ;
#40382=CARTESIAN_POINT ( 'NONE',  ( 4.999999999999992006, -8.660254037844389075, -128.2499999999999716 ) ) ;
#40383=CARTESIAN_POINT ( 'NONE',  ( 7.644554776091147741E-16, 12.48450537969573659, -130.1562500020483810 ) ) ;
#40385=CARTESIAN_POINT ( 'NONE',  ( 5.405949406249999534, 9.363379034771803333, -19.28125000204835970 ) ) ;
#40389=CARTESIAN_POINT ( 'NONE',  ( -9.999999999999998224, 1.224646799147353059E-15, -30.12500000409676204 ) ) ;
#40390=FACE_OUTER_BOUND ( 'NONE', #17351, .T. ) ;
#40392=CARTESIAN_POINT ( 'NONE',  ( 4.999999999999992006, -8.660254037844389075, -146.2500000000000000 ) ) ;
#40393=CARTESIAN_POINT ( 'NONE',  ( -10.81189881249999729, 1.324075727343319199E-15, -150.7812500020483810 ) ) ;
#40394=CARTESIAN_POINT ( 'NONE',  ( -10.81189881249999729, 6.242252689847871849, -138.7187500020483810 ) ) ;
#40395=CARTESIAN_POINT ( 'NONE',  ( -10.00000000000102496, 5.773502691895664007, -3.250000004096733619 ) ) ;
#40396=VERTEX_POINT ( 'NONE', #34872 ) ;
#40399=ORIENTED_EDGE ( 'NONE', *, *, #27555, .T. ) ;
#40401=EDGE_CURVE ( 'NONE', #18552, #40567, #33337, .T. ) ;
#40402=CARTESIAN_POINT ( 'NONE',  ( 5.405949406249999534, 9.363379034771803333, -109.0937500020483810 ) ) ;
#40403=VERTEX_POINT ( 'NONE', #1640 ) ;
#40404=ADVANCED_FACE ( 'NONE', ( #14557 ), #41315, .T. ) ;
#40405=EDGE_CURVE ( 'NONE', #4880, #10744, #9629, .T. ) ;
#40407=CARTESIAN_POINT ( 'NONE',  ( 10.81189881249999907, 6.242252689847868297, -193.2187500020484094 ) ) ;
#40408=CARTESIAN_POINT ( 'NONE',  ( 5.405949406249999534, 9.363379034771803333, -35.59375000204836681 ) ) ;
#40409=CARTESIAN_POINT ( 'NONE',  ( -2.129899540880850761, -10.13128953862508652, 1.243155832063081174E-14 ) ) ;
#40411=CARTESIAN_POINT ( 'NONE',  ( -5.405949406249996869, 9.363379034771805109, -170.3437500020484094 ) ) ;
#40412=CARTESIAN_POINT ( 'NONE',  ( 10.81189881249999907, 6.242252689847868297, -158.7187500020483810 ) ) ;
#40414=CARTESIAN_POINT ( 'NONE',  ( -2.121150477449813534E-15, -11.54700538379251284, -122.7500000040967905 ) ) ;
#40417=CARTESIAN_POINT ( 'NONE',  ( 9.999999999999998224, 0.000000000000000000, -155.0000000000000000 ) ) ;
#40418=CARTESIAN_POINT ( 'NONE',  ( 9.999999999999998224, 0.000000000000000000, -66.87500000409676204 ) ) ;
#40420=CARTESIAN_POINT ( 'NONE',  ( 5.405949406249999534, 9.363379034771803333, -88.09375000204836681 ) ) ;
#40421=FACE_OUTER_BOUND ( 'NONE', #37031, .T. ) ;
#40422=CARTESIAN_POINT ( 'NONE',  ( -10.81189881249999729, 1.324075727343319199E-15, -63.78125000204837391 ) ) ;
#40423=DIRECTION ( 'NONE',  ( 1.000000000000000000, 0.000000000000000000, 0.000000000000000000 ) ) ;
#40425=EDGE_CURVE ( 'NONE', #14436, #31963, #24142, .T. ) ;
#40426=CARTESIAN_POINT ( 'NONE',  ( -10.81189881249999729, 6.242252689847871849, -120.9062500020483952 ) ) ;
#40427=CARTESIAN_POINT ( 'NONE',  ( 10.81189881249999729, 0.000000000000000000, -154.5312500020484094 ) ) ;
#40429=CARTESIAN_POINT ( 'NONE',  ( -2.121150477449813534E-15, -11.54700538379251284, -130.2500000040967905 ) ) ;
#40431=ORIENTED_EDGE ( 'NONE', *, *, #40356, .T. ) ;
#40435=ADVANCED_FACE ( 'NONE', ( #5085 ), #37455, .T. ) ;
#40436=CARTESIAN_POINT ( 'NONE',  ( -10.81189881249999729, 6.242252689847871849, -186.9062500020484094 ) ) ;
#40437=ORIENTED_EDGE ( 'NONE', *, *, #1114, .T. ) ;
#40438=CARTESIAN_POINT ( 'NONE',  ( 10.00000000000000000, 5.773502691896255534, -46.87499999999996447 ) ) ;
#40440=CARTESIAN_POINT ( 'NONE',  ( -5.000000000000003553, -8.660254037844383745, -55.37500000409675494 ) ) ;
#40441=EDGE_CURVE ( 'NONE', #22759, #35200, #11108, .T. ) ;
#40445=CARTESIAN_POINT ( 'NONE',  ( -10.81189881249999729, 6.242252689847871849, -60.90625000204837391 ) ) ;
#40449=CARTESIAN_POINT ( 'NONE',  ( 10.81189881249999729, 0.000000000000000000, -178.5312500020483810 ) ) ;
#40451=CARTESIAN_POINT ( 'NONE',  ( -9.999999999999998224, 1.224646799147353059E-15, -88.24999999999998579 ) ) ;
#40454=CARTESIAN_POINT ( 'NONE',  ( 9.999999999999998224, 0.000000000000000000, -177.5000000000000000 ) ) ;
#40456=CARTESIAN_POINT ( 'NONE',  ( -2.293366432827344421E-15, -12.48450537969573659, -84.40625000204838102 ) ) ;
#40457=VERTEX_POINT ( 'NONE', #4868 ) ;
#40458=CARTESIAN_POINT ( 'NONE',  ( 9.999999999999998224, 0.000000000000000000, -92.37500000409677625 ) ) ;
#40461=CARTESIAN_POINT ( 'NONE',  ( 10.81189881249999729, 6.242252689847867408, -34.21875000204835260 ) ) ;
#40462=CARTESIAN_POINT ( 'NONE',  ( -5.405949406249996869, 9.363379034771805109, -26.34375000204835970 ) ) ;
#40463=CARTESIAN_POINT ( 'NONE',  ( -5.405949406249996869, 9.363379034771805109, -10.03125000204835260 ) ) ;
#40464=CARTESIAN_POINT ( 'NONE',  ( 10.81189881249999551, -6.242252689847874514, -65.96875000204836681 ) ) ;
#40465=DIRECTION ( 'NONE',  ( -0.000000000000000000, -0.000000000000000000, 1.000000000000000000 ) ) ;
#40467=CARTESIAN_POINT ( 'NONE',  ( -10.81189881249999729, 6.242252689847871849, -185.2187500020483810 ) ) ;
#40469=CARTESIAN_POINT ( 'NONE',  ( 10.81189881249999551, -6.242252689847874514, -2.968750002048361925 ) ) ;
#40470=CARTESIAN_POINT ( 'NONE',  ( -2.121150477449813534E-15, -11.54700538379251284, -192.8750000000000284 ) ) ;
#40471=CARTESIAN_POINT ( 'NONE',  ( -10.00000000000051337, 5.773502691895962435, -70.75000000409677625 ) ) ;
#40473=FACE_OUTER_BOUND ( 'NONE', #13112, .T. ) ;
#40474=CARTESIAN_POINT ( 'NONE',  ( 10.81189881249999907, 6.242252689847868297, -116.7187500020483810 ) ) ;
#40475=CARTESIAN_POINT ( 'NONE',  ( 5.000000000000000000, 8.660254037844385522, -15.24999999999995737 ) ) ;
#40476=CARTESIAN_POINT ( 'NONE',  ( 10.81189881249999729, 0.000000000000000000, -93.03125000204838102 ) ) ;
#40477=CARTESIAN_POINT ( 'NONE',  ( 5.405949406249992428, -9.363379034771808662, -99.09375000204838102 ) ) ;
#40478=VECTOR ( 'NONE', #35469, 1000.000000000000000 ) ;
#40481=CARTESIAN_POINT ( 'NONE',  ( -4.999999999999996447, 8.660254037844387298, -150.3750000040967905 ) ) ;
#40483=( BOUNDED_CURVE ( )  B_SPLINE_CURVE ( 2, ( #41375, #34073, #18078, #24800, #11592, #37294, #17426 ),
 .UNSPECIFIED., .F., .F. ) 
 B_SPLINE_CURVE_WITH_KNOTS ( ( 3, 2, 2, 3 ),
 ( 0.02238805970149256030, 0.02363184079601992477, 0.02487562189054729270, 0.02611940298507465369 ),
 .UNSPECIFIED. ) 
 CURVE ( )  GEOMETRIC_REPRESENTATION_ITEM ( )  RATIONAL_B_SPLINE_CURVE ( ( 0.9999999999999973355, 0.8660254037844413721, 1.000000000000000000, 0.8660254037844387076, 1.000000000000000000, 0.8660254037844357100, 1.000000000000003109 ) ) 
 REPRESENTATION_ITEM ( '' )  );
#40487=CARTESIAN_POINT ( 'NONE',  ( 9.999999999999998224, 0.000000000000000000, -101.3750000040967905 ) ) ;
#40489=CARTESIAN_POINT ( 'NONE',  ( 7.070501591499376803E-16, 11.54700538379251284, -10.62499999999995381 ) ) ;
#40490=CARTESIAN_POINT ( 'NONE',  ( 4.999999999999992006, -8.660254037844389075, -75.74999999999998579 ) ) ;
#40492=CARTESIAN_POINT ( 'NONE',  ( -5.000000000000003553, -8.660254037844383745, -91.37500000409677625 ) ) ;
#40493=CARTESIAN_POINT ( 'NONE',  ( 9.999999999999872102, 5.773502691896329253, -168.7500000040967905 ) ) ;
#40495=CARTESIAN_POINT ( 'NONE',  ( 5.405949406249992428, -9.363379034771808662, -85.78125000204838102 ) ) ;
#40496=( BOUNDED_CURVE ( )  B_SPLINE_CURVE ( 2, ( #32294, #18902, #29466, #32502, #25808, #32083, #19310 ),
 .UNSPECIFIED., .F., .F. ) 
 B_SPLINE_CURVE_WITH_KNOTS ( ( 3, 2, 2, 3 ),
 ( 0.01492537313432837180, 0.01616915422885573453, 0.01741293532338310246, 0.01865671641791046345 ),
 .UNSPECIFIED. ) 
 CURVE ( )  GEOMETRIC_REPRESENTATION_ITEM ( )  RATIONAL_B_SPLINE_CURVE ( ( 0.9999999999999984457, 0.8660254037844402619, 1.000000000000000000, 0.8660254037844387076, 1.000000000000000000, 0.8660254037844368202, 1.000000000000001776 ) ) 
 REPRESENTATION_ITEM ( '' )  );
#40498=CARTESIAN_POINT ( 'NONE',  ( 9.999999999999998224, 0.000000000000000000, -19.99999999999996092 ) ) ;
#40500=ORIENTED_EDGE ( 'NONE', *, *, #6966, .F. ) ;
#40501=CARTESIAN_POINT ( 'NONE',  ( 9.999999999999996447, -5.773502691896262640, -2.124999999999945821 ) ) ;
#40503=CARTESIAN_POINT ( 'NONE',  ( -10.81189881249999729, 1.324075727343319199E-15, -17.09375000204835260 ) ) ;
#40506=CARTESIAN_POINT ( 'NONE',  ( -10.81189881249999729, 6.242252689847871849, -132.9062500020483810 ) ) ;
#40507=( BOUNDED_CURVE ( )  B_SPLINE_CURVE ( 2, ( #23265, #13098, #13524, #16550, #26710, #29748, #2995 ),
 .UNSPECIFIED., .F., .F. ) 
 B_SPLINE_CURVE_WITH_KNOTS ( ( 3, 2, 2, 3 ),
 ( 0.04850746268656720706, 0.04975124378109457846, 0.05099502487562193598, 0.05223880597014930738 ),
 .UNSPECIFIED. ) 
 CURVE ( )  GEOMETRIC_REPRESENTATION_ITEM ( )  RATIONAL_B_SPLINE_CURVE ( ( 0.9999999999999955591, 0.8660254037844431485, 1.000000000000000000, 0.8660254037844387076, 1.000000000000000000, 0.8660254037844327124, 1.000000000000005995 ) ) 
 REPRESENTATION_ITEM ( '' )  );
#40508=CARTESIAN_POINT ( 'NONE',  ( -9.999999999999998224, 1.224646799147353059E-15, -185.7500000000000000 ) ) ;
#40509=DIRECTION ( 'NONE',  ( -0.000000000000000000, -0.000000000000000000, 1.000000000000000000 ) ) ;
#40510=CARTESIAN_POINT ( 'NONE',  ( 10.81189881249999551, -6.242252689847874514, -112.6562500020483810 ) ) ;
#40512=VECTOR ( 'NONE', #14788, 1000.000000000000000 ) ;
#40513=DIRECTION ( 'NONE',  ( -0.000000000000000000, -0.000000000000000000, 1.000000000000000000 ) ) ;
#40515=ORIENTED_EDGE ( 'NONE', *, *, #3288, .F. ) ;
#40516=CARTESIAN_POINT ( 'NONE',  ( 7.644554776091147741E-16, 12.48450537969573659, -34.15625000204836681 ) ) ;
#40518=CARTESIAN_POINT ( 'NONE',  ( -10.81189881249999907, -6.242252689847864744, -97.96875000204838102 ) ) ;
#40519=DIRECTION ( 'NONE',  ( -0.000000000000000000, -0.000000000000000000, 1.000000000000000000 ) ) ;
#40520=CARTESIAN_POINT ( 'NONE',  ( 9.999999999999998224, 0.000000000000000000, -147.8750000040967905 ) ) ;
#40521=CARTESIAN_POINT ( 'NONE',  ( 7.644554776091147741E-16, 12.48450537969573659, -197.4687500020484094 ) ) ;
#40523=CARTESIAN_POINT ( 'NONE',  ( 9.999999999999998224, 0.000000000000000000, -138.5000000000000000 ) ) ;
#40524=ADVANCED_FACE ( 'NONE', ( #31214 ), #28182, .T. ) ;
#40525=CARTESIAN_POINT ( 'NONE',  ( 10.81189881249999729, 0.000000000000000000, -122.8437500020483952 ) ) ;
#40527=CARTESIAN_POINT ( 'NONE',  ( -5.405949406250003975, -9.363379034771801557, -5.031250002048376579 ) ) ;
#40530=CARTESIAN_POINT ( 'NONE',  ( 10.00000000000000000, 5.773502691896255534, -179.2500000040967905 ) ) ;
#40532=CARTESIAN_POINT ( 'NONE',  ( -5.405949406250003975, -9.363379034771801557, -180.5312500020483810 ) ) ;
#40533=CARTESIAN_POINT ( 'NONE',  ( 9.999999999999998224, 0.000000000000000000, -106.9999999999999858 ) ) ;
#40534=CARTESIAN_POINT ( 'NONE',  ( -9.999999999999998224, 1.224646799147353059E-15, -86.74999999999998579 ) ) ;
#40536=CARTESIAN_POINT ( 'NONE',  ( -10.81189881249999729, -6.242252689847864744, -52.96875000204837391 ) ) ;
#40537=CARTESIAN_POINT ( 'NONE',  ( -10.81189881249999907, -6.242252689847864744, -42.46875000204835260 ) ) ;
#40539=CARTESIAN_POINT ( 'NONE',  ( 7.644554776091147741E-16, 12.48450537969573659, -7.156250002048365921 ) ) ;
#40541=CARTESIAN_POINT ( 'NONE',  ( -9.999999999999998224, 1.224646799147353059E-15, -93.12500000409677625 ) ) ;
#40543=CARTESIAN_POINT ( 'NONE',  ( 10.00000000000000000, 5.773502691896255534, -97.87499999999998579 ) ) ;
#40545=CARTESIAN_POINT ( 'NONE',  ( -9.999999999999998224, 1.224646799147353059E-15, -112.6250000040967763 ) ) ;
#40546=CARTESIAN_POINT ( 'NONE',  ( 4.999999999999992006, -8.660254037844389075, -26.62500000409676204 ) ) ;
#40549=CARTESIAN_POINT ( 'NONE',  ( -5.405949406250003975, -9.363379034771801557, -104.0312500020483810 ) ) ;
#40550=EDGE_CURVE ( 'NONE', #35982, #26720, #12636, .T. ) ;
#40551=ORIENTED_EDGE ( 'NONE', *, *, #36754, .T. ) ;
#40554=CARTESIAN_POINT ( 'NONE',  ( -10.00000000000051337, 5.773502691895962435, -141.2500000040967905 ) ) ;
#40555=CARTESIAN_POINT ( 'NONE',  ( 10.81189881249999551, -6.242252689847874514, -165.1562500020483526 ) ) ;
#40557=ORIENTED_EDGE ( 'NONE', *, *, #33639, .T. ) ;
#40558=CARTESIAN_POINT ( 'NONE',  ( 5.000000000000000000, 8.660254037844385522, -25.74999999999996803 ) ) ;
#40559=CARTESIAN_POINT ( 'NONE',  ( 5.405949406249992428, -9.363379034771808662, -34.78125000204837391 ) ) ;
#40560=CARTESIAN_POINT ( 'NONE',  ( -9.999999999999998224, 1.224646799147353059E-15, -164.7500000000000000 ) ) ;
#40563=CARTESIAN_POINT ( 'NONE',  ( -2.293366432827344421E-15, -12.48450537969573659, -135.4062500020483810 ) ) ;
#40564=CARTESIAN_POINT ( 'NONE',  ( 8.421130500909246308, 6.441071276087089181, -7.741086494507740905E-15 ) ) ;
#40565=CYLINDRICAL_SURFACE ( 'NONE', #3849, 9.999999999999998224 ) ;
#40567=VERTEX_POINT ( 'NONE', #32060 ) ;
#40568=ORIENTED_EDGE ( 'NONE', *, *, #42224, .F. ) ;
#40570=( BOUNDED_CURVE ( )  B_SPLINE_CURVE ( 2, ( #9396, #2091, #31876, #12612, #25805, #25386, #15221 ),
 .UNSPECIFIED., .F., .F. ) 
 B_SPLINE_CURVE_WITH_KNOTS ( ( 3, 2, 2, 3 ),
 ( 0.8694029850746272103, 0.8706467661691545956, 0.8718905472636818699, 0.8731343283582092551 ),
 .UNSPECIFIED. ) 
 CURVE ( )  GEOMETRIC_REPRESENTATION_ITEM ( )  RATIONAL_B_SPLINE_CURVE ( ( 0.9999999999999641398, 0.8660254037844745678, 1.000000000000000000, 0.8660254037844387076, 1.000000000000000000, 0.8660254037844028474, 1.000000000000035971 ) ) 
 REPRESENTATION_ITEM ( '' )  );
#40572=CARTESIAN_POINT ( 'NONE',  ( -9.999999999999227285, -5.773502691896698735, -134.6249999999999716 ) ) ;
#40573=CARTESIAN_POINT ( 'NONE',  ( 5.405949406249999534, 9.363379034771803333, -167.5937500020484094 ) ) ;
#40576=CARTESIAN_POINT ( 'NONE',  ( -10.81189881249999729, 1.324075727343319199E-15, -18.59375000204835260 ) ) ;
#40577=AXIS2_PLACEMENT_3D ( 'NONE', #39652, #11568, #11786 ) ;
#40578=FACE_OUTER_BOUND ( 'NONE', #31642, .T. ) ;
#40579=CARTESIAN_POINT ( 'NONE',  ( 10.81189881249999551, -6.242252689847874514, -146.9687500020484094 ) ) ;
#40580=CARTESIAN_POINT ( 'NONE',  ( -10.81189881249999729, 1.324075727343319199E-15, -137.0937500020483810 ) ) ;
#40581=CARTESIAN_POINT ( 'NONE',  ( 5.405949406249992428, -9.363379034771808662, -105.2812500020483810 ) ) ;
#40585=CARTESIAN_POINT ( 'NONE',  ( 10.81189881249999551, -6.242252689847874514, -11.96875000204837214 ) ) ;
#40588=CARTESIAN_POINT ( 'NONE',  ( -10.00000000000019362, -5.773502691896140959, -178.5000000040968189 ) ) ;
#40591=CARTESIAN_POINT ( 'NONE',  ( 10.81189881249999729, 0.000000000000000000, -77.84375000204838102 ) ) ;
#40592=CARTESIAN_POINT ( 'NONE',  ( 10.81189881249999729, 0.000000000000000000, -61.34375000204836681 ) ) ;
#40593=CARTESIAN_POINT ( 'NONE',  ( 9.999999999999998224, 0.000000000000000000, -200.0000000000000000 ) ) ;
#40594=CARTESIAN_POINT ( 'NONE',  ( -2.293366432827344421E-15, -12.48450537969573659, -33.40625000204835970 ) ) ;
#40597=CARTESIAN_POINT ( 'NONE',  ( 9.999999999999996447, -5.773502691896262640, -120.6250000000000000 ) ) ;
#40598=CARTESIAN_POINT ( 'NONE',  ( 5.405949406249992428, -9.363379034771808662, -129.2812500020483810 ) ) ;
#40599=CARTESIAN_POINT ( 'NONE',  ( -5.000000000000003553, -8.660254037844383745, -187.3750000040967905 ) ) ;
#40601=CARTESIAN_POINT ( 'NONE',  ( -10.81189881249999729, 6.242252689847871849, -15.90625000204837391 ) ) ;
#40602=ORIENTED_EDGE ( 'NONE', *, *, #15445, .F. ) ;
#40605=CARTESIAN_POINT ( 'NONE',  ( -9.999999999999998224, 1.224646799147353059E-15, -37.62500000409676915 ) ) ;
#40606=ADVANCED_FACE ( 'NONE', ( #38515 ), #35510, .T. ) ;
#40607=CARTESIAN_POINT ( 'NONE',  ( -2.121150477449813534E-15, -11.54700538379251284, -2.750000004096757156 ) ) ;
#40609=CARTESIAN_POINT ( 'NONE',  ( -5.405949406249996869, 9.363379034771805109, -152.5312500020484094 ) ) ;
#40610=AXIS2_PLACEMENT_3D ( 'NONE', #17209, #36866, #10954 ) ;
#40611=CARTESIAN_POINT ( 'NONE',  ( -2.293366432827344421E-15, -12.48450537969573659, -126.2187500020483952 ) ) ;
#40613=ORIENTED_EDGE ( 'NONE', *, *, #11920, .T. ) ;
#40614=CARTESIAN_POINT ( 'NONE',  ( 9.999999999998456346, 5.773502691897149042, -22.87499999999994316 ) ) ;
#40616=( BOUNDED_CURVE ( )  B_SPLINE_CURVE ( 2, ( #33548, #747, #17113, #33760, #27489, #27065, #4181 ),
 .UNSPECIFIED., .F., .F. ) 
 B_SPLINE_CURVE_WITH_KNOTS ( ( 3, 2, 2, 3 ),
 ( 0.6791044776119405935, 0.6803482587064679787, 0.6815920398009952530, 0.6828358208955226383 ),
 .UNSPECIFIED. ) 
 CURVE ( )  GEOMETRIC_REPRESENTATION_ITEM ( )  RATIONAL_B_SPLINE_CURVE ( ( 0.9999999999999641398, 0.8660254037844745678, 1.000000000000000000, 0.8660254037844387076, 1.000000000000000000, 0.8660254037844148378, 1.000000000000023981 ) ) 
 REPRESENTATION_ITEM ( '' )  );
#40618=ORIENTED_EDGE ( 'NONE', *, *, #1972, .F. ) ;
#40619=CARTESIAN_POINT ( 'NONE',  ( -5.405949406249996869, 9.363379034771805109, -108.8437500020483810 ) ) ;
#40620=ORIENTED_EDGE ( 'NONE', *, *, #5677, .T. ) ;
#40621=CARTESIAN_POINT ( 'NONE',  ( -9.999999999999998224, 1.224646799147353059E-15, -188.7500000000000000 ) ) ;
#40622=CARTESIAN_POINT ( 'NONE',  ( -10.81189881249999907, -6.242252689847864744, -186.4687500020484094 ) ) ;
#40623=CARTESIAN_POINT ( 'NONE',  ( 10.81189881249999729, 0.000000000000000000, -41.84375000204837391 ) ) ;
#40624=CARTESIAN_POINT ( 'NONE',  ( -5.000000000000003553, -8.660254037844383745, -155.8750000040967905 ) ) ;
#40625=CARTESIAN_POINT ( 'NONE',  ( -5.405949406250003975, -9.363379034771801557, -169.8437500020484094 ) ) ;
#40626=CARTESIAN_POINT ( 'NONE',  ( 10.81189881249999551, -6.242252689847874514, -163.4687500020483810 ) ) ;
#40627=DIRECTION ( 'NONE',  ( -0.000000000000000000, -0.000000000000000000, 1.000000000000000000 ) ) ;
#40630=CARTESIAN_POINT ( 'NONE',  ( -9.999999999999479527, -5.773502691896549521, -94.12499999999997158 ) ) ;
#40633=AXIS2_PLACEMENT_3D ( 'NONE', #22180, #35565, #9012 ) ;
#40634=CARTESIAN_POINT ( 'NONE',  ( -10.81189881249999907, -6.242252689847864744, -90.46875000204836681 ) ) ;
#40636=CARTESIAN_POINT ( 'NONE',  ( 5.405949406249992428, -9.363379034771808662, -58.78125000204836681 ) ) ;
#40637=CARTESIAN_POINT ( 'NONE',  ( 7.070501591499376803E-16, 11.54700538379251284, -146.0000000040967905 ) ) ;
#40639=CARTESIAN_POINT ( 'NONE',  ( -5.405949406250003975, -9.363379034771801557, -111.5312500020483810 ) ) ;
#40640=CARTESIAN_POINT ( 'NONE',  ( -10.81189881249999729, -6.242252689847864744, -150.6562500020484094 ) ) ;
#40643=CARTESIAN_POINT ( 'NONE',  ( -9.999999999999998224, 1.224646799147353059E-15, -129.1250000040967620 ) ) ;
#40645=EDGE_LOOP ( 'NONE', ( #4531, #34908, #26004, #18885 ) ) ;
#40648=CARTESIAN_POINT ( 'NONE',  ( -10.81189881249999907, -6.242252689847864744, -186.6562500020484094 ) ) ;
#40649=EDGE_LOOP ( 'NONE', ( #7399, #27483, #39567, #34394 ) ) ;
#40650=CARTESIAN_POINT ( 'NONE',  ( 9.999999999999996447, -5.773502691896262640, -45.62499999999995737 ) ) ;
#40652=CARTESIAN_POINT ( 'NONE',  ( 5.000000000000000000, 8.660254037844385522, -59.12500000409676204 ) ) ;
#40653=EDGE_CURVE ( 'NONE', #311, #16498, #37736, .T. ) ;
#40654=CARTESIAN_POINT ( 'NONE',  ( 4.999999999999992006, -8.660254037844389075, -18.74999999999996092 ) ) ;
#40655=DIRECTION ( 'NONE',  ( -1.000000000000000000, -4.506943796211477094E-16, -0.000000000000000000 ) ) ;
#40658=CARTESIAN_POINT ( 'NONE',  ( 10.81189881249999551, -6.242252689847874514, -48.15625000204836681 ) ) ;
#40662=CARTESIAN_POINT ( 'NONE',  ( 5.405949406249999534, 9.363379034771803333, -176.7812500020484094 ) ) ;
#40664=LINE ( 'NONE', #4435, #15943 ) ;
#40666=CARTESIAN_POINT ( 'NONE',  ( 5.000000000000000000, 8.660254037844385522, -117.2500000000000000 ) ) ;
#40667=LINE ( 'NONE', #40248, #26597 ) ;
#40668=CARTESIAN_POINT ( 'NONE',  ( 9.999999999999998224, 0.000000000000000000, -19.99999999999996092 ) ) ;
#40670=CARTESIAN_POINT ( 'NONE',  ( 10.81189881249999551, -6.242252689847874514, -85.65625000204838102 ) ) ;
#40671=ORIENTED_EDGE ( 'NONE', *, *, #41532, .F. ) ;
#40673=EDGE_CURVE ( 'NONE', #29666, #27948, #12384, .T. ) ;
#40674=DIRECTION ( 'NONE',  ( -0.000000000000000000, -0.000000000000000000, -1.000000000000000000 ) ) ;
#40677=CARTESIAN_POINT ( 'NONE',  ( 5.405949406249992428, -9.363379034771808662, -39.09375000204837391 ) ) ;
#40678=CARTESIAN_POINT ( 'NONE',  ( 5.405949406249992428, -9.363379034771808662, -24.09375000204835970 ) ) ;
#40679=CARTESIAN_POINT ( 'NONE',  ( -2.293366432827344421E-15, -12.48450537969573659, -13.90625000204836503 ) ) ;
#40680=CARTESIAN_POINT ( 'NONE',  ( 7.644554776091147741E-16, 12.48450537969573659, -60.96875000204838102 ) ) ;
#40683=EDGE_CURVE ( 'NONE', #34991, #19338, #9876, .T. ) ;
#40684=CARTESIAN_POINT ( 'NONE',  ( 10.81189881249999729, 0.000000000000000000, -181.3437500020483810 ) ) ;
#40687=CARTESIAN_POINT ( 'NONE',  ( 10.00000000000000000, 5.773502691896255534, -132.3750000000000000 ) ) ;
#40690=LINE ( 'NONE', #13931, #8135 ) ;
#40691=CARTESIAN_POINT ( 'NONE',  ( 10.81189881249999907, 6.242252689847868297, -109.2187500020483810 ) ) ;
#40692=CARTESIAN_POINT ( 'NONE',  ( 5.321294541346989426, 0.000000000000000000, -220.0000000000000000 ) ) ;
#40693=CARTESIAN_POINT ( 'NONE',  ( -10.81189881249999729, 1.324075727343319199E-15, -78.78125000204838102 ) ) ;
#40694=CARTESIAN_POINT ( 'NONE',  ( -10.81189881249999729, 1.324075727343319199E-15, -99.59375000204838102 ) ) ;
#40697=CARTESIAN_POINT ( 'NONE',  ( 4.999999999999992006, -8.660254037844389075, -157.1250000040967905 ) ) ;
#40702=FACE_BOUND ( 'NONE', #14866, .T. ) ;
#40703=CARTESIAN_POINT ( 'NONE',  ( -5.000000000000003553, -8.660254037844383745, -197.5000000000000000 ) ) ;
#40706=CARTESIAN_POINT ( 'NONE',  ( 5.000000000000000000, 8.660254037844385522, -72.24999999999998579 ) ) ;
#40708=CARTESIAN_POINT ( 'NONE',  ( -2.121150477449813534E-15, -11.54700538379251284, -85.25000000409676204 ) ) ;
#40710=CARTESIAN_POINT ( 'NONE',  ( 9.999999999999479527, 5.773502691896553074, -115.8749999999999858 ) ) ;
#40712=CARTESIAN_POINT ( 'NONE',  ( -5.405949406249996869, 9.363379034771805109, -74.53125000204838102 ) ) ;
#40718=CARTESIAN_POINT ( 'NONE',  ( -5.405949406249996869, 9.363379034771805109, -199.0312500020484094 ) ) ;
#40719=ADVANCED_FACE ( 'NONE', ( #7516 ), #33642, .T. ) ;
#40721=CARTESIAN_POINT ( 'NONE',  ( -10.81189881249999729, 1.324075727343319199E-15, -15.59375000204835082 ) ) ;
#40725=CARTESIAN_POINT ( 'NONE',  ( 10.81189881249999551, -6.242252689847874514, -129.1562500020483810 ) ) ;
#40726=CARTESIAN_POINT ( 'NONE',  ( -5.000000000000003553, -8.660254037844383745, -182.5000000000000000 ) ) ;
#40727=CARTESIAN_POINT ( 'NONE',  ( -10.81189881249999729, 1.324075727343319199E-15, -111.7812500020483810 ) ) ;
#40728=ORIENTED_EDGE ( 'NONE', *, *, #18568, .T. ) ;
#40729=CARTESIAN_POINT ( 'NONE',  ( -2.121150477449813534E-15, -11.54700538379251284, -154.2500000040968189 ) ) ;
#40731=EDGE_LOOP ( 'NONE', ( #4813, #22652, #27379, #39207 ) ) ;
#40732=EDGE_CURVE ( 'NONE', #39394, #12699, #16779, .T. ) ;
#40733=AXIS2_PLACEMENT_3D ( 'NONE', #21588, #24199, #14665 ) ;
#40734=CARTESIAN_POINT ( 'NONE',  ( 10.81189881249999907, 6.242252689847868297, -38.90625000204835970 ) ) ;
#40737=CARTESIAN_POINT ( 'NONE',  ( 7.644554776091147741E-16, 12.48450537969573659, -89.46875000204838102 ) ) ;
#40739=CARTESIAN_POINT ( 'NONE',  ( 7.070501591499376803E-16, 11.54700538379251284, -174.1250000000000000 ) ) ;
#40740=( BOUNDED_CURVE ( )  B_SPLINE_CURVE ( 2, ( #28663, #9212, #12434, #25630, #8005, #40992, #18348 ),
 .UNSPECIFIED., .F., .F. ) 
 B_SPLINE_CURVE_WITH_KNOTS ( ( 3, 2, 2, 3 ),
 ( 0.2910447761194031036, 0.2922885572139304333, 0.2935323383084578186, 0.2947761194029852039 ),
 .UNSPECIFIED. ) 
 CURVE ( )  GEOMETRIC_REPRESENTATION_ITEM ( )  RATIONAL_B_SPLINE_CURVE ( ( 0.9999999999999880096, 0.8660254037844506980, 1.000000000000000000, 0.8660254037844387076, 1.000000000000000000, 0.8660254037844267172, 1.000000000000011990 ) ) 
 REPRESENTATION_ITEM ( '' )  );
#40741=FACE_OUTER_BOUND ( 'NONE', #20026, .T. ) ;
#40744=CARTESIAN_POINT ( 'NONE',  ( -10.81189881249999729, 1.324075727343319199E-15, -125.0937500020483668 ) ) ;
#40746=CARTESIAN_POINT ( 'NONE',  ( 0.000000000000000000, 0.000000000000000000, -200.0000000000000000 ) ) ;
#40749=CARTESIAN_POINT ( 'NONE',  ( 9.999999999999996447, -5.773502691896262640, -175.0000000040968189 ) ) ;
#40751=CARTESIAN_POINT ( 'NONE',  ( 5.405949406249999534, 9.363379034771803333, -175.2812500020484094 ) ) ;
#40752=LINE ( 'NONE', #661, #10281 ) ;
#40755=CARTESIAN_POINT ( 'NONE',  ( 10.81189881249999551, -6.242252689847874514, -50.96875000204836681 ) ) ;
#40757=CARTESIAN_POINT ( 'NONE',  ( 5.405949406249992428, -9.363379034771808662, -7.781250002048350822 ) ) ;
#40759=CARTESIAN_POINT ( 'NONE',  ( -9.999999999999872102, -5.773502691896326589, -193.5000000040967620 ) ) ;
#40761=CARTESIAN_POINT ( 'NONE',  ( 4.999999999999992006, -8.660254037844389075, -98.24999999999998579 ) ) ;
#40763=CARTESIAN_POINT ( 'NONE',  ( -2.121150477449813534E-15, -11.54700538379251284, -107.7500000040967763 ) ) ;
#40767=CARTESIAN_POINT ( 'NONE',  ( -10.81189881249999729, -6.242252689847864744, -105.6562500020483952 ) ) ;
#40768=ORIENTED_EDGE ( 'NONE', *, *, #28566, .T. ) ;
#40771=CARTESIAN_POINT ( 'NONE',  ( 10.81189881249999729, 0.000000000000000000, -162.0312500020484094 ) ) ;
#40773=VERTEX_POINT ( 'NONE', #40094 ) ;
#40774=CARTESIAN_POINT ( 'NONE',  ( -4.999999999999996447, 8.660254037844387298, -25.49999999999996803 ) ) ;
#40776=CARTESIAN_POINT ( 'NONE',  ( -10.81189881249999729, 6.242252689847871849, -33.90625000204836681 ) ) ;
#40777=CARTESIAN_POINT ( 'NONE',  ( 5.000000000000000000, 8.660254037844385522, -159.2500000000000000 ) ) ;
#40782=CARTESIAN_POINT ( 'NONE',  ( 5.405949406249992428, -9.363379034771808662, -130.7812500020483810 ) ) ;
#40783=CARTESIAN_POINT ( 'NONE',  ( -4.638487482233418113, 8.887449022414848798, 2.775557561562891982E-14 ) ) ;
#40785=EDGE_LOOP ( 'NONE', ( #23184, #17006, #9682, #19087 ) ) ;
#40788=VECTOR ( 'NONE', #8251, 1000.000000000000000 ) ;
#40789=CARTESIAN_POINT ( 'NONE',  ( 9.999999999999994671, -5.773502691896262640, -134.1250000000000000 ) ) ;
#40790=CARTESIAN_POINT ( 'NONE',  ( 10.81189881249999551, -6.242252689847874514, -166.4687500020484094 ) ) ;
#40792=CARTESIAN_POINT ( 'NONE',  ( -10.81189881249999729, 1.324075727343319199E-15, -12.59375000204834905 ) ) ;
#40793=CARTESIAN_POINT ( 'NONE',  ( 9.999999999999998224, 0.000000000000000000, -22.99999999999996447 ) ) ;
#40794=CARTESIAN_POINT ( 'NONE',  ( -10.81189881249999729, 6.242252689847871849, -149.2187500020484379 ) ) ;
#40795=CARTESIAN_POINT ( 'NONE',  ( -5.405949406249996869, 9.363379034771805109, -137.3437500020484094 ) ) ;
#40796=CARTESIAN_POINT ( 'NONE',  ( -2.293366432827344421E-15, -12.48450537969573659, -109.9062500020483952 ) ) ;
#40800=CARTESIAN_POINT ( 'NONE',  ( -10.81189881249999729, 1.324075727343319199E-15, -5.093750002048369474 ) ) ;
#40802=CARTESIAN_POINT ( 'NONE',  ( 9.999999999999998224, 0.000000000000000000, -81.87500000409676204 ) ) ;
#40806=VECTOR ( 'NONE', #7402, 1000.000000000000000 ) ;
#40807=CARTESIAN_POINT ( 'NONE',  ( -10.81189881249999729, -6.242252689847864744, -75.46875000204836681 ) ) ;
#40808=CARTESIAN_POINT ( 'NONE',  ( 10.81189881249999551, -6.242252689847874514, -67.46875000204838102 ) ) ;
#40810=CARTESIAN_POINT ( 'NONE',  ( 10.81189881249999551, -6.242252689847874514, -36.15625000204835970 ) ) ;
#40814=CARTESIAN_POINT ( 'NONE',  ( -5.000000000000003553, -8.660254037844383745, -118.0000000000000000 ) ) ;
#40815=CARTESIAN_POINT ( 'NONE',  ( 5.405949406249999534, 9.363379034771803333, -128.7812500020483810 ) ) ;
#40816=CARTESIAN_POINT ( 'NONE',  ( -9.999999999999998224, 1.224646799147353059E-15, -67.62500000409676204 ) ) ;
#40818=CARTESIAN_POINT ( 'NONE',  ( -5.405949406250003975, -9.363379034771801557, -21.53125000204836326 ) ) ;
#40822=CARTESIAN_POINT ( 'NONE',  ( -9.999999999999998224, 1.224646799147353059E-15, -57.12500000409676204 ) ) ;
#40823=CARTESIAN_POINT ( 'NONE',  ( -10.00000000000000000, -5.773502691896251982, -37.50000000409676204 ) ) ;
#40825=CARTESIAN_POINT ( 'NONE',  ( 9.999999999999479527, 5.773502691896553074, -147.3750000000000000 ) ) ;
#40826=CARTESIAN_POINT ( 'NONE',  ( 10.81189881249999907, 6.242252689847868297, -155.9062500020484094 ) ) ;
#40827=CARTESIAN_POINT ( 'NONE',  ( -10.81189881249999907, -6.242252689847864744, -130.9687500020483810 ) ) ;
#40828=CARTESIAN_POINT ( 'NONE',  ( 7.070501591499376803E-16, 11.54700538379251284, -104.0000000040967763 ) ) ;
#40831=DIRECTION ( 'NONE',  ( 1.000000000000000000, 0.000000000000000000, 0.000000000000000000 ) ) ;
#40832=EDGE_LOOP ( 'NONE', ( #22570, #17944, #32273, #41748 ) ) ;
#40834=ORIENTED_EDGE ( 'NONE', *, *, #4286, .T. ) ;
#40835=CARTESIAN_POINT ( 'NONE',  ( -5.405949406250003975, -9.363379034771801557, -114.3437500020483810 ) ) ;
#40837=ADVANCED_FACE ( 'NONE', ( #6878 ), #1044, .T. ) ;
#40838=DIRECTION ( 'NONE',  ( -0.000000000000000000, -0.000000000000000000, 1.000000000000000000 ) ) ;
#40839=CARTESIAN_POINT ( 'NONE',  ( 7.644554776091147741E-16, 12.48450537969573659, -191.4687500020484094 ) ) ;
#40840=CARTESIAN_POINT ( 'NONE',  ( -5.405949406250003975, -9.363379034771801557, -37.84375000204837391 ) ) ;
#40841=CARTESIAN_POINT ( 'NONE',  ( 6.060903205933096061, -8.803638040079722060, -4.316514933816155161E-15 ) ) ;
#40842=CARTESIAN_POINT ( 'NONE',  ( 10.00000000000051159, -5.773502691895965988, -74.12499999999995737 ) ) ;
#40843=CARTESIAN_POINT ( 'NONE',  ( 5.405949406249992428, -9.363379034771808662, -169.5937500020484094 ) ) ;
#40844=CARTESIAN_POINT ( 'NONE',  ( 10.81189881249999729, 0.000000000000000000, -160.3437500020484094 ) ) ;
#40849=CARTESIAN_POINT ( 'NONE',  ( 9.999999999999998224, 0.000000000000000000, -42.49999999999998579 ) ) ;
#40852=CARTESIAN_POINT ( 'NONE',  ( 7.644554776091147741E-16, 12.48450537969573659, -89.46875000204838102 ) ) ;
#40854=CARTESIAN_POINT ( 'NONE',  ( 10.81189881249999551, -6.242252689847874514, -55.65625000204836681 ) ) ;
#40856=CARTESIAN_POINT ( 'NONE',  ( 5.405949406249999534, 9.363379034771803333, -118.2812500020483952 ) ) ;
#40857=CARTESIAN_POINT ( 'NONE',  ( 10.81189881249999551, -6.242252689847874514, -157.6562500020484094 ) ) ;
#40858=CARTESIAN_POINT ( 'NONE',  ( -9.999999999999998224, 1.224646799147353059E-15, -200.0000000000000000 ) ) ;
#40860=CARTESIAN_POINT ( 'NONE',  ( 5.000000000000000000, 8.660254037844385522, -129.6250000040967620 ) ) ;
#40862=VERTEX_POINT ( 'NONE', #23282 ) ;
#40865=CARTESIAN_POINT ( 'NONE',  ( 9.999999999999998224, 0.000000000000000000, -68.37500000409677625 ) ) ;
#40866=CARTESIAN_POINT ( 'NONE',  ( 5.405949406249999534, 9.363379034771803333, -181.2812500020483810 ) ) ;
#40867=VERTEX_POINT ( 'NONE', #13747 ) ;
#40868=CARTESIAN_POINT ( 'NONE',  ( 9.999999999999998224, 0.000000000000000000, -49.99999999999998579 ) ) ;
#40870=CARTESIAN_POINT ( 'NONE',  ( 10.00000000000000000, 5.773502691896255534, -54.75000000409678336 ) ) ;
#40871=FACE_OUTER_BOUND ( 'NONE', #6618, .T. ) ;
#40872=DIRECTION ( 'NONE',  ( -0.000000000000000000, -0.000000000000000000, 1.000000000000000000 ) ) ;
#40874=CARTESIAN_POINT ( 'NONE',  ( 10.81189881249999729, 0.000000000000000000, -55.53125000204836681 ) ) ;
#40878=CARTESIAN_POINT ( 'NONE',  ( -5.405949406250003975, -9.363379034771801557, -177.5312500020483810 ) ) ;
#40879=CARTESIAN_POINT ( 'NONE',  ( 9.999999999999998224, 0.000000000000000000, -153.5000000000000000 ) ) ;
#40881=ORIENTED_EDGE ( 'NONE', *, *, #40946, .T. ) ;
#40882=CARTESIAN_POINT ( 'NONE',  ( -10.00000000000051337, 5.773502691895962435, -116.8749999999999858 ) ) ;
#40883=DIRECTION ( 'NONE',  ( 0.000000000000000000, 0.000000000000000000, -1.000000000000000000 ) ) ;
#40884=CARTESIAN_POINT ( 'NONE',  ( 5.405949406249999534, 9.363379034771803333, -86.78125000204838102 ) ) ;
#40885=ORIENTED_EDGE ( 'NONE', *, *, #19089, .T. ) ;
#40888=ORIENTED_EDGE ( 'NONE', *, *, #16988, .F. ) ;
#40889=ORIENTED_EDGE ( 'NONE', *, *, #1662, .T. ) ;
#40890=CARTESIAN_POINT ( 'NONE',  ( -2.293366432827344421E-15, -12.48450537969573659, -39.21875000204835970 ) ) ;
#40891=CARTESIAN_POINT ( 'NONE',  ( -5.405949406250003975, -9.363379034771801557, -27.34375000204835970 ) ) ;
#40892=CARTESIAN_POINT ( 'NONE',  ( 10.81189881249999907, 6.242252689847868297, -11.90625000204835615 ) ) ;
#40893=CARTESIAN_POINT ( 'NONE',  ( -10.81189881249999729, 6.242252689847871849, -65.21875000204838102 ) ) ;
#40894=ORIENTED_EDGE ( 'NONE', *, *, #39777, .F. ) ;
#40895=CARTESIAN_POINT ( 'NONE',  ( 0.000000000000000000, 0.000000000000000000, -200.0000000000000000 ) ) ;
#40896=ADVANCED_FACE ( 'NONE', ( #30616 ), #29765, .T. ) ;
#40898=CARTESIAN_POINT ( 'NONE',  ( 7.644554776091147741E-16, 12.48450537969573659, -188.4687500020484094 ) ) ;
#40899=EDGE_CURVE ( 'NONE', #38354, #10167, #2455, .T. ) ;
#40902=CARTESIAN_POINT ( 'NONE',  ( 7.070501591499376803E-16, 11.54700538379251284, -199.6250000000000284 ) ) ;
#40905=PLANE ( 'NONE',  #13607 ) ;
#40906=CARTESIAN_POINT ( 'NONE',  ( 10.81189881249999551, -6.242252689847874514, -112.4687500020483810 ) ) ;
#40907=DIRECTION ( 'NONE',  ( -0.000000000000000000, -1.000000000000000000, -0.000000000000000000 ) ) ;
#40908=CARTESIAN_POINT ( 'NONE',  ( 10.81189881249999907, 6.242252689847868297, -79.40625000204839523 ) ) ;
#40909=CARTESIAN_POINT ( 'NONE',  ( -10.81189881249999729, 6.242252689847871849, -101.2187500020483810 ) ) ;
#40912=CARTESIAN_POINT ( 'NONE',  ( -9.999999999999998224, 1.224646799147353059E-15, -157.6250000040967905 ) ) ;
#40916=CARTESIAN_POINT ( 'NONE',  ( -4.999999999999996447, 8.660254037844387298, -97.87500000409677625 ) ) ;
#40919=CARTESIAN_POINT ( 'NONE',  ( -5.000000000000003553, -8.660254037844383745, -72.99999999999998579 ) ) ;
#40921=CARTESIAN_POINT ( 'NONE',  ( 5.000000000000000000, 8.660254037844385522, -80.12500000409677625 ) ) ;
#40922=CARTESIAN_POINT ( 'NONE',  ( -10.00000000000154188, 5.773502691895366468, -25.75000000409673362 ) ) ;
#40924=CARTESIAN_POINT ( 'NONE',  ( 5.405949406249999534, 9.363379034771803333, -79.28125000204838102 ) ) ;
#40927=ORIENTED_EDGE ( 'NONE', *, *, #24415, .F. ) ;
#40928=CARTESIAN_POINT ( 'NONE',  ( 9.999999999999996447, -5.773502691896262640, -0.6249999999999709122 ) ) ;
#40931=CARTESIAN_POINT ( 'NONE',  ( 10.81189881249999729, 0.000000000000000000, -10.34375000204834549 ) ) ;
#40932=CARTESIAN_POINT ( 'NONE',  ( -9.999999999999998224, 1.224646799147353059E-15, -64.62500000409676204 ) ) ;
#40934=CARTESIAN_POINT ( 'NONE',  ( -10.81189881249999729, 6.242252689847871849, -126.9062500020483810 ) ) ;
#40935=CARTESIAN_POINT ( 'NONE',  ( 4.999999999999992006, -8.660254037844389075, -185.2500000000000000 ) ) ;
#40936=CYLINDRICAL_SURFACE ( 'NONE', #730, 9.999999999999998224 ) ;
#40937=CARTESIAN_POINT ( 'NONE',  ( -5.405949406249996869, 9.363379034771805109, -109.0312500020483810 ) ) ;
#40938=EDGE_LOOP ( 'NONE', ( #7471, #24836, #5184, #32109 ) ) ;
#40942=CARTESIAN_POINT ( 'NONE',  ( -10.81189881249999907, -6.242252689847864744, -39.65625000204835970 ) ) ;
#40944=CARTESIAN_POINT ( 'NONE',  ( 10.81189881249999729, 0.000000000000000000, -86.84375000204836681 ) ) ;
#40946=EDGE_CURVE ( 'NONE', #3072, #25696, #26727, .T. ) ;
#40947=EDGE_CURVE ( 'NONE', #36017, #16045, #22870, .T. ) ;
#40949=EDGE_CURVE ( 'NONE', #41097, #12174, #817, .T. ) ;
#40950=ADVANCED_FACE ( 'NONE', ( #33002 ), #36651, .T. ) ;
#40952=CARTESIAN_POINT ( 'NONE',  ( -4.999999999999996447, 8.660254037844387298, -138.0000000000000000 ) ) ;
#40953=CARTESIAN_POINT ( 'NONE',  ( 5.405949406249999534, 9.363379034771803333, -122.5937500020483952 ) ) ;
#40956=CARTESIAN_POINT ( 'NONE',  ( 7.644554776091147741E-16, 12.48450537969573659, -4.156250002048351710 ) ) ;
#40959=CARTESIAN_POINT ( 'NONE',  ( 9.999999999999996447, -5.773502691896262640, -179.5000000040968189 ) ) ;
#40960=CARTESIAN_POINT ( 'NONE',  ( -10.81189881249999729, -6.242252689847864744, -167.1562500020484094 ) ) ;
#40961=CARTESIAN_POINT ( 'NONE',  ( -9.999999999998456346, -5.773502691897145489, -28.50000000409671230 ) ) ;
#40964=CARTESIAN_POINT ( 'NONE',  ( -5.405949406250003975, -9.363379034771801557, -55.84375000204835970 ) ) ;
#40966=CARTESIAN_POINT ( 'NONE',  ( -5.405949406250003975, -9.363379034771801557, -14.03125000204835615 ) ) ;
#40970=CARTESIAN_POINT ( 'NONE',  ( 5.000000000000000000, 8.660254037844385522, -100.7499999999999858 ) ) ;
#40972=CARTESIAN_POINT ( 'NONE',  ( 9.999999999999998224, 0.000000000000000000, -105.8750000040967763 ) ) ;
#40973=CARTESIAN_POINT ( 'NONE',  ( 4.999999999999992006, -8.660254037844389075, -190.1250000040967905 ) ) ;
#40976=CARTESIAN_POINT ( 'NONE',  ( -10.81189881249999729, 1.324075727343319199E-15, -96.78125000204839523 ) ) ;
#40981=CARTESIAN_POINT ( 'NONE',  ( -10.81189881249999907, -6.242252689847864744, -164.1562500020484094 ) ) ;
#40983=ORIENTED_EDGE ( 'NONE', *, *, #31744, .T. ) ;
#40984=EDGE_CURVE ( 'NONE', #30365, #38772, #24261, .T. ) ;
#40985=CARTESIAN_POINT ( 'NONE',  ( 4.999999999999992006, -8.660254037844389075, -24.74999999999996803 ) ) ;
#40986=CARTESIAN_POINT ( 'NONE',  ( 5.405949406249999534, 9.363379034771803333, -31.28125000204837036 ) ) ;
#40987=CARTESIAN_POINT ( 'NONE',  ( -10.00000000000000000, -5.773502691896251982, -158.6250000000000284 ) ) ;
#40988=FACE_OUTER_BOUND ( 'NONE', #20289, .T. ) ;
#40990=CARTESIAN_POINT ( 'NONE',  ( -9.999999999998969713, -5.773502691896847949, -23.62499999999995737 ) ) ;
#40991=CARTESIAN_POINT ( 'NONE',  ( -2.293366432827344421E-15, -12.48450537969573659, -133.9062500020483810 ) ) ;
#40992=CARTESIAN_POINT ( 'NONE',  ( -10.00000000000051337, 5.773502691895962435, -139.7500000040967905 ) ) ;
#40994=( BOUNDED_CURVE ( )  B_SPLINE_CURVE ( 2, ( #18884, #19292, #31641, #32486, #12388, #38310, #11970 ),
 .UNSPECIFIED., .F., .F. ) 
 B_SPLINE_CURVE_WITH_KNOTS ( ( 3, 2, 2, 3 ),
 ( 0.04850746268656720706, 0.04975124378109457846, 0.05099502487562193598, 0.05223880597014930738 ),
 .UNSPECIFIED. ) 
 CURVE ( )  GEOMETRIC_REPRESENTATION_ITEM ( )  RATIONAL_B_SPLINE_CURVE ( ( 0.9999999999999955591, 0.8660254037844431485, 1.000000000000000000, 0.8660254037844387076, 1.000000000000000000, 0.8660254037844327124, 1.000000000000005995 ) ) 
 REPRESENTATION_ITEM ( '' )  );
#40995=CARTESIAN_POINT ( 'NONE',  ( 5.405949406249992428, -9.363379034771808662, -61.78125000204837391 ) ) ;
#40996=ORIENTED_EDGE ( 'NONE', *, *, #16948, .T. ) ;
#40997=ORIENTED_EDGE ( 'NONE', *, *, #38893, .T. ) ;
#40999=DIRECTION ( 'NONE',  ( -0.000000000000000000, -0.000000000000000000, 1.000000000000000000 ) ) ;
#41000=CARTESIAN_POINT ( 'NONE',  ( -10.81189881249999729, 1.324075727343319199E-15, -159.5937500020484094 ) ) ;
#41002=CARTESIAN_POINT ( 'NONE',  ( -5.405949406249996869, 9.363379034771805109, -18.84375000204835260 ) ) ;
#41004=CARTESIAN_POINT ( 'NONE',  ( -2.293366432827344421E-15, -12.48450537969573659, -150.2187500020484094 ) ) ;
#41005=CARTESIAN_POINT ( 'NONE',  ( 10.81189881249999729, 0.000000000000000000, -128.8437500020484094 ) ) ;
#41006=CARTESIAN_POINT ( 'NONE',  ( -10.81189881249999729, 6.242252689847871849, -104.4062500020483810 ) ) ;
#41009=CARTESIAN_POINT ( 'NONE',  ( -5.405949406250003975, -9.363379034771801557, -0.3437500020483652552 ) ) ;
#41016=CARTESIAN_POINT ( 'NONE',  ( 7.644554776091147741E-16, 12.48450537969573659, -78.96875000204838102 ) ) ;
#41017=CARTESIAN_POINT ( 'NONE',  ( -10.81189881249999729, 6.242252689847871849, -60.71875000204838102 ) ) ;
#41019=CARTESIAN_POINT ( 'NONE',  ( 10.81189881249999729, 0.000000000000000000, -36.03125000204837391 ) ) ;
#41021=CYLINDRICAL_SURFACE ( 'NONE', #3354, 9.999999999999998224 ) ;
#41023=CARTESIAN_POINT ( 'NONE',  ( -9.999999999999998224, 5.773502691896259087, -121.3750000000000000 ) ) ;
#41024=CARTESIAN_POINT ( 'NONE',  ( -2.121150477449813534E-15, -11.54700538379251284, -187.2500000040967905 ) ) ;
#41027=CARTESIAN_POINT ( 'NONE',  ( 10.81189881249999551, -6.242252689847874514, -9.156250002048375691 ) ) ;
#41028=ORIENTED_EDGE ( 'NONE', *, *, #30335, .F. ) ;
#41031=CARTESIAN_POINT ( 'NONE',  ( -2.121150477449813534E-15, -11.54700538379251284, -179.7500000040967905 ) ) ;
#41033=CARTESIAN_POINT ( 'NONE',  ( -5.000000000000003553, -8.660254037844383745, -35.87500000409676915 ) ) ;
#41037=CARTESIAN_POINT ( 'NONE',  ( -10.81189881249999729, 6.242252689847871849, -153.9062500020483810 ) ) ;
#41038=CARTESIAN_POINT ( 'NONE',  ( -5.405949406250003975, -9.363379034771801557, -129.3437500020484094 ) ) ;
#41039=CARTESIAN_POINT ( 'NONE',  ( 9.999999999999479527, 5.773502691896553074, -104.2500000040967478 ) ) ;
#41040=VERTEX_POINT ( 'NONE', #24361 ) ;
#41041=DIRECTION ( 'NONE',  ( -0.000000000000000000, -0.000000000000000000, 1.000000000000000000 ) ) ;
#41042=ORIENTED_EDGE ( 'NONE', *, *, #4875, .F. ) ;
#41043=ORIENTED_EDGE ( 'NONE', *, *, #40356, .F. ) ;
#41046=CARTESIAN_POINT ( 'NONE',  ( 10.81189881249999729, 0.000000000000000000, -191.8437500020484094 ) ) ;
#41047=CARTESIAN_POINT ( 'NONE',  ( -10.81189881249999907, -6.242252689847864744, -39.46875000204835970 ) ) ;
#41050=CARTESIAN_POINT ( 'NONE',  ( -10.81189881249999729, -6.242252689847864744, -169.9687500020483526 ) ) ;
#41052=CARTESIAN_POINT ( 'NONE',  ( -5.405949406250003975, -9.363379034771801557, -150.3437500020483810 ) ) ;
#41053=CARTESIAN_POINT ( 'NONE',  ( -5.000000000000003553, -8.660254037844383745, -122.8750000040967905 ) ) ;
#41057=CARTESIAN_POINT ( 'NONE',  ( -9.999999999998969713, -5.773502691896847949, -43.12499999999995737 ) ) ;
#41060=CARTESIAN_POINT ( 'NONE',  ( 10.81189881249999551, -6.242252689847874514, -89.96875000204838102 ) ) ;
#41061=CARTESIAN_POINT ( 'NONE',  ( 5.405949406249992428, -9.363379034771808662, -61.78125000204837391 ) ) ;
#41064=CARTESIAN_POINT ( 'NONE',  ( 10.81189881249999551, -6.242252689847874514, -111.1562500020483952 ) ) ;
#41065=CARTESIAN_POINT ( 'NONE',  ( -10.81189881249999729, 1.324075727343319199E-15, -152.2812500020484094 ) ) ;
#41066=CARTESIAN_POINT ( 'NONE',  ( -9.999999999998456346, -5.773502691897145489, -11.62499999999992184 ) ) ;
#41068=CARTESIAN_POINT ( 'NONE',  ( -5.000000000000003553, -8.660254037844383745, -128.8750000040967905 ) ) ;
#41070=VERTEX_POINT ( 'NONE', #21310 ) ;
#41073=CARTESIAN_POINT ( 'NONE',  ( -9.999999999999998224, 1.224646799147353059E-15, -192.1250000040967905 ) ) ;
#41074=CARTESIAN_POINT ( 'NONE',  ( -10.81189881249999907, -6.242252689847864744, -180.6562500020484094 ) ) ;
#41077=CARTESIAN_POINT ( 'NONE',  ( -10.00000000000000000, -5.773502691896251982, -60.00000000409676915 ) ) ;
#41078=CARTESIAN_POINT ( 'NONE',  ( -9.999999999998456346, -5.773502691897145489, -19.12499999999994316 ) ) ;
#41079=( BOUNDED_CURVE ( )  B_SPLINE_CURVE ( 2, ( #32555, #26283, #23041, #39435, #23472, #181, #36413 ),
 .UNSPECIFIED., .F., .F. ) 
 B_SPLINE_CURVE_WITH_KNOTS ( ( 3, 2, 2, 3 ),
 ( 0.7388059701492539766, 0.7400497512437813619, 0.7412935323383087471, 0.7425373134328361324 ),
 .UNSPECIFIED. ) 
 CURVE ( )  GEOMETRIC_REPRESENTATION_ITEM ( )  RATIONAL_B_SPLINE_CURVE ( ( 0.9999999999999761302, 0.8660254037844625774, 1.000000000000000000, 0.8660254037844387076, 1.000000000000000000, 0.8660254037844028474, 1.000000000000035971 ) ) 
 REPRESENTATION_ITEM ( '' )  );
#41080=CARTESIAN_POINT ( 'NONE',  ( 9.999999999999998224, 0.000000000000000000, -135.8750000040967905 ) ) ;
#41082=CARTESIAN_POINT ( 'NONE',  ( 5.405949406249999534, 9.363379034771803333, -49.28125000204838813 ) ) ;
#41083=EDGE_CURVE ( 'NONE', #26629, #8170, #9374, .T. ) ;
#41086=CARTESIAN_POINT ( 'NONE',  ( -5.000000000000003553, -8.660254037844383745, -29.87500000409676204 ) ) ;
#41087=CARTESIAN_POINT ( 'NONE',  ( -5.405949406249996869, 9.363379034771805109, -181.0312500020483810 ) ) ;
#41088=DIRECTION ( 'NONE',  ( -0.000000000000000000, -0.000000000000000000, 1.000000000000000000 ) ) ;
#41089=DIRECTION ( 'NONE',  ( 1.000000000000000000, 0.000000000000000000, 0.000000000000000000 ) ) ;
#41090=VERTEX_POINT ( 'NONE', #1690 ) ;
#41091=CARTESIAN_POINT ( 'NONE',  ( -5.000000000000003553, -8.660254037844383745, -0.9999999999999731326 ) ) ;
#41092=DIRECTION ( 'NONE',  ( 1.000000000000000000, 0.000000000000000000, 0.000000000000000000 ) ) ;
#41093=DIRECTION ( 'NONE',  ( -0.000000000000000000, -0.000000000000000000, 1.000000000000000000 ) ) ;
#41094=CARTESIAN_POINT ( 'NONE',  ( 10.81189881249999907, 6.242252689847868297, -89.90625000204839523 ) ) ;
#41096=DIRECTION ( 'NONE',  ( 1.000000000000000000, -0.000000000000000000, -0.000000000000000000 ) ) ;
#41097=VERTEX_POINT ( 'NONE', #34923 ) ;
#41098=VERTEX_POINT ( 'NONE', #25006 ) ;
#41099=CARTESIAN_POINT ( 'NONE',  ( 10.81189881249999551, -6.242252689847874514, -37.46875000204836681 ) ) ;
#41101=CARTESIAN_POINT ( 'NONE',  ( 5.405949406249999534, 9.363379034771803333, -11.78125000204835438 ) ) ;
#41102=CARTESIAN_POINT ( 'NONE',  ( -2.293366432827344421E-15, -12.48450537969573659, -60.21875000204837391 ) ) ;
#41103=ORIENTED_EDGE ( 'NONE', *, *, #35465, .F. ) ;
#41105=EDGE_CURVE ( 'NONE', #38843, #17527, #14264, .T. ) ;
#41107=CARTESIAN_POINT ( 'NONE',  ( 10.81189881249999907, 6.242252689847868297, -182.7187500020484094 ) ) ;
#41110=EDGE_CURVE ( 'NONE', #22821, #31054, #4978, .T. ) ;
#41111=CARTESIAN_POINT ( 'NONE',  ( -10.00000000000102496, 5.773502691895664007, -131.8749999999999432 ) ) ;
#41113=CARTESIAN_POINT ( 'NONE',  ( -5.000000000000003553, -8.660254037844383745, -20.87500000409675494 ) ) ;
#41115=CARTESIAN_POINT ( 'NONE',  ( 10.81189881249999551, -6.242252689847874514, -115.4687500020483810 ) ) ;
#41116=LINE ( 'NONE', #11555, #20423 ) ;
#41118=CARTESIAN_POINT ( 'NONE',  ( -5.405949406250003975, -9.363379034771801557, -78.53125000204838102 ) ) ;
#41119=CARTESIAN_POINT ( 'NONE',  ( -5.405949406250003975, -9.363379034771801557, -91.84375000204838102 ) ) ;
#41122=CARTESIAN_POINT ( 'NONE',  ( 9.999999999999998224, 0.000000000000000000, -150.8750000040967905 ) ) ;
#41128=CARTESIAN_POINT ( 'NONE',  ( 0.000000000000000000, 0.000000000000000000, -200.0000000000000000 ) ) ;
#41130=CARTESIAN_POINT ( 'NONE',  ( 9.999999999999998224, 0.000000000000000000, -42.87500000409677625 ) ) ;
#41131=CARTESIAN_POINT ( 'NONE',  ( 4.999999999999992006, -8.660254037844389075, -71.24999999999998579 ) ) ;
#41133=CARTESIAN_POINT ( 'NONE',  ( 10.00000000000000000, 5.773502691896255534, -78.75000000409679046 ) ) ;
#41135=CARTESIAN_POINT ( 'NONE',  ( 10.81189881249999729, 0.000000000000000000, -73.53125000204838102 ) ) ;
#41138=CARTESIAN_POINT ( 'NONE',  ( -9.999999999999998224, 1.224646799147353059E-15, -59.74999999999997158 ) ) ;
#41140=EDGE_LOOP ( 'NONE', ( #25398, #6184, #9002, #25164 ) ) ;
#41141=CARTESIAN_POINT ( 'NONE',  ( -5.000000000000003553, -8.660254037844383745, -0.9999999999999731326 ) ) ;
#41144=CARTESIAN_POINT ( 'NONE',  ( 10.81189881249999551, -6.242252689847874514, -13.46875000204836326 ) ) ;
#41146=CARTESIAN_POINT ( 'NONE',  ( 10.81189881249999907, 6.242252689847868297, -143.7187500020483810 ) ) ;
#41147=CARTESIAN_POINT ( 'NONE',  ( -9.999999999999998224, 1.224646799147353059E-15, -66.12500000409676204 ) ) ;
#41149=CARTESIAN_POINT ( 'NONE',  ( -10.81189881249999907, -6.242252689847864744, -132.6562500020484094 ) ) ;
#41150=CARTESIAN_POINT ( 'NONE',  ( 5.000000000000000000, 8.660254037844385522, -181.7500000000000000 ) ) ;
#41151=CARTESIAN_POINT ( 'NONE',  ( 4.999999999999992006, -8.660254037844389075, -35.62500000409676915 ) ) ;
#41152=CARTESIAN_POINT ( 'NONE',  ( 10.81189881249999907, 6.242252689847868297, -110.9062500020483952 ) ) ;
#41153=ORIENTED_EDGE ( 'NONE', *, *, #3222, .F. ) ;
#41154=CARTESIAN_POINT ( 'NONE',  ( 4.999999999999992006, -8.660254037844389075, -154.1250000040967905 ) ) ;
#41155=ORIENTED_EDGE ( 'NONE', *, *, #3091, .F. ) ;
#41156=ORIENTED_EDGE ( 'NONE', *, *, #40070, .F. ) ;
#41157=CARTESIAN_POINT ( 'NONE',  ( -10.81189881249999729, 6.242252689847871849, -38.40625000204835260 ) ) ;
#41159=CARTESIAN_POINT ( 'NONE',  ( -5.405949406249996869, 9.363379034771805109, -90.84375000204838102 ) ) ;
#41163=CARTESIAN_POINT ( 'NONE',  ( 5.000000000000000000, 8.660254037844385522, -123.2500000000000000 ) ) ;
#41165=CARTESIAN_POINT ( 'NONE',  ( -9.999999999999998224, 1.224646799147353059E-15, -54.12500000409675494 ) ) ;
#41166=CARTESIAN_POINT ( 'NONE',  ( 5.405949406249992428, -9.363379034771808662, -112.5937500020483810 ) ) ;
#41168=CARTESIAN_POINT ( 'NONE',  ( -2.293366432827344421E-15, -12.48450537969573659, -4.906250002048355263 ) ) ;
#41171=CARTESIAN_POINT ( 'NONE',  ( -9.999999999999998224, 1.224646799147353059E-15, -180.1250000040968189 ) ) ;
#41172=CARTESIAN_POINT ( 'NONE',  ( -10.81189881249999729, -6.242252689847864744, -173.1562500020484379 ) ) ;
#41173=CARTESIAN_POINT ( 'NONE',  ( -4.999999999999996447, 8.660254037844387298, -103.5000000000000000 ) ) ;
#41176=CARTESIAN_POINT ( 'NONE',  ( -10.81189881249999729, -6.242252689847864744, -54.46875000204838102 ) ) ;
#41178=CARTESIAN_POINT ( 'NONE',  ( -10.81189881249999729, 1.324075727343319199E-15, -8.281250002048350822 ) ) ;
#41180=CARTESIAN_POINT ( 'NONE',  ( -4.999999999999996447, 8.660254037844387298, -53.99999999999996447 ) ) ;
#41182=CARTESIAN_POINT ( 'NONE',  ( -9.999999999999998224, 1.224646799147353059E-15, -94.24999999999998579 ) ) ;
#41184=CARTESIAN_POINT ( 'NONE',  ( -2.121150477449813534E-15, -11.54700538379251284, -109.2500000040967763 ) ) ;
#41185=CARTESIAN_POINT ( 'NONE',  ( 0.000000000000000000, 0.000000000000000000, -200.0000000000000000 ) ) ;
#41188=CARTESIAN_POINT ( 'NONE',  ( -10.81189881249999729, -6.242252689847864744, -96.65625000204839523 ) ) ;
#41191=CARTESIAN_POINT ( 'NONE',  ( -9.999999999999998224, 1.224646799147353059E-15, -141.1250000040967905 ) ) ;
#41192=CARTESIAN_POINT ( 'NONE',  ( 7.644554776091147741E-16, 12.48450537969573659, -160.1562500020484094 ) ) ;
#41195=CARTESIAN_POINT ( 'NONE',  ( 9.999999999999998224, 0.000000000000000000, -28.99999999999997158 ) ) ;
#41198=CARTESIAN_POINT ( 'NONE',  ( 5.405949406249999534, 9.363379034771803333, -25.28125000204836681 ) ) ;
#41199=CARTESIAN_POINT ( 'NONE',  ( -2.121150477449813534E-15, -11.54700538379251284, -162.8750000000000000 ) ) ;
#41201=CARTESIAN_POINT ( 'NONE',  ( 10.00000000000051159, -5.773502691895965988, -90.62499999999997158 ) ) ;
#41203=EDGE_CURVE ( 'NONE', #27433, #7656, #12228, .T. ) ;
#41204=CARTESIAN_POINT ( 'NONE',  ( -1.040834085586084257E-14, -20.00000000000000355, 22.49999999999999289 ) ) ;
#41205=CARTESIAN_POINT ( 'NONE',  ( -10.81189881249999729, 6.242252689847871849, -134.4062500020484094 ) ) ;
#41206=CARTESIAN_POINT ( 'NONE',  ( 9.999999999999998224, 0.000000000000000000, -75.87500000409677625 ) ) ;
#41208=CARTESIAN_POINT ( 'NONE',  ( 10.00000000000102318, -5.773502691895667560, -68.50000000409674783 ) ) ;
#41209=ORIENTED_EDGE ( 'NONE', *, *, #1968, .T. ) ;
#41210=CARTESIAN_POINT ( 'NONE',  ( 10.81189881249999907, 6.242252689847868297, -64.40625000204839523 ) ) ;
#41212=ORIENTED_EDGE ( 'NONE', *, *, #16204, .F. ) ;
#41215=CARTESIAN_POINT ( 'NONE',  ( -4.999999999999996447, 8.660254037844387298, -181.8750000040967905 ) ) ;
#41217=CARTESIAN_POINT ( 'NONE',  ( 5.405949406249999534, 9.363379034771803333, -157.0937500020483810 ) ) ;
#41219=CARTESIAN_POINT ( 'NONE',  ( 10.81189881249999551, -6.242252689847874514, -7.468750002048351710 ) ) ;
#41220=FACE_OUTER_BOUND ( 'NONE', #25271, .T. ) ;
#41221=ADVANCED_FACE ( 'NONE', ( #28453 ), #9636, .T. ) ;
#41222=CARTESIAN_POINT ( 'NONE',  ( -10.81189881249999729, 6.242252689847871849, -146.2187500020484094 ) ) ;
#41224=CARTESIAN_POINT ( 'NONE',  ( 7.644554776091147741E-16, 12.48450537969573659, -103.1562500020483952 ) ) ;
#41226=CARTESIAN_POINT ( 'NONE',  ( 9.999999999999998224, 0.000000000000000000, -55.99999999999996447 ) ) ;
#41228=CARTESIAN_POINT ( 'NONE',  ( -10.81189881249999729, 6.242252689847871849, -5.218750002048340164 ) ) ;
#41230=CARTESIAN_POINT ( 'NONE',  ( -5.405949406249996869, 9.363379034771805109, -193.0312500020484094 ) ) ;
#41234=CARTESIAN_POINT ( 'NONE',  ( 7.644554776091147741E-16, 12.48450537969573659, -74.46875000204838102 ) ) ;
#41235=CARTESIAN_POINT ( 'NONE',  ( 7.644554776091147741E-16, 12.48450537969573659, -60.96875000204838102 ) ) ;
#41237=CARTESIAN_POINT ( 'NONE',  ( 5.405949406249992428, -9.363379034771808662, -31.78125000204837391 ) ) ;
#41241=CARTESIAN_POINT ( 'NONE',  ( -9.999999999999998224, 5.773502691896259087, -119.8750000000000000 ) ) ;
#41245=CARTESIAN_POINT ( 'NONE',  ( -5.405949406250003975, -9.363379034771801557, -14.03125000204835615 ) ) ;
#41246=ORIENTED_EDGE ( 'NONE', *, *, #3499, .F. ) ;
#41249=LINE ( 'NONE', #37821, #180 ) ;
#41251=CARTESIAN_POINT ( 'NONE',  ( -5.000000000000003553, -8.660254037844383745, -32.87500000409676915 ) ) ;
#41252=CARTESIAN_POINT ( 'NONE',  ( 9.999999999999998224, 0.000000000000000000, -200.0000000000000000 ) ) ;
#41256=CARTESIAN_POINT ( 'NONE',  ( -9.999999999999998224, 1.224646799147353059E-15, -23.74999999999996447 ) ) ;
#41257=CARTESIAN_POINT ( 'NONE',  ( 10.81189881249999551, -6.242252689847874514, -142.6562500020484094 ) ) ;
#41258=ADVANCED_FACE ( 'NONE', ( #22808 ), #38788, .T. ) ;
#41259=CARTESIAN_POINT ( 'NONE',  ( 10.81189881249999907, 6.242252689847868297, -125.7187500020483810 ) ) ;
#41260=CARTESIAN_POINT ( 'NONE',  ( -9.999999999999998224, 1.224646799147353059E-15, -59.74999999999997158 ) ) ;
#41264=ORIENTED_EDGE ( 'NONE', *, *, #3396, .F. ) ;
#41265=VECTOR ( 'NONE', #38339, 1000.000000000000000 ) ;
#41266=ORIENTED_EDGE ( 'NONE', *, *, #42334, .F. ) ;
#41267=ORIENTED_EDGE ( 'NONE', *, *, #10010, .F. ) ;
#41268=ADVANCED_FACE ( 'NONE', ( #16088 ), #32113, .T. ) ;
#41269=CARTESIAN_POINT ( 'NONE',  ( -9.999999999999479527, -5.773502691896549521, -145.5000000040967905 ) ) ;
#41270=CARTESIAN_POINT ( 'NONE',  ( 10.81189881249999729, 0.000000000000000000, -181.3437500020483810 ) ) ;
#41271=VECTOR ( 'NONE', #9506, 1000.000000000000000 ) ;
#41272=CARTESIAN_POINT ( 'NONE',  ( -10.81189881249999729, 1.324075727343319199E-15, -42.59375000204837391 ) ) ;
#41273=CARTESIAN_POINT ( 'NONE',  ( 5.000000000000000000, 8.660254037844385522, -110.1250000040967763 ) ) ;
#41274=CARTESIAN_POINT ( 'NONE',  ( 5.405949406249999534, 9.363379034771803333, -173.5937500020484094 ) ) ;
#41275=CARTESIAN_POINT ( 'NONE',  ( -10.81189881249999907, -6.242252689847864744, -153.4687500020484094 ) ) ;
#41276=CARTESIAN_POINT ( 'NONE',  ( -9.999999999999998224, 1.224646799147353059E-15, -200.0000000000000000 ) ) ;
#41280=CARTESIAN_POINT ( 'NONE',  ( -5.000000000000003553, -8.660254037844383745, -152.5000000000000000 ) ) ;
#41281=CARTESIAN_POINT ( 'NONE',  ( 7.070501591499376803E-16, 11.54700538379251284, -33.50000000409676204 ) ) ;
#41283=CARTESIAN_POINT ( 'NONE',  ( 10.81189881249999551, -6.242252689847874514, -82.46875000204836681 ) ) ;
#41284=CARTESIAN_POINT ( 'NONE',  ( -2.121150477449813534E-15, -11.54700538379251284, -135.8750000000000000 ) ) ;
#41285=CARTESIAN_POINT ( 'NONE',  ( 10.81189881249999907, 6.242252689847868297, -59.90625000204838813 ) ) ;
#41288=CARTESIAN_POINT ( 'NONE',  ( -10.81189881249999729, 1.324075727343319199E-15, -114.7812500020483952 ) ) ;
#41289=CARTESIAN_POINT ( 'NONE',  ( -5.405949406249996869, 9.363379034771805109, -154.0312500020484094 ) ) ;
#41290=CARTESIAN_POINT ( 'NONE',  ( 9.999999999998456346, 5.773502691897149042, -15.75000000409673540 ) ) ;
#41292=CARTESIAN_POINT ( 'NONE',  ( -4.999999999999996447, 8.660254037844387298, -120.3750000040967905 ) ) ;
#41294=ORIENTED_EDGE ( 'NONE', *, *, #375, .F. ) ;
#41298=VECTOR ( 'NONE', #5941, 1000.000000000000000 ) ;
#41299=CARTESIAN_POINT ( 'NONE',  ( 5.405949406249992428, -9.363379034771808662, -177.2812500020484094 ) ) ;
#41300=ORIENTED_EDGE ( 'NONE', *, *, #40673, .F. ) ;
#41302=CARTESIAN_POINT ( 'NONE',  ( -2.121150477449813534E-15, -11.54700538379251284, -58.25000000409676915 ) ) ;
#41308=CARTESIAN_POINT ( 'NONE',  ( 9.999999999999998224, 0.000000000000000000, -134.3750000040967905 ) ) ;
#41309=CARTESIAN_POINT ( 'NONE',  ( -10.81189881249999907, -6.242252689847864744, -173.1562500020484094 ) ) ;
#41313=CARTESIAN_POINT ( 'NONE',  ( 9.999999999999998224, 0.000000000000000000, -84.87500000409677625 ) ) ;
#41314=DIRECTION ( 'NONE',  ( 0.8660254037844387076, -0.4999999999999998335, 0.000000000000000000 ) ) ;
#41315=CYLINDRICAL_SURFACE ( 'NONE', #13770, 9.999999999999998224 ) ;
#41316=EDGE_CURVE ( 'NONE', #40345, #4873, #18704, .T. ) ;
#41317=CARTESIAN_POINT ( 'NONE',  ( 10.81189881249999551, -6.242252689847874514, -75.15625000204838102 ) ) ;
#41318=VERTEX_POINT ( 'NONE', #18713 ) ;
#41320=DIRECTION ( 'NONE',  ( -0.7559289460184527298, -1.381779857339538216E-16, -0.6546536707079791961 ) ) ;
#41322=ORIENTED_EDGE ( 'NONE', *, *, #5930, .T. ) ;
#41323=CARTESIAN_POINT ( 'NONE',  ( -5.405949406250003975, -9.363379034771801557, -36.34375000204836681 ) ) ;
#41324=CARTESIAN_POINT ( 'NONE',  ( 4.999999999999992006, -8.660254037844389075, -186.7500000000000000 ) ) ;
#41325=CARTESIAN_POINT ( 'NONE',  ( -10.81189881249999729, 6.242252689847871849, -6.906250002048365033 ) ) ;
#41326=CARTESIAN_POINT ( 'NONE',  ( 5.405949406249999534, 9.363379034771803333, -67.09375000204836681 ) ) ;
#41327=VERTEX_POINT ( 'NONE', #32735 ) ;
#41330=CARTESIAN_POINT ( 'NONE',  ( -10.81189881249999729, 1.324075727343319199E-15, -197.0937500020484094 ) ) ;
#41331=CARTESIAN_POINT ( 'NONE',  ( -5.405949406249996869, 9.363379034771805109, -177.8437500020483810 ) ) ;
#41334=CARTESIAN_POINT ( 'NONE',  ( 7.070501591499376803E-16, 11.54700538379251284, -43.62499999999997158 ) ) ;
#41335=LINE ( 'NONE', #20631, #32937 ) ;
#41336=CARTESIAN_POINT ( 'NONE',  ( -2.121150477449813534E-15, -11.54700538379251284, -101.7500000040967763 ) ) ;
#41338=CARTESIAN_POINT ( 'NONE',  ( 10.81189881249999729, 0.000000000000000000, -103.3437500020483668 ) ) ;
#41340=CARTESIAN_POINT ( 'NONE',  ( 5.405949406249992428, -9.363379034771808662, -81.28125000204839523 ) ) ;
#41341=CARTESIAN_POINT ( 'NONE',  ( 5.405949406249992428, -9.363379034771808662, -91.59375000204838102 ) ) ;
#41344=CARTESIAN_POINT ( 'NONE',  ( 7.070501591499377789E-16, 11.54700538379251284, -152.0000000040967905 ) ) ;
#41349=CARTESIAN_POINT ( 'NONE',  ( -5.000000000000003553, -8.660254037844383745, -182.5000000000000000 ) ) ;
#41351=ORIENTED_EDGE ( 'NONE', *, *, #6560, .F. ) ;
#41352=CARTESIAN_POINT ( 'NONE',  ( -10.00000000000000000, -5.773502691896251982, -67.12500000000000000 ) ) ;
#41354=CARTESIAN_POINT ( 'NONE',  ( -10.00000000000000000, -5.773502691896251982, -85.50000000409677625 ) ) ;
#41356=CARTESIAN_POINT ( 'NONE',  ( -9.999999999999998224, 1.224646799147353059E-15, -7.625000004096743389 ) ) ;
#41358=CARTESIAN_POINT ( 'NONE',  ( 5.405949406249992428, -9.363379034771808662, -78.28125000204838102 ) ) ;
#41360=DIRECTION ( 'NONE',  ( -0.000000000000000000, -0.000000000000000000, 1.000000000000000000 ) ) ;
#41363=CARTESIAN_POINT ( 'NONE',  ( 10.81189881249999907, 6.242252689847868297, -190.4062500020484094 ) ) ;
#41364=VECTOR ( 'NONE', #39836, 1000.000000000000000 ) ;
#41366=CARTESIAN_POINT ( 'NONE',  ( 10.81189881249999729, 6.242252689847867408, -5.718750002048342829 ) ) ;
#41367=CARTESIAN_POINT ( 'NONE',  ( -9.999999999999998224, 1.224646799147353059E-15, -177.1250000040968189 ) ) ;
#41368=CARTESIAN_POINT ( 'NONE',  ( -5.405949406249996869, 9.363379034771805109, -141.8437500020483810 ) ) ;
#41369=CARTESIAN_POINT ( 'NONE',  ( 9.999999999999998224, 0.000000000000000000, -161.3750000040967905 ) ) ;
#41370=EDGE_CURVE ( 'NONE', #30730, #31040, #30309, .T. ) ;
#41371=CARTESIAN_POINT ( 'NONE',  ( 4.999999999999992006, -8.660254037844389075, -180.7500000000000284 ) ) ;
#41372=CARTESIAN_POINT ( 'NONE',  ( -9.999999999998969713, -5.773502691896847949, -36.00000000409673362 ) ) ;
#41373=CARTESIAN_POINT ( 'NONE',  ( 10.81189881249999907, 6.242252689847868297, -104.9062500020483952 ) ) ;
#41375=CARTESIAN_POINT ( 'NONE',  ( 9.999999999999998224, 0.000000000000000000, -195.5000000000000000 ) ) ;
#41376=EDGE_LOOP ( 'NONE', ( #743, #15767, #35393, #3122 ) ) ;
#41377=VERTEX_POINT ( 'NONE', #28872 ) ;
#41378=CARTESIAN_POINT ( 'NONE',  ( 10.81189881249999907, 6.242252689847868297, -34.40625000204836681 ) ) ;
#41380=CARTESIAN_POINT ( 'NONE',  ( -2.293366432827344421E-15, -12.48450537969573659, -85.71875000204838102 ) ) ;
#41383=CARTESIAN_POINT ( 'NONE',  ( -10.00000000000076916, 5.773502691895813221, -125.8749999999999858 ) ) ;
#41384=( BOUNDED_CURVE ( )  B_SPLINE_CURVE ( 2, ( #8383, #5347, #25422, #38360, #18931, #21746, #21533 ),
 .UNSPECIFIED., .F., .F. ) 
 B_SPLINE_CURVE_WITH_KNOTS ( ( 3, 2, 2, 3 ),
 ( 0.7425373134328361324, 0.7437810945273634067, 0.7450248756218907920, 0.7462686567164180662 ),
 .UNSPECIFIED. ) 
 CURVE ( )  GEOMETRIC_REPRESENTATION_ITEM ( )  RATIONAL_B_SPLINE_CURVE ( ( 0.9999999999999641398, 0.8660254037844745678, 1.000000000000000000, 0.8660254037844387076, 1.000000000000000000, 0.8660254037844267172, 1.000000000000011990 ) ) 
 REPRESENTATION_ITEM ( '' )  );
#41385=CARTESIAN_POINT ( 'NONE',  ( 9.999999999999998224, 0.000000000000000000, -110.3750000040967763 ) ) ;
#41387=CARTESIAN_POINT ( 'NONE',  ( -2.121150477449813534E-15, -11.54700538379251284, -198.8750000000000284 ) ) ;
#41388=AXIS2_PLACEMENT_3D ( 'NONE', #13701, #7257, #13287 ) ;
#41389=AXIS2_PLACEMENT_3D ( 'NONE', #18393, #31581, #22069 ) ;
#41390=CARTESIAN_POINT ( 'NONE',  ( 7.644554776091147741E-16, 12.48450537969573659, -114.9687500020483668 ) ) ;
#41392=CARTESIAN_POINT ( 'NONE',  ( -5.405949406250003975, -9.363379034771801557, -3.531250002048374803 ) ) ;
#41395=CARTESIAN_POINT ( 'NONE',  ( -4.999999999999996447, 8.660254037844387298, -174.3750000040968189 ) ) ;
#41396=CARTESIAN_POINT ( 'NONE',  ( -10.81189881249999729, 6.242252689847871849, -168.9062500020484094 ) ) ;
#41397=( BOUNDED_CURVE ( )  B_SPLINE_CURVE ( 2, ( #1817, #30533, #41053, #40414, #14943, #24270, #27921 ),
 .UNSPECIFIED., .F., .F. ) 
 B_SPLINE_CURVE_WITH_KNOTS ( ( 3, 2, 2, 3 ),
 ( 0.3768656716417911334, 0.3781094527363185187, 0.3793532338308459040, 0.3805970149253732338 ),
 .UNSPECIFIED. ) 
 CURVE ( )  GEOMETRIC_REPRESENTATION_ITEM ( )  RATIONAL_B_SPLINE_CURVE ( ( 0.9999999999999880096, 0.8660254037844506980, 1.000000000000000000, 0.8660254037844387076, 1.000000000000000000, 0.8660254037844267172, 1.000000000000011990 ) ) 
 REPRESENTATION_ITEM ( '' )  );
#41398=CARTESIAN_POINT ( 'NONE',  ( 9.999999999999998224, 0.000000000000000000, -0.8750000040967653714 ) ) ;
#41401=CARTESIAN_POINT ( 'NONE',  ( -10.81189881249999729, 6.242252689847871849, -42.71875000204835970 ) ) ;
#41403=CARTESIAN_POINT ( 'NONE',  ( 10.81189881249999551, -6.242252689847874514, -3.156250002048346381 ) ) ;
#41405=CARTESIAN_POINT ( 'NONE',  ( -9.999999999999742428, -5.773502691896402084, -159.0000000040967905 ) ) ;
#41407=CARTESIAN_POINT ( 'NONE',  ( -4.999999999999996447, 8.660254037844387298, -86.99999999999998579 ) ) ;
#41409=CARTESIAN_POINT ( 'NONE',  ( -9.999999999999998224, 5.773502691896259087, -105.2500000040967763 ) ) ;
#41410=CARTESIAN_POINT ( 'NONE',  ( 9.999999999999998224, 0.000000000000000000, -14.37500000409674961 ) ) ;
#41413=CARTESIAN_POINT ( 'NONE',  ( -10.81189881249999729, -6.242252689847864744, -102.6562500020483952 ) ) ;
#41417=CARTESIAN_POINT ( 'NONE',  ( 10.81189881249999729, 0.000000000000000000, -159.0312500020484094 ) ) ;
#41420=CARTESIAN_POINT ( 'NONE',  ( -5.000000000000003553, -8.660254037844383745, -23.49999999999996447 ) ) ;
#41421=CARTESIAN_POINT ( 'NONE',  ( -10.81189881249999729, 6.242252689847871849, -30.90625000204834905 ) ) ;
#41422=CARTESIAN_POINT ( 'NONE',  ( -9.999999999999998224, 5.773502691896259087, -158.8749999999999716 ) ) ;
#41426=CARTESIAN_POINT ( 'NONE',  ( -2.121150477449813534E-15, -11.54700538379251284, -23.37499999999998224 ) ) ;
#41427=CARTESIAN_POINT ( 'NONE',  ( 10.81189881249999729, 0.000000000000000000, -132.0312500020484094 ) ) ;
#41428=CARTESIAN_POINT ( 'NONE',  ( 9.999999999999998224, 0.000000000000000000, -45.49999999999998579 ) ) ;
#41429=CARTESIAN_POINT ( 'NONE',  ( -9.999999999999998224, 1.224646799147353059E-15, -157.2500000000000000 ) ) ;
#41431=CARTESIAN_POINT ( 'NONE',  ( -5.405949406249996869, 9.363379034771805109, -58.03125000204836681 ) ) ;
#41435=CARTESIAN_POINT ( 'NONE',  ( -5.000000000000003553, -8.660254037844383745, -121.0000000000000000 ) ) ;
#41436=DIRECTION ( 'NONE',  ( -0.000000000000000000, -0.000000000000000000, 1.000000000000000000 ) ) ;
#41437=CARTESIAN_POINT ( 'NONE',  ( -2.293366432827344421E-15, -12.48450537969573659, -157.7187500020484094 ) ) ;
#41439=CARTESIAN_POINT ( 'NONE',  ( 10.81189881249999907, 6.242252689847868297, -8.718750002048356151 ) ) ;
#41440=EDGE_CURVE ( 'NONE', #10196, #18513, #40740, .T. ) ;
#41441=CARTESIAN_POINT ( 'NONE',  ( -10.81189881249999729, 6.242252689847871849, -137.2187500020483810 ) ) ;
#41442=EDGE_CURVE ( 'NONE', #16199, #19338, #5411, .T. ) ;
#41443=CARTESIAN_POINT ( 'NONE',  ( -5.405949406249996869, 9.363379034771805109, -95.53125000204838102 ) ) ;
#41445=CARTESIAN_POINT ( 'NONE',  ( 7.070501591499376803E-16, 11.54700538379251284, -187.6250000000000000 ) ) ;
#41447=CARTESIAN_POINT ( 'NONE',  ( -2.293366432827344421E-15, -12.48450537969573659, -0.2187500020483489072 ) ) ;
#41449=VECTOR ( 'NONE', #29080, 1000.000000000000000 ) ;
#41450=CARTESIAN_POINT ( 'NONE',  ( -10.81189881249999729, -6.242252689847864744, -194.1562500020484094 ) ) ;
#41451=CARTESIAN_POINT ( 'NONE',  ( 7.070501591499376803E-16, 11.54700538379251284, -165.5000000040967905 ) ) ;
#41455=CARTESIAN_POINT ( 'NONE',  ( -2.293366432827344421E-15, -12.48450537969573659, -64.71875000204838102 ) ) ;
#41456=CARTESIAN_POINT ( 'NONE',  ( -10.81189881249999907, -6.242252689847864744, -57.46875000204835970 ) ) ;
#41458=CARTESIAN_POINT ( 'NONE',  ( 5.405949406249992428, -9.363379034771808662, -30.28125000204837036 ) ) ;
#41460=CARTESIAN_POINT ( 'NONE',  ( -9.999999999999998224, 1.224646799147353059E-15, -52.62500000409675494 ) ) ;
#41462=CARTESIAN_POINT ( 'NONE',  ( 9.999999999999998224, 0.000000000000000000, -120.5000000000000000 ) ) ;
#41463=CARTESIAN_POINT ( 'NONE',  ( -9.999999999999998224, 1.224646799147353059E-15, -41.74999999999997868 ) ) ;
#41466=CARTESIAN_POINT ( 'NONE',  ( 5.405949406249992428, -9.363379034771808662, -6.281250002048377468 ) ) ;
#41473=CARTESIAN_POINT ( 'NONE',  ( -5.000000000000003553, -8.660254037844383745, -25.37500000409675849 ) ) ;
#41475=( BOUNDED_CURVE ( )  B_SPLINE_CURVE ( 2, ( #27464, #10826, #40599, #41024, #33524, #3947, #11042 ),
 .UNSPECIFIED., .F., .F. ) 
 B_SPLINE_CURVE_WITH_KNOTS ( ( 3, 2, 2, 3 ),
 ( 0.05597014925373139382, 0.05721393034825875828, 0.05845771144278612275, 0.05970149253731348721 ),
 .UNSPECIFIED. ) 
 CURVE ( )  GEOMETRIC_REPRESENTATION_ITEM ( )  RATIONAL_B_SPLINE_CURVE ( ( 0.9999999999999947820, 0.8660254037844439257, 1.000000000000000000, 0.8660254037844387076, 1.000000000000000000, 0.8660254037844327124, 1.000000000000005995 ) ) 
 REPRESENTATION_ITEM ( '' )  );
#41476=FACE_OUTER_BOUND ( 'NONE', #17637, .T. ) ;
#41478=CARTESIAN_POINT ( 'NONE',  ( 9.999999999999998224, 0.000000000000000000, -200.0000000000000000 ) ) ;
#41479=CARTESIAN_POINT ( 'NONE',  ( 5.405949406249992428, -9.363379034771808662, -148.7812500020483810 ) ) ;
#41480=CARTESIAN_POINT ( 'NONE',  ( -10.81189881249999729, 6.242252689847871849, -128.2187500020483810 ) ) ;
#41481=CARTESIAN_POINT ( 'NONE',  ( 7.070501591499376803E-16, 11.54700538379251284, -51.12499999999998579 ) ) ;
#41482=CARTESIAN_POINT ( 'NONE',  ( 10.00000000000102318, -5.773502691895667560, -57.62499999999995737 ) ) ;
#41483=ORIENTED_EDGE ( 'NONE', *, *, #356, .F. ) ;
#41485=VERTEX_POINT ( 'NONE', #31322 ) ;
#41486=EDGE_LOOP ( 'NONE', ( #532, #25822, #13324, #1158 ) ) ;
#41487=CARTESIAN_POINT ( 'NONE',  ( -9.999999999998456346, -5.773502691897145489, -7.500000004096707862 ) ) ;
#41488=CARTESIAN_POINT ( 'NONE',  ( 10.81189881249999907, 6.242252689847868297, -179.7187500020484094 ) ) ;
#41489=AXIS2_PLACEMENT_3D ( 'NONE', #41204, #8220, #4980 ) ;
#41490=CARTESIAN_POINT ( 'NONE',  ( 5.405949406249992428, -9.363379034771808662, -31.59375000204836681 ) ) ;
#41491=CARTESIAN_POINT ( 'NONE',  ( 10.00000000000102318, -5.773502691895667560, -41.12499999999993605 ) ) ;
#41492=ADVANCED_FACE ( 'NONE', ( #1964 ), #7798, .T. ) ;
#41493=CARTESIAN_POINT ( 'NONE',  ( 10.81189881249999729, 0.000000000000000000, -160.3437500020484094 ) ) ;
#41494=CARTESIAN_POINT ( 'NONE',  ( 5.405949406249999534, 9.363379034771803333, -155.5937500020483810 ) ) ;
#41495=DIRECTION ( 'NONE',  ( -0.000000000000000000, -0.000000000000000000, 1.000000000000000000 ) ) ;
#41499=EDGE_CURVE ( 'NONE', #12699, #15995, #30055, .T. ) ;
#41500=CARTESIAN_POINT ( 'NONE',  ( 11.54700538379253416, -19.99999999999999289, 45.00000000000009237 ) ) ;
#41503=EDGE_CURVE ( 'NONE', #3056, #6810, #34477, .T. ) ;
#41504=CARTESIAN_POINT ( 'NONE',  ( 5.405949406249992428, -9.363379034771808662, -81.09375000204838102 ) ) ;
#41506=CARTESIAN_POINT ( 'NONE',  ( 7.644554776091147741E-16, 12.48450537969573659, -59.65625000204838813 ) ) ;
#41509=CARTESIAN_POINT ( 'NONE',  ( -5.405949406250003975, -9.363379034771801557, -116.0312500020483952 ) ) ;
#41510=CARTESIAN_POINT ( 'NONE',  ( 10.81189881249999729, 6.242252689847867408, -143.9062500020484094 ) ) ;
#41512=CARTESIAN_POINT ( 'NONE',  ( -9.999999999998456346, -5.773502691897145489, -29.62499999999991829 ) ) ;
#41514=CARTESIAN_POINT ( 'NONE',  ( -10.00000000000000000, -5.773502691896251982, -121.5000000040967905 ) ) ;
#41517=( BOUNDED_CURVE ( )  B_SPLINE_CURVE ( 2, ( #12891, #39236, #16122, #32149, #29532, #29319, #42674 ),
 .UNSPECIFIED., .F., .F. ) 
 B_SPLINE_CURVE_WITH_KNOTS ( ( 3, 2, 2, 3 ),
 ( 0.3582089552238806873, 0.3594527363184080726, 0.3606965174129355134, 0.3619402985074628432 ),
 .UNSPECIFIED. ) 
 CURVE ( )  GEOMETRIC_REPRESENTATION_ITEM ( )  RATIONAL_B_SPLINE_CURVE ( ( 0.9999999999999880096, 0.8660254037844506980, 1.000000000000000000, 0.8660254037844387076, 1.000000000000000000, 0.8660254037844207220, 1.000000000000017986 ) ) 
 REPRESENTATION_ITEM ( '' )  );
#41518=ORIENTED_EDGE ( 'NONE', *, *, #17831, .F. ) ;
#41521=CARTESIAN_POINT ( 'NONE',  ( 7.070501591499376803E-16, 11.54700538379251284, -68.00000000409679046 ) ) ;
#41522=CARTESIAN_POINT ( 'NONE',  ( 5.405949406249999534, 9.363379034771803333, -178.2812500020484094 ) ) ;
#41523=EDGE_LOOP ( 'NONE', ( #31586, #12420, #29992, #5566 ) ) ;
#41525=CARTESIAN_POINT ( 'NONE',  ( 9.999999999999998224, 0.000000000000000000, -50.37500000409675494 ) ) ;
#41526=CARTESIAN_POINT ( 'NONE',  ( -9.999999999999998224, 1.224646799147353059E-15, -145.2500000000000000 ) ) ;
#41527=FACE_OUTER_BOUND ( 'NONE', #36185, .T. ) ;
#41530=CARTESIAN_POINT ( 'NONE',  ( 9.999999999999998224, 0.000000000000000000, -84.49999999999997158 ) ) ;
#41531=CARTESIAN_POINT ( 'NONE',  ( -10.81189881249999729, 1.324075727343319199E-15, -170.2812500020484094 ) ) ;
#41532=EDGE_CURVE ( 'NONE', #18570, #8575, #36094, .T. ) ;
#41533=VECTOR ( 'NONE', #40, 1000.000000000000000 ) ;
#41534=CARTESIAN_POINT ( 'NONE',  ( -10.00000000000031797, 5.773502691896072569, -183.2500000040967905 ) ) ;
#41535=CARTESIAN_POINT ( 'NONE',  ( -2.121150477449813534E-15, -11.54700538379251284, -34.25000000409674783 ) ) ;
#41537=CYLINDRICAL_SURFACE ( 'NONE', #22891, 9.999999999999998224 ) ;
#41538=CARTESIAN_POINT ( 'NONE',  ( 9.999999999999998224, 0.000000000000000000, -111.4999999999999858 ) ) ;
#41540=CARTESIAN_POINT ( 'NONE',  ( 5.405949406249999534, 9.363379034771803333, -76.28125000204838102 ) ) ;
#41542=CARTESIAN_POINT ( 'NONE',  ( 4.999999999999992006, -8.660254037844389075, -143.2500000000000000 ) ) ;
#41543=ORIENTED_EDGE ( 'NONE', *, *, #36546, .F. ) ;
#41544=VERTEX_POINT ( 'NONE', #41428 ) ;
#41545=CARTESIAN_POINT ( 'NONE',  ( 10.81189881249999729, 0.000000000000000000, -26.84375000204835970 ) ) ;
#41546=CARTESIAN_POINT ( 'NONE',  ( 10.00000000000031619, -5.773502691896077010, -186.6250000000000284 ) ) ;
#41547=CARTESIAN_POINT ( 'NONE',  ( 5.405949406249999534, 9.363379034771803333, -4.281250002048375691 ) ) ;
#41548=CARTESIAN_POINT ( 'NONE',  ( -10.81189881249999729, 6.242252689847871849, -57.71875000204836681 ) ) ;
#41552=CARTESIAN_POINT ( 'NONE',  ( 7.644554776091147741E-16, 12.48450537969573659, -194.4687500020484094 ) ) ;
#41553=CARTESIAN_POINT ( 'NONE',  ( 5.405949406249999534, 9.363379034771803333, -179.5937500020484094 ) ) ;
#41555=DIRECTION ( 'NONE',  ( -0.000000000000000000, -0.000000000000000000, 1.000000000000000000 ) ) ;
#41558=CARTESIAN_POINT ( 'NONE',  ( 10.81189881249999907, 6.242252689847868297, -106.2187500020483668 ) ) ;
#41559=FACE_OUTER_BOUND ( 'NONE', #18614, .T. ) ;
#41560=CARTESIAN_POINT ( 'NONE',  ( -5.405949406250003975, -9.363379034771801557, -84.53125000204838102 ) ) ;
#41561=CARTESIAN_POINT ( 'NONE',  ( -10.81189881249999729, 6.242252689847871849, -89.21875000204838102 ) ) ;
#41563=CARTESIAN_POINT ( 'NONE',  ( 4.999999999999992006, -8.660254037844389075, -146.6250000040967905 ) ) ;
#41568=EDGE_CURVE ( 'NONE', #41596, #36111, #20254, .T. ) ;
#41569=CARTESIAN_POINT ( 'NONE',  ( 9.999999999999998224, 0.000000000000000000, -39.49999999999997868 ) ) ;
#41570=DIRECTION ( 'NONE',  ( -0.000000000000000000, -0.000000000000000000, 1.000000000000000000 ) ) ;
#41573=CARTESIAN_POINT ( 'NONE',  ( -9.999999999999998224, 1.224646799147353059E-15, -68.74999999999997158 ) ) ;
#41575=CARTESIAN_POINT ( 'NONE',  ( -4.999999999999996447, 8.660254037844387298, -72.37500000409677625 ) ) ;
#41579=CARTESIAN_POINT ( 'NONE',  ( 5.405949406249999534, 9.363379034771803333, -77.78125000204838102 ) ) ;
#41581=CARTESIAN_POINT ( 'NONE',  ( -9.999999999999998224, 1.224646799147353059E-15, -200.0000000000000000 ) ) ;
#41584=CARTESIAN_POINT ( 'NONE',  ( -5.405949406250003975, -9.363379034771801557, -195.5312500020484094 ) ) ;
#41586=CARTESIAN_POINT ( 'NONE',  ( -5.405949406249996869, 9.363379034771805109, -6.843750002048371250 ) ) ;
#41588=CARTESIAN_POINT ( 'NONE',  ( 7.644554776091147741E-16, 12.48450537969573659, -144.9687500020483810 ) ) ;
#41590=CARTESIAN_POINT ( 'NONE',  ( -5.000000000000003553, -8.660254037844383745, -173.5000000000000284 ) ) ;
#41591=CARTESIAN_POINT ( 'NONE',  ( -9.999999999999998224, 1.224646799147353059E-15, -170.7500000000000000 ) ) ;
#41592=CARTESIAN_POINT ( 'NONE',  ( -4.999999999999996447, 8.660254037844387298, -175.8750000040967905 ) ) ;
#41593=CARTESIAN_POINT ( 'NONE',  ( -5.405949406250003975, -9.363379034771801557, -99.53125000204839523 ) ) ;
#41594=ORIENTED_EDGE ( 'NONE', *, *, #32029, .F. ) ;
#41595=CARTESIAN_POINT ( 'NONE',  ( 4.999999999999992006, -8.660254037844389075, -164.2500000000000000 ) ) ;
#41596=VERTEX_POINT ( 'NONE', #41848 ) ;
#41598=CARTESIAN_POINT ( 'NONE',  ( 5.405949406249999534, 9.363379034771803333, -32.78125000204837391 ) ) ;
#41599=CARTESIAN_POINT ( 'NONE',  ( 5.405949406249999534, 9.363379034771803333, -79.09375000204838102 ) ) ;
#41601=CARTESIAN_POINT ( 'NONE',  ( 9.999999999999742428, 5.773502691896404748, -126.3749999999999858 ) ) ;
#41602=( BOUNDED_CURVE ( )  B_SPLINE_CURVE ( 2, ( #9009, #41794, #32535, #19141, #29284, #12232, #25423 ),
 .UNSPECIFIED., .F., .F. ) 
 B_SPLINE_CURVE_WITH_KNOTS ( ( 3, 2, 2, 3 ),
 ( 0.1940298507462686894, 0.1952736318407960470, 0.1965174129353234322, 0.1977611940298507898 ),
 .UNSPECIFIED. ) 
 CURVE ( )  GEOMETRIC_REPRESENTATION_ITEM ( )  RATIONAL_B_SPLINE_CURVE ( ( 0.9999999999999970024, 0.8660254037844417052, 1.000000000000000000, 0.8660254037844387076, 1.000000000000000000, 0.8660254037844327124, 1.000000000000005995 ) ) 
 REPRESENTATION_ITEM ( '' )  );
#41605=CARTESIAN_POINT ( 'NONE',  ( -10.00000000000000000, -5.773502691896251982, -10.50000000409676204 ) ) ;
#41606=CARTESIAN_POINT ( 'NONE',  ( 9.999999999999998224, 0.000000000000000000, -36.87500000409676915 ) ) ;
#41607=CARTESIAN_POINT ( 'NONE',  ( 5.405949406249992428, -9.363379034771808662, -118.5937500020483810 ) ) ;
#41611=CARTESIAN_POINT ( 'NONE',  ( -9.999999999999998224, 5.773502691896259087, -168.2500000040967905 ) ) ;
#41612=CARTESIAN_POINT ( 'NONE',  ( -5.405949406250003975, -9.363379034771801557, -171.5312500020484094 ) ) ;
#41613=CARTESIAN_POINT ( 'NONE',  ( -2.121150477449813534E-15, -11.54700538379251284, -28.25000000409675138 ) ) ;
#41616=CARTESIAN_POINT ( 'NONE',  ( 10.81189881249999551, -6.242252689847874514, -41.96875000204834549 ) ) ;
#41618=CARTESIAN_POINT ( 'NONE',  ( -2.293366432827344421E-15, -12.48450537969573659, -3.406250002048348158 ) ) ;
#41620=CARTESIAN_POINT ( 'NONE',  ( 4.999999999999992006, -8.660254037844389075, -158.6250000040967905 ) ) ;
#41622=CARTESIAN_POINT ( 'NONE',  ( -5.000000000000003553, -8.660254037844383745, -87.99999999999998579 ) ) ;
#41624=CARTESIAN_POINT ( 'NONE',  ( 5.000000000000000000, 8.660254037844385522, -105.6250000040967763 ) ) ;
#41625=CARTESIAN_POINT ( 'NONE',  ( 0.000000000000000000, 0.000000000000000000, -200.0000000000000000 ) ) ;
#41627=CARTESIAN_POINT ( 'NONE',  ( -10.81189881249999729, 1.324075727343319199E-15, -102.7812500020483952 ) ) ;
#41628=VERTEX_POINT ( 'NONE', #28723 ) ;
#41631=CARTESIAN_POINT ( 'NONE',  ( 10.81189881249999907, 6.242252689847868297, -154.4062500020484094 ) ) ;
#41633=EDGE_LOOP ( 'NONE', ( #10003, #27295, #26472, #4930 ) ) ;
#41634=CARTESIAN_POINT ( 'NONE',  ( 9.999999999999998224, 0.000000000000000000, -16.99999999999996092 ) ) ;
#41635=CARTESIAN_POINT ( 'NONE',  ( -5.405949406249996869, 9.363379034771805109, -31.03125000204837036 ) ) ;
#41636=CARTESIAN_POINT ( 'NONE',  ( 10.00000000000000000, 5.773502691896255534, -154.8750000000000000 ) ) ;
#41638=EDGE_CURVE ( 'NONE', #30453, #29986, #6603, .T. ) ;
#41639=CARTESIAN_POINT ( 'NONE',  ( -9.999999999999998224, 1.224646799147353059E-15, -196.2500000000000000 ) ) ;
#41640=CARTESIAN_POINT ( 'NONE',  ( -5.405949406250003975, -9.363379034771801557, -125.0312500020483952 ) ) ;
#41641=CARTESIAN_POINT ( 'NONE',  ( -5.000000000000003553, -8.660254037844383745, -21.99999999999996447 ) ) ;
#41644=( BOUNDED_CURVE ( )  B_SPLINE_CURVE ( 2, ( #10568, #39508, #30456, #40140, #883, #16611, #9938 ),
 .UNSPECIFIED., .F., .F. ) 
 B_SPLINE_CURVE_WITH_KNOTS ( ( 3, 2, 2, 3 ),
 ( 0.9589552238805971740, 0.9601990049751244483, 0.9614427860696519446, 0.9626865671641793298 ),
 .UNSPECIFIED. ) 
 CURVE ( )  GEOMETRIC_REPRESENTATION_ITEM ( )  RATIONAL_B_SPLINE_CURVE ( ( 0.9999999999999880096, 0.8660254037844506980, 1.000000000000000000, 0.8660254037844387076, 1.000000000000000000, 0.8660254037844148378, 1.000000000000023981 ) ) 
 REPRESENTATION_ITEM ( '' )  );
#41645=CARTESIAN_POINT ( 'NONE',  ( 10.81189881249999551, -6.242252689847874514, -55.65625000204836681 ) ) ;
#41647=CARTESIAN_POINT ( 'NONE',  ( 5.405949406249992428, -9.363379034771808662, -114.0937500020483810 ) ) ;
#41648=ORIENTED_EDGE ( 'NONE', *, *, #5631, .F. ) ;
#41649=ORIENTED_EDGE ( 'NONE', *, *, #11440, .F. ) ;
#41652=CARTESIAN_POINT ( 'NONE',  ( 10.81189881249999907, 6.242252689847868297, -157.2187500020483810 ) ) ;
#41653=( BOUNDED_CURVE ( )  B_SPLINE_CURVE ( 2, ( #27007, #30889, #14457, #4555, #24429, #1109, #24210 ),
 .UNSPECIFIED., .F., .F. ) 
 B_SPLINE_CURVE_WITH_KNOTS ( ( 3, 2, 2, 3 ),
 ( 0.2574626865671643117, 0.2587064676616916414, 0.2599502487562190267, 0.2611940298507463565 ),
 .UNSPECIFIED. ) 
 CURVE ( )  GEOMETRIC_REPRESENTATION_ITEM ( )  RATIONAL_B_SPLINE_CURVE ( ( 0.9999999999999880096, 0.8660254037844506980, 1.000000000000000000, 0.8660254037844387076, 1.000000000000000000, 0.8660254037844267172, 1.000000000000011990 ) ) 
 REPRESENTATION_ITEM ( '' )  );
#41655=CARTESIAN_POINT ( 'NONE',  ( 10.81189881249999551, -6.242252689847874514, -5.968750002048344605 ) ) ;
#41656=EDGE_CURVE ( 'NONE', #20021, #22821, #41887, .T. ) ;
#41657=CARTESIAN_POINT ( 'NONE',  ( -10.81189881249999729, 6.242252689847871849, -143.2187500020483810 ) ) ;
#41659=CARTESIAN_POINT ( 'NONE',  ( 9.999999999999998224, 0.000000000000000000, -188.0000000000000000 ) ) ;
#41661=CARTESIAN_POINT ( 'NONE',  ( 10.81189881249999907, 6.242252689847868297, -5.718750002048342829 ) ) ;
#41663=CARTESIAN_POINT ( 'NONE',  ( -10.81189881249999729, 1.324075727343319199E-15, -197.2812500020484094 ) ) ;
#41667=CARTESIAN_POINT ( 'NONE',  ( -10.81189881249999729, 6.242252689847871849, -69.71875000204838102 ) ) ;
#41668=CARTESIAN_POINT ( 'NONE',  ( 7.644554776091147741E-16, 12.48450537969573659, -56.46875000204837391 ) ) ;
#41670=CARTESIAN_POINT ( 'NONE',  ( 5.405949406249999534, 9.363379034771803333, -26.78125000204836681 ) ) ;
#41672=CARTESIAN_POINT ( 'NONE',  ( 5.000000000000000000, 8.660254037844385522, -95.12500000409677625 ) ) ;
#41674=CARTESIAN_POINT ( 'NONE',  ( 9.999999999999998224, 0.000000000000000000, -115.9999999999999858 ) ) ;
#41678=CARTESIAN_POINT ( 'NONE',  ( -10.81189881249999729, -6.242252689847864744, -9.656250002048379244 ) ) ;
#41680=CARTESIAN_POINT ( 'NONE',  ( 9.999999999999998224, 0.000000000000000000, -61.99999999999997158 ) ) ;
#41682=CARTESIAN_POINT ( 'NONE',  ( -10.00000000000154188, 5.773502691895366468, -8.874999999999937828 ) ) ;
#41684=CARTESIAN_POINT ( 'NONE',  ( -9.999999999999998224, 5.773502691896259087, -38.87499999999995737 ) ) ;
#41685=CARTESIAN_POINT ( 'NONE',  ( 7.070501591499377789E-16, 11.54700538379251284, -23.00000000409677270 ) ) ;
#41686=CARTESIAN_POINT ( 'NONE',  ( -9.999999999999998224, 1.224646799147353059E-15, -142.2500000000000000 ) ) ;
#41688=CARTESIAN_POINT ( 'NONE',  ( -2.121150477449813534E-15, -11.54700538379251284, -99.87500000000000000 ) ) ;
#41689=CARTESIAN_POINT ( 'NONE',  ( -2.293366432827344421E-15, -12.48450537969573659, -141.4062500020483810 ) ) ;
#41690=CARTESIAN_POINT ( 'NONE',  ( -5.405949406249996869, 9.363379034771805109, -148.0312500020483810 ) ) ;
#41691=CARTESIAN_POINT ( 'NONE',  ( -10.00000000000154188, 5.773502691895366468, -59.87499999999995026 ) ) ;
#41692=EDGE_CURVE ( 'NONE', #41040, #13865, #28679, .T. ) ;
#41695=ORIENTED_EDGE ( 'NONE', *, *, #6508, .T. ) ;
#41696=ORIENTED_EDGE ( 'NONE', *, *, #40550, .F. ) ;
#41697=CARTESIAN_POINT ( 'NONE',  ( -9.999999999999998224, 1.224646799147353059E-15, -100.6250000040967905 ) ) ;
#41698=CARTESIAN_POINT ( 'NONE',  ( 10.81189881249999907, 6.242252689847868297, -178.2187500020483810 ) ) ;
#41699=CARTESIAN_POINT ( 'NONE',  ( -10.81189881249999907, -6.242252689847864744, -30.46875000204834549 ) ) ;
#41700=DIRECTION ( 'NONE',  ( 1.000000000000000000, 0.000000000000000000, 0.000000000000000000 ) ) ;
#41701=CARTESIAN_POINT ( 'NONE',  ( 10.81189881249999729, 6.242252689847867408, -166.2187500020483810 ) ) ;
#41702=CARTESIAN_POINT ( 'NONE',  ( -5.405949406250003975, -9.363379034771801557, -156.3437500020483810 ) ) ;
#41704=VECTOR ( 'NONE', #27197, 1000.000000000000000 ) ;
#41707=CARTESIAN_POINT ( 'NONE',  ( -9.999999999999742428, -5.773502691896402084, -152.6249999999999716 ) ) ;
#41708=CARTESIAN_POINT ( 'NONE',  ( -9.999999999999998224, 1.224646799147353059E-15, -75.12500000409677625 ) ) ;
#41710=CARTESIAN_POINT ( 'NONE',  ( -10.81189881249999729, 1.324075727343319199E-15, -83.09375000204836681 ) ) ;
#41711=CARTESIAN_POINT ( 'NONE',  ( 5.405949406249992428, -9.363379034771808662, -52.78125000204836681 ) ) ;
#41712=DIRECTION ( 'NONE',  ( -0.000000000000000000, -0.000000000000000000, 1.000000000000000000 ) ) ;
#41714=CARTESIAN_POINT ( 'NONE',  ( 4.999999999999992006, -8.660254037844389075, -134.2499999999999716 ) ) ;
#41715=VECTOR ( 'NONE', #14451, 1000.000000000000000 ) ;
#41716=CARTESIAN_POINT ( 'NONE',  ( -10.81189881249999729, -6.242252689847864744, -149.1562500020484094 ) ) ;
#41717=( BOUNDED_CURVE ( )  B_SPLINE_CURVE ( 2, ( #36050, #16374, #3248, #19424, #16166, #42501, #12929 ),
 .UNSPECIFIED., .F., .F. ) 
 B_SPLINE_CURVE_WITH_KNOTS ( ( 3, 2, 2, 3 ),
 ( 0.06343283582089558059, 0.06467661691542293811, 0.06592039800995032339, 0.06716417910447768091 ),
 .UNSPECIFIED. ) 
 CURVE ( )  GEOMETRIC_REPRESENTATION_ITEM ( )  RATIONAL_B_SPLINE_CURVE ( ( 0.9999999999999940048, 0.8660254037844447028, 1.000000000000000000, 0.8660254037844387076, 1.000000000000000000, 0.8660254037844312691, 1.000000000000007550 ) ) 
 REPRESENTATION_ITEM ( '' )  );
#41718=DIRECTION ( 'NONE',  ( -0.000000000000000000, -0.000000000000000000, 1.000000000000000000 ) ) ;
#41720=CARTESIAN_POINT ( 'NONE',  ( 9.999999999999996447, -5.773502691896262640, -122.5000000040967905 ) ) ;
#41722=EDGE_LOOP ( 'NONE', ( #9275, #13758, #6264, #37649 ) ) ;
#41725=CARTESIAN_POINT ( 'NONE',  ( 0.000000000000000000, 0.000000000000000000, -200.0000000000000000 ) ) ;
#41726=CARTESIAN_POINT ( 'NONE',  ( 7.644554776091147741E-16, 12.48450537969573659, -181.1562500020484094 ) ) ;
#41727=VERTEX_POINT ( 'NONE', #6256 ) ;
#41728=CARTESIAN_POINT ( 'NONE',  ( 4.999999999999992006, -8.660254037844389075, -50.62500000409675494 ) ) ;
#41729=DIRECTION ( 'NONE',  ( -0.000000000000000000, -0.000000000000000000, 1.000000000000000000 ) ) ;
#41731=CYLINDRICAL_SURFACE ( 'NONE', #13128, 9.999999999999998224 ) ;
#41732=CARTESIAN_POINT ( 'NONE',  ( 10.81189881249999729, 0.000000000000000000, -172.5312500020484094 ) ) ;
#41733=CYLINDRICAL_SURFACE ( 'NONE', #5668, 9.999999999999998224 ) ;
#41734=LINE ( 'NONE', #2692, #35819 ) ;
#41738=ADVANCED_FACE ( 'NONE', ( #25272 ), #22020, .T. ) ;
#41743=CARTESIAN_POINT ( 'NONE',  ( -10.81189881249999907, -6.242252689847864744, -77.15625000204836681 ) ) ;
#41744=ORIENTED_EDGE ( 'NONE', *, *, #42385, .F. ) ;
#41746=CARTESIAN_POINT ( 'NONE',  ( -9.999999999999998224, 1.224646799147353059E-15, -53.74999999999996447 ) ) ;
#41747=EDGE_LOOP ( 'NONE', ( #5630, #2101, #16150, #41799 ) ) ;
#41748=ORIENTED_EDGE ( 'NONE', *, *, #30704, .F. ) ;
#41749=CARTESIAN_POINT ( 'NONE',  ( -10.81189881249999729, 6.242252689847871849, -29.21875000204835615 ) ) ;
#41750=CARTESIAN_POINT ( 'NONE',  ( -4.999999999999996447, 8.660254037844387298, -73.87500000409677625 ) ) ;
#41751=CARTESIAN_POINT ( 'NONE',  ( -10.81189881249999729, 1.324075727343319199E-15, -6.781250002048377468 ) ) ;
#41752=CARTESIAN_POINT ( 'NONE',  ( 7.644554776091147741E-16, 12.48450537969573659, -57.96875000204836681 ) ) ;
#41755=EDGE_CURVE ( 'NONE', #28241, #1967, #13759, .T. ) ;
#41756=CARTESIAN_POINT ( 'NONE',  ( 7.644554776091147741E-16, 12.48450537969573659, -191.4687500020484094 ) ) ;
#41757=CARTESIAN_POINT ( 'NONE',  ( -10.81189881249999729, 1.324075727343319199E-15, -179.0937500020484094 ) ) ;
#41761=CARTESIAN_POINT ( 'NONE',  ( -9.999999999999998224, 1.224646799147353059E-15, -18.12500000409675138 ) ) ;
#41762=CARTESIAN_POINT ( 'NONE',  ( 4.999999999999992006, -8.660254037844389075, -101.6250000040967905 ) ) ;
#41763=EDGE_CURVE ( 'NONE', #20093, #30868, #18183, .T. ) ;
#41765=CARTESIAN_POINT ( 'NONE',  ( -10.81189881249999729, 1.324075727343319199E-15, -105.5937500020483810 ) ) ;
#41766=CARTESIAN_POINT ( 'NONE',  ( 5.405949406249999534, 9.363379034771803333, -76.28125000204838102 ) ) ;
#41767=CARTESIAN_POINT ( 'NONE',  ( -10.81189881249999729, -6.242252689847864744, -91.96875000204838102 ) ) ;
#41768=EDGE_CURVE ( 'NONE', #28673, #18350, #38418, .T. ) ;
#41771=CARTESIAN_POINT ( 'NONE',  ( -2.121150477449813534E-15, -11.54700538379251284, -143.7500000040968189 ) ) ;
#41775=CARTESIAN_POINT ( 'NONE',  ( -9.999999999999998224, 1.224646799147353059E-15, -175.2500000000000284 ) ) ;
#41778=CARTESIAN_POINT ( 'NONE',  ( -2.121150477449813534E-15, -11.54700538379251284, -62.37499999999997868 ) ) ;
#41780=CARTESIAN_POINT ( 'NONE',  ( -10.00000000000000000, -5.773502691896251982, -78.00000000409677625 ) ) ;
#41781=EDGE_CURVE ( 'NONE', #32484, #14676, #40302, .T. ) ;
#41783=CARTESIAN_POINT ( 'NONE',  ( -5.000000000000003553, -8.660254037844383745, -11.87500000409674783 ) ) ;
#41785=CARTESIAN_POINT ( 'NONE',  ( -10.81189881249999729, 1.324075727343319199E-15, -65.28125000204838102 ) ) ;
#41787=DIRECTION ( 'NONE',  ( -0.000000000000000000, -0.000000000000000000, 1.000000000000000000 ) ) ;
#41790=CARTESIAN_POINT ( 'NONE',  ( 7.644554776091147741E-16, 12.48450537969573659, -191.6562500020484094 ) ) ;
#41792=CARTESIAN_POINT ( 'NONE',  ( 7.644554776091147741E-16, 12.48450537969573659, -6.968750002048348158 ) ) ;
#41793=CARTESIAN_POINT ( 'NONE',  ( -5.000000000000003553, -8.660254037844383745, -110.8750000040967763 ) ) ;
#41794=CARTESIAN_POINT ( 'NONE',  ( 9.999999999999872102, 5.773502691896329253, -159.7500000040967905 ) ) ;
#41795=EDGE_CURVE ( 'NONE', #848, #26104, #42132, .T. ) ;
#41796=CARTESIAN_POINT ( 'NONE',  ( 5.000000000000000000, 8.660254037844385522, -172.7500000000000284 ) ) ;
#41797=CARTESIAN_POINT ( 'NONE',  ( -4.999999999999996447, 8.660254037844387298, -1.499999999999973577 ) ) ;
#41798=CARTESIAN_POINT ( 'NONE',  ( 5.405949406249999534, 9.363379034771803333, -100.2812500020483952 ) ) ;
#41799=ORIENTED_EDGE ( 'NONE', *, *, #27150, .F. ) ;
#41801=ORIENTED_EDGE ( 'NONE', *, *, #5631, .T. ) ;
#41803=CARTESIAN_POINT ( 'NONE',  ( -10.81189881249999907, -6.242252689847864744, -32.15625000204835970 ) ) ;
#41804=CARTESIAN_POINT ( 'NONE',  ( 9.999999999999998224, 0.000000000000000000, -149.0000000000000000 ) ) ;
#41806=CARTESIAN_POINT ( 'NONE',  ( -10.81189881249999729, 6.242252689847871849, -77.21875000204838102 ) ) ;
#41807=CYLINDRICAL_SURFACE ( 'NONE', #11849, 9.999999999999998224 ) ;
#41809=EDGE_CURVE ( 'NONE', #5939, #8336, #39114, .T. ) ;
#41810=DIRECTION ( 'NONE',  ( -0.000000000000000000, -0.000000000000000000, 1.000000000000000000 ) ) ;
#41812=CARTESIAN_POINT ( 'NONE',  ( 4.999999999999992006, -8.660254037844389075, -11.62500000409674783 ) ) ;
#41813=CARTESIAN_POINT ( 'NONE',  ( -5.000000000000003553, -8.660254037844383745, -199.0000000000000000 ) ) ;
#41814=CARTESIAN_POINT ( 'NONE',  ( 5.405949406249992428, -9.363379034771808662, -130.5937500020483810 ) ) ;
#41815=CARTESIAN_POINT ( 'NONE',  ( 10.81189881249999551, -6.242252689847874514, -112.4687500020483810 ) ) ;
#41818=CARTESIAN_POINT ( 'NONE',  ( 4.999999999999992006, -8.660254037844389075, -173.6250000040968189 ) ) ;
#41819=CARTESIAN_POINT ( 'NONE',  ( 10.81189881249999729, 6.242252689847867408, -169.4062500020484094 ) ) ;
#41820=CARTESIAN_POINT ( 'NONE',  ( -9.999999999999998224, 1.224646799147353059E-15, -102.1250000040967905 ) ) ;
#41823=CARTESIAN_POINT ( 'NONE',  ( -5.405949406249996869, 9.363379034771805109, -47.34375000204838102 ) ) ;
#41825=CARTESIAN_POINT ( 'NONE',  ( -4.999999999999996447, 8.660254037844387298, -85.87500000409677625 ) ) ;
#41829=CARTESIAN_POINT ( 'NONE',  ( 7.070501591499377789E-16, 11.54700538379251284, -85.62499999999997158 ) ) ;
#41831=CARTESIAN_POINT ( 'NONE',  ( 9.999999999999996447, -5.773502691896262640, -97.00000000409677625 ) ) ;
#41832=CARTESIAN_POINT ( 'NONE',  ( 9.999999999999998224, 0.000000000000000000, -200.0000000000000000 ) ) ;
#41834=CARTESIAN_POINT ( 'NONE',  ( 5.405949406249992428, -9.363379034771808662, -100.7812500020483952 ) ) ;
#41838=CARTESIAN_POINT ( 'NONE',  ( 7.644554776091147741E-16, 12.48450537969573659, -158.6562500020484094 ) ) ;
#41840=ORIENTED_EDGE ( 'NONE', *, *, #12921, .T. ) ;
#41841=CARTESIAN_POINT ( 'NONE',  ( -2.121150477449813534E-15, -11.54700538379251284, -18.87499999999997513 ) ) ;
#41842=CARTESIAN_POINT ( 'NONE',  ( -10.81189881249999729, -6.242252689847864744, -24.65625000204838457 ) ) ;
#41843=CARTESIAN_POINT ( 'NONE',  ( -2.121150477449813534E-15, -11.54700538379251284, -150.8750000000000284 ) ) ;
#41846=CARTESIAN_POINT ( 'NONE',  ( 10.81189881249999907, 6.242252689847868297, -128.9062500020483810 ) ) ;
#41847=ORIENTED_EDGE ( 'NONE', *, *, #35860, .F. ) ;
#41848=CARTESIAN_POINT ( 'NONE',  ( -5.000020801129981152, 8.660290040615111096, 0.000000000000000000 ) ) ;
#41849=( BOUNDED_CURVE ( )  B_SPLINE_CURVE ( 2, ( #28659, #5772, #15667, #28868, #42002, #12430, #38783 ),
 .UNSPECIFIED., .F., .F. ) 
 B_SPLINE_CURVE_WITH_KNOTS ( ( 3, 2, 2, 3 ),
 ( 0.7537313432835822669, 0.7549751243781096521, 0.7562189054726369264, 0.7574626865671643117 ),
 .UNSPECIFIED. ) 
 CURVE ( )  GEOMETRIC_REPRESENTATION_ITEM ( )  RATIONAL_B_SPLINE_CURVE ( ( 0.9999999999999761302, 0.8660254037844625774, 1.000000000000000000, 0.8660254037844387076, 1.000000000000000000, 0.8660254037844267172, 1.000000000000011990 ) ) 
 REPRESENTATION_ITEM ( '' )  );
#41851=CARTESIAN_POINT ( 'NONE',  ( -10.81189881249999729, 1.324075727343319199E-15, -57.78125000204836681 ) ) ;
#41853=ADVANCED_FACE ( 'NONE', ( #17212 ), #13966, .T. ) ;
#41854=CARTESIAN_POINT ( 'NONE',  ( 10.81189881249999729, 0.000000000000000000, -101.8437500020483810 ) ) ;
#41855=VERTEX_POINT ( 'NONE', #33649 ) ;
#41859=CARTESIAN_POINT ( 'NONE',  ( -10.81189881249999907, -6.242252689847864744, -160.9687500020484094 ) ) ;
#41861=CARTESIAN_POINT ( 'NONE',  ( 5.405949406249992428, -9.363379034771808662, -4.593750002048368586 ) ) ;
#41862=CARTESIAN_POINT ( 'NONE',  ( 10.81189881249999551, -6.242252689847874514, -143.9687500020484094 ) ) ;
#41864=CYLINDRICAL_SURFACE ( 'NONE', #30454, 9.999999999999998224 ) ;
#41866=CARTESIAN_POINT ( 'NONE',  ( -9.999999999999998224, 1.224646799147353059E-15, -193.6250000040967905 ) ) ;
#41868=EDGE_CURVE ( 'NONE', #33849, #28241, #5229, .T. ) ;
#41869=CARTESIAN_POINT ( 'NONE',  ( -10.81189881249999729, 6.242252689847871849, -197.4062500020484094 ) ) ;
#41870=CARTESIAN_POINT ( 'NONE',  ( -4.999999999999996447, 8.660254037844387298, -11.99999999999995559 ) ) ;
#41873=CARTESIAN_POINT ( 'NONE',  ( -2.293366432827344421E-15, -12.48450537969573659, -66.21875000204836681 ) ) ;
#41874=CARTESIAN_POINT ( 'NONE',  ( 10.81189881249999551, -6.242252689847874514, -53.96875000204838102 ) ) ;
#41876=CARTESIAN_POINT ( 'NONE',  ( -5.405949406249996869, 9.363379034771805109, -25.03125000204836681 ) ) ;
#41881=CARTESIAN_POINT ( 'NONE',  ( 7.070501591499377789E-16, 11.54700538379251284, -114.1249999999999858 ) ) ;
#41886=CARTESIAN_POINT ( 'NONE',  ( 10.81189881249999729, 6.242252689847867408, -8.906250002048373915 ) ) ;
#41887=( BOUNDED_CURVE ( )  B_SPLINE_CURVE ( 2, ( #28510, #5831, #39259, #38629, #15939, #31961, #9692 ),
 .UNSPECIFIED., .F., .F. ) 
 B_SPLINE_CURVE_WITH_KNOTS ( ( 3, 2, 2, 3 ),
 ( 0.6641791044776121922, 0.6654228855721395774, 0.6666666666666668517, 0.6679104477611942370 ),
 .UNSPECIFIED. ) 
 CURVE ( )  GEOMETRIC_REPRESENTATION_ITEM ( )  RATIONAL_B_SPLINE_CURVE ( ( 0.9999999999999761302, 0.8660254037844625774, 1.000000000000000000, 0.8660254037844387076, 1.000000000000000000, 0.8660254037844148378, 1.000000000000023981 ) ) 
 REPRESENTATION_ITEM ( '' )  );
#41888=VERTEX_POINT ( 'NONE', #19610 ) ;
#41893=CARTESIAN_POINT ( 'NONE',  ( 9.999999999999996447, -5.773502691896262640, -39.62499999999995737 ) ) ;
#41894=CARTESIAN_POINT ( 'NONE',  ( 4.999999999999992006, -8.660254037844389075, -28.12500000409676204 ) ) ;
#41895=CARTESIAN_POINT ( 'NONE',  ( -5.405949406249996869, 9.363379034771805109, -53.53125000204836681 ) ) ;
#41899=CARTESIAN_POINT ( 'NONE',  ( 9.999999999998456346, 5.773502691897149042, -24.37499999999995381 ) ) ;
#41900=CARTESIAN_POINT ( 'NONE',  ( -10.81189881249999907, -6.242252689847864744, -149.1562500020483810 ) ) ;
#41901=CARTESIAN_POINT ( 'NONE',  ( 10.81189881249999907, 6.242252689847868297, -149.9062500020484094 ) ) ;
#41902=FACE_OUTER_BOUND ( 'NONE', #41747, .T. ) ;
#41903=CARTESIAN_POINT ( 'NONE',  ( -2.121150477449813534E-15, -11.54700538379251284, -57.87499999999998579 ) ) ;
#41904=EDGE_LOOP ( 'NONE', ( #40303, #21363, #30884, #31684 ) ) ;
#41905=EDGE_CURVE ( 'NONE', #8575, #8431, #14011, .T. ) ;
#41906=( BOUNDED_CURVE ( )  B_SPLINE_CURVE ( 2, ( #42490, #9911, #26746, #9701, #25903, #26112, #35833 ),
 .UNSPECIFIED., .F., .F. ) 
 B_SPLINE_CURVE_WITH_KNOTS ( ( 3, 2, 2, 3 ),
 ( 0.6044776119402985870, 0.6057213930348259723, 0.6069651741293533576, 0.6082089552238807428 ),
 .UNSPECIFIED. ) 
 CURVE ( )  GEOMETRIC_REPRESENTATION_ITEM ( )  RATIONAL_B_SPLINE_CURVE ( ( 0.9999999999999880096, 0.8660254037844506980, 1.000000000000000000, 0.8660254037844387076, 1.000000000000000000, 0.8660254037844267172, 1.000000000000011990 ) ) 
 REPRESENTATION_ITEM ( '' )  );
#41910=CARTESIAN_POINT ( 'NONE',  ( -9.999999999999998224, 1.224646799147353059E-15, -200.0000000000000000 ) ) ;
#41911=CARTESIAN_POINT ( 'NONE',  ( -2.293366432827344421E-15, -12.48450537969573659, -183.2187500020484094 ) ) ;
#41912=CARTESIAN_POINT ( 'NONE',  ( 10.81189881249999551, -6.242252689847874514, -32.96875000204834549 ) ) ;
#41914=CARTESIAN_POINT ( 'NONE',  ( 5.405949406249992428, -9.363379034771808662, -162.0937500020484094 ) ) ;
#41915=CARTESIAN_POINT ( 'NONE',  ( -5.405949406249996869, 9.363379034771805109, -152.3437500020483810 ) ) ;
#41919=CARTESIAN_POINT ( 'NONE',  ( -10.81189881249999729, 1.324075727343319199E-15, -15.59375000204835082 ) ) ;
#41922=CARTESIAN_POINT ( 'NONE',  ( -4.999999999999996447, 8.660254037844387298, -177.3750000040967905 ) ) ;
#41924=CARTESIAN_POINT ( 'NONE',  ( 10.81189881249999729, 0.000000000000000000, -83.84375000204836681 ) ) ;
#41926=CARTESIAN_POINT ( 'NONE',  ( 10.81189881249999907, 6.242252689847868297, -50.90625000204838102 ) ) ;
#41931=CARTESIAN_POINT ( 'NONE',  ( -4.999999999999996447, 8.660254037844387298, -141.0000000000000000 ) ) ;
#41932=CARTESIAN_POINT ( 'NONE',  ( 10.81189881249999551, -6.242252689847874514, -142.6562500020484094 ) ) ;
#41933=FACE_OUTER_BOUND ( 'NONE', #9527, .T. ) ;
#41935=CARTESIAN_POINT ( 'NONE',  ( -9.999999999999998224, 5.773502691896259087, -124.7500000040967763 ) ) ;
#41937=ORIENTED_EDGE ( 'NONE', *, *, #15907, .F. ) ;
#41940=CARTESIAN_POINT ( 'NONE',  ( -9.999999999999998224, 1.224646799147353059E-15, -22.62500000409675849 ) ) ;
#41941=CARTESIAN_POINT ( 'NONE',  ( -2.293366432827344421E-15, -12.48450537969573659, -169.9062500020483810 ) ) ;
#41942=CARTESIAN_POINT ( 'NONE',  ( 5.000000000000000000, 8.660254037844385522, -47.12500000409677625 ) ) ;
#41946=CARTESIAN_POINT ( 'NONE',  ( -9.999999999999479527, -5.773502691896549521, -148.5000000040967336 ) ) ;
#41947=CARTESIAN_POINT ( 'NONE',  ( 7.644554776091147741E-16, 12.48450537969573659, -170.6562500020484094 ) ) ;
#41949=CARTESIAN_POINT ( 'NONE',  ( -10.00000000000019185, -5.773502691896140071, -178.1249999999999432 ) ) ;
#41950=ORIENTED_EDGE ( 'NONE', *, *, #18971, .T. ) ;
#41951=CARTESIAN_POINT ( 'NONE',  ( 0.000000000000000000, 0.000000000000000000, -200.0000000000000000 ) ) ;
#41952=CARTESIAN_POINT ( 'NONE',  ( 10.00000000000102318, -5.773502691895667560, -71.12499999999995737 ) ) ;
#41953=CARTESIAN_POINT ( 'NONE',  ( 5.405949406249999534, 9.363379034771803333, -80.78125000204838102 ) ) ;
#41956=CARTESIAN_POINT ( 'NONE',  ( -9.999999999999479527, -5.773502691896549521, -140.6250000000000000 ) ) ;
#41958=ORIENTED_EDGE ( 'NONE', *, *, #19707, .F. ) ;
#41959=CARTESIAN_POINT ( 'NONE',  ( 7.644554776091147741E-16, 12.48450537969573659, -26.46875000204837747 ) ) ;
#41960=CARTESIAN_POINT ( 'NONE',  ( -2.121150477449813534E-15, -11.54700538379251284, -53.37499999999997868 ) ) ;
#41961=CARTESIAN_POINT ( 'NONE',  ( -5.405949406250003975, -9.363379034771801557, -2.031250002048373915 ) ) ;
#41962=CARTESIAN_POINT ( 'NONE',  ( -2.293366432827344421E-15, -12.48450537969573659, -52.71875000204837391 ) ) ;
#41964=CARTESIAN_POINT ( 'NONE',  ( -9.999999999999998224, 1.224646799147353059E-15, -4.249999999999976019 ) ) ;
#41966=CARTESIAN_POINT ( 'NONE',  ( 5.405949406249999534, 9.363379034771803333, -187.0937500020483810 ) ) ;
#41967=CARTESIAN_POINT ( 'NONE',  ( -5.405949406249996869, 9.363379034771805109, -180.8437500020483810 ) ) ;
#41968=( BOUNDED_CURVE ( )  B_SPLINE_CURVE ( 2, ( #20749, #1126, #11244, #14249, #11030, #4781, #26810 ),
 .UNSPECIFIED., .F., .F. ) 
 B_SPLINE_CURVE_WITH_KNOTS ( ( 3, 2, 2, 3 ),
 ( 0.01119402985074628015, 0.01243781094527364461, 0.01368159203980100908, 0.01492537313432837180 ),
 .UNSPECIFIED. ) 
 CURVE ( )  GEOMETRIC_REPRESENTATION_ITEM ( )  RATIONAL_B_SPLINE_CURVE ( ( 0.9999999999999986677, 0.8660254037844400399, 1.000000000000000000, 0.8660254037844387076, 1.000000000000000000, 0.8660254037844372643, 1.000000000000001554 ) ) 
 REPRESENTATION_ITEM ( '' )  );
#41971=DIRECTION ( 'NONE',  ( -0.000000000000000000, -0.000000000000000000, 1.000000000000000000 ) ) ;
#41972=DIRECTION ( 'NONE',  ( -0.000000000000000000, -0.000000000000000000, 1.000000000000000000 ) ) ;
#41974=VECTOR ( 'NONE', #19622, 1000.000000000000000 ) ;
#41975=CARTESIAN_POINT ( 'NONE',  ( 7.644554776091147741E-16, 12.48450537969573659, -107.4687500020483668 ) ) ;
#41977=CARTESIAN_POINT ( 'NONE',  ( 5.405949406249999534, 9.363379034771803333, -77.78125000204838102 ) ) ;
#41978=EDGE_CURVE ( 'NONE', #28714, #2188, #10112, .T. ) ;
#41979=CARTESIAN_POINT ( 'NONE',  ( -2.293366432827344421E-15, -12.48450537969573659, -88.71875000204838102 ) ) ;
#41982=CARTESIAN_POINT ( 'NONE',  ( -5.000000000000003553, -8.660254037844383745, -149.8750000040967905 ) ) ;
#41984=ORIENTED_EDGE ( 'NONE', *, *, #2158, .F. ) ;
#41985=AXIS2_PLACEMENT_3D ( 'NONE', #42035, #29313, #19166 ) ;
#41988=CARTESIAN_POINT ( 'NONE',  ( 5.405949406249999534, 9.363379034771803333, -196.2812500020484094 ) ) ;
#41989=DIRECTION ( 'NONE',  ( -0.000000000000000000, -0.000000000000000000, 1.000000000000000000 ) ) ;
#41991=ORIENTED_EDGE ( 'NONE', *, *, #13519, .F. ) ;
#41992=CARTESIAN_POINT ( 'NONE',  ( 5.000000000000000000, 8.660254037844385522, -66.24999999999997158 ) ) ;
#41994=CARTESIAN_POINT ( 'NONE',  ( -9.999999999999998224, 1.224646799147353059E-15, -70.62500000409677625 ) ) ;
#41996=CARTESIAN_POINT ( 'NONE',  ( 9.999999999999998224, 0.000000000000000000, -200.0000000000000000 ) ) ;
#41998=CARTESIAN_POINT ( 'NONE',  ( 7.644554776091147741E-16, 12.48450537969573659, -64.15625000204838102 ) ) ;
#42000=CARTESIAN_POINT ( 'NONE',  ( 0.000000000000000000, 0.000000000000000000, -200.0000000000000000 ) ) ;
#42002=CARTESIAN_POINT ( 'NONE',  ( -4.999999999999996447, 8.660254037844387298, -46.87500000409677625 ) ) ;
#42003=CARTESIAN_POINT ( 'NONE',  ( 10.81189881249999907, 6.242252689847868297, -194.9062500020484379 ) ) ;
#42005=CARTESIAN_POINT ( 'NONE',  ( -10.81189881249999729, 1.324075727343319199E-15, -5.093750002048369474 ) ) ;
#42006=DIRECTION ( 'NONE',  ( 1.000000000000000000, 0.000000000000000000, 0.000000000000000000 ) ) ;
#42007=CARTESIAN_POINT ( 'NONE',  ( 9.999999999999998224, 0.000000000000000000, -36.87500000409676915 ) ) ;
#42008=CARTESIAN_POINT ( 'NONE',  ( -9.999999999999998224, 1.224646799147353059E-15, -39.12500000409676915 ) ) ;
#42009=CARTESIAN_POINT ( 'NONE',  ( -4.999999999999996447, 8.660254037844387298, -175.5000000000000284 ) ) ;
#42010=DIRECTION ( 'NONE',  ( -0.000000000000000000, -0.000000000000000000, 1.000000000000000000 ) ) ;
#42011=CARTESIAN_POINT ( 'NONE',  ( -5.405949406250003975, -9.363379034771801557, -101.0312500020483952 ) ) ;
#42012=ORIENTED_EDGE ( 'NONE', *, *, #19620, .T. ) ;
#42013=DIRECTION ( 'NONE',  ( -0.000000000000000000, -0.000000000000000000, 1.000000000000000000 ) ) ;
#42014=ADVANCED_FACE ( 'NONE', ( #36450 ), #9903, .T. ) ;
#42015=ORIENTED_EDGE ( 'NONE', *, *, #25929, .T. ) ;
#42016=ORIENTED_EDGE ( 'NONE', *, *, #22928, .F. ) ;
#42017=( BOUNDED_CURVE ( )  B_SPLINE_CURVE ( 2, ( #27711, #31175, #24052, #5049, #37193, #21438, #40417 ),
 .UNSPECIFIED., .F., .F. ) 
 B_SPLINE_CURVE_WITH_KNOTS ( ( 3, 2, 2, 3 ),
 ( 0.2201492537313433639, 0.2213930348258707215, 0.2226368159203980790, 0.2238805970149254365 ),
 .UNSPECIFIED. ) 
 CURVE ( )  GEOMETRIC_REPRESENTATION_ITEM ( )  RATIONAL_B_SPLINE_CURVE ( ( 0.9999999999999910072, 0.8660254037844477004, 1.000000000000000000, 0.8660254037844387076, 1.000000000000000000, 0.8660254037844327124, 1.000000000000005995 ) ) 
 REPRESENTATION_ITEM ( '' )  );
#42018=CARTESIAN_POINT ( 'NONE',  ( -5.405949406249996869, 9.363379034771805109, -26.53125000204836681 ) ) ;
#42020=CARTESIAN_POINT ( 'NONE',  ( -5.405949406249996869, 9.363379034771805109, -80.34375000204838102 ) ) ;
#42022=FACE_OUTER_BOUND ( 'NONE', #7799, .T. ) ;
#42024=LINE ( 'NONE', #25647, #22577 ) ;
#42026=CARTESIAN_POINT ( 'NONE',  ( -4.999999999999996447, 8.660254037844387298, -7.875000004096744277 ) ) ;
#42028=CARTESIAN_POINT ( 'NONE',  ( -2.293366432827344421E-15, -12.48450537969573659, -130.7187500020483810 ) ) ;
#42029=EDGE_CURVE ( 'NONE', #35877, #900, #40483, .T. ) ;
#42030=CARTESIAN_POINT ( 'NONE',  ( 10.81189881249999729, 0.000000000000000000, -118.3437500020483810 ) ) ;
#42033=CARTESIAN_POINT ( 'NONE',  ( -9.999999999999998224, 1.224646799147353059E-15, -169.6250000040967905 ) ) ;
#42034=ADVANCED_FACE ( 'NONE', ( #27808 ), #30623, .T. ) ;
#42035=CARTESIAN_POINT ( 'NONE',  ( 0.000000000000000000, 0.000000000000000000, -200.0000000000000000 ) ) ;
#42038=CARTESIAN_POINT ( 'NONE',  ( -5.405949406249996869, 9.363379034771805109, -45.84375000204838102 ) ) ;
#42039=AXIS2_PLACEMENT_3D ( 'NONE', #3431, #33434, #30825 ) ;
#42040=EDGE_CURVE ( 'NONE', #27003, #14981, #8002, .T. ) ;
#42042=CARTESIAN_POINT ( 'NONE',  ( -10.81189881249999729, 6.242252689847871849, -5.406250002048357928 ) ) ;
#42044=CARTESIAN_POINT ( 'NONE',  ( 4.999999999999992006, -8.660254037844389075, -126.7499999999999716 ) ) ;
#42046=CARTESIAN_POINT ( 'NONE',  ( 9.999999999999998224, 0.000000000000000000, -88.99999999999998579 ) ) ;
#42048=CARTESIAN_POINT ( 'NONE',  ( -5.000000000000003553, -8.660254037844383745, -97.37500000409677625 ) ) ;
#42051=CARTESIAN_POINT ( 'NONE',  ( -2.293366432827344421E-15, -12.48450537969573659, -94.90625000204838102 ) ) ;
#42052=ORIENTED_EDGE ( 'NONE', *, *, #2395, .T. ) ;
#42056=ORIENTED_EDGE ( 'NONE', *, *, #29392, .T. ) ;
#42057=CARTESIAN_POINT ( 'NONE',  ( 5.000000000000000000, 8.660254037844385522, -21.24999999999996447 ) ) ;
#42058=CARTESIAN_POINT ( 'NONE',  ( -5.405949406249996869, 9.363379034771805109, -23.53125000204836681 ) ) ;
#42059=CARTESIAN_POINT ( 'NONE',  ( -4.999999999999996447, 8.660254037844387298, -150.0000000000000000 ) ) ;
#42062=EDGE_CURVE ( 'NONE', #17414, #42281, #570, .T. ) ;
#42063=CARTESIAN_POINT ( 'NONE',  ( 9.999999999999996447, -5.773502691896262640, -197.1250000000000284 ) ) ;
#42064=CARTESIAN_POINT ( 'NONE',  ( -5.405949406249996869, 9.363379034771805109, -124.0312500020483952 ) ) ;
#42068=CARTESIAN_POINT ( 'NONE',  ( -5.405949406249996869, 9.363379034771805109, -50.53125000204835970 ) ) ;
#42070=AXIS2_PLACEMENT_3D ( 'NONE', #3385, #17160, #9852 ) ;
#42071=CARTESIAN_POINT ( 'NONE',  ( -10.81189881249999729, 1.324075727343319199E-15, -107.0937500020483810 ) ) ;
#42072=VERTEX_POINT ( 'NONE', #14619 ) ;
#42073=EDGE_LOOP ( 'NONE', ( #22599, #42571, #32123, #7259 ) ) ;
#42075=CARTESIAN_POINT ( 'NONE',  ( -9.999999999999998224, 1.224646799147353059E-15, -112.6250000040967763 ) ) ;
#42076=CARTESIAN_POINT ( 'NONE',  ( 7.644554776091147741E-16, 12.48450537969573659, -150.9687500020483810 ) ) ;
#42078=CARTESIAN_POINT ( 'NONE',  ( -10.81189881249999907, -6.242252689847864744, -3.468750002048364145 ) ) ;
#42080=CARTESIAN_POINT ( 'NONE',  ( -10.81189881249999729, 1.324075727343319199E-15, -138.5937500020483810 ) ) ;
#42082=CARTESIAN_POINT ( 'NONE',  ( -9.999999999999479527, -5.773502691896549521, -148.1249999999999716 ) ) ;
#42084=CARTESIAN_POINT ( 'NONE',  ( -9.999999999999998224, 1.224646799147353059E-15, -190.6250000040967905 ) ) ;
#42086=CARTESIAN_POINT ( 'NONE',  ( -2.293366432827344421E-15, -12.48450537969573659, -195.4062500020484094 ) ) ;
#42087=CARTESIAN_POINT ( 'NONE',  ( -23.09401076758503280, 0.000000000000000000, 49.99999999999998579 ) ) ;
#42090=CARTESIAN_POINT ( 'NONE',  ( 5.405949406249992428, -9.363379034771808662, -70.59375000204836681 ) ) ;
#42091=CARTESIAN_POINT ( 'NONE',  ( 10.81189881249999729, 0.000000000000000000, -50.84375000204835260 ) ) ;
#42093=CARTESIAN_POINT ( 'NONE',  ( 7.644554776091147741E-16, 12.48450537969573659, -25.15625000204838457 ) ) ;
#42096=CARTESIAN_POINT ( 'NONE',  ( -4.999999999999996447, 8.660254037844387298, -113.9999999999999858 ) ) ;
#42097=CARTESIAN_POINT ( 'NONE',  ( 9.999999999999998224, 0.000000000000000000, -42.49999999999998579 ) ) ;
#42100=CARTESIAN_POINT ( 'NONE',  ( 5.405949406249992428, -9.363379034771808662, -118.7812500020483952 ) ) ;
#42101=VERTEX_POINT ( 'NONE', #20674 ) ;
#42102=CARTESIAN_POINT ( 'NONE',  ( -2.121150477449813534E-15, -11.54700538379251284, -176.3750000000000000 ) ) ;
#42104=CARTESIAN_POINT ( 'NONE',  ( -9.999999999999227285, -5.773502691896698735, -128.6249999999999716 ) ) ;
#42106=CARTESIAN_POINT ( 'NONE',  ( -9.999999999999998224, 1.224646799147353059E-15, -40.24999999999997868 ) ) ;
#42108=EDGE_CURVE ( 'NONE', #10196, #23394, #34721, .T. ) ;
#42109=CARTESIAN_POINT ( 'NONE',  ( 9.999999999999998224, 0.000000000000000000, -27.87500000409676204 ) ) ;
#42110=CARTESIAN_POINT ( 'NONE',  ( -2.293366432827344421E-15, -12.48450537969573659, -49.90625000204837391 ) ) ;
#42111=CARTESIAN_POINT ( 'NONE',  ( -5.000000000000003553, -8.660254037844383745, -142.0000000000000000 ) ) ;
#42114=CARTESIAN_POINT ( 'NONE',  ( 10.81189881249999729, 0.000000000000000000, -138.0312500020484094 ) ) ;
#42115=CARTESIAN_POINT ( 'NONE',  ( 10.81189881249999551, -6.242252689847874514, -148.6562500020484094 ) ) ;
#42118=VERTEX_POINT ( 'NONE', #14176 ) ;
#42119=ORIENTED_EDGE ( 'NONE', *, *, #19360, .F. ) ;
#42121=AXIS2_PLACEMENT_3D ( 'NONE', #14925, #34173, #30926 ) ;
#42122=LINE ( 'NONE', #41910, #14558 ) ;
#42123=CARTESIAN_POINT ( 'NONE',  ( 5.405949406249999534, 9.363379034771803333, -181.0937500020483810 ) ) ;
#42125=CARTESIAN_POINT ( 'NONE',  ( -10.81189881249999907, -6.242252689847864744, -27.46875000204838457 ) ) ;
#42126=CARTESIAN_POINT ( 'NONE',  ( 9.999999999999998224, 0.000000000000000000, -21.49999999999996447 ) ) ;
#42127=CARTESIAN_POINT ( 'NONE',  ( 10.81189881249999729, 0.000000000000000000, -164.8437500020484094 ) ) ;
#42128=CARTESIAN_POINT ( 'NONE',  ( 5.405949406249992428, -9.363379034771808662, -148.5937500020483810 ) ) ;
#42132=( BOUNDED_CURVE ( )  B_SPLINE_CURVE ( 2, ( #23079, #33441, #16785, #7310, #23716, #26735, #36237 ),
 .UNSPECIFIED., .F., .F. ) 
 B_SPLINE_CURVE_WITH_KNOTS ( ( 3, 2, 2, 3 ),
 ( 0.8731343283582092551, 0.8743781094527366404, 0.8756218905472639147, 0.8768656716417913000 ),
 .UNSPECIFIED. ) 
 CURVE ( )  GEOMETRIC_REPRESENTATION_ITEM ( )  RATIONAL_B_SPLINE_CURVE ( ( 0.9999999999999641398, 0.8660254037844745678, 1.000000000000000000, 0.8660254037844387076, 1.000000000000000000, 0.8660254037844148378, 1.000000000000023981 ) ) 
 REPRESENTATION_ITEM ( '' )  );
#42133=CARTESIAN_POINT ( 'NONE',  ( 10.81189881249999729, 0.000000000000000000, -20.84375000204835615 ) ) ;
#42136=CARTESIAN_POINT ( 'NONE',  ( 9.999999999998969713, 5.773502691896851502, -70.87499999999997158 ) ) ;
#42139=CARTESIAN_POINT ( 'NONE',  ( -2.293366432827344421E-15, -12.48450537969573659, -79.71875000204838102 ) ) ;
#42140=CARTESIAN_POINT ( 'NONE',  ( -10.81189881249999729, 1.324075727343319199E-15, -48.78125000204838813 ) ) ;
#42142=CARTESIAN_POINT ( 'NONE',  ( -10.00000000000102496, 5.773502691895664007, -56.87499999999995026 ) ) ;
#42144=CARTESIAN_POINT ( 'NONE',  ( -10.00000000000000000, -5.773502691896251982, -140.6249999999999716 ) ) ;
#42145=CARTESIAN_POINT ( 'NONE',  ( 5.405949406249999534, 9.363379034771803333, -145.2812500020483810 ) ) ;
#42146=DIRECTION ( 'NONE',  ( -0.000000000000000000, -0.000000000000000000, 1.000000000000000000 ) ) ;
#42147=CARTESIAN_POINT ( 'NONE',  ( -4.999999999999996447, 8.660254037844387298, -118.8750000040967905 ) ) ;
#42152=CARTESIAN_POINT ( 'NONE',  ( -9.999999999999998224, 1.224646799147353059E-15, -49.24999999999998579 ) ) ;
#42153=CARTESIAN_POINT ( 'NONE',  ( 10.81189881249999729, 0.000000000000000000, -171.0312500020484094 ) ) ;
#42154=CARTESIAN_POINT ( 'NONE',  ( 4.999999999999992006, -8.660254037844389075, -49.12500000409678336 ) ) ;
#42155=CARTESIAN_POINT ( 'NONE',  ( 9.999999999999998224, 0.000000000000000000, -30.49999999999997158 ) ) ;
#42157=CARTESIAN_POINT ( 'NONE',  ( -9.999999999999998224, 1.224646799147353059E-15, -148.6250000040967905 ) ) ;
#42158=CARTESIAN_POINT ( 'NONE',  ( 10.81189881249999729, 0.000000000000000000, -166.5312500020484094 ) ) ;
#42160=LINE ( 'NONE', #12591, #35298 ) ;
#42161=CARTESIAN_POINT ( 'NONE',  ( 0.000000000000000000, 0.000000000000000000, -200.0000000000000000 ) ) ;
#42162=ORIENTED_EDGE ( 'NONE', *, *, #28084, .F. ) ;
#42164=CARTESIAN_POINT ( 'NONE',  ( -9.999999999999479527, -5.773502691896549521, -71.62499999999998579 ) ) ;
#42166=CARTESIAN_POINT ( 'NONE',  ( 7.644554776091147741E-16, 12.48450537969573659, -79.15625000204838102 ) ) ;
#42167=VERTEX_POINT ( 'NONE', #5145 ) ;
#42169=LINE ( 'NONE', #28404, #692 ) ;
#42170=ORIENTED_EDGE ( 'NONE', *, *, #37881, .F. ) ;
#42171=ORIENTED_EDGE ( 'NONE', *, *, #42504, .T. ) ;
#42172=CARTESIAN_POINT ( 'NONE',  ( -2.293366432827344421E-15, -12.48450537969573659, -31.71875000204835260 ) ) ;
#42173=CYLINDRICAL_SURFACE ( 'NONE', #429, 9.999999999999998224 ) ;
#42174=CARTESIAN_POINT ( 'NONE',  ( 10.81189881249999907, 6.242252689847868297, -5.906250002048359704 ) ) ;
#42175=CARTESIAN_POINT ( 'NONE',  ( 10.81189881249999907, 6.242252689847868297, -52.21875000204837391 ) ) ;
#42176=ORIENTED_EDGE ( 'NONE', *, *, #32327, .T. ) ;
#42177=CARTESIAN_POINT ( 'NONE',  ( -9.999999999999998224, 1.224646799147353059E-15, -71.74999999999998579 ) ) ;
#42179=CARTESIAN_POINT ( 'NONE',  ( -5.405949406250003975, -9.363379034771801557, -186.3437500020483810 ) ) ;
#42180=CARTESIAN_POINT ( 'NONE',  ( -2.293366432827344421E-15, -12.48450537969573659, -174.2187500020484094 ) ) ;
#42185=CARTESIAN_POINT ( 'NONE',  ( -9.999999999999998224, 1.224646799147353059E-15, -200.0000000000000000 ) ) ;
#42187=CARTESIAN_POINT ( 'NONE',  ( -10.81189881249999729, 6.242252689847871849, -107.2187500020483810 ) ) ;
#42188=LINE ( 'NONE', #9813, #33450 ) ;
#42189=CARTESIAN_POINT ( 'NONE',  ( -5.405949406249996869, 9.363379034771805109, -71.53125000204838102 ) ) ;
#42190=CARTESIAN_POINT ( 'NONE',  ( -9.999999999999227285, -5.773502691896698735, -132.0000000040967620 ) ) ;
#42191=CARTESIAN_POINT ( 'NONE',  ( 10.81189881249999729, 0.000000000000000000, -83.84375000204836681 ) ) ;
#42193=CARTESIAN_POINT ( 'NONE',  ( 10.00000000000000000, 5.773502691896255534, -144.7500000040967905 ) ) ;
#42195=ORIENTED_EDGE ( 'NONE', *, *, #7580, .F. ) ;
#42198=AXIS2_PLACEMENT_3D ( 'NONE', #25985, #8945, #12583 ) ;
#42199=CARTESIAN_POINT ( 'NONE',  ( 10.81189881249999729, 0.000000000000000000, -198.0312500020484094 ) ) ;
#42203=CARTESIAN_POINT ( 'NONE',  ( -5.000000000000003553, -8.660254037844383745, -66.99999999999997158 ) ) ;
#42205=CARTESIAN_POINT ( 'NONE',  ( 9.999999999999998224, 0.000000000000000000, -74.37500000409677625 ) ) ;
#42206=FACE_OUTER_BOUND ( 'NONE', #28461, .T. ) ;
#42207=CARTESIAN_POINT ( 'NONE',  ( -9.999999999999998224, 1.224646799147353059E-15, -12.12500000409674783 ) ) ;
#42209=CARTESIAN_POINT ( 'NONE',  ( -10.81189881249999729, 1.324075727343319199E-15, -63.78125000204837391 ) ) ;
#42213=CARTESIAN_POINT ( 'NONE',  ( -10.81189881249999729, 1.324075727343319199E-15, -194.2812500020484094 ) ) ;
#42215=CARTESIAN_POINT ( 'NONE',  ( -10.81189881249999729, -6.242252689847864744, -3.468750002048364145 ) ) ;
#42216=CARTESIAN_POINT ( 'NONE',  ( -9.999999999999227285, -5.773502691896698735, -111.0000000040967620 ) ) ;
#42218=CARTESIAN_POINT ( 'NONE',  ( -10.00000000000000000, -5.773502691896252870, -173.6249999999999716 ) ) ;
#42219=CARTESIAN_POINT ( 'NONE',  ( 10.00000000000000000, 5.773502691896255534, -172.8750000000000000 ) ) ;
#42220=CARTESIAN_POINT ( 'NONE',  ( -9.999999999999998224, 1.224646799147353059E-15, -169.6250000040967905 ) ) ;
#42221=CARTESIAN_POINT ( 'NONE',  ( 10.81189881249999551, -6.242252689847874514, -99.15625000204838102 ) ) ;
#42224=EDGE_CURVE ( 'NONE', #4287, #13498, #7740, .T. ) ;
#42225=ORIENTED_EDGE ( 'NONE', *, *, #1000, .F. ) ;
#42227=EDGE_CURVE ( 'NONE', #39036, #20043, #21104, .T. ) ;
#42229=CARTESIAN_POINT ( 'NONE',  ( 10.81189881249999729, 0.000000000000000000, -35.84375000204836681 ) ) ;
#42230=CARTESIAN_POINT ( 'NONE',  ( 5.405949406249999534, 9.363379034771803333, -29.78125000204837036 ) ) ;
#42232=CARTESIAN_POINT ( 'NONE',  ( 10.81189881249999907, 6.242252689847868297, -76.21875000204836681 ) ) ;
#42235=CARTESIAN_POINT ( 'NONE',  ( -9.999999999999998224, 1.224646799147353059E-15, -69.12500000409677625 ) ) ;
#42238=CARTESIAN_POINT ( 'NONE',  ( -9.999999999999998224, 1.224646799147353059E-15, -13.62500000409674961 ) ) ;
#42239=CYLINDRICAL_SURFACE ( 'NONE', #38444, 9.999999999999998224 ) ;
#42240=CARTESIAN_POINT ( 'NONE',  ( -10.81189881249999729, 6.242252689847871849, -132.7187500020483810 ) ) ;
#42241=CARTESIAN_POINT ( 'NONE',  ( -5.405949406249996869, 9.363379034771805109, -98.53125000204839523 ) ) ;
#42242=CARTESIAN_POINT ( 'NONE',  ( 10.81189881249999729, 0.000000000000000000, -104.8437500020483810 ) ) ;
#42245=CARTESIAN_POINT ( 'NONE',  ( -10.00000000000000000, -5.773502691896251982, -168.0000000040967905 ) ) ;
#42246=CARTESIAN_POINT ( 'NONE',  ( -2.121150477449813534E-15, -11.54700538379251284, -66.87500000000000000 ) ) ;
#42250=CARTESIAN_POINT ( 'NONE',  ( -10.81189881249999729, 1.324075727343319199E-15, -3.781250002048375247 ) ) ;
#42252=CARTESIAN_POINT ( 'NONE',  ( 9.999999999999998224, 0.000000000000000000, -200.0000000000000000 ) ) ;
#42254=CARTESIAN_POINT ( 'NONE',  ( 5.000000000000000000, 8.660254037844385522, -90.24999999999998579 ) ) ;
#42256=CARTESIAN_POINT ( 'NONE',  ( 10.00000000000000000, 5.773502691896255534, -99.75000000409679046 ) ) ;
#42257=DIRECTION ( 'NONE',  ( 1.000000000000000000, 0.000000000000000000, 0.000000000000000000 ) ) ;
#42259=CARTESIAN_POINT ( 'NONE',  ( 5.405949406249992428, -9.363379034771808662, -90.28125000204838102 ) ) ;
#42260=ORIENTED_EDGE ( 'NONE', *, *, #4814, .T. ) ;
#42262=CARTESIAN_POINT ( 'NONE',  ( 5.000000000000000000, 8.660254037844385522, -4.749999999999976907 ) ) ;
#42264=ORIENTED_EDGE ( 'NONE', *, *, #42543, .F. ) ;
#42265=CARTESIAN_POINT ( 'NONE',  ( 4.999999999999992006, -8.660254037844389075, -20.24999999999996092 ) ) ;
#42266=CARTESIAN_POINT ( 'NONE',  ( -4.999999999999996447, 8.660254037844387298, -157.5000000000000000 ) ) ;
#42268=( BOUNDED_CURVE ( )  B_SPLINE_CURVE ( 2, ( #35152, #28890, #9025, #26068, #29098, #25855, #42235 ),
 .UNSPECIFIED., .F., .F. ) 
 B_SPLINE_CURVE_WITH_KNOTS ( ( 3, 2, 2, 3 ),
 ( 0.6417910447761195902, 0.6430348258706469755, 0.6442786069651742498, 0.6455223880597016350 ),
 .UNSPECIFIED. ) 
 CURVE ( )  GEOMETRIC_REPRESENTATION_ITEM ( )  RATIONAL_B_SPLINE_CURVE ( ( 0.9999999999999761302, 0.8660254037844625774, 1.000000000000000000, 0.8660254037844387076, 1.000000000000000000, 0.8660254037844267172, 1.000000000000011990 ) ) 
 REPRESENTATION_ITEM ( '' )  );
#42269=CARTESIAN_POINT ( 'NONE',  ( 7.070501591499377789E-16, 11.54700538379251284, -196.6250000000000284 ) ) ;
#42270=CARTESIAN_POINT ( 'NONE',  ( -10.81189881249999729, 6.242252689847871849, -122.4062500020483952 ) ) ;
#42271=ORIENTED_EDGE ( 'NONE', *, *, #21736, .T. ) ;
#42275=ORIENTED_EDGE ( 'NONE', *, *, #10365, .F. ) ;
#42277=CARTESIAN_POINT ( 'NONE',  ( 10.81189881249999907, 6.242252689847868297, -53.90625000204838102 ) ) ;
#42279=CARTESIAN_POINT ( 'NONE',  ( -10.81189881249999729, 1.324075727343319199E-15, -104.0937500020483810 ) ) ;
#42281=VERTEX_POINT ( 'NONE', #7954 ) ;
#42282=DIRECTION ( 'NONE',  ( -0.000000000000000000, -0.000000000000000000, 1.000000000000000000 ) ) ;
#42284=CARTESIAN_POINT ( 'NONE',  ( 9.999999999999998224, 0.000000000000000000, -33.49999999999997158 ) ) ;
#42286=CARTESIAN_POINT ( 'NONE',  ( 9.999999999999998224, 0.000000000000000000, -176.0000000000000000 ) ) ;
#42289=CARTESIAN_POINT ( 'NONE',  ( 5.405949406249992428, -9.363379034771808662, -138.0937500020483810 ) ) ;
#42291=FACE_BOUND ( 'NONE', #20203, .T. ) ;
#42293=CARTESIAN_POINT ( 'NONE',  ( 5.000000000000000000, 8.660254037844385522, -192.6250000040967905 ) ) ;
#42295=CARTESIAN_POINT ( 'NONE',  ( -10.81189881249999729, -6.242252689847864744, -189.6562500020484379 ) ) ;
#42296=FACE_OUTER_BOUND ( 'NONE', #23725, .T. ) ;
#42300=CARTESIAN_POINT ( 'NONE',  ( 7.644554776091147741E-16, 12.48450537969573659, -66.96875000204838102 ) ) ;
#42301=CARTESIAN_POINT ( 'NONE',  ( 7.644554776091147741E-16, 12.48450537969573659, -47.46875000204836681 ) ) ;
#42303=CARTESIAN_POINT ( 'NONE',  ( 5.405949406249992428, -9.363379034771808662, -28.78125000204837036 ) ) ;
#42307=CARTESIAN_POINT ( 'NONE',  ( 9.999999999999998224, 0.000000000000000000, -117.5000000000000000 ) ) ;
#42308=CARTESIAN_POINT ( 'NONE',  ( 7.070501591499376803E-16, 11.54700538379251284, -163.6250000000000284 ) ) ;
#42311=CARTESIAN_POINT ( 'NONE',  ( -5.405949406250003975, -9.363379034771801557, -119.0312500020483952 ) ) ;
#42313=CARTESIAN_POINT ( 'NONE',  ( 9.999999999999998224, 0.000000000000000000, -7.999999999999952038 ) ) ;
#42315=CARTESIAN_POINT ( 'NONE',  ( 10.00000000000102318, -5.773502691895667560, -86.50000000409674783 ) ) ;
#42317=CARTESIAN_POINT ( 'NONE',  ( -2.121150477449813534E-15, -11.54700538379251284, -42.87499999999997868 ) ) ;
#42318=CARTESIAN_POINT ( 'NONE',  ( -4.999999999999996447, 8.660254037844387298, -18.37500000409675494 ) ) ;
#42319=CARTESIAN_POINT ( 'NONE',  ( -2.293366432827344421E-15, -12.48450537969573659, -43.90625000204838102 ) ) ;
#42321=CARTESIAN_POINT ( 'NONE',  ( 9.999999999998456346, 5.773502691897149042, -16.87499999999993250 ) ) ;
#42324=DIRECTION ( 'NONE',  ( -0.000000000000000000, -0.000000000000000000, 1.000000000000000000 ) ) ;
#42325=CARTESIAN_POINT ( 'NONE',  ( 7.644554776091147741E-16, 12.48450537969573659, -140.6562500020484094 ) ) ;
#42326=CARTESIAN_POINT ( 'NONE',  ( 5.405949406249999534, 9.363379034771803333, -146.7812500020483810 ) ) ;
#42327=FACE_OUTER_BOUND ( 'NONE', #37892, .T. ) ;
#42331=CARTESIAN_POINT ( 'NONE',  ( 9.999999999999998224, 0.000000000000000000, -108.8750000040967763 ) ) ;
#42332=CARTESIAN_POINT ( 'NONE',  ( -10.81189881249999729, 6.242252689847871849, -176.2187500020483810 ) ) ;
#42333=CARTESIAN_POINT ( 'NONE',  ( -10.81189881249999729, 6.242252689847871849, -23.21875000204836326 ) ) ;
#42334=EDGE_CURVE ( 'NONE', #28132, #1053, #25844, .T. ) ;
#42335=CARTESIAN_POINT ( 'NONE',  ( 10.00000000000025402, -5.773502691896113426, -128.5000000040967905 ) ) ;
#42336=CARTESIAN_POINT ( 'NONE',  ( 10.81189881249999551, -6.242252689847874514, -167.9687500020483810 ) ) ;
#42337=CARTESIAN_POINT ( 'NONE',  ( 10.81189881249999907, 6.242252689847868297, -146.7187500020484094 ) ) ;
#42341=CARTESIAN_POINT ( 'NONE',  ( -5.405949406249996869, 9.363379034771805109, -18.84375000204835260 ) ) ;
#42344=CARTESIAN_POINT ( 'NONE',  ( -10.00000000000154188, 5.773502691895366468, -25.37499999999993605 ) ) ;
#42346=CARTESIAN_POINT ( 'NONE',  ( -9.999999999999998224, 1.224646799147353059E-15, -55.62500000409676204 ) ) ;
#42347=CARTESIAN_POINT ( 'NONE',  ( -5.405949406250003975, -9.363379034771801557, -73.84375000204838102 ) ) ;
#42348=CARTESIAN_POINT ( 'NONE',  ( -2.293366432827344421E-15, -12.48450537969573659, -48.40625000204837391 ) ) ;
#42350=LINE ( 'NONE', #16434, #26793 ) ;
#42352=CARTESIAN_POINT ( 'NONE',  ( -9.999999999999998224, 5.773502691896259087, -136.3750000000000000 ) ) ;
#42353=CARTESIAN_POINT ( 'NONE',  ( 5.405949406249999534, 9.363379034771803333, -146.7812500020483810 ) ) ;
#42354=DIRECTION ( 'NONE',  ( -0.000000000000000000, -0.000000000000000000, 1.000000000000000000 ) ) ;
#42355=CARTESIAN_POINT ( 'NONE',  ( 5.000000000000000000, 8.660254037844385522, -111.6250000040967763 ) ) ;
#42357=ORIENTED_EDGE ( 'NONE', *, *, #27427, .F. ) ;
#42360=CARTESIAN_POINT ( 'NONE',  ( -9.999999999999479527, -5.773502691896549521, -49.12499999999995737 ) ) ;
#42361=CARTESIAN_POINT ( 'NONE',  ( 10.81189881249999907, 6.242252689847868297, -175.4062500020484094 ) ) ;
#42362=CARTESIAN_POINT ( 'NONE',  ( -2.121150477449813534E-15, -11.54700538379251284, -47.75000000409676204 ) ) ;
#42365=VECTOR ( 'NONE', #34223, 1000.000000000000000 ) ;
#42366=CARTESIAN_POINT ( 'NONE',  ( 9.999999999999998224, 0.000000000000000000, -76.99999999999998579 ) ) ;
#42367=CARTESIAN_POINT ( 'NONE',  ( -5.405949406249996869, 9.363379034771805109, -163.0312500020484094 ) ) ;
#42368=CARTESIAN_POINT ( 'NONE',  ( 5.405949406249999534, 9.363379034771803333, -140.5937500020483810 ) ) ;
#42369=CARTESIAN_POINT ( 'NONE',  ( 9.999999999999479527, 5.773502691896553074, -100.8749999999999716 ) ) ;
#42370=CYLINDRICAL_SURFACE ( 'NONE', #22711, 9.999999999999998224 ) ;
#42372=CARTESIAN_POINT ( 'NONE',  ( 0.000000000000000000, 0.000000000000000000, -200.0000000000000000 ) ) ;
#42373=CARTESIAN_POINT ( 'NONE',  ( 5.405949406249992428, -9.363379034771808662, -72.28125000204838102 ) ) ;
#42374=ORIENTED_EDGE ( 'NONE', *, *, #37263, .F. ) ;
#42376=CARTESIAN_POINT ( 'NONE',  ( -10.81189881249999729, 1.324075727343319199E-15, -122.0937500020483952 ) ) ;
#42378=ORIENTED_EDGE ( 'NONE', *, *, #36968, .F. ) ;
#42379=AXIS2_PLACEMENT_3D ( 'NONE', #38065, #11075, #31390 ) ;
#42380=( BOUNDED_CURVE ( )  B_SPLINE_CURVE ( 2, ( #20141, #13643, #26835, #39987, #7192, #34604, #11270 ),
 .UNSPECIFIED., .F., .F. ) 
 B_SPLINE_CURVE_WITH_KNOTS ( ( 3, 2, 2, 3 ),
 ( 0.2388059701492538378, 0.2400497512437811953, 0.2412935323383085806, 0.2425373134328359381 ),
 .UNSPECIFIED. ) 
 CURVE ( )  GEOMETRIC_REPRESENTATION_ITEM ( )  RATIONAL_B_SPLINE_CURVE ( ( 0.9999999999999880096, 0.8660254037844506980, 1.000000000000000000, 0.8660254037844387076, 1.000000000000000000, 0.8660254037844267172, 1.000000000000011990 ) ) 
 REPRESENTATION_ITEM ( '' )  );
#42381=CARTESIAN_POINT ( 'NONE',  ( 5.405949406249999534, 9.363379034771803333, -32.59375000204836681 ) ) ;
#42382=FACE_OUTER_BOUND ( 'NONE', #2049, .T. ) ;
#42383=CARTESIAN_POINT ( 'NONE',  ( 10.81189881249999551, -6.242252689847874514, -0.1562500020483646446 ) ) ;
#42384=CARTESIAN_POINT ( 'NONE',  ( -10.81189881249999729, 6.242252689847871849, -56.21875000204837391 ) ) ;
#42385=EDGE_CURVE ( 'NONE', #29474, #5068, #11007, .T. ) ;
#42388=CARTESIAN_POINT ( 'NONE',  ( 5.405949406249999534, 9.363379034771803333, -185.5937500020483810 ) ) ;
#42389=CARTESIAN_POINT ( 'NONE',  ( -10.81189881249999729, 1.324075727343319199E-15, -170.0937500020484094 ) ) ;
#42393=VECTOR ( 'NONE', #26975, 1000.000000000000000 ) ;
#42396=CARTESIAN_POINT ( 'NONE',  ( 5.405949406249992428, -9.363379034771808662, -94.59375000204838102 ) ) ;
#42397=CARTESIAN_POINT ( 'NONE',  ( 9.999999999999998224, 0.000000000000000000, -47.37500000409677625 ) ) ;
#42398=CARTESIAN_POINT ( 'NONE',  ( -10.81189881249999729, 6.242252689847871849, -74.40625000204836681 ) ) ;
#42399=CARTESIAN_POINT ( 'NONE',  ( -2.121150477449813534E-15, -11.54700538379251284, -131.7500000040967905 ) ) ;
#42401=CARTESIAN_POINT ( 'NONE',  ( 10.81189881249999729, 6.242252689847867408, -85.21875000204836681 ) ) ;
#42403=CARTESIAN_POINT ( 'NONE',  ( -2.121150477449813534E-15, -11.54700538379251284, -148.2500000040968189 ) ) ;
#42405=EDGE_CURVE ( 'NONE', #14673, #11901, #27019, .T. ) ;
#42406=ORIENTED_EDGE ( 'NONE', *, *, #12220, .F. ) ;
#42410=LINE ( 'NONE', #6394, #27515 ) ;
#42412=ORIENTED_EDGE ( 'NONE', *, *, #42224, .T. ) ;
#42413=CARTESIAN_POINT ( 'NONE',  ( -9.999999999999998224, 1.224646799147353059E-15, -61.24999999999997158 ) ) ;
#42415=CARTESIAN_POINT ( 'NONE',  ( -2.121150477449813534E-15, -11.54700538379251284, -71.75000000409674783 ) ) ;
#42417=CARTESIAN_POINT ( 'NONE',  ( 9.999999999999998224, 0.000000000000000000, -12.87500000409674783 ) ) ;
#42419=CARTESIAN_POINT ( 'NONE',  ( 5.405949406249992428, -9.363379034771808662, -70.78125000204838102 ) ) ;
#42423=CARTESIAN_POINT ( 'NONE',  ( 0.000000000000000000, 0.000000000000000000, -200.0000000000000000 ) ) ;
#42424=CARTESIAN_POINT ( 'NONE',  ( 5.405949406249992428, -9.363379034771808662, -181.7812500020483810 ) ) ;
#42428=CARTESIAN_POINT ( 'NONE',  ( -9.999999999999998224, 1.224646799147353059E-15, -28.62500000409676204 ) ) ;
#42429=CARTESIAN_POINT ( 'NONE',  ( -9.999999999999998224, 1.224646799147353059E-15, -200.0000000000000000 ) ) ;
#42430=CARTESIAN_POINT ( 'NONE',  ( 9.999999999999998224, 0.000000000000000000, -176.0000000000000000 ) ) ;
#42431=CARTESIAN_POINT ( 'NONE',  ( -9.999999999999996447, 5.773502691896259975, -166.3750000000000000 ) ) ;
#42432=CARTESIAN_POINT ( 'NONE',  ( -5.405949406250003975, -9.363379034771801557, -96.53125000204839523 ) ) ;
#42433=ORIENTED_EDGE ( 'NONE', *, *, #19089, .F. ) ;
#42436=ORIENTED_EDGE ( 'NONE', *, *, #2377, .T. ) ;
#42438=ADVANCED_FACE ( 'NONE', ( #19145 ), #25429, .T. ) ;
#42439=CARTESIAN_POINT ( 'NONE',  ( -10.81189881249999729, 6.242252689847871849, -35.21875000204835260 ) ) ;
#42440=CARTESIAN_POINT ( 'NONE',  ( 7.644554776091147741E-16, 12.48450537969573659, -32.65625000204835970 ) ) ;
#42442=CARTESIAN_POINT ( 'NONE',  ( -2.293366432827344421E-15, -12.48450537969573659, -82.71875000204838102 ) ) ;
#42443=FACE_OUTER_BOUND ( 'NONE', #4390, .T. ) ;
#42444=CARTESIAN_POINT ( 'NONE',  ( 5.405949406249999534, 9.363379034771803333, -193.0937500020484094 ) ) ;
#42447=CARTESIAN_POINT ( 'NONE',  ( -9.999999999999479527, -5.773502691896549521, -144.0000000040967620 ) ) ;
#42449=CARTESIAN_POINT ( 'NONE',  ( -10.00000000000000000, -5.773502691896251982, -12.00000000409676915 ) ) ;
#42450=CARTESIAN_POINT ( 'NONE',  ( 9.999999999999998224, 0.000000000000000000, -79.99999999999998579 ) ) ;
#42451=CARTESIAN_POINT ( 'NONE',  ( 10.81189881249999551, -6.242252689847874514, -130.4687500020483810 ) ) ;
#42452=CARTESIAN_POINT ( 'NONE',  ( -10.81189881249999907, -6.242252689847864744, -99.65625000204839523 ) ) ;
#42453=CARTESIAN_POINT ( 'NONE',  ( -5.405949406249996869, 9.363379034771805109, -105.8437500020483810 ) ) ;
#42456=CARTESIAN_POINT ( 'NONE',  ( 9.999999999999998224, 0.000000000000000000, -173.3750000040968189 ) ) ;
#42457=CARTESIAN_POINT ( 'NONE',  ( -9.999999999999998224, 1.224646799147353059E-15, -45.12500000409677625 ) ) ;
#42464=ADVANCED_FACE ( 'NONE', ( #9015 ), #12028, .T. ) ;
#42465=CARTESIAN_POINT ( 'NONE',  ( -10.00000000000000000, -5.773502691896251982, -82.12499999999998579 ) ) ;
#42467=CARTESIAN_POINT ( 'NONE',  ( -2.121150477449813534E-15, -11.54700538379251284, -98.75000000409677625 ) ) ;
#42470=CARTESIAN_POINT ( 'NONE',  ( 10.81189881249999551, -6.242252689847874514, -91.65625000204838102 ) ) ;
#42471=ORIENTED_EDGE ( 'NONE', *, *, #7221, .F. ) ;
#42474=ORIENTED_EDGE ( 'NONE', *, *, #3634, .T. ) ;
#42475=CARTESIAN_POINT ( 'NONE',  ( -9.999999999999998224, 5.773502691896259087, -14.87499999999997335 ) ) ;
#42476=CARTESIAN_POINT ( 'NONE',  ( 7.070501591499377789E-16, 11.54700538379251284, -151.6250000000000000 ) ) ;
#42481=CARTESIAN_POINT ( 'NONE',  ( -5.405949406250003975, -9.363379034771801557, -120.5312500020483952 ) ) ;
#42483=CARTESIAN_POINT ( 'NONE',  ( -9.999999999999998224, 1.224646799147353059E-15, -117.1250000040967905 ) ) ;
#42485=CARTESIAN_POINT ( 'NONE',  ( 10.81189881249999551, -6.242252689847874514, -52.65625000204837391 ) ) ;
#42487=CARTESIAN_POINT ( 'NONE',  ( -5.405949406249996869, 9.363379034771805109, -99.84375000204838102 ) ) ;
#42488=ORIENTED_EDGE ( 'NONE', *, *, #25736, .F. ) ;
#42490=CARTESIAN_POINT ( 'NONE',  ( 9.999999999999998224, 0.000000000000000000, -78.49999999999998579 ) ) ;
#42492=CARTESIAN_POINT ( 'NONE',  ( -10.81189881249999907, -6.242252689847864744, -0.4687500020483501006 ) ) ;
#42493=FACE_OUTER_BOUND ( 'NONE', #27696, .T. ) ;
#42494=CARTESIAN_POINT ( 'NONE',  ( 10.81189881249999729, 0.000000000000000000, -133.3437500020484094 ) ) ;
#42498=CARTESIAN_POINT ( 'NONE',  ( 10.00000000000000000, 5.773502691896255534, -197.2500000040968189 ) ) ;
#42500=CARTESIAN_POINT ( 'NONE',  ( -5.405949406250003975, -9.363379034771801557, -185.0312500020484094 ) ) ;
#42501=CARTESIAN_POINT ( 'NONE',  ( 10.00000000000031619, -5.773502691896077010, -185.5000000040967905 ) ) ;
#42504=EDGE_CURVE ( 'NONE', #34637, #36657, #33076, .T. ) ;
#42505=CARTESIAN_POINT ( 'NONE',  ( -10.81189881249999729, -6.242252689847864744, -61.96875000204838813 ) ) ;
#42506=CARTESIAN_POINT ( 'NONE',  ( 7.644554776091147741E-16, 12.48450537969573659, -48.96875000204835970 ) ) ;
#42507=DESIGN_CONTEXT ( 'detailed design', #844, 'design' ) ;
#42509=CARTESIAN_POINT ( 'NONE',  ( -2.293366432827344421E-15, -12.48450537969573659, -15.40625000204837391 ) ) ;
#42513=EDGE_CURVE ( 'NONE', #41090, #28241, #9435, .T. ) ;
#42514=CARTESIAN_POINT ( 'NONE',  ( 9.999999999999996447, -5.773502691896262640, -111.6249999999999858 ) ) ;
#42519=CARTESIAN_POINT ( 'NONE',  ( -10.81189881249999729, 1.324075727343319199E-15, -114.7812500020483952 ) ) ;
#42520=ORIENTED_EDGE ( 'NONE', *, *, #2395, .F. ) ;
#42521=( BOUNDED_CURVE ( )  B_SPLINE_CURVE ( 2, ( #7464, #37025, #37229, #4437, #36812, #4012, #10473 ),
 .UNSPECIFIED., .F., .F. ) 
 B_SPLINE_CURVE_WITH_KNOTS ( ( 3, 2, 2, 3 ),
 ( 0.5485074626865672487, 0.5497512437810946340, 0.5509950248756221303, 0.5522388059701495155 ),
 .UNSPECIFIED. ) 
 CURVE ( )  GEOMETRIC_REPRESENTATION_ITEM ( )  RATIONAL_B_SPLINE_CURVE ( ( 0.9999999999999880096, 0.8660254037844506980, 1.000000000000000000, 0.8660254037844387076, 1.000000000000000000, 0.8660254037844148378, 1.000000000000023981 ) ) 
 REPRESENTATION_ITEM ( '' )  );
#42522=CARTESIAN_POINT ( 'NONE',  ( -9.999999999999998224, 1.224646799147353059E-15, -196.6250000040967905 ) ) ;
#42524=CARTESIAN_POINT ( 'NONE',  ( 0.000000000000000000, 0.000000000000000000, -200.0000000000000000 ) ) ;
#42526=EDGE_LOOP ( 'NONE', ( #38212, #17302, #4494, #21598 ) ) ;
#42527=CARTESIAN_POINT ( 'NONE',  ( 10.00000000000000000, 5.773502691896255534, -40.87499999999997158 ) ) ;
#42528=CARTESIAN_POINT ( 'NONE',  ( 9.999999999999998224, 0.000000000000000000, -17.37500000409675138 ) ) ;
#42529=CARTESIAN_POINT ( 'NONE',  ( 10.81189881249999729, 0.000000000000000000, -45.03125000204838102 ) ) ;
#42530=CARTESIAN_POINT ( 'NONE',  ( 7.070501591499376803E-16, 11.54700538379251284, -16.62499999999996447 ) ) ;
#42535=CARTESIAN_POINT ( 'NONE',  ( 10.81189881249999729, 0.000000000000000000, -136.5312500020484094 ) ) ;
#42536=CARTESIAN_POINT ( 'NONE',  ( -2.293366432827344421E-15, -12.48450537969573659, -153.4062500020483810 ) ) ;
#42537=EDGE_CURVE ( 'NONE', #14343, #14344, #19824, .T. ) ;
#42538=CARTESIAN_POINT ( 'NONE',  ( 9.999999999999998224, 0.000000000000000000, -192.5000000000000000 ) ) ;
#42539=ORIENTED_EDGE ( 'NONE', *, *, #27350, .F. ) ;
#42540=ORIENTED_EDGE ( 'NONE', *, *, #10106, .F. ) ;
#42541=ADVANCED_FACE ( 'NONE', ( #26267 ), #792, .T. ) ;
#42542=EDGE_LOOP ( 'NONE', ( #22392, #37837, #20927, #7845 ) ) ;
#42543=EDGE_CURVE ( 'NONE', #7196, #31273, #36181, .T. ) ;
#42544=LINE ( 'NONE', #23135, #33203 ) ;
#42545=CARTESIAN_POINT ( 'NONE',  ( -10.81189881249999907, -6.242252689847864744, -175.9687500020483526 ) ) ;
#42546=CARTESIAN_POINT ( 'NONE',  ( -2.293366432827344421E-15, -12.48450537969573659, -22.71875000204837747 ) ) ;
#42548=CARTESIAN_POINT ( 'NONE',  ( -5.405949406249996869, 9.363379034771805109, -155.3437500020483810 ) ) ;
#42549=CARTESIAN_POINT ( 'NONE',  ( 7.644554776091147741E-16, 12.48450537969573659, -144.9687500020483810 ) ) ;
#42553=CARTESIAN_POINT ( 'NONE',  ( 10.81189881249999551, -6.242252689847874514, -20.96875000204836681 ) ) ;
#42555=CARTESIAN_POINT ( 'NONE',  ( -9.999999999999998224, 1.224646799147353059E-15, -88.62500000409677625 ) ) ;
#42556=CARTESIAN_POINT ( 'NONE',  ( 5.000000000000000000, 8.660254037844385522, -120.2500000000000000 ) ) ;
#42559=CARTESIAN_POINT ( 'NONE',  ( -10.81189881249999907, -6.242252689847864744, -69.46875000204838102 ) ) ;
#42560=CARTESIAN_POINT ( 'NONE',  ( -2.293366432827344421E-15, -12.48450537969573659, -52.90625000204837391 ) ) ;
#42562=CARTESIAN_POINT ( 'NONE',  ( -4.999999999999996447, 8.660254037844387298, -56.99999999999996447 ) ) ;
#42564=EDGE_CURVE ( 'NONE', #21267, #23881, #6855, .T. ) ;
#42565=CARTESIAN_POINT ( 'NONE',  ( 9.999999999999996447, -5.773502691896262640, -137.1250000000000000 ) ) ;
#42566=CARTESIAN_POINT ( 'NONE',  ( 10.81189881249999729, 0.000000000000000000, -136.5312500020484094 ) ) ;
#42567=CARTESIAN_POINT ( 'NONE',  ( -2.121150477449813534E-15, -11.54700538379251284, -150.8750000000000000 ) ) ;
#42568=CARTESIAN_POINT ( 'NONE',  ( 10.00000000000000000, 5.773502691896255534, -110.2500000040967905 ) ) ;
#42570=ADVANCED_FACE ( 'NONE', ( #19772 ), #164, .T. ) ;
#42571=ORIENTED_EDGE ( 'NONE', *, *, #35671, .T. ) ;
#42574=CARTESIAN_POINT ( 'NONE',  ( 9.999999999999998224, 0.000000000000000000, -21.87500000409675494 ) ) ;
#42575=EDGE_CURVE ( 'NONE', #10245, #13289, #20408, .T. ) ;
#42576=CARTESIAN_POINT ( 'NONE',  ( -5.405949406249996869, 9.363379034771805109, -173.5312500020484094 ) ) ;
#42577=CARTESIAN_POINT ( 'NONE',  ( -9.999999999999998224, 5.773502691896259087, -42.25000000409674783 ) ) ;
#42578=CARTESIAN_POINT ( 'NONE',  ( 0.000000000000000000, 0.000000000000000000, -200.0000000000000000 ) ) ;
#42580=CARTESIAN_POINT ( 'NONE',  ( 7.070501591499376803E-16, 11.54700538379251284, -156.1250000000000000 ) ) ;
#42581=CARTESIAN_POINT ( 'NONE',  ( -5.405949406249996869, 9.363379034771805109, -164.5312500020484094 ) ) ;
#42582=CARTESIAN_POINT ( 'NONE',  ( 10.81189881249999729, 0.000000000000000000, -143.8437500020483810 ) ) ;
#42584=DIRECTION ( 'NONE',  ( 1.000000000000000000, 0.000000000000000000, 0.000000000000000000 ) ) ;
#42585=CARTESIAN_POINT ( 'NONE',  ( -4.999999999999996447, 8.660254037844387298, -150.0000000000000000 ) ) ;
#42586=ORIENTED_EDGE ( 'NONE', *, *, #34175, .T. ) ;
#42588=EDGE_CURVE ( 'NONE', #38971, #26946, #37483, .T. ) ;
#42589=CARTESIAN_POINT ( 'NONE',  ( -5.405949406250003975, -9.363379034771801557, -69.53125000204838102 ) ) ;
#42590=VERTEX_POINT ( 'NONE', #36398 ) ;
#42592=CARTESIAN_POINT ( 'NONE',  ( -2.293366432827344421E-15, -12.48450537969573659, -117.2187500020483952 ) ) ;
#42595=ORIENTED_EDGE ( 'NONE', *, *, #41763, .F. ) ;
#42596=CARTESIAN_POINT ( 'NONE',  ( -10.81189881249999729, 6.242252689847871849, -20.21875000204836326 ) ) ;
#42597=CARTESIAN_POINT ( 'NONE',  ( 10.81189881249999729, 0.000000000000000000, -0.03125000204837191653 ) ) ;
#42598=CARTESIAN_POINT ( 'NONE',  ( -5.405949406250003975, -9.363379034771801557, -48.34375000204838102 ) ) ;
#42599=LINE ( 'NONE', #3340, #24690 ) ;
#42601=CARTESIAN_POINT ( 'NONE',  ( -10.81189881249999729, -6.242252689847864744, -184.9687500020484094 ) ) ;
#42602=CARTESIAN_POINT ( 'NONE',  ( -2.293366432827344421E-15, -12.48450537969573659, -171.2187500020484094 ) ) ;
#42605=CARTESIAN_POINT ( 'NONE',  ( -9.999999999999998224, 1.224646799147353059E-15, -40.62500000409677625 ) ) ;
#42607=CARTESIAN_POINT ( 'NONE',  ( 7.644554776091147741E-16, 12.48450537969573659, -96.96875000204838102 ) ) ;
#42608=DIRECTION ( 'NONE',  ( 1.000000000000000000, 0.000000000000000000, 0.000000000000000000 ) ) ;
#42609=CARTESIAN_POINT ( 'NONE',  ( -10.81189881249999729, 1.324075727343319199E-15, -74.28125000204838102 ) ) ;
#42610=CARTESIAN_POINT ( 'NONE',  ( 9.999999999999998224, 0.000000000000000000, -89.37500000409677625 ) ) ;
#42612=CARTESIAN_POINT ( 'NONE',  ( -5.405949406250003975, -9.363379034771801557, -162.5312500020484094 ) ) ;
#42614=CARTESIAN_POINT ( 'NONE',  ( -9.999999999999998224, 1.224646799147353059E-15, -139.6250000040967905 ) ) ;
#42619=CARTESIAN_POINT ( 'NONE',  ( -5.405949406249996869, 9.363379034771805109, -199.0312500020484094 ) ) ;
#42621=EDGE_LOOP ( 'NONE', ( #38100, #9380, #29985, #5506 ) ) ;
#42622=CARTESIAN_POINT ( 'NONE',  ( -9.999999999999998224, 1.224646799147353059E-15, -53.74999999999996447 ) ) ;
#42624=CARTESIAN_POINT ( 'NONE',  ( 4.999999999999992006, -8.660254037844389075, -67.12500000409676204 ) ) ;
#42625=CYLINDRICAL_SURFACE ( 'NONE', #7949, 9.999999999999998224 ) ;
#42628=CARTESIAN_POINT ( 'NONE',  ( -5.405949406249996869, 9.363379034771805109, -68.53125000204838102 ) ) ;
#42631=CARTESIAN_POINT ( 'NONE',  ( 9.999999999998969713, 5.773502691896851502, -38.25000000409674072 ) ) ;
#42632=CARTESIAN_POINT ( 'NONE',  ( 5.405949406249992428, -9.363379034771808662, -187.7812500020484094 ) ) ;
#42633=EDGE_CURVE ( 'NONE', #12497, #24317, #16787, .T. ) ;
#42635=CARTESIAN_POINT ( 'NONE',  ( 7.295574285832478800, -8.272403601877444501, -0.05005682399628019752 ) ) ;
#42636=CARTESIAN_POINT ( 'NONE',  ( -11.54700538379250396, -20.00000000000000355, 0.000000000000000000 ) ) ;
#42637=CARTESIAN_POINT ( 'NONE',  ( -9.886419945013566135, -1.735418534722659389, -0.000000000000000000 ) ) ;
#42638=CARTESIAN_POINT ( 'NONE',  ( 9.999999999999998224, 0.000000000000000000, -122.3750000040967905 ) ) ;
#42640=CARTESIAN_POINT ( 'NONE',  ( -10.00000000000000000, -5.773502691896251982, -170.6250000000000284 ) ) ;
#42641=CARTESIAN_POINT ( 'NONE',  ( 7.070501591499376803E-16, 11.54700538379251284, -1.624999999999975575 ) ) ;
#42642=CARTESIAN_POINT ( 'NONE',  ( -10.81189881249999907, -6.242252689847864744, -92.15625000204839523 ) ) ;
#42643=ORIENTED_EDGE ( 'NONE', *, *, #40051, .F. ) ;
#42644=DIRECTION ( 'NONE',  ( -0.000000000000000000, -0.000000000000000000, 1.000000000000000000 ) ) ;
#42645=FACE_OUTER_BOUND ( 'NONE', #17314, .T. ) ;
#42646=ORIENTED_EDGE ( 'NONE', *, *, #4837, .F. ) ;
#42647=ORIENTED_EDGE ( 'NONE', *, *, #41568, .T. ) ;
#42648=EDGE_CURVE ( 'NONE', #26059, #5330, #21212, .T. ) ;
#42649=CARTESIAN_POINT ( 'NONE',  ( 5.405949406249992428, -9.363379034771808662, -31.59375000204836681 ) ) ;
#42650=CARTESIAN_POINT ( 'NONE',  ( -2.293366432827344421E-15, -12.48450537969573659, -21.40625000204837036 ) ) ;
#42652=AXIS2_PLACEMENT_3D ( 'NONE', #12208, #25401, #34481 ) ;
#42653=CARTESIAN_POINT ( 'NONE',  ( 10.81189881249999729, 0.000000000000000000, -67.34375000204836681 ) ) ;
#42654=CARTESIAN_POINT ( 'NONE',  ( 9.999999999999998224, 0.000000000000000000, -200.0000000000000000 ) ) ;
#42655=CARTESIAN_POINT ( 'NONE',  ( 5.405949406249999534, 9.363379034771803333, -191.5937500020484094 ) ) ;
#42656=CARTESIAN_POINT ( 'NONE',  ( 9.999999999999479527, 5.773502691896553074, -72.75000000409673362 ) ) ;
#42658=CARTESIAN_POINT ( 'NONE',  ( -9.999999999999998224, 1.224646799147353059E-15, -144.1250000040967905 ) ) ;
#42660=CARTESIAN_POINT ( 'NONE',  ( -2.121150477449813534E-15, -11.54700538379251284, -7.250000004096746054 ) ) ;
#42661=CARTESIAN_POINT ( 'NONE',  ( -5.000000000000003553, -8.660254037844383745, -103.3750000040967763 ) ) ;
#42662=CARTESIAN_POINT ( 'NONE',  ( -5.405949406250003975, -9.363379034771801557, -118.8437500020483810 ) ) ;
#42663=CARTESIAN_POINT ( 'NONE',  ( 10.81189881249999907, 6.242252689847868297, -98.90625000204839523 ) ) ;
#42664=CARTESIAN_POINT ( 'NONE',  ( 7.644554776091147741E-16, 12.48450537969573659, -111.9687500020483668 ) ) ;
#42667=CARTESIAN_POINT ( 'NONE',  ( 9.999999999999996447, -5.773502691896262640, -161.5000000040968189 ) ) ;
#42668=CYLINDRICAL_SURFACE ( 'NONE', #1341, 9.999999999999998224 ) ;
#42672=CARTESIAN_POINT ( 'NONE',  ( -5.000000000000003553, -8.660254037844383745, -157.0000000000000000 ) ) ;
#42674=CARTESIAN_POINT ( 'NONE',  ( -9.999999999999998224, 1.224646799147353059E-15, -127.2499999999999716 ) ) ;
#42676=CARTESIAN_POINT ( 'NONE',  ( 9.999999999999998224, 0.000000000000000000, -84.49999999999997158 ) ) ;
#42678=CARTESIAN_POINT ( 'NONE',  ( -9.999999999999998224, 5.773502691896259087, -99.25000000409677625 ) ) ;
#42681=CARTESIAN_POINT ( 'NONE',  ( -10.81189881249999729, 1.324075727343319199E-15, -90.78125000204838102 ) ) ;
#42682=EDGE_LOOP ( 'NONE', ( #6804, #22029, #13016, #6364 ) ) ;
#42683=EDGE_CURVE ( 'NONE', #21484, #34431, #14771, .T. ) ;
#42687=ORIENTED_EDGE ( 'NONE', *, *, #14286, .F. ) ;
#42688=CARTESIAN_POINT ( 'NONE',  ( -9.999999999999998224, 1.224646799147353059E-15, -13.24999999999995559 ) ) ;
#42690=ADVANCED_FACE ( 'NONE', ( #5088 ), #37235, .T. ) ;
#42732=COLOUR_RGB('Black', 0.08235294, 0.09019608, 0.10196078);
#42733=FILL_AREA_STYLE_COLOUR('',#42732);
#42734=FILL_AREA_STYLE('',(#42733));
#42735=SURFACE_STYLE_FILL_AREA(#42734);
#42736=SURFACE_SIDE_STYLE('',(#42735));
#42737=SURFACE_STYLE_USAGE(.BOTH.,#42736);
#42738=PRESENTATION_STYLE_ASSIGNMENT((#42737));
#42749=STYLED_ITEM('',(#42738),#30024);
#42750=MECHANICAL_DESIGN_GEOMETRIC_PRESENTATION_REPRESENTATION('',(#42749),#15874);
ENDSEC;
END-ISO-10303-21;
